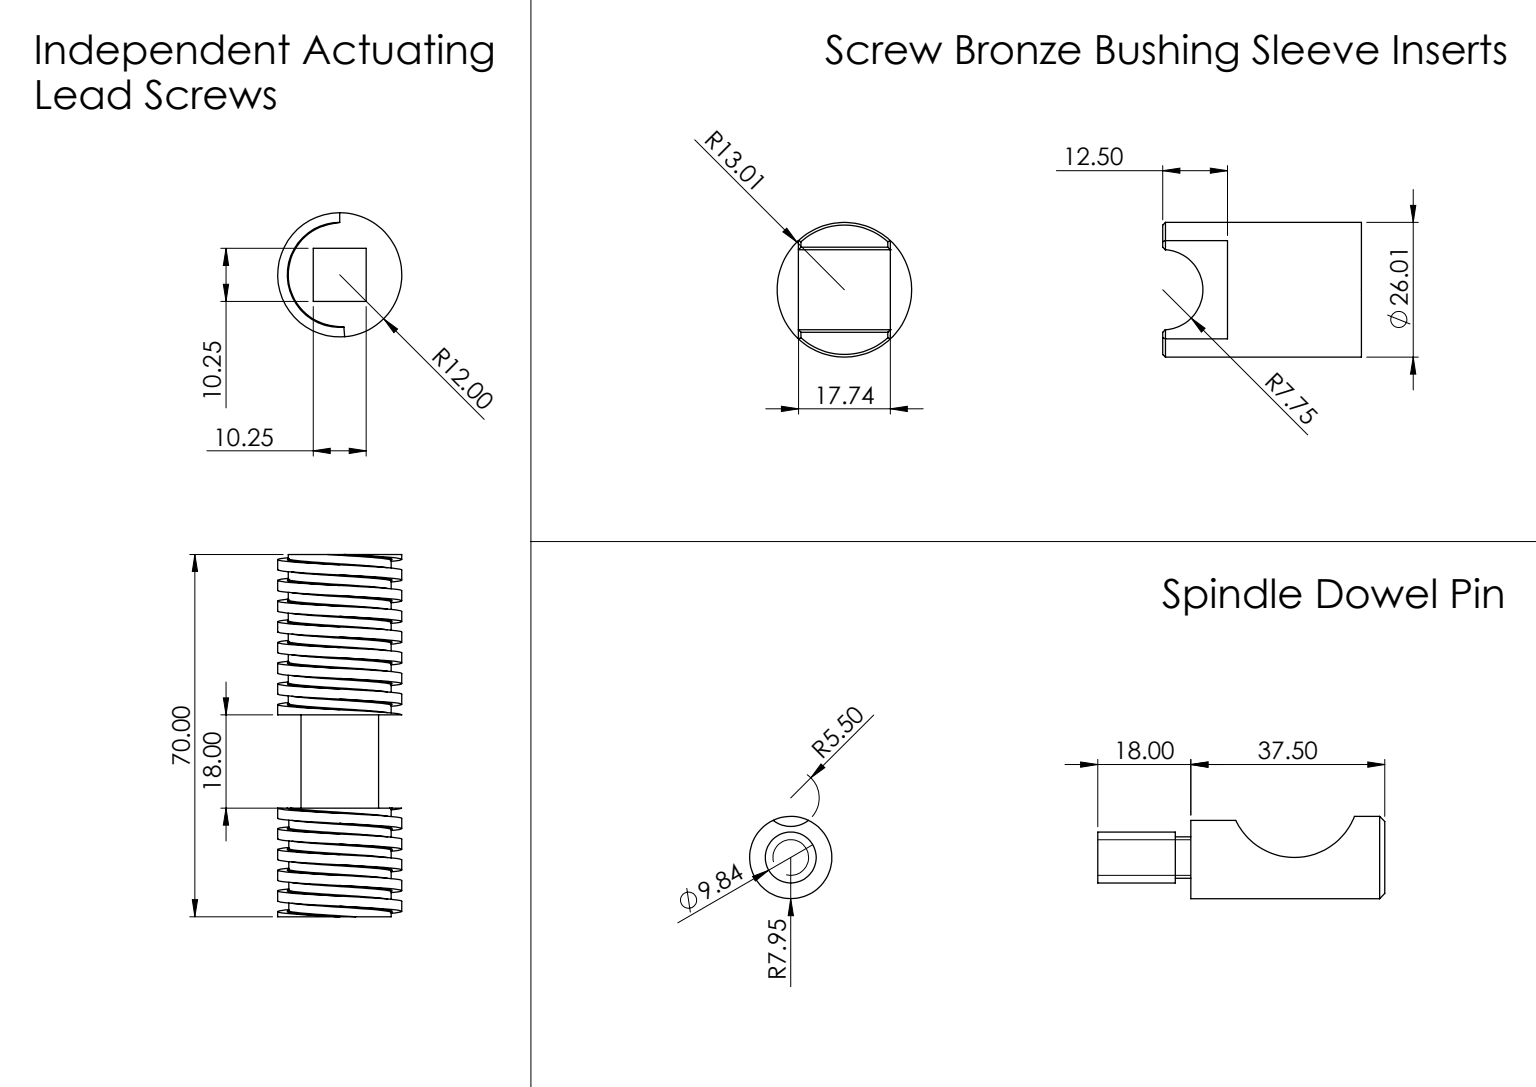
ISO-10303-21;
HEADER;
FILE_DESCRIPTION (('STEP AP214'),
    '1' );
FILE_NAME ('Independent Actuating Lead Screws.step',
    '2026-10-09T08:48:44',
    ( '' ),
    ( '' ),
    'SwSTEP 2.0',
    'SolidWorks 2026',
    '' );
FILE_SCHEMA (( 'AUTOMOTIVE_DESIGN' ));
ENDSEC;

DATA;
#1=( BOUNDED_CURVE ( )  B_SPLINE_CURVE ( 2, ( #10533, #60209, #55118, #80827, #73261, #48394, #10118, #21906, #55527, #48810, #23141, #53876, #74509 ),
 .UNSPECIFIED., .F., .F. ) 
 B_SPLINE_CURVE_WITH_KNOTS ( ( 3, 2, 2, 2, 2, 2, 3 ),
 ( 0.7124999999999999112, 0.7166666666666665630, 0.7208333333333332149, 0.7249999999999998668, 0.7291666666666665186, 0.7333333333333331705, 0.7374999999999999334 ),
 .UNSPECIFIED. ) 
 CURVE ( )  GEOMETRIC_REPRESENTATION_ITEM ( )  RATIONAL_B_SPLINE_CURVE ( ( 1.000000000000000888, 0.9659258262890674240, 1.000000000000000000, 0.9659258262890683122, 1.000000000000000000, 0.9659258262890683122, 1.000000000000000000, 0.9659258262890683122, 1.000000000000000000, 0.9659258262890683122, 1.000000000000000000, 0.9659258262890692004, 0.9999999999999991118 ) ) 
 REPRESENTATION_ITEM ( '' )  );
#2=CARTESIAN_POINT ( 'NONE',  ( 0.3392501089628018329, 0.1958661417322835607, -1.790682414698162805 ) ) ;
#8=CARTESIAN_POINT ( 'NONE',  ( 0.4091458600556403535, 0.2362204724409449896, -1.625328083989501460 ) ) ;
#11=CARTESIAN_POINT ( 'NONE',  ( 0.3949938075777409408, -0.1058382717557499186, -1.133202099737532720 ) ) ;
#20=CARTESIAN_POINT ( 'NONE',  ( 0.1070741851644053388, 0.3996062992125986035, -1.959973753280839892 ) ) ;
#23=CARTESIAN_POINT ( 'NONE',  ( -0.1958661417322834497, -0.3392501089628018884, -1.562972810202412521 ) ) ;
#34=CARTESIAN_POINT ( 'NONE',  ( 0.3996062992125986035, -0.1070741851644052972, -0.03083989501312336262 ) ) ;
#36=CARTESIAN_POINT ( 'NONE',  ( 0.1958661417322836440, -0.3392501089628017219, -0.9639107611548557442 ) ) ;
#40=DIRECTION ( 'NONE',  ( 0.000000000000000000, 0.000000000000000000, 1.000000000000000000 ) ) ;
#45=CARTESIAN_POINT ( 'NONE',  ( 0.4091458600556404646, -0.2362204724409448231, -2.624671916010498762 ) ) ;
#52=CARTESIAN_POINT ( 'NONE',  ( 0.4724409448818898682, 2.892866454678787531E-17, -2.322834645669291209 ) ) ;
#56=CARTESIAN_POINT ( 'NONE',  ( 0.2867679344610366554, -0.2867679344610365444, -2.610236220472440749 ) ) ;
#59=CARTESIAN_POINT ( 'NONE',  ( 5.785732909357575061E-17, -0.4724409448818898682, -0.3937007874015748254 ) ) ;
#60=CARTESIAN_POINT ( 'NONE',  ( -0.1070741851644051862, -0.3996062992125987146, -0.07217847769028871985 ) ) ;
#63=CARTESIAN_POINT ( 'NONE',  ( -0.1049643490035302024, -0.3917322834645671215, -1.796587926509185973 ) ) ;
#64=EDGE_LOOP ( 'NONE', ( #43919, #18024, #48228, #40467 ) ) ;
#66=CARTESIAN_POINT ( 'NONE',  ( -0.4724409448818898682, -8.678599364036362592E-17, -2.716535433070865757 ) ) ;
#74=CARTESIAN_POINT ( 'NONE',  ( 4.797336870675655290E-17, -0.3917322834645669549, -0.9461749099399457963 ) ) ;
#81=CARTESIAN_POINT ( 'NONE',  ( 0.1049643490035304799, -0.3917322834645670104, -2.444245037566615597 ) ) ;
#89=CARTESIAN_POINT ( 'NONE',  ( -0.1049643490035302024, -0.3917322834645671215, -1.416666666666666519 ) ) ;
#104=CARTESIAN_POINT ( 'NONE',  ( -0.3392501089628019995, 0.1958661417322832277, -1.213254593175852936 ) ) ;
#105=CARTESIAN_POINT ( 'NONE',  ( -0.4091458600556405756, 0.2362204724409446288, -0.1030183727034120617 ) ) ;
#108=CARTESIAN_POINT ( 'NONE',  ( 0.2891555358219910499, 0.2891555358219910499, 0.1003937007874015630 ) ) ;
#113=CARTESIAN_POINT ( 'NONE',  ( -0.3949938075777409963, -7.255918531996591613E-17, 0.04133858267716533641 ) ) ;
#120=CARTESIAN_POINT ( 'NONE',  ( -9.787531504996566615E-17, 0.3996062992125985480, -0.7066929133858268486 ) ) ;
#122=CARTESIAN_POINT ( 'NONE',  ( -0.3392501089628017219, -0.1958661417322836718, -0.6745406824146981117 ) ) ;
#124=DIRECTION ( 'NONE',  ( 1.000000000000000000, 0.000000000000000000, -0.000000000000000000 ) ) ;
#139=CARTESIAN_POINT ( 'NONE',  ( -0.2362204724409447953, -0.4091458600556404646, -2.347112860892388575 ) ) ;
#159=CARTESIAN_POINT ( 'NONE',  ( 0.1070741851644053666, 0.3996062992125986035, -0.4658792650918635037 ) ) ;
#160=CARTESIAN_POINT ( 'NONE',  ( -0.1070741851644051862, -0.3996062992125986590, -2.668635170603674833 ) ) ;
#165=CARTESIAN_POINT ( 'NONE',  ( 0.2925321140481932369, 0.2925321140481932369, -2.342519685039369914 ) ) ;
#166=CARTESIAN_POINT ( 'NONE',  ( 0.3420746716998660508, -0.1974969037888703871, -1.994750656167979086 ) ) ;
#167=CARTESIAN_POINT ( 'NONE',  ( -0.3917322834645671215, 0.1049643490035301469, -0.4973753280839895430 ) ) ;
#168=CARTESIAN_POINT ( 'NONE',  ( -1.157146581871515012E-16, 0.4724409448818898682, -2.519685039370078705 ) ) ;
#169=CARTESIAN_POINT ( 'NONE',  ( 0.1049643490035304799, -0.3917322834645669549, -0.8648293963254591876 ) ) ;
#172=CARTESIAN_POINT ( 'NONE',  ( -0.3420746716998662729, 0.1974969037888702206, -2.780183727034121866 ) ) ;
#177=CARTESIAN_POINT ( 'NONE',  ( 0.2362204724409451007, -0.4091458600556402980, -2.769028871391076230 ) ) ;
#178=CARTESIAN_POINT ( 'NONE',  ( 0.2925321140481932369, 0.2925321140481932369, -2.185039370078739829 ) ) ;
#179=CARTESIAN_POINT ( 'NONE',  ( -0.3392501089628017219, -0.1958661417322836995, -0.8366334890101857491 ) ) ;
#185=CARTESIAN_POINT ( 'NONE',  ( -0.2867679344610364334, -0.2867679344610367109, -0.1437007874015748810 ) ) ;
#194=CARTESIAN_POINT ( 'NONE',  ( -0.3917322834645670104, -7.196005306013484475E-17, -0.7539370078740157410 ) ) ;
#195=CARTESIAN_POINT ( 'NONE',  ( 0.3917322834645669549, 0.1049643490035304660, -1.691601049868766360 ) ) ;
#196=CARTESIAN_POINT ( 'NONE',  ( -0.3917322834645671215, 0.1049643490035301469, -2.859580052493438274 ) ) ;
#198=CARTESIAN_POINT ( 'NONE',  ( -0.2925321140481930704, -0.2925321140481933480, -0.2165354330708662012 ) ) ;
#202=CARTESIAN_POINT ( 'NONE',  ( -0.3996062992125986035, -0.1070741851644056997, -1.620734908136482799 ) ) ;
#204=CARTESIAN_POINT ( 'NONE',  ( -0.4724409448818899238, 0.1265901696524986964, -2.471784776902886893 ) ) ;
#207=CARTESIAN_POINT ( 'NONE',  ( 0.3392501089628018884, -0.1958661417322834220, -0.6620734908136483021 ) ) ;
#216=CARTESIAN_POINT ( 'NONE',  ( -0.2362204724409447953, -0.4091458600556404646, -2.112860892388451539 ) ) ;
#223=ADVANCED_FACE ( 'NONE', ( #9541 ), #47687, .T. ) ;
#224=CARTESIAN_POINT ( 'NONE',  ( 0.3458507752293908943, -0.3458507752293908943, -2.537401574803149984 ) ) ;
#228=CARTESIAN_POINT ( 'NONE',  ( -0.3917322834645669549, -7.196005306013483243E-17, -0.7493245162391581893 ) ) ;
#231=CARTESIAN_POINT ( 'NONE',  ( 0.1958661417322836440, -0.3392501089628017219, -0.9639107611548557442 ) ) ;
#236=CARTESIAN_POINT ( 'NONE',  ( -0.3392501089628017219, -0.1958661417322836718, -2.879265091863516979 ) ) ;
#240=CARTESIAN_POINT ( 'NONE',  ( -1.157146581871515012E-16, 0.4724409448818898682, -1.021653543307086576 ) ) ;
#253=CARTESIAN_POINT ( 'NONE',  ( -0.3996062992125984925, -0.1070741851644056858, -2.484908136482939955 ) ) ;
#257=CARTESIAN_POINT ( 'NONE',  ( 0.1070741851644053388, 0.3996062992125986035, -1.330052493438320438 ) ) ;
#263=CARTESIAN_POINT ( 'NONE',  ( -0.2925321140481930149, -0.2925321140481933480, -0.7657480314960628531 ) ) ;
#264=CARTESIAN_POINT ( 'NONE',  ( 0.1998031496062994405, -0.3460692066303958092, -0.8792650918635170898 ) ) ;
#265=CARTESIAN_POINT ( 'NONE',  ( 0.3420746716998659953, 0.1974969037888705536, -0.2887139107611549349 ) ) ;
#271=CARTESIAN_POINT ( 'NONE',  ( -0.1974969037888704149, -0.3420746716998661063, -1.244750656167979086 ) ) ;
#276=CARTESIAN_POINT ( 'NONE',  ( -0.3458507752293906723, -0.3458507752293910609, -1.633858267716534973 ) ) ;
#277=CARTESIAN_POINT ( 'NONE',  ( 4.893765752498283924E-17, -0.3996062992125986035, -2.598425196850393970 ) ) ;
#284=CARTESIAN_POINT ( 'NONE',  ( -9.594673741351310580E-17, 0.3917322834645669549, -1.969796957184039909 ) ) ;
#285=CARTESIAN_POINT ( 'NONE',  ( -9.787531504996566615E-17, 0.3996062992125985480, -2.753937007874015741 ) ) ;
#290=CARTESIAN_POINT ( 'NONE',  ( -0.1958661417322834220, -0.3392501089628018884, -1.317585301837270295 ) ) ;
#293=CARTESIAN_POINT ( 'NONE',  ( 0.1974969037888704704, 0.3420746716998660508, -2.034120734908136718 ) ) ;
#298=CARTESIAN_POINT ( 'NONE',  ( -0.1998031496062994683, 0.3460692066303958092, -0.3280839895013123453 ) ) ;
#306=CARTESIAN_POINT ( 'NONE',  ( 0.1049643490035303689, 0.3917322834645670104, -0.5505249343832020470 ) ) ;
#314=CARTESIAN_POINT ( 'NONE',  ( 0.2925321140481932369, -0.2925321140481931814, -2.064960629921259283 ) ) ;
#320=CARTESIAN_POINT ( 'NONE',  ( -0.3458507752293906723, -0.3458507752293910609, -0.8464566929133857665 ) ) ;
#322=CARTESIAN_POINT ( 'NONE',  ( -0.1049643490035302024, -0.3917322834645671215, -0.2217847769028870319 ) ) ;
#323=CARTESIAN_POINT ( 'NONE',  ( 0.3808816823641231752, -0.09156050430092187165, -1.929133858267716661 ) ) ;
#327=CARTESIAN_POINT ( 'NONE',  ( 0.2362204724409451007, -0.4091458600556402980, -2.845800524934383624 ) ) ;
#331=CARTESIAN_POINT ( 'NONE',  ( -0.1058382717557497660, -0.3949938075777411073, -2.668635170603674833 ) ) ;
#339=CARTESIAN_POINT ( 'NONE',  ( 0.2867679344610365999, -0.2867679344610365444, -1.350393700787401619 ) ) ;
#342=CARTESIAN_POINT ( 'NONE',  ( -0.1265901696524993347, 0.4724409448818895907, 0.2316272965879264956 ) ) ;
#354=CARTESIAN_POINT ( 'NONE',  ( 0.3996062992125985480, 2.446882876249141654E-17, -0.9822834645669291653 ) ) ;
#355=CARTESIAN_POINT ( 'NONE',  ( 0.1049643490035303689, 0.3917322834645670104, -2.597769028871390606 ) ) ;
#365=CARTESIAN_POINT ( 'NONE',  ( -0.3996062992125987146, 0.1070741851644051862, 0.1246719160104986790 ) ) ;
#367=CARTESIAN_POINT ( 'NONE',  ( -0.3917322834645670659, -7.196005306013484475E-17, -1.925872334154542509 ) ) ;
#373=CARTESIAN_POINT ( 'NONE',  ( 0.1049643490035303689, 0.3917322834645670104, -1.810367454068241511 ) ) ;
#380=CARTESIAN_POINT ( 'NONE',  ( 0.1998031496062992740, 0.3460692066303959757, -1.404199475065616820 ) ) ;
#382=CARTESIAN_POINT ( 'NONE',  ( 4.797336870675656522E-17, -0.3917322834645670659, 0.08200168159348891761 ) ) ;
#395=CARTESIAN_POINT ( 'NONE',  ( 0.2867679344610365999, -0.2867679344610365444, -0.2480314960629920740 ) ) ;
#398=CARTESIAN_POINT ( 'NONE',  ( -0.3420746716998661618, 0.1974969037888702206, -0.6561679790026245795 ) ) ;
#400=VERTEX_POINT ( 'NONE', #34658 ) ;
#407=CARTESIAN_POINT ( 'NONE',  ( 0.3392501089628018884, -0.1958661417322833942, -1.519048187172915343 ) ) ;
#414=CARTESIAN_POINT ( 'NONE',  ( -0.1070741851644056997, 0.3996062992125986035, -1.266404199475065440 ) ) ;
#416=CARTESIAN_POINT ( 'NONE',  ( 0.1998031496062994128, -0.3460692066303957537, -0.6410761154855643129 ) ) ;
#417=CARTESIAN_POINT ( 'NONE',  ( -0.3460692066303957537, -0.1998031496062994405, -0.2867454068241469534 ) ) ;
#419=CARTESIAN_POINT ( 'NONE',  ( -0.3460692066303960868, 0.1998031496062990242, -2.860892388451443669 ) ) ;
#420=CARTESIAN_POINT ( 'NONE',  ( 0.2867679344610365999, 0.2867679344610365999, -2.269685039370078705 ) ) ;
#426=CARTESIAN_POINT ( 'NONE',  ( -0.4724409448818898682, -8.678599364036362592E-17, -1.375984251968503713 ) ) ;
#430=CARTESIAN_POINT ( 'NONE',  ( 0.1058382717557500852, -0.3949938075777408852, -1.264435695538058013 ) ) ;
#440=CARTESIAN_POINT ( 'NONE',  ( 0.1070741851644053388, 0.3996062992125986035, -2.274934383202099397 ) ) ;
#442=CARTESIAN_POINT ( 'NONE',  ( 0.2867679344610365999, 0.2867679344610365999, -1.477670972932071614 ) ) ;
#450=CARTESIAN_POINT ( 'NONE',  ( 0.1265901696524989184, 0.4724409448818898127, -2.355643044619422533 ) ) ;
#453=CARTESIAN_POINT ( 'NONE',  ( 0.2925321140481932369, -0.2925321140481931814, -0.01771653543307087630 ) ) ;
#455=CARTESIAN_POINT ( 'NONE',  ( 0.1049643490035304938, -0.3917322834645669549, -1.272309711286089273 ) ) ;
#464=CARTESIAN_POINT ( 'NONE',  ( -0.4724409448818898682, 5.785732909357575061E-17, -2.755905511811024056 ) ) ;
#476=CARTESIAN_POINT ( 'NONE',  ( 0.1049643490035303689, 0.3917322834645670104, -2.505249343832020692 ) ) ;
#479=CARTESIAN_POINT ( 'NONE',  ( -0.3458507752293909498, 0.3458507752293907833, -0.8070866141732284671 ) ) ;
#480=CARTESIAN_POINT ( 'NONE',  ( -0.2925321140481930704, -0.2925321140481933480, 0.09842519685039367860 ) ) ;
#484=CARTESIAN_POINT ( 'NONE',  ( -0.3917322834645671215, 0.1049643490035301469, -1.757217847769028340 ) ) ;
#488=CARTESIAN_POINT ( 'NONE',  ( -0.1265901696524986964, -0.4724409448818899238, -2.906824146981627610 ) ) ;
#495=CARTESIAN_POINT ( 'NONE',  ( -0.1958661417322834497, -0.3392501089628018884, -1.248012180281152794 ) ) ;
#503=ORIENTED_EDGE ( 'NONE', *, *, #38239, .F. ) ;
#504=CARTESIAN_POINT ( 'NONE',  ( 0.1958661417322834775, 0.3392501089628018884, -2.503300155676852157 ) ) ;
#513=CARTESIAN_POINT ( 'NONE',  ( -0.1958661417322834220, -0.3392501089628018884, -1.725065616797900381 ) ) ;
#524=ORIENTED_EDGE ( 'NONE', *, *, #54320, .F. ) ;
#528=CARTESIAN_POINT ( 'NONE',  ( 0.000000000000000000, 0.000000000000000000, -0.3937007874015748254 ) ) ;
#529=CARTESIAN_POINT ( 'NONE',  ( 0.3458507752293908943, -0.3458507752293908943, -0.1751968503937007537 ) ) ;
#532=CARTESIAN_POINT ( 'NONE',  ( 4.837279021331061486E-17, -0.3949938075777409963, -0.3129921259842520231 ) ) ;
#538=CARTESIAN_POINT ( 'NONE',  ( 0.1058382717557500852, -0.3949938075777408852, -0.004593175853018378711 ) ) ;
#545=CARTESIAN_POINT ( 'NONE',  ( 4.893765752498283308E-17, -0.3996062992125985480, -0.7854330708661416693 ) ) ;
#547=CARTESIAN_POINT ( 'NONE',  ( -0.2867679344610365999, 0.2867679344610364889, -0.7992125984251968740 ) ) ;
#563=CARTESIAN_POINT ( 'NONE',  ( 0.1265901696524989462, 0.4724409448818897572, -2.274934383202099397 ) ) ;
#579=CARTESIAN_POINT ( 'NONE',  ( 4.893765752498283924E-17, -0.3996062992125986035, -0.2362204724409449341 ) ) ;
#580=CARTESIAN_POINT ( 'NONE',  ( -0.4724409448818898682, -8.678599364036362592E-17, -1.218503937007874072 ) ) ;
#584=CARTESIAN_POINT ( 'NONE',  ( -0.1070741851644056997, 0.3996062992125986035, -2.526246719160104792 ) ) ;
#585=CARTESIAN_POINT ( 'NONE',  ( -0.3949938075777409963, -7.255918531996591613E-17, -2.086614173228346303 ) ) ;
#586=CARTESIAN_POINT ( 'NONE',  ( -9.594673741351313045E-17, 0.3917322834645670104, -0.6220472440944880832 ) ) ;
#589=CARTESIAN_POINT ( 'NONE',  ( -0.1958661417322834220, -0.3392501089628018884, -1.160104986876640210 ) ) ;
#591=CARTESIAN_POINT ( 'NONE',  ( -0.1049643490035307020, 0.3917322834645669549, -1.258530183727033958 ) ) ;
#593=CARTESIAN_POINT ( 'NONE',  ( -0.3917322834645668994, -0.1049643490035306742, 0.03151537877396508314 ) ) ;
#598=CARTESIAN_POINT ( 'NONE',  ( -0.4091458600556405756, 0.2362204724409446288, -2.860892388451443669 ) ) ;
#599=CARTESIAN_POINT ( 'NONE',  ( 0.3460692066303959757, -0.1998031496062991907, -2.624671916010498762 ) ) ;
#600=CARTESIAN_POINT ( 'NONE',  ( -0.3392501089628017219, -0.1958661417322836995, -1.151594118931445365 ) ) ;
#606=CARTESIAN_POINT ( 'NONE',  ( 0.1049643490035303689, 0.3917322834645670104, -0.07808398950131241467 ) ) ;
#614=CARTESIAN_POINT ( 'NONE',  ( -0.05870088567476314939, -0.3874523867754370854, -1.929133858267717549 ) ) ;
#615=CARTESIAN_POINT ( 'NONE',  ( -0.1958661417322834220, -0.3392501089628018884, -1.790026246719160330 ) ) ;
#616=CARTESIAN_POINT ( 'NONE',  ( 0.3392501089628018329, 0.1958661417322835607, -2.800524934383201714 ) ) ;
#618=CARTESIAN_POINT ( 'NONE',  ( -0.3996062992125986035, -0.1070741851644056997, -0.2034120734908136385 ) ) ;
#622=CARTESIAN_POINT ( 'NONE',  ( 0.1265901696524989184, 0.4724409448818898127, -2.432414698162729483 ) ) ;
#625=CARTESIAN_POINT ( 'NONE',  ( 0.3392501089628018884, -0.1958661417322834220, -0.8195538057742782767 ) ) ;
#645=CARTESIAN_POINT ( 'NONE',  ( 0.1958661417322836162, -0.3392501089628018329, -0.8018179545593683288 ) ) ;
#648=CARTESIAN_POINT ( 'NONE',  ( 0.4091458600556403535, 0.2362204724409449896, -0.7611548556430446366 ) ) ;
#649=( GEOMETRIC_REPRESENTATION_CONTEXT ( 3 ) GLOBAL_UNCERTAINTY_ASSIGNED_CONTEXT ( ( #13385 ) ) GLOBAL_UNIT_ASSIGNED_CONTEXT ( ( #28477, #67211, #3642 ) ) REPRESENTATION_CONTEXT ( 'NONE', 'WORKASPACE' ) );
#654=CARTESIAN_POINT ( 'NONE',  ( 0.1049643490035303689, 0.3917322834645670104, -2.662729658792650778 ) ) ;
#658=CARTESIAN_POINT ( 'NONE',  ( -0.2362204724409447953, -0.4091458600556404646, -1.087270341207349000 ) ) ;
#671=ORIENTED_EDGE ( 'NONE', *, *, #74772, .T. ) ;
#673=CARTESIAN_POINT ( 'NONE',  ( -0.1998031496062991630, -0.3460692066303959202, -2.504593175853018661 ) ) ;
#677=CARTESIAN_POINT ( 'NONE',  ( 0.3996062992125985480, 2.446882876249141654E-17, -1.769685039370078927 ) ) ;
#682=CARTESIAN_POINT ( 'NONE',  ( 0.3996062992125984925, 0.1070741851644054499, -1.146325459317585116 ) ) ;
#683=CARTESIAN_POINT ( 'NONE',  ( -0.3460692066303958092, -0.1998031496062994683, -1.469816272965879245 ) ) ;
#684=CARTESIAN_POINT ( 'NONE',  ( 0.3420746716998659953, 0.1974969037888705536, -0.6036745406824147731 ) ) ;
#690=CARTESIAN_POINT ( 'NONE',  ( -0.3949938075777411073, 0.1058382717557497660, -1.841863517060367661 ) ) ;
#695=CARTESIAN_POINT ( 'NONE',  ( 0.1265901696524989462, 0.4724409448818897572, -1.410761154855643129 ) ) ;
#703=CARTESIAN_POINT ( 'NONE',  ( 0.2867679344610365999, -0.2867679344610365999, -2.068222154034434546 ) ) ;
#710=CARTESIAN_POINT ( 'NONE',  ( 0.1958661417322836440, -0.3392501089628017219, -1.501312335958005173 ) ) ;
#713=CARTESIAN_POINT ( 'NONE',  ( -0.3420746716998661618, 0.1974969037888702206, -1.758530183727034180 ) ) ;
#719=CARTESIAN_POINT ( 'NONE',  ( -0.3996062992125986035, -0.1070741851644056997, -0.3608923884514435576 ) ) ;
#728=CARTESIAN_POINT ( 'NONE',  ( -0.2867679344610364334, -0.2867679344610367109, -0.4586614173228347746 ) ) ;
#735=EDGE_LOOP ( 'NONE', ( #48750, #68189, #51593, #70339 ) ) ;
#736=CARTESIAN_POINT ( 'NONE',  ( -0.1070741851644051862, -0.3996062992125986590, -2.038713910761154491 ) ) ;
#739=FACE_BOUND ( 'NONE', #72764, .T. ) ;
#740=CARTESIAN_POINT ( 'NONE',  ( -0.1265901696524993347, 0.4724409448818895907, -0.7939632545931758489 ) ) ;
#742=CARTESIAN_POINT ( 'NONE',  ( -0.3392501089628019995, 0.1958661417322832277, -0.3333333333333333148 ) ) ;
#747=CARTESIAN_POINT ( 'NONE',  ( -0.1998031496062994405, 0.3460692066303957537, 0.2250656167979002420 ) ) ;
#749=CARTESIAN_POINT ( 'NONE',  ( -0.3458507752293906723, -0.3458507752293910609, -1.080708661417322691 ) ) ;
#752=CARTESIAN_POINT ( 'NONE',  ( -0.2891555358219909388, -0.2891555358219912164, -2.498031496062992574 ) ) ;
#759=CARTESIAN_POINT ( 'NONE',  ( -0.2867679344610365999, 0.2867679344610364889, -1.586614173228346747 ) ) ;
#762=CARTESIAN_POINT ( 'NONE',  ( -0.4091458600556405756, 0.2362204724409446288, 0.2119422572178477626 ) ) ;
#775=CARTESIAN_POINT ( 'NONE',  ( -0.1998031496062994405, 0.3460692066303957537, -1.034776902887139194 ) ) ;
#776=CARTESIAN_POINT ( 'NONE',  ( 0.3917322834645670104, 2.398668435337828261E-17, -2.722440944881889369 ) ) ;
#788=CARTESIAN_POINT ( 'NONE',  ( -0.1958661417322836995, 0.3392501089628017219, -2.372066559876327307 ) ) ;
#795=CARTESIAN_POINT ( 'NONE',  ( -0.3392501089628019995, 0.1958661417322832277, -1.843175853018372834 ) ) ;
#800=CARTESIAN_POINT ( 'NONE',  ( -0.3996062992125985480, -7.340648628747423112E-17, -2.635826771653543066 ) ) ;
#802=CARTESIAN_POINT ( 'NONE',  ( -0.1070741851644056997, 0.3996062992125986035, -1.423884514435695525 ) ) ;
#804=CARTESIAN_POINT ( 'NONE',  ( 0.3917322834645670104, -0.1049643490035303411, -2.938320209973753538 ) ) ;
#818=CARTESIAN_POINT ( 'NONE',  ( 0.1958661417322834775, 0.3392501089628018884, -0.2939632545931757934 ) ) ;
#821=CARTESIAN_POINT ( 'NONE',  ( 0.2891555358219910499, 0.2891555358219910499, -0.7677165354330709457 ) ) ;
#839=CARTESIAN_POINT ( 'NONE',  ( 0.1998031496062994405, -0.3460692066303958092, -1.351706036745406792 ) ) ;
#841=CARTESIAN_POINT ( 'NONE',  ( 0.3996062992125986035, -0.1070741851644052972, -0.8182414698162727706 ) ) ;
#842=CARTESIAN_POINT ( 'NONE',  ( -0.2925321140481930149, -0.2925321140481933480, 0.02165354330708658959 ) ) ;
#844=CARTESIAN_POINT ( 'NONE',  ( 0.2925321140481932369, 0.2925321140481932369, -2.814960629921259727 ) ) ;
#846=CARTESIAN_POINT ( 'NONE',  ( -0.1958661417322836718, 0.3392501089628017219, -1.987532808398950079 ) ) ;
#852=CARTESIAN_POINT ( 'NONE',  ( 0.4724409448818898682, 2.892866454678787531E-17, -1.612204724409448842 ) ) ;
#855=CARTESIAN_POINT ( 'NONE',  ( -0.2891555358219911054, 0.2891555358219909388, -1.513779527559055094 ) ) ;
#865=CARTESIAN_POINT ( 'NONE',  ( 0.2925321140481932369, 0.2925321140481932369, -2.104330708661417582 ) ) ;
#867=CARTESIAN_POINT ( 'NONE',  ( 0.1049643490035303689, 0.3917322834645668994, -1.963235277394014267 ) ) ;
#879=CARTESIAN_POINT ( 'NONE',  ( 0.3460692066303959202, -0.1998031496062991630, -0.02427821522309711946 ) ) ;
#882=CARTESIAN_POINT ( 'NONE',  ( -0.3392501089628017219, -0.1958661417322836718, -1.554461942257217899 ) ) ;
#893=CARTESIAN_POINT ( 'NONE',  ( -0.4724409448818896462, -0.1265901696524993070, -2.565616797900262647 ) ) ;
#905=CARTESIAN_POINT ( 'NONE',  ( 0.1049643490035303689, 0.3917322834645670104, -2.662729658792650778 ) ) ;
#909=CARTESIAN_POINT ( 'NONE',  ( 0.3458507752293908943, -0.3458507752293908943, -0.5708661417322833387 ) ) ;
#910=CARTESIAN_POINT ( 'NONE',  ( -0.1998031496062991907, -0.3460692066303959757, -0.06561679790026248016 ) ) ;
#911=ORIENTED_EDGE ( 'NONE', *, *, #49585, .T. ) ;
#913=CARTESIAN_POINT ( 'NONE',  ( -0.2867679344610364334, -0.2867679344610367109, -1.625984251968503491 ) ) ;
#917=CARTESIAN_POINT ( 'NONE',  ( -0.2362204724409447953, -0.4091458600556404646, -2.900262467191600635 ) ) ;
#924=CARTESIAN_POINT ( 'NONE',  ( 0.1049643490035303689, 0.3917322834645668994, -1.333314017551494368 ) ) ;
#930=CARTESIAN_POINT ( 'NONE',  ( 0.1958661417322834775, 0.3392501089628018884, -2.345819840716222515 ) ) ;
#938=CARTESIAN_POINT ( 'NONE',  ( 0.3917322834645670104, 2.398668435337828261E-17, -1.777559055118110409 ) ) ;
#956=CARTESIAN_POINT ( 'NONE',  ( -0.1265901696524986964, -0.4724409448818899238, -0.1489501312335958227 ) ) ;
#959=CARTESIAN_POINT ( 'NONE',  ( -0.1058382717557497660, -0.3949938075777411073, 0.008530183727034110208 ) ) ;
#965=CARTESIAN_POINT ( 'NONE',  ( 0.3420746716998660508, 0.1974969037888705814, -0.05052493438320211638 ) ) ;
#972=CARTESIAN_POINT ( 'NONE',  ( -0.3996062992125985480, -7.340648628747423112E-17, -1.061023622047243986 ) ) ;
#974=CARTESIAN_POINT ( 'NONE',  ( 0.1049643490035304938, -0.3917322834645669549, -0.7073490813648293241 ) ) ;
#988=CARTESIAN_POINT ( 'NONE',  ( -1.157146581871515012E-16, 0.4724409448818898682, -2.281496062992125928 ) ) ;
#1003=CARTESIAN_POINT ( 'NONE',  ( 0.4724409448818898682, 2.892866454678787531E-17, -0.4330708661417322913 ) ) ;
#1005=CIRCLE ( 'NONE', #37280, 0.2952755905511810774 ) ;
#1006=CARTESIAN_POINT ( 'NONE',  ( 0.3996062992125986035, 2.446882876249141962E-17, -0.4330708661417322913 ) ) ;
#1011=CARTESIAN_POINT ( 'NONE',  ( -0.1070741851644051862, -0.3996062992125987146, -2.749343832020996636 ) ) ;
#1012=CARTESIAN_POINT ( 'NONE',  ( -0.3420746716998659953, -0.1974969037888706647, -2.099737532808398921 ) ) ;
#1013=CARTESIAN_POINT ( 'NONE',  ( -0.3392501089628017219, -0.1958661417322836718, -0.6745406824146981117 ) ) ;
#1015=CARTESIAN_POINT ( 'NONE',  ( -0.1958661417322836718, 0.3392501089628017219, -0.9501312335958004285 ) ) ;
#1017=CARTESIAN_POINT ( 'NONE',  ( -0.1049643490035307020, 0.3917322834645669549, -1.101049868766403872 ) ) ;
#1019=CARTESIAN_POINT ( 'NONE',  ( 4.797336870675655290E-17, -0.3917322834645669549, -0.001293020176166160412 ) ) ;
#1025=CARTESIAN_POINT ( 'NONE',  ( -0.3996062992125986035, -0.1070741851644056997, -2.723097112860892288 ) ) ;
#1026=CARTESIAN_POINT ( 'NONE',  ( 0.1958661417322834775, 0.3392501089628018884, -1.085977321031183163 ) ) ;
#1031=CARTESIAN_POINT ( 'NONE',  ( 0.3917322834645670104, -0.1049643490035303411, -0.5111548556430445256 ) ) ;
#1040=CARTESIAN_POINT ( 'NONE',  ( -0.3917322834645669549, -0.1049643490035306603, -1.927821522309711044 ) ) ;
#1041=ORIENTED_EDGE ( 'NONE', *, *, #25445, .F. ) ;
#1042=CARTESIAN_POINT ( 'NONE',  ( 0.2925321140481932369, -0.2925321140481932369, -0.09842519685039373412 ) ) ;
#1049=CARTESIAN_POINT ( 'NONE',  ( 0.3917322834645670104, -0.1049643490035303411, -0.6686351706036747222 ) ) ;
#1059=CARTESIAN_POINT ( 'NONE',  ( -0.3458507752293909498, 0.3458507752293908388, -2.696850393700787052 ) ) ;
#1060=CYLINDRICAL_SURFACE ( 'NONE', #55948, 0.4724409448818898682 ) ;
#1064=AXIS2_PLACEMENT_3D ( 'NONE', #67446, #9780, #68282 ) ;
#1070=CARTESIAN_POINT ( 'NONE',  ( 0.2867679344610365999, -0.2867679344610365999, -0.8083796343493945269 ) ) ;
#1073=CARTESIAN_POINT ( 'NONE',  ( -0.3676198365746922714, 0.1467283321115996353, -1.216801570222568740 ) ) ;
#1079=CARTESIAN_POINT ( 'NONE',  ( -9.594673741351313045E-17, 0.3917322834645670659, -0.1542187908474559610 ) ) ;
#1083=CARTESIAN_POINT ( 'NONE',  ( 0.1265901696524989462, 0.4724409448818897572, -1.330052493438320216 ) ) ;
#1098=CARTESIAN_POINT ( 'NONE',  ( -0.3460692066303957537, -0.1998031496062994405, -2.333989501312335957 ) ) ;
#1102=CARTESIAN_POINT ( 'NONE',  ( 0.2925321140481932369, 0.2925321140481932369, -1.631889763779527325 ) ) ;
#1108=CARTESIAN_POINT ( 'NONE',  ( 0.3996062992125985480, 2.446882876249141654E-17, -1.139763779527559029 ) ) ;
#1109=CARTESIAN_POINT ( 'NONE',  ( -0.3460692066303960868, 0.1998031496062990242, -1.443569553805774230 ) ) ;
#1110=CARTESIAN_POINT ( 'NONE',  ( 0.1974969037888706369, -0.3420746716998659953, -0.7217847769028871152 ) ) ;
#1116=CARTESIAN_POINT ( 'NONE',  ( 0.3949938075777408852, 0.1058382717557500435, -1.933727034120735100 ) ) ;
#1121=CARTESIAN_POINT ( 'NONE',  ( -0.4724409448818898682, -8.678599364036362592E-17, -1.929133858267716439 ) ) ;
#1122=VECTOR ( 'NONE', #79900, 39.37007874015748143 ) ;
#1129=CARTESIAN_POINT ( 'NONE',  ( 0.3917322834645669549, 2.398668435337827645E-17, -2.245387508365142892 ) ) ;
#1135=CARTESIAN_POINT ( 'NONE',  ( 0.3917322834645670104, -0.1049643490035303411, 0.1187664041994749703 ) ) ;
#1137=CARTESIAN_POINT ( 'NONE',  ( -0.1049643490035307020, 0.3917322834645669549, -2.045931758530183497 ) ) ;
#1140=CARTESIAN_POINT ( 'NONE',  ( -0.1974969037888706647, 0.3420746716998658843, -1.902887139107611869 ) ) ;
#1145=CARTESIAN_POINT ( 'NONE',  ( -9.787531504996567848E-17, 0.3996062992125986035, -0.6299212598425196763 ) ) ;
#1153=CARTESIAN_POINT ( 'NONE',  ( 0.2867679344610365999, -0.2867679344610365444, -0.3405511811023621549 ) ) ;
#1160=CARTESIAN_POINT ( 'NONE',  ( 4.893765752498283308E-17, -0.3996062992125985480, -2.202755905511811108 ) ) ;
#1165=CARTESIAN_POINT ( 'NONE',  ( -0.4724409448818898682, -8.678599364036362592E-17, -1.141732283464566899 ) ) ;
#1167=CARTESIAN_POINT ( 'NONE',  ( 0.3392501089628018329, 0.1958661417322835607, -0.1233595800524933811 ) ) ;
#1168=CARTESIAN_POINT ( 'NONE',  ( -0.2867679344610366554, 0.2867679344610365444, -2.624015748031495843 ) ) ;
#1172=CARTESIAN_POINT ( 'NONE',  ( -0.1070741851644051862, -0.3996062992125986590, -0.1489501312335958227 ) ) ;
#1177=CARTESIAN_POINT ( 'NONE',  ( -0.2891555358219909388, -0.2891555358219912164, -2.812992125984251857 ) ) ;
#1179=CARTESIAN_POINT ( 'NONE',  ( 0.3917322834645670104, 2.398668435337828261E-17, -0.2027559055118111353 ) ) ;
#1184=CARTESIAN_POINT ( 'NONE',  ( 0.3917322834645669549, 0.1049643490035304660, -1.849081364829396223 ) ) ;
#1188=CARTESIAN_POINT ( 'NONE',  ( 0.2362204724409451007, -0.4091458600556402980, 0.1463254593175852825 ) ) ;
#1192=CARTESIAN_POINT ( 'NONE',  ( 0.4091458600556403535, 0.2362204724409449896, -0.6804461942257218343 ) ) ;
#1201=CARTESIAN_POINT ( 'NONE',  ( 0.3996062992125984925, 0.1070741851644054637, -0.9888451443569553634 ) ) ;
#1202=CARTESIAN_POINT ( 'NONE',  ( -0.2867679344610365999, 0.2867679344610364889, -2.781496062992125040 ) ) ;
#1211=CARTESIAN_POINT ( 'NONE',  ( -0.1998031496062994683, 0.3460692066303958092, -0.1706036745406823985 ) ) ;
#1212=CARTESIAN_POINT ( 'NONE',  ( 0.3917322834645670104, 0.1049643490035304660, -2.483615116306773452 ) ) ;
#1219=CARTESIAN_POINT ( 'NONE',  ( 0.2867679344610365999, 0.2867679344610365999, -2.269685039370078705 ) ) ;
#1227=CARTESIAN_POINT ( 'NONE',  ( -0.3460692066303958092, -0.1998031496062994683, -1.469816272965879245 ) ) ;
#1228=ORIENTED_EDGE ( 'NONE', *, *, #71870, .F. ) ;
#1229=CARTESIAN_POINT ( 'NONE',  ( 0.1049643490035303967, 0.3917322834645670659, -0.1476571110574297074 ) ) ;
#1241=CARTESIAN_POINT ( 'NONE',  ( 4.797336870675656522E-17, -0.3917322834645670104, -0.2283464566929133410 ) ) ;
#1244=CARTESIAN_POINT ( 'NONE',  ( 0.3420746716998659953, 0.1974969037888705536, -0.6036745406824147731 ) ) ;
#1260=CARTESIAN_POINT ( 'NONE',  ( 0.1070741851644053527, 0.3996062992125986590, -1.410761154855643129 ) ) ;
#1262=CARTESIAN_POINT ( 'NONE',  ( -0.1070741851644056997, 0.3996062992125984925, -0.7132545931758530466 ) ) ;
#1263=CARTESIAN_POINT ( 'NONE',  ( -0.3460692066303960313, 0.1998031496062989965, -0.1030183727034120894 ) ) ;
#1265=CARTESIAN_POINT ( 'NONE',  ( 0.3460692066303959202, 0.1998031496062993295, -2.650918635170603554 ) ) ;
#1266=CARTESIAN_POINT ( 'NONE',  ( 0.3392501089628018329, 0.1958661417322835607, -1.948162729658792891 ) ) ;
#1272=CARTESIAN_POINT ( 'NONE',  ( 0.1265901696524989462, 0.4724409448818897572, -1.330052493438320216 ) ) ;
#1275=CARTESIAN_POINT ( 'NONE',  ( 0.3420746716998660508, -0.1974969037888704149, -1.284120734908136718 ) ) ;
#1285=CARTESIAN_POINT ( 'NONE',  ( -0.1070741851644051862, -0.3996062992125986590, -2.353674540682414662 ) ) ;
#1286=CARTESIAN_POINT ( 'NONE',  ( 0.2867679344610365999, -0.2867679344610365999, -1.910741839073804016 ) ) ;
#1299=CARTESIAN_POINT ( 'NONE',  ( -0.3996062992125985480, -7.340648628747423112E-17, 0.04133858267716534335 ) ) ;
#1301=CARTESIAN_POINT ( 'NONE',  ( 0.1049643490035304938, -0.3917322834645669549, -1.587270341207349222 ) ) ;
#1322=CARTESIAN_POINT ( 'NONE',  ( 0.2867679344610366554, 0.2867679344610366554, -2.334645669291338432 ) ) ;
#1325=CARTESIAN_POINT ( 'NONE',  ( 0.4724409448818897572, -0.1265901696524988906, -0.7414698162729659314 ) ) ;
#1326=CARTESIAN_POINT ( 'NONE',  ( 0.1070741851644053527, 0.3996062992125986590, 0.006561679790026227546 ) ) ;
#1329=CARTESIAN_POINT ( 'NONE',  ( 4.797336870675656522E-17, -0.3917322834645670104, -1.803149606299212726 ) ) ;
#1339=CARTESIAN_POINT ( 'NONE',  ( 4.797336870675655290E-17, -0.3917322834645669549, -1.103655224900575993 ) ) ;
#1346=CARTESIAN_POINT ( 'NONE',  ( 0.2867679344610366554, 0.2867679344610366554, -2.654218790847456155 ) ) ;
#1348=ORIENTED_EDGE ( 'NONE', *, *, #13593, .T. ) ;
#1354=CARTESIAN_POINT ( 'NONE',  ( 0.1049643490035303689, 0.3917322834645670104, -1.810367454068241511 ) ) ;
#1368=CARTESIAN_POINT ( 'NONE',  ( -0.3458507752293906723, -0.3458507752293910609, -0.4507874015748031815 ) ) ;
#1372=CARTESIAN_POINT ( 'NONE',  ( -0.3420746716998660508, -0.1974969037888706924, -0.1292650918635170898 ) ) ;
#1376=EDGE_CURVE ( 'NONE', #53683, #11079, #1562, .T. ) ;
#1377=CARTESIAN_POINT ( 'NONE',  ( 0.2891555358219910499, -0.2891555358219909944, 0.1397637795275590844 ) ) ;
#1383=CARTESIAN_POINT ( 'NONE',  ( -0.1998031496062994405, 0.3460692066303957537, -0.8772965879265091083 ) ) ;
#1385=CARTESIAN_POINT ( 'NONE',  ( 0.1049643490035304938, -0.3917322834645669549, -0.8648293963254591876 ) ) ;
#1397=CARTESIAN_POINT ( 'NONE',  ( -0.3951562584566667424, -0.01150853369506067876, -1.220472440945443493 ) ) ;
#1399=CARTESIAN_POINT ( 'NONE',  ( 0.4091458600556404646, -0.2362204724409448231, -2.858923884514435798 ) ) ;
#1406=CARTESIAN_POINT ( 'NONE',  ( 0.1265901696524989184, 0.4724409448818898127, -2.040682414698162361 ) ) ;
#1416=CARTESIAN_POINT ( 'NONE',  ( -0.1070741851644057135, 0.3996062992125985480, -0.9514435695538056015 ) ) ;
#1421=CARTESIAN_POINT ( 'NONE',  ( 0.1998031496062994405, -0.3460692066303958092, -2.611548556430446144 ) ) ;
#1422=CARTESIAN_POINT ( 'NONE',  ( 0.1974969037888706369, -0.3420746716998659953, -1.824146981627296382 ) ) ;
#1423=CARTESIAN_POINT ( 'NONE',  ( 0.1049643490035304938, -0.3917322834645669549, -0.7073490813648293241 ) ) ;
#1424=CARTESIAN_POINT ( 'NONE',  ( 0.3917322834645669549, 0.1049643490035304660, -1.061679790026246684 ) ) ;
#1426=CARTESIAN_POINT ( 'NONE',  ( -0.3917322834645671215, 0.1049643490035301469, -1.284776902887139194 ) ) ;
#1428=CARTESIAN_POINT ( 'NONE',  ( 0.2867679344610365999, -0.2867679344610365999, 0.1365022554143850153 ) ) ;
#1434=CARTESIAN_POINT ( 'NONE',  ( 0.1070741851644054915, -0.3996062992125986035, -2.762467191601049255 ) ) ;
#1435=CARTESIAN_POINT ( 'NONE',  ( 0.3917322834645670659, 2.398668435337828261E-17, -1.059730601871078148 ) ) ;
#1441=CARTESIAN_POINT ( 'NONE',  ( -0.1958661417322834220, -0.3392501089628018884, -0.6227034120734910028 ) ) ;
#1449=CARTESIAN_POINT ( 'NONE',  ( 0.4724409448818892576, 0.1265901696524997788, -0.5164041994750656617 ) ) ;
#1450=CARTESIAN_POINT ( 'NONE',  ( -0.1049643490035302024, -0.3917322834645671215, -1.796587926509185973 ) ) ;
#1452=CARTESIAN_POINT ( 'NONE',  ( 0.3460692066303959202, 0.1998031496062993295, -0.2887139107611548794 ) ) ;
#1459=CARTESIAN_POINT ( 'NONE',  ( 0.3392501089628018329, 0.1958661417322835607, -1.003280839895013266 ) ) ;
#1462=CARTESIAN_POINT ( 'NONE',  ( -0.3726288332202236653, -0.1208384647423932784, -1.929133858267952473 ) ) ;
#1481=CARTESIAN_POINT ( 'NONE',  ( 0.3917322834645668994, -0.1049643490035303134, -0.9789833088900768976 ) ) ;
#1484=CARTESIAN_POINT ( 'NONE',  ( -0.1049643490035307020, 0.3917322834645669549, -1.193569553805774230 ) ) ;
#1491=CARTESIAN_POINT ( 'NONE',  ( 0.2867679344610366554, -0.2867679344610365999, -0.09516367273721974829 ) ) ;
#1495=CARTESIAN_POINT ( 'NONE',  ( 0.4724409448818897572, -0.1265901696524988906, -1.448162729658792669 ) ) ;
#1504=CARTESIAN_POINT ( 'NONE',  ( 0.1265901696524989184, 0.4724409448818898127, -2.117454068241469756 ) ) ;
#1510=CARTESIAN_POINT ( 'NONE',  ( 0.1070741851644054776, -0.3996062992125984925, -2.681758530183727895 ) ) ;
#1515=CARTESIAN_POINT ( 'NONE',  ( -0.2925321140481932369, 0.2925321140481931259, -1.986220472440945128 ) ) ;
#1520=CARTESIAN_POINT ( 'NONE',  ( 0.3460692066303959202, -0.1998031496062991630, -0.9691601049868766582 ) ) ;
#1521=CARTESIAN_POINT ( 'NONE',  ( -9.787531504996567848E-17, 0.3996062992125986035, -1.417322834645669216 ) ) ;
#1522=CARTESIAN_POINT ( 'NONE',  ( 0.1058382717557499880, 0.3949938075777411073, -0.4658792650918635592 ) ) ;
#1527=CARTESIAN_POINT ( 'NONE',  ( -9.674558042662122972E-17, 0.3949938075777409963, -1.809055118110236560 ) ) ;
#1532=CARTESIAN_POINT ( 'NONE',  ( 0.1265901696524990294, -0.4724409448818896462, -1.975065616797900381 ) ) ;
#1539=CARTESIAN_POINT ( 'NONE',  ( 0.3392501089628018329, 0.1958661417322835052, -2.573471497866454794 ) ) ;
#1540=CARTESIAN_POINT ( 'NONE',  ( -0.3996062992125984925, -0.1070741851644056858, -2.799868766404198794 ) ) ;
#1546=CARTESIAN_POINT ( 'NONE',  ( -0.2867679344610366554, 0.2867679344610365444, -2.776883571357268821 ) ) ;
#1547=ADVANCED_FACE ( 'NONE', ( #6606 ), #64907, .T. ) ;
#1549=CARTESIAN_POINT ( 'NONE',  ( 0.3917322834645670104, 2.398668435337828261E-17, -2.000000000000000000 ) ) ;
#1552=CARTESIAN_POINT ( 'NONE',  ( 0.3420746716998660508, -0.1974969037888703871, -2.309711286089239035 ) ) ;
#1557=CARTESIAN_POINT ( 'NONE',  ( -0.3996062992125986035, -7.340648628747425578E-17, -0.5118110236220472231 ) ) ;
#1562=LINE ( 'NONE', #70580, #68456 ) ;
#1566=CARTESIAN_POINT ( 'NONE',  ( 0.3917322834645670104, -0.1049643490035303411, -0.5111548556430445256 ) ) ;
#1572=ORIENTED_EDGE ( 'NONE', *, *, #19166, .F. ) ;
#1577=CARTESIAN_POINT ( 'NONE',  ( 0.4091458600556403535, 0.2362204724409449896, -1.076115485564304475 ) ) ;
#1579=CARTESIAN_POINT ( 'NONE',  ( 4.797336870675656522E-17, -0.3917322834645670104, -0.3858267716535432879 ) ) ;
#1580=CARTESIAN_POINT ( 'NONE',  ( -0.1958661417322836718, 0.3392501089628017219, -2.459973753280839670 ) ) ;
#1583=CARTESIAN_POINT ( 'NONE',  ( 0.2925321140481932369, -0.2925321140481931814, 0.1397637795275590289 ) ) ;
#1588=CARTESIAN_POINT ( 'NONE',  ( 0.1058382717557499880, 0.3949938075777409408, -2.589895013123359124 ) ) ;
#1595=CARTESIAN_POINT ( 'NONE',  ( 0.1049643490035303689, 0.3917322834645670104, -1.875328083989501460 ) ) ;
#1598=CARTESIAN_POINT ( 'NONE',  ( -1.157146581871515012E-16, 0.4724409448818898682, -0.3917322834645669549 ) ) ;
#1610=CARTESIAN_POINT ( 'NONE',  ( -0.2925321140481932369, 0.2925321140481931259, -1.198818897637795367 ) ) ;
#1611=CARTESIAN_POINT ( 'NONE',  ( -0.1049643490035302024, -0.3917322834645671215, -2.519028871391075786 ) ) ;
#1620=CARTESIAN_POINT ( 'NONE',  ( 0.2925321140481932369, -0.2925321140481932369, -0.2559055118110235560 ) ) ;
#1621=CARTESIAN_POINT ( 'NONE',  ( -0.2867679344610367109, 0.2867679344610365444, -2.693588869587613566 ) ) ;
#1626=CARTESIAN_POINT ( 'NONE',  ( 4.797336870675656522E-17, -0.3917322834645670104, -2.525590551181102317 ) ) ;
#1631=CARTESIAN_POINT ( 'NONE',  ( 4.893765752498283924E-17, -0.3996062992125986035, -1.968503937007873850 ) ) ;
#1633=CARTESIAN_POINT ( 'NONE',  ( -0.3996062992125986035, -7.340648628747425578E-17, -1.771653543307086576 ) ) ;
#1635=CARTESIAN_POINT ( 'NONE',  ( 0.1049643490035304799, -0.3917322834645670104, -0.5544812580390570123 ) ) ;
#1649=CARTESIAN_POINT ( 'NONE',  ( -0.1958661417322836718, 0.3392501089628017219, -0.6351706036745405903 ) ) ;
#1652=CARTESIAN_POINT ( 'NONE',  ( 0.3420746716998660508, -0.1974969037888703871, -0.4199475065616798952 ) ) ;
#1653=ORIENTED_EDGE ( 'NONE', *, *, #51709, .F. ) ;
#1662=FACE_OUTER_BOUND ( 'NONE', #12098, .T. ) ;
#1667=CARTESIAN_POINT ( 'NONE',  ( -0.1070741851644051862, -0.3996062992125987146, -1.174540682414698001 ) ) ;
#1669=CARTESIAN_POINT ( 'NONE',  ( -0.3460692066303960313, 0.1998031496062989965, -0.5754593175853018883 ) ) ;
#1670=CARTESIAN_POINT ( 'NONE',  ( -0.2925321140481930149, -0.2925321140481933480, -0.6082677165354329896 ) ) ;
#1672=CARTESIAN_POINT ( 'NONE',  ( 0.3458507752293908943, -0.3458507752293908943, 0.05905511811023620578 ) ) ;
#1673=CARTESIAN_POINT ( 'NONE',  ( 0.1049643490035304938, -0.3917322834645669549, -1.902230971128608727 ) ) ;
#1679=CARTESIAN_POINT ( 'NONE',  ( -1.157146581871515012E-16, 0.4724409448818898682, -1.809055118110236560 ) ) ;
#1682=CARTESIAN_POINT ( 'NONE',  ( 4.837279021331061486E-17, -0.3949938075777409963, -1.572834645669291875 ) ) ;
#1693=CARTESIAN_POINT ( 'NONE',  ( 0.3996062992125986035, -0.1070741851644052972, -2.708005249343832688 ) ) ;
#1694=CARTESIAN_POINT ( 'NONE',  ( -0.1049643490035301746, -0.3917322834645670659, -1.884495119913699002 ) ) ;
#1708=CARTESIAN_POINT ( 'NONE',  ( 0.1070741851644054776, -0.3996062992125984925, -0.004593175853018378711 ) ) ;
#1710=CARTESIAN_POINT ( 'NONE',  ( 0.3392501089628018329, 0.1958661417322835607, -1.475721784776902856 ) ) ;
#1727=( BOUNDED_CURVE ( )  B_SPLINE_CURVE ( 2, ( #36399, #4412, #2768, #79802, #48608, #22118, #42290, #3177, #61664, #67987, #10332, #4005, #73479 ),
 .UNSPECIFIED., .F., .F. ) 
 B_SPLINE_CURVE_WITH_KNOTS ( ( 3, 2, 2, 2, 2, 2, 3 ),
 ( 0.2375000000000000167, 0.2416666666666666963, 0.2458333333333333204, 0.2500000000000000000, 0.2541666666666666519, 0.2583333333333333037, 0.2624999999999999556 ),
 .UNSPECIFIED. ) 
 CURVE ( )  GEOMETRIC_REPRESENTATION_ITEM ( )  RATIONAL_B_SPLINE_CURVE ( ( 0.9999999999999997780, 0.9659258262890685343, 1.000000000000000000, 0.9659258262890683122, 1.000000000000000000, 0.9659258262890683122, 1.000000000000000000, 0.9659258262890683122, 1.000000000000000000, 0.9659258262890683122, 1.000000000000000000, 0.9659258262890687563, 0.9999999999999995559 ) ) 
 REPRESENTATION_ITEM ( '' )  );
#1732=CARTESIAN_POINT ( 'NONE',  ( 0.1958661417322834775, 0.3392501089628018884, -2.341207349081364963 ) ) ;
#1735=CARTESIAN_POINT ( 'NONE',  ( 0.1998031496062994405, -0.3460692066303958092, -0.09186351706036746667 ) ) ;
#1738=CARTESIAN_POINT ( 'NONE',  ( 0.2867679344610365999, 0.2867679344610365999, -1.862204724409449064 ) ) ;
#1749=CARTESIAN_POINT ( 'NONE',  ( -9.594673741351310580E-17, 0.3917322834645669549, -1.182395382380890592 ) ) ;
#1755=CARTESIAN_POINT ( 'NONE',  ( 0.2867679344610366554, 0.2867679344610366554, -2.496738475886826070 ) ) ;
#1763=CARTESIAN_POINT ( 'NONE',  ( -0.2867679344610365999, 0.2867679344610364889, -1.994094488188976610 ) ) ;
#1767=CYLINDRICAL_SURFACE ( 'NONE', #31510, 0.4724409448818898682 ) ;
#1772=CARTESIAN_POINT ( 'NONE',  ( 0.3996062992125986590, -0.1070741851644053111, -2.001312335958005395 ) ) ;
#1777=CARTESIAN_POINT ( 'NONE',  ( 0.4724409448818898682, 2.892866454678787531E-17, -0.6673228346456693272 ) ) ;
#1780=CARTESIAN_POINT ( 'NONE',  ( 0.1974969037888706092, -0.3420746716998660508, -0.01115485564304462274 ) ) ;
#1785=CARTESIAN_POINT ( 'NONE',  ( -0.1058382717557497660, -0.3949938075777411073, -0.4639107611548556331 ) ) ;
#1792=CARTESIAN_POINT ( 'NONE',  ( 0.2925321140481932369, -0.2925321140481931814, -0.9625984251968502381 ) ) ;
#1794=CARTESIAN_POINT ( 'NONE',  ( -0.1958661417322834220, -0.3392501089628018884, -0.6876640419947506189 ) ) ;
#1809=CARTESIAN_POINT ( 'NONE',  ( 0.3996062992125985480, 2.446882876249141654E-17, 0.1200787401574802959 ) ) ;
#1816=CARTESIAN_POINT ( 'NONE',  ( -0.4724409448818898682, -8.678599364036362592E-17, -2.086614173228346303 ) ) ;
#1827=CARTESIAN_POINT ( 'NONE',  ( 0.1070741851644053666, 0.3996062992125986035, -0.6233595800524933672 ) ) ;
#1832=EDGE_CURVE ( 'NONE', #2851, #40183, #25750, .T. ) ;
#1833=CARTESIAN_POINT ( 'NONE',  ( -0.3460692066303958092, -0.1998031496062994683, -2.414698162729658648 ) ) ;
#1834=CARTESIAN_POINT ( 'NONE',  ( -0.3420746716998661618, 0.1974969037888702206, -1.758530183727034180 ) ) ;
#1835=CARTESIAN_POINT ( 'NONE',  ( 0.3917322834645669549, 0.1049643490035304660, -0.7467191601049868455 ) ) ;
#1839=CARTESIAN_POINT ( 'NONE',  ( 4.797336870675656522E-17, -0.3917322834645670104, -1.015748031496062964 ) ) ;
#1841=CARTESIAN_POINT ( 'NONE',  ( 0.1049643490035303689, 0.3917322834645668994, -0.07347149786645487679 ) ) ;
#1846=CARTESIAN_POINT ( 'NONE',  ( -0.4724409448818898682, -8.678599364036362592E-17, -0.1161417322834645827 ) ) ;
#1847=CARTESIAN_POINT ( 'NONE',  ( 0.1998031496062994405, -0.3460692066303958092, -2.611548556430446144 ) ) ;
#1848=CARTESIAN_POINT ( 'NONE',  ( -0.1958661417322833942, -0.3392501089628018884, -1.322197793472127625 ) ) ;
#1853=CARTESIAN_POINT ( 'NONE',  ( -0.3917322834645670104, -7.196005306013484475E-17, -0.4389763779527560139 ) ) ;
#1861=LINE ( 'NONE', #14911, #80277 ) ;
#1863=CARTESIAN_POINT ( 'NONE',  ( -0.1958661417322836718, 0.3392501089628017219, -1.895013123359580165 ) ) ;
#1865=CARTESIAN_POINT ( 'NONE',  ( -0.1070741851644051862, -0.3996062992125987146, -0.3871391076115485719 ) ) ;
#1870=CARTESIAN_POINT ( 'NONE',  ( -0.03178304480585582292, 0.3983403474834776858, -2.755905511811024500 ) ) ;
#1872=CARTESIAN_POINT ( 'NONE',  ( -0.3917322834645670104, -7.196005306013484475E-17, -1.383858267716535417 ) ) ;
#1894=CARTESIAN_POINT ( 'NONE',  ( 0.3392501089628018329, -0.1958661417322834497, -1.129901944060680563 ) ) ;
#1897=CARTESIAN_POINT ( 'NONE',  ( 0.1265901696524989184, 0.4724409448818898127, -0.7808398950131233418 ) ) ;
#1903=CARTESIAN_POINT ( 'NONE',  ( -0.3917322834645671770, 0.1049643490035302024, -0.1870271897975872011 ) ) ;
#1906=CARTESIAN_POINT ( 'NONE',  ( -0.1265901696524993347, 0.4724409448818895907, -1.815616797900262425 ) ) ;
#1915=FACE_OUTER_BOUND ( 'NONE', #60545, .T. ) ;
#1922=CARTESIAN_POINT ( 'NONE',  ( -0.3949938075777409963, -7.255918531996591613E-17, 0.1988188976377952832 ) ) ;
#1927=CARTESIAN_POINT ( 'NONE',  ( 0.3460692066303959202, -0.1998031496062991630, -1.914041994750656395 ) ) ;
#1932=CARTESIAN_POINT ( 'NONE',  ( -0.3996062992125986035, 0.1070741851644051584, -1.211942257217847541 ) ) ;
#1934=CARTESIAN_POINT ( 'NONE',  ( 0.3996062992125986035, 2.446882876249141962E-17, -1.535433070866141669 ) ) ;
#1936=CARTESIAN_POINT ( 'NONE',  ( -0.1058382717557503211, 0.3949938075777409408, -0.7939632545931760710 ) ) ;
#1941=CARTESIAN_POINT ( 'NONE',  ( 0.1974969037888706092, -0.3420746716998660508, -1.900918635170603554 ) ) ;
#1945=CARTESIAN_POINT ( 'NONE',  ( -0.1265901696524986964, -0.4724409448818899238, -2.119422572178477626 ) ) ;
#1946=CARTESIAN_POINT ( 'NONE',  ( 0.3874523867751310524, -0.05870088567678984764, -2.755905511811023612 ) ) ;
#1952=CARTESIAN_POINT ( 'NONE',  ( -0.1049643490035306742, 0.3917322834645668994, -2.448799581855955587 ) ) ;
#1958=CARTESIAN_POINT ( 'NONE',  ( -0.1958661417322834497, -0.3392501089628018884, -2.665335014926823121 ) ) ;
#1960=CARTESIAN_POINT ( 'NONE',  ( -0.1958661417322836718, 0.3392501089628017219, -2.052493438320210029 ) ) ;
#1963=CARTESIAN_POINT ( 'NONE',  ( 4.837279021331060870E-17, -0.3949938075777409963, -2.125984251968503713 ) ) ;
#1968=CARTESIAN_POINT ( 'NONE',  ( 0.1998031496062992740, 0.3460692066303959757, -0.7742782152230971437 ) ) ;
#1972=CARTESIAN_POINT ( 'NONE',  ( -0.3917322834645670104, -7.196005306013484475E-17, 0.03346456692913377107 ) ) ;
#1974=CARTESIAN_POINT ( 'NONE',  ( 0.1049643490035304938, -0.3917322834645669549, -0.6423884514435697080 ) ) ;
#1980=CARTESIAN_POINT ( 'NONE',  ( 0.1049643490035303689, 0.3917322834645670104, 0.01443569553805778768 ) ) ;
#1986=CARTESIAN_POINT ( 'NONE',  ( 0.3458507752293908943, -0.3458507752293908943, -1.358267716535433101 ) ) ;
#1988=CARTESIAN_POINT ( 'NONE',  ( -0.3917322834645670104, -7.196005306013484475E-17, -0.5039370078740157410 ) ) ;
#1989=CARTESIAN_POINT ( 'NONE',  ( 0.2867679344610366554, -0.2867679344610365444, -2.545275590551181022 ) ) ;
#1992=CARTESIAN_POINT ( 'NONE',  ( 0.3996062992125985480, 2.446882876249141654E-17, 0.1200787401574802959 ) ) ;
#1997=VECTOR ( 'NONE', #9942, 39.37007874015748143 ) ;
#1998=CARTESIAN_POINT ( 'NONE',  ( -0.1049643490035306742, 0.3917322834645668994, 0.2283657724747524265 ) ) ;
#2000=CARTESIAN_POINT ( 'NONE',  ( -0.3917322834645670104, -7.196005306013484475E-17, -0.1240157480314961758 ) ) ;
#2005=CARTESIAN_POINT ( 'NONE',  ( -0.3917322834645671215, 0.1049643490035301469, -1.757217847769028340 ) ) ;
#2009=CARTESIAN_POINT ( 'NONE',  ( -0.2362204724409451284, 0.4091458600556402425, -0.4048556430446194621 ) ) ;
#2021=CARTESIAN_POINT ( 'NONE',  ( -0.2925321140481932369, 0.2925321140481931259, -1.356299212598425230 ) ) ;
#2023=CARTESIAN_POINT ( 'NONE',  ( 0.2867679344610365999, 0.2867679344610365999, -2.584645669291338876 ) ) ;
#2031=CARTESIAN_POINT ( 'NONE',  ( -0.2925321140481930704, -0.2925321140481933480, 0.09842519685039367860 ) ) ;
#2032=CARTESIAN_POINT ( 'NONE',  ( -0.1958661417322836995, 0.3392501089628017219, -2.529546874836956949 ) ) ;
#2038=CARTESIAN_POINT ( 'NONE',  ( -0.1049643490035307020, 0.3917322834645669549, -2.295931758530183497 ) ) ;
#2047=CARTESIAN_POINT ( 'NONE',  ( -0.1958661417322833942, -0.3392501089628018884, -0.2198355887477184134 ) ) ;
#2060=CARTESIAN_POINT ( 'NONE',  ( -0.2867679344610365999, 0.2867679344610364889, -0.6417322834645668994 ) ) ;
#2062=ORIENTED_EDGE ( 'NONE', *, *, #29607, .F. ) ;
#2063=CARTESIAN_POINT ( 'NONE',  ( 0.3949938075777411073, -0.1058382717557499464, -1.213910761154855633 ) ) ;
#2080=CARTESIAN_POINT ( 'NONE',  ( -0.1998031496062991907, -0.3460692066303959757, -1.325459317585301777 ) ) ;
#2082=CARTESIAN_POINT ( 'NONE',  ( 0.2925321140481932369, 0.2925321140481932369, -1.001968503937007871 ) ) ;
#2083=CARTESIAN_POINT ( 'NONE',  ( 0.1998031496062994128, -0.3460692066303957537, -0.4835958005249343938 ) ) ;
#2085=CARTESIAN_POINT ( 'NONE',  ( -0.2362204724409447953, -0.4091458600556404646, 0.09186351706036745279 ) ) ;
#2086=CARTESIAN_POINT ( 'NONE',  ( 0.3917322834645670104, -0.1049643490035303411, -2.243438320209974357 ) ) ;
#2092=CARTESIAN_POINT ( 'NONE',  ( 0.4724409448818897572, -0.1265901696524988906, -1.763123359580051952 ) ) ;
#2095=CARTESIAN_POINT ( 'NONE',  ( -0.2891555358219911054, 0.2891555358219909388, -1.198818897637795589 ) ) ;
#2105=CARTESIAN_POINT ( 'NONE',  ( 0.1998031496062992463, 0.3460692066303959202, -2.583333333333333481 ) ) ;
#2106=CARTESIAN_POINT ( 'NONE',  ( 0.3917322834645669549, 2.398668435337827645E-17, -2.087907193404512363 ) ) ;
#2116=CARTESIAN_POINT ( 'NONE',  ( -0.2362204724409447953, -0.4091458600556404646, -0.8530183727034120755 ) ) ;
#2119=CARTESIAN_POINT ( 'NONE',  ( -0.2925321140481930149, -0.2925321140481933480, -0.4507874015748031815 ) ) ;
#2122=CARTESIAN_POINT ( 'NONE',  ( -0.1049643490035307020, 0.3917322834645669549, -1.508530183727033736 ) ) ;
#2131=CARTESIAN_POINT ( 'NONE',  ( -0.2925321140481930149, -0.2925321140481933480, -1.080708661417322691 ) ) ;
#2137=CARTESIAN_POINT ( 'NONE',  ( 0.3992723400743284912, 9.133324503354010218E-17, -1.220472440944882164 ) ) ;
#2143=CARTESIAN_POINT ( 'NONE',  ( -0.3917322834645671215, 0.1049643490035301469, -2.702099737532808188 ) ) ;
#2147=CARTESIAN_POINT ( 'NONE',  ( 0.3996062992125986035, 2.446882876249141962E-17, -0.4330708661417322913 ) ) ;
#2150=CARTESIAN_POINT ( 'NONE',  ( -0.1958661417322834220, -0.3392501089628018884, -2.104986876640420057 ) ) ;
#2157=CARTESIAN_POINT ( 'NONE',  ( -0.2362204724409447953, -0.4091458600556404646, -2.032152230971128848 ) ) ;
#2162=CARTESIAN_POINT ( 'NONE',  ( 0.2867679344610365999, -0.2867679344610365999, -1.595781209152543845 ) ) ;
#2168=CARTESIAN_POINT ( 'NONE',  ( 4.837279021331060870E-17, -0.3949938075777409963, 0.07874015748031490403 ) ) ;
#2177=CARTESIAN_POINT ( 'NONE',  ( 0.3392501089628018329, 0.1958661417322835607, -1.633202099737532942 ) ) ;
#2181=FACE_OUTER_BOUND ( 'NONE', #64280, .T. ) ;
#2186=CARTESIAN_POINT ( 'NONE',  ( 0.1998031496062992740, 0.3460692066303959757, -2.034120734908136718 ) ) ;
#2192=CARTESIAN_POINT ( 'NONE',  ( 0.1265901696524990294, -0.4724409448818896462, -0.7919947506561679784 ) ) ;
#2195=CARTESIAN_POINT ( 'NONE',  ( 0.3420746716998660508, -0.1974969037888704149, -0.1817585301837270073 ) ) ;
#2200=CARTESIAN_POINT ( 'NONE',  ( 0.1058382717557499880, 0.3949938075777409408, -0.5426509186351705649 ) ) ;
#2204=CARTESIAN_POINT ( 'NONE',  ( -0.3458507752293906723, -0.3458507752293910609, -0.1358267716535432879 ) ) ;
#2207=CARTESIAN_POINT ( 'NONE',  ( -0.2925321140481930149, -0.2925321140481933480, -1.238188976377952999 ) ) ;
#2209=CARTESIAN_POINT ( 'NONE',  ( -9.594673741351313045E-17, 0.3917322834645670104, -0.9370078740157480324 ) ) ;
#2225=CARTESIAN_POINT ( 'NONE',  ( 0.4091458600556404646, -0.2362204724409448231, -2.701443569553806157 ) ) ;
#2232=CARTESIAN_POINT ( 'NONE',  ( -1.157146581871515012E-16, 0.4724409448818898682, -2.047244094488188892 ) ) ;
#2241=CARTESIAN_POINT ( 'NONE',  ( -0.2925321140481932369, 0.2925321140481931814, -0.6496062992125984925 ) ) ;
#2242=CARTESIAN_POINT ( 'NONE',  ( 0.4724409448818898682, 2.892866454678787531E-17, -0.5098425196850393526 ) ) ;
#2245=CARTESIAN_POINT ( 'NONE',  ( 0.2925321140481932369, -0.2925321140481932369, -2.460629921259842146 ) ) ;
#2246=CARTESIAN_POINT ( 'NONE',  ( 0.3949938075777409408, 0.1058382717557500574, -2.171916010498687655 ) ) ;
#2248=CARTESIAN_POINT ( 'NONE',  ( -0.1958661417322834220, -0.3392501089628018884, -0.8451443569553805935 ) ) ;
#2251=CARTESIAN_POINT ( 'NONE',  ( -0.1958661417322834220, -0.3392501089628018884, -1.160104986876640210 ) ) ;
#2254=CARTESIAN_POINT ( 'NONE',  ( 0.1049643490035304522, -0.3917322834645668994, 0.1496256149944375224 ) ) ;
#2261=CARTESIAN_POINT ( 'NONE',  ( 0.3996062992125986590, -0.1070741851644053111, -2.631233595800525293 ) ) ;
#2262=CARTESIAN_POINT ( 'NONE',  ( 0.3392501089628018884, -0.1958661417322833942, -1.361567872212285257 ) ) ;
#2270=CARTESIAN_POINT ( 'NONE',  ( -0.3392501089628019995, 0.1958661417322832277, -0.5833333333333334814 ) ) ;
#2278=CARTESIAN_POINT ( 'NONE',  ( 0.1584414948832921777, -0.3588842212252807418, -1.929133858267716883 ) ) ;
#2279=CARTESIAN_POINT ( 'NONE',  ( -0.1958661417322836718, 0.3392501089628017219, -2.052493438320210029 ) ) ;
#2280=ORIENTED_EDGE ( 'NONE', *, *, #7637, .T. ) ;
#2282=CARTESIAN_POINT ( 'NONE',  ( -0.2925321140481932924, 0.2925321140481931814, -0.3346456692913385988 ) ) ;
#2290=CARTESIAN_POINT ( 'NONE',  ( 0.1958661417322834775, 0.3392501089628018884, -1.331364829396325611 ) ) ;
#2300=CARTESIAN_POINT ( 'NONE',  ( 4.893765752498283308E-17, -0.3996062992125985480, -2.045275590551181466 ) ) ;
#2310=CARTESIAN_POINT ( 'NONE',  ( 0.1049643490035303689, 0.3917322834645668994, -1.333314017551494368 ) ) ;
#2313=CARTESIAN_POINT ( 'NONE',  ( 0.3392501089628018329, 0.1958661417322835607, -1.160761154855643129 ) ) ;
#2320=CARTESIAN_POINT ( 'NONE',  ( -0.3917322834645671770, 0.1049643490035302024, 0.1279334401236726371 ) ) ;
#2326=CARTESIAN_POINT ( 'NONE',  ( -1.157146581871515012E-16, 0.4724409448818898682, -1.494094488188976388 ) ) ;
#2327=AXIS2_PLACEMENT_3D ( 'NONE', #62752, #43773, #24838 ) ;
#2343=CARTESIAN_POINT ( 'NONE',  ( -0.2925321140481932369, 0.2925321140481931259, -2.616141732283464805 ) ) ;
#2348=CARTESIAN_POINT ( 'NONE',  ( -0.1070741851644056997, 0.3996062992125984925, -1.815616797900262425 ) ) ;
#2353=CARTESIAN_POINT ( 'NONE',  ( -0.3460692066303957537, -0.1998031496062994405, -0.9166666666666666297 ) ) ;
#2354=CARTESIAN_POINT ( 'NONE',  ( 0.2925321140481932369, -0.2925321140481932369, -1.358267716535433101 ) ) ;
#2355=CARTESIAN_POINT ( 'NONE',  ( 0.1974969037888704704, 0.3420746716998660508, -0.7742782152230970327 ) ) ;
#2356=CARTESIAN_POINT ( 'NONE',  ( 4.797336870675656522E-17, -0.3917322834645670104, -0.07086614173228342195 ) ) ;
#2360=CARTESIAN_POINT ( 'NONE',  ( -0.2891555358219909388, -0.2891555358219912164, -1.868110236220472009 ) ) ;
#2365=CARTESIAN_POINT ( 'NONE',  ( -0.3458507752293909498, 0.3458507752293907833, -2.224409448818897239 ) ) ;
#2366=CARTESIAN_POINT ( 'NONE',  ( 0.1988659768032885744, -0.3401783215957593365, -2.755905511811026276 ) ) ;
#2367=ORIENTED_EDGE ( 'NONE', *, *, #75384, .F. ) ;
#2373=CARTESIAN_POINT ( 'NONE',  ( 0.1049643490035303689, 0.3917322834645668994, -2.593156537236534387 ) ) ;
#2376=CARTESIAN_POINT ( 'NONE',  ( -0.4091458600556402980, -0.2362204724409451284, -2.414698162729658648 ) ) ;
#2380=CARTESIAN_POINT ( 'NONE',  ( 0.2867679344610365999, -0.2867679344610365999, -2.698143413876953556 ) ) ;
#2382=CARTESIAN_POINT ( 'NONE',  ( 0.3917322834645670104, -0.1049643490035303411, -1.993438320209974135 ) ) ;
#2385=CARTESIAN_POINT ( 'NONE',  ( 4.837279021331060870E-17, -0.3949938075777409963, -2.440944881889763884 ) ) ;
#2391=CARTESIAN_POINT ( 'NONE',  ( -9.787531504996567848E-17, 0.3996062992125986035, -0.4724409448818898127 ) ) ;
#2394=LINE ( 'NONE', #80257, #1997 ) ;
#2395=CARTESIAN_POINT ( 'NONE',  ( 0.02500110683995874009, -0.3941128856533797631, -2.755905511810075481 ) ) ;
#2396=CARTESIAN_POINT ( 'NONE',  ( 0.1049643490035304938, -0.3917322834645669549, -0.01246719160104995359 ) ) ;
#2402=CARTESIAN_POINT ( 'NONE',  ( -0.1958661417322836718, 0.3392501089628017219, -0.005249343832020952200 ) ) ;
#2406=DIRECTION ( 'NONE',  ( 0.000000000000000000, 0.000000000000000000, 1.000000000000000000 ) ) ;
#2407=CARTESIAN_POINT ( 'NONE',  ( -0.3458507752293906723, -0.3458507752293910609, -1.161417322834645383 ) ) ;
#2409=CARTESIAN_POINT ( 'NONE',  ( 0.3392501089628018884, -0.1958661417322834220, -0.7270341207349080292 ) ) ;
#2410=CARTESIAN_POINT ( 'NONE',  ( 0.1958661417322836440, -0.3392501089628017219, -2.381233595800524849 ) ) ;
#2413=CARTESIAN_POINT ( 'NONE',  ( 0.3460692066303959202, -0.1998031496062991630, 0.1332020997375328031 ) ) ;
#2419=CARTESIAN_POINT ( 'NONE',  ( 0.3917322834645668994, 0.1049643490035304522, 0.1102555362542800566 ) ) ;
#2421=CARTESIAN_POINT ( 'NONE',  ( 0.3917322834645669549, 0.1049643490035304660, -0.05183727034120743510 ) ) ;
#2427=CARTESIAN_POINT ( 'NONE',  ( -0.3392501089628017219, -0.1958661417322836718, -2.091863517060367439 ) ) ;
#2431=CARTESIAN_POINT ( 'NONE',  ( 0.3458507752293908943, -0.3458507752293908943, -0.4901574803149606474 ) ) ;
#2444=CARTESIAN_POINT ( 'NONE',  ( -0.2925321140481932369, 0.2925321140481931259, -1.671259842519685179 ) ) ;
#2454=CARTESIAN_POINT ( 'NONE',  ( -0.1070741851644051862, -0.3996062992125987146, -0.2296587926509186250 ) ) ;
#2455=CARTESIAN_POINT ( 'NONE',  ( -0.1049643490035302301, -0.3917322834645671770, -2.588601992947193509 ) ) ;
#2458=LINE ( 'NONE', #54186, #1122 ) ;
#2460=CARTESIAN_POINT ( 'NONE',  ( -0.3917322834645670104, -7.196005306013484475E-17, -2.486220472440944906 ) ) ;
#2465=CARTESIAN_POINT ( 'NONE',  ( 0.3460692066303959202, 0.1998031496062993295, -2.020997375328084100 ) ) ;
#2468=CARTESIAN_POINT ( 'NONE',  ( -0.2867679344610365444, -0.2867679344610367664, -0.5282345388789521090 ) ) ;
#2481=CARTESIAN_POINT ( 'NONE',  ( 0.2867679344610365999, -0.2867679344610365444, -0.4055118110236220486 ) ) ;
#2484=CARTESIAN_POINT ( 'NONE',  ( 0.1058382717557500713, -0.3949938075777409408, -0.8727034120734908917 ) ) ;
#2500=VERTEX_POINT ( 'NONE', #7271 ) ;
#2501=CARTESIAN_POINT ( 'NONE',  ( 0.3996062992125986035, 0.1070741851644054776, -1.856955380577427928 ) ) ;
#2503=CARTESIAN_POINT ( 'NONE',  ( -0.3460692066303960313, 0.1998031496062989965, -1.205380577427821454 ) ) ;
#2504=CARTESIAN_POINT ( 'NONE',  ( 0.1998031496062994128, -0.3460692066303957537, -0.6410761154855643129 ) ) ;
#2506=CARTESIAN_POINT ( 'NONE',  ( 0.1265901696524989462, 0.4724409448818897572, 0.006561679790026246628 ) ) ;
#2507=CARTESIAN_POINT ( 'NONE',  ( 0.2867679344610365999, 0.2867679344610365999, -2.427165354330708347 ) ) ;
#2513=CARTESIAN_POINT ( 'NONE',  ( -0.1265901696524993347, 0.4724409448818895907, -2.130577427821522374 ) ) ;
#2517=CARTESIAN_POINT ( 'NONE',  ( -0.1974969037888704149, -0.3420746716998661063, -2.032152230971128848 ) ) ;
#2527=CARTESIAN_POINT ( 'NONE',  ( -0.3460692066303957537, -0.1998031496062994405, -2.491469816272966042 ) ) ;
#2528=CARTESIAN_POINT ( 'NONE',  ( -0.2867679344610364334, -0.2867679344610368219, -1.871371760333646606 ) ) ;
#2540=CARTESIAN_POINT ( 'NONE',  ( -0.2925321140481932369, 0.2925321140481931259, -0.09645669291338582196 ) ) ;
#2542=CARTESIAN_POINT ( 'NONE',  ( -0.3917322834645671215, 0.1049643490035301469, -1.692257217847769057 ) ) ;
#2547=LINE ( 'NONE', #74080, #7790 ) ;
#2551=CARTESIAN_POINT ( 'NONE',  ( -0.3460692066303960313, 0.1998031496062989965, -0.8904199475065617264 ) ) ;
#2566=CARTESIAN_POINT ( 'NONE',  ( 0.1998031496062994405, -0.3460692066303958092, -0.4068241469816273326 ) ) ;
#2569=CARTESIAN_POINT ( 'NONE',  ( -0.2867679344610365999, 0.2867679344610364889, -2.216535433070866201 ) ) ;
#2570=VERTEX_POINT ( 'NONE', #45553 ) ;
#2576=CYLINDRICAL_SURFACE ( 'NONE', #22505, 0.4724409448818898682 ) ;
#2580=CARTESIAN_POINT ( 'NONE',  ( -0.2867679344610366554, 0.2867679344610365444, -1.674521366632859110 ) ) ;
#2586=CARTESIAN_POINT ( 'NONE',  ( 0.3917322834645670659, 2.398668435337828261E-17, -2.949494381398636733 ) ) ;
#2596=CARTESIAN_POINT ( 'NONE',  ( -0.3392501089628017219, -0.1958661417322836718, -2.026902887139107712 ) ) ;
#2603=CARTESIAN_POINT ( 'NONE',  ( 4.893765752498283308E-17, -0.3996062992125985480, 0.1594488188976377896 ) ) ;
#2605=CARTESIAN_POINT ( 'NONE',  ( -0.1070741851644056997, 0.3996062992125986035, -2.053805774278214979 ) ) ;
#2612=CARTESIAN_POINT ( 'NONE',  ( 0.4724409448818898682, 2.892866454678787531E-17, -0.5098425196850393526 ) ) ;
#2616=CARTESIAN_POINT ( 'NONE',  ( -0.2891555358219911054, 0.2891555358219909388, -0.5688976377952756902 ) ) ;
#2621=CARTESIAN_POINT ( 'NONE',  ( -0.1974969037888704149, -0.3420746716998661063, -0.4573490813648294906 ) ) ;
#2628=CARTESIAN_POINT ( 'NONE',  ( -0.3996062992125985480, -7.340648628747423112E-17, -1.533464566929134021 ) ) ;
#2630=CARTESIAN_POINT ( 'NONE',  ( -0.1049643490035307020, 0.3917322834645669549, -0.9435695538057740084 ) ) ;
#2631=CARTESIAN_POINT ( 'NONE',  ( 0.1265901696524990572, -0.4724409448818897017, -0.4770341207349080848 ) ) ;
#2640=CARTESIAN_POINT ( 'NONE',  ( -0.3458507752293909498, 0.3458507752293908388, -0.2539370078740156855 ) ) ;
#2642=CARTESIAN_POINT ( 'NONE',  ( -0.1070741851644051862, -0.3996062992125986590, 0.1660104986876640154 ) ) ;
#2659=CARTESIAN_POINT ( 'NONE',  ( 0.3996062992125986035, -0.1070741851644053111, -0.8989501312335956840 ) ) ;
#2663=CARTESIAN_POINT ( 'NONE',  ( -0.2362204724409451284, 0.4091458600556402425, 0.1443569553805774397 ) ) ;
#2664=CARTESIAN_POINT ( 'NONE',  ( 0.1058382717557499880, 0.3949938075777411073, -2.355643044619422533 ) ) ;
#2667=CARTESIAN_POINT ( 'NONE',  ( 0.1958661417322834775, 0.3392501089628018884, -0.9238845144356954142 ) ) ;
#2673=CARTESIAN_POINT ( 'NONE',  ( 0.3392501089628018329, -0.1958661417322834497, -0.4999806842181608868 ) ) ;
#2679=CARTESIAN_POINT ( 'NONE',  ( 0.2925321140481932369, 0.2925321140481932369, -2.814960629921259727 ) ) ;
#2680=CARTESIAN_POINT ( 'NONE',  ( 0.3392501089628018884, -0.1958661417322833942, -1.519048187172915343 ) ) ;
#2686=CARTESIAN_POINT ( 'NONE',  ( 0.1958661417322834775, 0.3392501089628018884, -0.8589238845144357981 ) ) ;
#2695=CARTESIAN_POINT ( 'NONE',  ( 0.3392501089628018884, -0.1958661417322834220, -2.459317585301837195 ) ) ;
#2703=CARTESIAN_POINT ( 'NONE',  ( 0.3917322834645670104, 2.398668435337828261E-17, -1.305118110236220375 ) ) ;
#2704=CARTESIAN_POINT ( 'NONE',  ( 0.3996062992125984925, 0.1070741851644054637, -2.091207349081364519 ) ) ;
#2712=CARTESIAN_POINT ( 'NONE',  ( 0.3460692066303958092, 0.1998031496062993018, -2.097769028871391050 ) ) ;
#2715=CARTESIAN_POINT ( 'NONE',  ( 0.3392501089628018329, 0.1958661417322835607, 0.03412073490813653104 ) ) ;
#2722=CARTESIAN_POINT ( 'NONE',  ( -0.3917322834645670659, 0.1049643490035301607, -1.215203781331021915 ) ) ;
#2732=CARTESIAN_POINT ( 'NONE',  ( 0.3392501089628018329, 0.1958661417322835607, -0.2854523866479808936 ) ) ;
#2737=CARTESIAN_POINT ( 'NONE',  ( 0.2362204724409451007, -0.4091458600556402980, -1.743438320209973469 ) ) ;
#2753=CARTESIAN_POINT ( 'NONE',  ( -0.1998031496062991630, -0.3460692066303959202, -2.662073490813648746 ) ) ;
#2759=CARTESIAN_POINT ( 'NONE',  ( -0.1070741851644051862, -0.3996062992125986590, -2.196194225721784576 ) ) ;
#2765=CARTESIAN_POINT ( 'NONE',  ( 0.1070741851644054915, -0.3996062992125986035, -1.975065616797900381 ) ) ;
#2766=CARTESIAN_POINT ( 'NONE',  ( -0.1974969037888703871, -0.3420746716998661063, -1.167979002624671914 ) ) ;
#2767=CARTESIAN_POINT ( 'NONE',  ( 0.2925321140481932369, -0.2925321140481932369, -2.618110236220472675 ) ) ;
#2768=CARTESIAN_POINT ( 'NONE',  ( 0.4091458600556403535, 0.2362204724409449896, -0.6036745406824146620 ) ) ;
#2769=CARTESIAN_POINT ( 'NONE',  ( -0.3917322834645670104, -7.196005306013484475E-17, -0.3464566929133857665 ) ) ;
#2773=CARTESIAN_POINT ( 'NONE',  ( 0.1974969037888704704, 0.3420746716998660508, -2.110892388451443225 ) ) ;
#2777=CARTESIAN_POINT ( 'NONE',  ( 0.4091458600556404646, -0.2362204724409448231, -1.994750656167979086 ) ) ;
#2778=CARTESIAN_POINT ( 'NONE',  ( 0.1324727617108047706, 0.3692639355350287866, -2.755905511811024944 ) ) ;
#2785=CARTESIAN_POINT ( 'NONE',  ( 0.2867679344610365999, -0.2867679344610365999, -2.225702468995064187 ) ) ;
#2788=CARTESIAN_POINT ( 'NONE',  ( -0.3458507752293906723, -0.3458507752293910609, -2.421259842519684735 ) ) ;
#2793=CARTESIAN_POINT ( 'NONE',  ( -9.594673741351313045E-17, 0.3917322834645670104, 0.07283464566929125084 ) ) ;
#2795=CARTESIAN_POINT ( 'NONE',  ( -0.3917322834645671215, 0.1049643490035301469, -1.757217847769028340 ) ) ;
#2797=VERTEX_POINT ( 'NONE', #53539 ) ;
#2798=CARTESIAN_POINT ( 'NONE',  ( 0.3949938075777409408, 0.1058382717557500574, -2.486876640419947382 ) ) ;
#2802=CARTESIAN_POINT ( 'NONE',  ( 0.1070741851644053527, 0.3996062992125986590, -0.4658792650918635592 ) ) ;
#2807=CARTESIAN_POINT ( 'NONE',  ( 0.3392501089628018884, -0.1958661417322834220, -0.1896325459317586282 ) ) ;
#2813=CARTESIAN_POINT ( 'NONE',  ( -0.2867679344610364334, -0.2867679344610367109, -0.05118110236220468900 ) ) ;
#2817=CARTESIAN_POINT ( 'NONE',  ( 0.2362204724409449064, 0.4091458600556404646, -1.246719160104986734 ) ) ;
#2820=CARTESIAN_POINT ( 'NONE',  ( 0.1049643490035304938, -0.3917322834645669549, -0.7073490813648293241 ) ) ;
#2821=CARTESIAN_POINT ( 'NONE',  ( 0.1958661417322836440, -0.3392501089628017219, -2.538713910761154491 ) ) ;
#2824=CARTESIAN_POINT ( 'NONE',  ( 0.2925321140481932369, 0.2925321140481932369, -0.2145669291338583029 ) ) ;
#2829=CARTESIAN_POINT ( 'NONE',  ( 0.1049643490035304522, -0.3917322834645668994, -0.007854699966192403571 ) ) ;
#2831=CARTESIAN_POINT ( 'NONE',  ( -0.2867679344610364334, -0.2867679344610367109, -0.3011811023622048000 ) ) ;
#2836=CARTESIAN_POINT ( 'NONE',  ( -9.594673741351313045E-17, 0.3917322834645670104, -1.724409448818897683 ) ) ;
#2840=CARTESIAN_POINT ( 'NONE',  ( 0.1265901696524989462, 0.4724409448818897572, -0.5426509186351704539 ) ) ;
#2851=VERTEX_POINT ( 'NONE', #40925 ) ;
#2852=CARTESIAN_POINT ( 'NONE',  ( -0.3460692066303957537, -0.1998031496062994405, -1.704068241469816058 ) ) ;
#2861=CARTESIAN_POINT ( 'NONE',  ( 0.1998031496062992740, 0.3460692066303959757, -0.3018372703412073310 ) ) ;
#2862=CARTESIAN_POINT ( 'NONE',  ( -0.3420746716998661618, 0.1974969037888702206, -0.02624671916010504202 ) ) ;
#2864=CARTESIAN_POINT ( 'NONE',  ( -0.01966910102760595011, -0.3928700489057011525, -1.862014699505723656E-17 ) ) ;
#2868=CARTESIAN_POINT ( 'NONE',  ( 0.3392501089628018329, 0.1958661417322835607, -2.420603674540682260 ) ) ;
#2873=CARTESIAN_POINT ( 'NONE',  ( -0.1265901696524986964, -0.4724409448818899238, -0.7020997375328084100 ) ) ;
#2878=CARTESIAN_POINT ( 'NONE',  ( 0.1049643490035304799, -0.3917322834645670104, -0.2395206281177972019 ) ) ;
#2885=EDGE_CURVE ( 'NONE', #60134, #49144, #47453, .T. ) ;
#2892=CARTESIAN_POINT ( 'NONE',  ( -0.1049643490035307020, 0.3917322834645669549, -0.6286089238845143923 ) ) ;
#2895=CARTESIAN_POINT ( 'NONE',  ( 0.3420746716998660508, -0.1974969037888703871, -0.8923884514435694859 ) ) ;
#2912=CARTESIAN_POINT ( 'NONE',  ( 4.893765752498283924E-17, -0.3996062992125986035, -1.653543307086614123 ) ) ;
#2915=CARTESIAN_POINT ( 'NONE',  ( -0.2925321140481930149, -0.2925321140481933480, -1.238188976377952999 ) ) ;
#2916=CARTESIAN_POINT ( 'NONE',  ( -0.3996062992125984925, -0.1070741851644056858, -0.5951443569553805935 ) ) ;
#2919=CARTESIAN_POINT ( 'NONE',  ( -0.3458507752293906723, -0.3458507752293910609, 0.09842519685039372024 ) ) ;
#2920=CARTESIAN_POINT ( 'NONE',  ( -0.1049643490035302024, -0.3917322834645671215, -2.519028871391075786 ) ) ;
#2926=CARTESIAN_POINT ( 'NONE',  ( -0.4091458600556405756, 0.2362204724409446288, -1.992782152230971437 ) ) ;
#2929=CARTESIAN_POINT ( 'NONE',  ( -0.3949938075777409963, -7.255918531996591613E-17, -1.848425196850393970 ) ) ;
#2932=CYLINDRICAL_SURFACE ( 'NONE', #72948, 0.2952755905511810774 ) ;
#2938=CARTESIAN_POINT ( 'NONE',  ( -0.3460692066303957537, -0.1998031496062994405, -2.648950131233595684 ) ) ;
#2939=CARTESIAN_POINT ( 'NONE',  ( 0.3917322834645668994, 0.1049643490035304522, -2.409429503115799065 ) ) ;
#2948=CARTESIAN_POINT ( 'NONE',  ( 0.3458507752293908943, -0.3458507752293908943, -0.8858267716535431768 ) ) ;
#2951=CARTESIAN_POINT ( 'NONE',  ( 0.3460692066303958092, 0.1998031496062993018, -0.3654855643044619407 ) ) ;
#2953=CARTESIAN_POINT ( 'NONE',  ( -0.2867679344610364334, -0.2867679344610367109, -1.875984251968503935 ) ) ;
#2962=CARTESIAN_POINT ( 'NONE',  ( 0.3996062992125985480, 2.446882876249141654E-17, -0.9822834645669291653 ) ) ;
#2969=CARTESIAN_POINT ( 'NONE',  ( 0.3960428127060660608, 0.01218835185196203222, -1.220472440944882386 ) ) ;
#2978=CARTESIAN_POINT ( 'NONE',  ( 0.1998031496062994405, -0.3460692066303958092, -0.5643044619422572516 ) ) ;
#2981=CARTESIAN_POINT ( 'NONE',  ( -0.1049643490035302024, -0.3917322834645671215, -2.426509186351705427 ) ) ;
#2988=CARTESIAN_POINT ( 'NONE',  ( -0.4724409448818914226, -0.1265901696524962816, -2.012467191601050143 ) ) ;
#2991=CARTESIAN_POINT ( 'NONE',  ( 4.797336870675655290E-17, -0.3917322834645669549, -1.576096169782465140 ) ) ;
#2997=CARTESIAN_POINT ( 'NONE',  ( 0.3420746716998659953, 0.1974969037888705536, 0.02624671916010492753 ) ) ;
#3006=CARTESIAN_POINT ( 'NONE',  ( -0.3392501089628017219, -0.1958661417322836718, -2.341863517060367439 ) ) ;
#3015=CARTESIAN_POINT ( 'NONE',  ( -0.2925321140481930704, -0.2925321140481933480, -1.791338582677165059 ) ) ;
#3020=CARTESIAN_POINT ( 'NONE',  ( 0.1265901696524990294, -0.4724409448818896462, -0.6345144356955381149 ) ) ;
#3023=CARTESIAN_POINT ( 'NONE',  ( 0.1058382717557499880, 0.3949938075777409408, -0.3851706036745406458 ) ) ;
#3029=CARTESIAN_POINT ( 'NONE',  ( -0.1058382717557503072, 0.3949938075777408852, -0.5557742782152231831 ) ) ;
#3037=CARTESIAN_POINT ( 'NONE',  ( 0.3996062992125985480, 2.446882876249141654E-17, -1.297244094488189115 ) ) ;
#3039=CARTESIAN_POINT ( 'NONE',  ( -0.3392501089628017219, -0.1958661417322836718, -1.146981627296587813 ) ) ;
#3041=CARTESIAN_POINT ( 'NONE',  ( -0.2661962643026954400, 0.2881610400590603471, -1.506228638669167268E-17 ) ) ;
#3053=CARTESIAN_POINT ( 'NONE',  ( -0.4091458600556402980, -0.2362204724409451284, -0.2867454068241469534 ) ) ;
#3067=CARTESIAN_POINT ( 'NONE',  ( -0.2925321140481930704, -0.2925321140481933480, -0.8464566929133857665 ) ) ;
#3072=CARTESIAN_POINT ( 'NONE',  ( -0.4724409448818898682, -8.678599364036362592E-17, 0.1181102362204724532 ) ) ;
#3073=CARTESIAN_POINT ( 'NONE',  ( 0.2891555358219910499, -0.2891555358219909944, -2.460629921259842590 ) ) ;
#3077=CARTESIAN_POINT ( 'NONE',  ( -0.1049643490035302024, -0.3917322834645671215, -1.166666666666666519 ) ) ;
#3085=CARTESIAN_POINT ( 'NONE',  ( -0.1049643490035301746, -0.3917322834645670659, -0.1522116553467698086 ) ) ;
#3091=CARTESIAN_POINT ( 'NONE',  ( 0.1998031496062992740, 0.3460692066303959757, -2.821522309711286258 ) ) ;
#3092=CARTESIAN_POINT ( 'NONE',  ( -0.2867679344610365444, -0.2867679344610367664, -1.630596743603361265 ) ) ;
#3098=CARTESIAN_POINT ( 'NONE',  ( 0.3392501089628018884, -0.1958661417322834220, -0.8195538057742782767 ) ) ;
#3107=CARTESIAN_POINT ( 'NONE',  ( -9.594673741351313045E-17, 0.3917322834645670104, -2.511811023622047223 ) ) ;
#3112=CARTESIAN_POINT ( 'NONE',  ( 0.000000000000000000, 0.000000000000000000, -2.755905511811024056 ) ) ;
#3115=CARTESIAN_POINT ( 'NONE',  ( -0.1958661417322834220, -0.3392501089628018884, -1.095144356955380704 ) ) ;
#3116=CARTESIAN_POINT ( 'NONE',  ( 0.3460692066303958092, 0.1998031496062993018, -2.412729658792650778 ) ) ;
#3118=CIRCLE ( 'NONE', #50133, 0.2952755905511810774 ) ;
#3128=CARTESIAN_POINT ( 'NONE',  ( 4.797336870675656522E-17, -0.3917322834645670104, 0.08661417322834649712 ) ) ;
#3136=CARTESIAN_POINT ( 'NONE',  ( -0.3392501089628019439, 0.1958661417322832554, -1.051161786580365742 ) ) ;
#3146=CARTESIAN_POINT ( 'NONE',  ( 0.3917322834645670104, 0.1049643490035304660, -0.4363710218185846146 ) ) ;
#3148=CARTESIAN_POINT ( 'NONE',  ( 0.2362204724409451007, -0.4091458600556402980, -0.2493438320209973857 ) ) ;
#3149=CARTESIAN_POINT ( 'NONE',  ( 0.4091458600556404646, -0.2362204724409448231, -1.756561679790026309 ) ) ;
#3162=CARTESIAN_POINT ( 'NONE',  ( 0.000000000000000000, 0.000000000000000000, -2.755905511811024056 ) ) ;
#3169=CARTESIAN_POINT ( 'NONE',  ( -0.1998031496062991630, -0.3460692066303959202, -2.347112860892388575 ) ) ;
#3174=CARTESIAN_POINT ( 'NONE',  ( -0.1070741851644051862, -0.3996062992125987146, -1.804461942257217677 ) ) ;
#3175=CARTESIAN_POINT ( 'NONE',  ( -0.1058382717557503211, 0.3949938075777409408, -1.108923884514435798 ) ) ;
#3176=CARTESIAN_POINT ( 'NONE',  ( 0.2925321140481932369, -0.2925321140481932369, -2.303149606299212060 ) ) ;
#3177=CARTESIAN_POINT ( 'NONE',  ( -0.1265901696524993347, 0.4724409448818896462, -0.6364829396325458744 ) ) ;
#3179=CARTESIAN_POINT ( 'NONE',  ( 4.797336870675656522E-17, -0.3917322834645670104, -0.3858267716535432879 ) ) ;
#3183=CARTESIAN_POINT ( 'NONE',  ( -0.1058382717557497660, -0.3949938075777411073, -2.038713910761155379 ) ) ;
#3187=CARTESIAN_POINT ( 'NONE',  ( 0.4091458600556404646, -0.2362204724409448231, -2.624671916010498762 ) ) ;
#3188=CARTESIAN_POINT ( 'NONE',  ( -0.1070741851644056997, 0.3996062992125986035, -1.896325459317584894 ) ) ;
#3196=CARTESIAN_POINT ( 'NONE',  ( 0.1958661417322836440, -0.3392501089628017219, 0.1384514435695537171 ) ) ;
#3199=CARTESIAN_POINT ( 'NONE',  ( 0.4724409448818898127, -0.1265901696524988629, -2.473753280839894764 ) ) ;
#3204=CARTESIAN_POINT ( 'NONE',  ( 0.1958661417322836440, -0.3392501089628017219, -0.01902887139107619849 ) ) ;
#3207=CARTESIAN_POINT ( 'NONE',  ( -0.3917322834645670104, -7.196005306013484475E-17, -2.236220472440944906 ) ) ;
#3210=CARTESIAN_POINT ( 'NONE',  ( -0.1058382717557497937, -0.3949938075777411628, -2.119422572178478070 ) ) ;
#3214=CARTESIAN_POINT ( 'NONE',  ( -0.2925321140481932924, 0.2925321140481931814, -1.122047244094488194 ) ) ;
#3219=CARTESIAN_POINT ( 'NONE',  ( 0.1049643490035304938, -0.3917322834645669549, 0.1450131233595799429 ) ) ;
#3228=DIRECTION ( 'NONE',  ( 0.000000000000000000, 0.000000000000000000, 1.000000000000000000 ) ) ;
#3229=CARTESIAN_POINT ( 'NONE',  ( 0.2362204724409449064, 0.4091458600556404646, -1.876640419947506411 ) ) ;
#3231=ADVANCED_FACE ( 'NONE', ( #37078 ), #31584, .T. ) ;
#3232=CARTESIAN_POINT ( 'NONE',  ( 0.3917322834645670104, -0.1049643490035303411, -0.7335958005249343383 ) ) ;
#3233=CARTESIAN_POINT ( 'NONE',  ( 0.4724409448818898682, 2.892866454678787531E-17, -0.9822834645669291653 ) ) ;
#3237=CARTESIAN_POINT ( 'NONE',  ( -0.4724409448818898682, 5.785732909357575061E-17, -2.755905511811024056 ) ) ;
#3240=CARTESIAN_POINT ( 'NONE',  ( 0.1049643490035303689, 0.3917322834645668994, 0.08400881709417505616 ) ) ;
#3242=CARTESIAN_POINT ( 'NONE',  ( 0.1958661417322836440, -0.3392501089628017219, -0.4914698162729659869 ) ) ;
#3249=CARTESIAN_POINT ( 'NONE',  ( 0.2867679344610365999, 0.2867679344610365999, -2.334645669291338432 ) ) ;
#3253=CARTESIAN_POINT ( 'NONE',  ( 0.4724409448818896462, 0.1265901696524990294, -0.3589238845144357426 ) ) ;
#3263=CARTESIAN_POINT ( 'NONE',  ( -0.1998031496062991630, -0.3460692066303959202, -1.402230971128609172 ) ) ;
#3272=CARTESIAN_POINT ( 'NONE',  ( -0.3996062992125985480, -7.340648628747423112E-17, -0.2736220472440945017 ) ) ;
#3273=CARTESIAN_POINT ( 'NONE',  ( -0.1070741851644051862, -0.3996062992125987146, -0.7020997375328084100 ) ) ;
#3274=CARTESIAN_POINT ( 'NONE',  ( -0.1958661417322836995, 0.3392501089628017219, -2.844507504758217120 ) ) ;
#3279=CARTESIAN_POINT ( 'NONE',  ( 4.837279021331061486E-17, -0.3949938075777409963, -0.9429133858267715329 ) ) ;
#3284=CARTESIAN_POINT ( 'NONE',  ( -0.2362204724409447953, -0.4091458600556404646, -1.325459317585301777 ) ) ;
#3285=CARTESIAN_POINT ( 'NONE',  ( 4.893765752498283924E-17, -0.3996062992125986035, -2.283464566929133799 ) ) ;
#3288=CARTESIAN_POINT ( 'NONE',  ( -0.3392501089628019995, 0.1958661417322831999, -0.4954261399288207857 ) ) ;
#3300=CARTESIAN_POINT ( 'NONE',  ( 0.1958661417322836440, -0.3392501089628017219, -0.8713910761154854967 ) ) ;
#3303=CARTESIAN_POINT ( 'NONE',  ( -0.3949938075777411628, 0.1058382717557497937, -1.135170603674540812 ) ) ;
#3307=CARTESIAN_POINT ( 'NONE',  ( -0.3460692066303958092, -0.1998031496062994683, 0.1049868766404199322 ) ) ;
#3315=CARTESIAN_POINT ( 'NONE',  ( -0.4724409448818904789, -0.1265901696524977804, -0.5951443569553804824 ) ) ;
#3320=CARTESIAN_POINT ( 'NONE',  ( 0.3996062992125986035, 2.446882876249141962E-17, -1.535433070866141669 ) ) ;
#3323=CARTESIAN_POINT ( 'NONE',  ( -0.1998031496062994405, 0.3460692066303957537, -1.034776902887139194 ) ) ;
#3324=CARTESIAN_POINT ( 'NONE',  ( -0.3460692066303957537, -0.1998031496062994405, -0.4442257217847768724 ) ) ;
#3327=CARTESIAN_POINT ( 'NONE',  ( -0.4091458600556402980, -0.2362204724409451284, -0.05249343832020997302 ) ) ;
#3328=CARTESIAN_POINT ( 'NONE',  ( -0.1049643490035302024, -0.3917322834645671215, -2.676509186351705871 ) ) ;
#3334=CARTESIAN_POINT ( 'NONE',  ( -0.4091458600556405756, 0.2362204724409446288, -2.307742782152230721 ) ) ;
#3337=CARTESIAN_POINT ( 'NONE',  ( -9.674558042662122972E-17, 0.3949938075777409963, -1.651574803149606474 ) ) ;
#3347=CARTESIAN_POINT ( 'NONE',  ( -0.1958661417322834497, -0.3392501089628018884, -2.350374385005562505 ) ) ;
#3362=CARTESIAN_POINT ( 'NONE',  ( -0.1070741851644051862, -0.3996062992125986590, -0.4639107611548556331 ) ) ;
#3364=CARTESIAN_POINT ( 'NONE',  ( -0.1049643490035307020, 0.3917322834645669549, -1.666010498687664043 ) ) ;
#3374=CARTESIAN_POINT ( 'NONE',  ( -0.3460692066303960313, 0.1998031496062989965, -1.047900262467191590 ) ) ;
#3383=CARTESIAN_POINT ( 'NONE',  ( -0.2867679344610365999, 0.2867679344610364889, -1.679133858267716661 ) ) ;
#3388=CARTESIAN_POINT ( 'NONE',  ( 0.2925321140481931814, -0.2925321140481931259, -2.222440944881889813 ) ) ;
#3390=CARTESIAN_POINT ( 'NONE',  ( 4.893765752498283924E-17, -0.3996062992125986035, -0.5511811023622047445 ) ) ;
#3394=CARTESIAN_POINT ( 'NONE',  ( -0.1049643490035302024, -0.3917322834645671215, -2.111548556430446144 ) ) ;
#3404=CARTESIAN_POINT ( 'NONE',  ( -0.2867679344610364334, -0.2867679344610368219, -1.398930815451756793 ) ) ;
#3411=CARTESIAN_POINT ( 'NONE',  ( -0.1049643490035307158, 0.3917322834645670104, -2.837945824968191477 ) ) ;
#3419=CARTESIAN_POINT ( 'NONE',  ( 0.3917322834645670659, -0.1049643490035303273, -1.053168922081052283 ) ) ;
#3421=CARTESIAN_POINT ( 'NONE',  ( 0.3917322834645670104, 2.398668435337828261E-17, -2.407480314960630086 ) ) ;
#3427=CARTESIAN_POINT ( 'NONE',  ( -0.3460692066303957537, -0.1998031496062994405, 0.1856955380577427484 ) ) ;
#3429=CARTESIAN_POINT ( 'NONE',  ( 0.1070741851644053527, 0.3996062992125986590, -1.725721784776903078 ) ) ;
#3435=CARTESIAN_POINT ( 'NONE',  ( -0.4724409448818895907, -0.1265901696524993070, -0.5951443569553805935 ) ) ;
#3438=CARTESIAN_POINT ( 'NONE',  ( -0.3949938075777408852, -0.1058382717557502933, -0.5951443569553805935 ) ) ;
#3443=CARTESIAN_POINT ( 'NONE',  ( 0.1974969037888704704, 0.3420746716998660508, -0.5360892388451443669 ) ) ;
#3450=CARTESIAN_POINT ( 'NONE',  ( 4.893765752498283308E-17, -0.3996062992125985480, -1.415354330708661568 ) ) ;
#3452=CARTESIAN_POINT ( 'NONE',  ( 0.1049643490035303689, 0.3917322834645670104, -1.087926509186351476 ) ) ;
#3454=CARTESIAN_POINT ( 'NONE',  ( -0.3738583250858234508, -0.1188761721681601269, 7.390873527593494894E-17 ) ) ;
#3464=CARTESIAN_POINT ( 'NONE',  ( 0.4091458600556403535, 0.2362204724409449896, -0.2080052493438320216 ) ) ;
#3480=CARTESIAN_POINT ( 'NONE',  ( 0.1070741851644054915, -0.3996062992125985480, -1.030183727034120533 ) ) ;
#3485=CARTESIAN_POINT ( 'NONE',  ( -0.3458507752293909498, 0.3458507752293907833, -0.01968503937007874335 ) ) ;
#3486=CARTESIAN_POINT ( 'NONE',  ( -0.2891555358219911054, 0.2891555358219909388, -2.539370078740157854 ) ) ;
#3489=CARTESIAN_POINT ( 'NONE',  ( -0.3917322834645671215, 0.1049643490035301469, -0.9698162729658791337 ) ) ;
#3491=CARTESIAN_POINT ( 'NONE',  ( 0.2362204724409449064, 0.4091458600556404646, -2.349081364829396446 ) ) ;
#3497=CARTESIAN_POINT ( 'NONE',  ( 0.3392501089628018329, -0.1958661417322834497, -0.1850200542969010764 ) ) ;
#3503=CARTESIAN_POINT ( 'NONE',  ( -0.2925321140481932924, 0.2925321140481931814, -2.854330708661417138 ) ) ;
#3504=CARTESIAN_POINT ( 'NONE',  ( -0.3392501089628019995, 0.1958661417322831999, -1.755268659613860249 ) ) ;
#3510=CARTESIAN_POINT ( 'NONE',  ( -0.1958661417322834220, -0.3392501089628018884, -0.9376640419947508409 ) ) ;
#3518=CARTESIAN_POINT ( 'NONE',  ( -0.3458507752293906723, -0.3458507752293910609, -0.9232283464566929387 ) ) ;
#3519=CARTESIAN_POINT ( 'NONE',  ( 0.1958661417322834775, 0.3392501089628018884, -2.498687664041994605 ) ) ;
#3529=CARTESIAN_POINT ( 'NONE',  ( -0.3917322834645669549, -0.1049643490035306603, -0.9179790026246721357 ) ) ;
#3531=CARTESIAN_POINT ( 'NONE',  ( 0.3980111619244091625, 0.03175677952935741788, -1.929133858267720436 ) ) ;
#3532=CARTESIAN_POINT ( 'NONE',  ( 0.3917322834645669549, 0.1049643490035304660, -1.469160104986876769 ) ) ;
#3533=CARTESIAN_POINT ( 'NONE',  ( 0.1998031496062992463, 0.3460692066303959202, -2.583333333333333481 ) ) ;
#3542=CARTESIAN_POINT ( 'NONE',  ( -9.787531504996566615E-17, 0.3996062992125985480, -1.966535433070866201 ) ) ;
#3544=CARTESIAN_POINT ( 'NONE',  ( -0.1049643490035307020, 0.3917322834645669549, 0.1587926509186352031 ) ) ;
#3553=CARTESIAN_POINT ( 'NONE',  ( -0.2867679344610364334, -0.2867679344610368219, -1.398930815451756793 ) ) ;
#3561=CARTESIAN_POINT ( 'NONE',  ( -0.3917322834645670104, -0.1049643490035307020, -0.6725914942595296875 ) ) ;
#3564=CARTESIAN_POINT ( 'NONE',  ( -0.4724409448818899238, 0.1265901696524986686, -1.999343832020997525 ) ) ;
#3585=CARTESIAN_POINT ( 'NONE',  ( 0.3996062992125985480, 2.446882876249141654E-17, -2.242125984251968518 ) ) ;
#3591=CARTESIAN_POINT ( 'NONE',  ( 0.2925321140481932369, -0.2925321140481932369, -1.830708661417322913 ) ) ;
#3592=CARTESIAN_POINT ( 'NONE',  ( 0.2891555358219910499, -0.2891555358219909944, -1.200787401574803237 ) ) ;
#3593=CARTESIAN_POINT ( 'NONE',  ( -0.3996062992125987146, 0.1070741851644051862, -2.395013123359580387 ) ) ;
#3595=CARTESIAN_POINT ( 'NONE',  ( 0.3392501089628018329, 0.1958661417322835607, -0.1233595800524933811 ) ) ;
#3599=CARTESIAN_POINT ( 'NONE',  ( -0.1058382717557503072, 0.3949938075777408852, -2.288057742782152459 ) ) ;
#3603=CARTESIAN_POINT ( 'NONE',  ( 0.4724409448818898682, 2.892866454678787531E-17, -2.637795275590551380 ) ) ;
#3604=CARTESIAN_POINT ( 'NONE',  ( 0.2925321140481932369, 0.2925321140481932369, -1.870078740157480546 ) ) ;
#3611=CARTESIAN_POINT ( 'NONE',  ( -0.2867679344610365999, 0.2867679344610364889, 0.2106299212598424508 ) ) ;
#3618=CARTESIAN_POINT ( 'NONE',  ( -0.3917322834645670104, -7.196005306013484475E-17, 0.03346456692913377107 ) ) ;
#3620=CARTESIAN_POINT ( 'NONE',  ( 0.1958661417322836440, -0.3392501089628017219, -2.288713910761154935 ) ) ;
#3623=CARTESIAN_POINT ( 'NONE',  ( -0.1974969037888703871, -0.3420746716998661063, -2.585301837270341352 ) ) ;
#3627=CARTESIAN_POINT ( 'NONE',  ( 0.2925321140481932369, 0.2925321140481932369, -0.9251968503937008093 ) ) ;
#3631=CARTESIAN_POINT ( 'NONE',  ( 0.08106202739151405212, -0.3841287887292352266, -2.755905511811023612 ) ) ;
#3632=CARTESIAN_POINT ( 'NONE',  ( -9.594673741351313045E-17, 0.3917322834645670104, 0.07283464566929125084 ) ) ;
#3638=CARTESIAN_POINT ( 'NONE',  ( -0.2867679344610365999, 0.2867679344610364889, -0.01181102362204719709 ) ) ;
#3642=( NAMED_UNIT ( * ) SI_UNIT ( $, .STERADIAN. ) SOLID_ANGLE_UNIT ( ) );
#3644=CARTESIAN_POINT ( 'NONE',  ( -0.3458507752293909498, 0.3458507752293907833, -1.594488188976378229 ) ) ;
#3647=CARTESIAN_POINT ( 'NONE',  ( -0.3917322834645670104, -7.196005306013484475E-17, -0.6614173228346454936 ) ) ;
#3655=CARTESIAN_POINT ( 'NONE',  ( -0.1265901696524986964, -0.4724409448818899238, -1.961942257217847763 ) ) ;
#3658=CARTESIAN_POINT ( 'NONE',  ( -0.3917322834645669549, -7.196005306013483243E-17, 0.03807705856399132283 ) ) ;
#3660=CARTESIAN_POINT ( 'NONE',  ( 0.2867679344610366554, 0.2867679344610366554, -0.3799212598425197318 ) ) ;
#3665=CARTESIAN_POINT ( 'NONE',  ( 0.3392501089628018884, -0.1958661417322834220, -2.459317585301837195 ) ) ;
#3668=CARTESIAN_POINT ( 'NONE',  ( -0.4091458600556402980, -0.2362204724409451284, -0.9166666666666666297 ) ) ;
#3678=CARTESIAN_POINT ( 'NONE',  ( -0.3460692066303960313, 0.1998031496062989965, -1.677821522309711266 ) ) ;
#3686=CARTESIAN_POINT ( 'NONE',  ( 0.3996062992125984925, 0.1070741851644054499, -0.2014435695538057958 ) ) ;
#3687=CARTESIAN_POINT ( 'NONE',  ( 0.2925321140481932369, -0.2925321140481932369, -0.7283464566929134243 ) ) ;
#3688=CARTESIAN_POINT ( 'NONE',  ( -0.3917322834645671770, 0.1049643490035302024, -2.864192544128295825 ) ) ;
#3694=CARTESIAN_POINT ( 'NONE',  ( 0.1058382717557500852, -0.3949938075777408852, -0.7919947506561679784 ) ) ;
#3700=CARTESIAN_POINT ( 'NONE',  ( -0.2362204724409451284, 0.4091458600556402425, -1.272965879265091749 ) ) ;
#3702=CARTESIAN_POINT ( 'NONE',  ( -0.3460692066303960868, 0.1998031496062990242, -2.388451443569553856 ) ) ;
#3705=CARTESIAN_POINT ( 'NONE',  ( -9.594673741351313045E-17, 0.3917322834645670659, -0.7841400506899758316 ) ) ;
#3716=CARTESIAN_POINT ( 'NONE',  ( -0.1958661417322836718, 0.3392501089628017219, -0.9501312335958004285 ) ) ;
#3719=CARTESIAN_POINT ( 'NONE',  ( -0.1974969037888706647, 0.3420746716998658843, -0.9580052493438320216 ) ) ;
#3735=CARTESIAN_POINT ( 'NONE',  ( -0.2925321140481932924, 0.2925321140481931814, -1.751968503937007648 ) ) ;
#3738=CARTESIAN_POINT ( 'NONE',  ( 0.1070741851644054776, -0.3996062992125984925, -1.106955380577427706 ) ) ;
#3742=CARTESIAN_POINT ( 'NONE',  ( 0.4724409448818898682, 2.892866454678787531E-17, -0.4330708661417322913 ) ) ;
#3743=CARTESIAN_POINT ( 'NONE',  ( 4.797336870675656522E-17, -0.3917322834645670104, -2.683070866141731958 ) ) ;
#3749=CARTESIAN_POINT ( 'NONE',  ( -1.157146581871515012E-16, 0.4724409448818898682, -2.438976377952756014 ) ) ;
#3751=CARTESIAN_POINT ( 'NONE',  ( 0.3420746716998660508, 0.1974969037888705814, -1.782808398950131101 ) ) ;
#3762=CARTESIAN_POINT ( 'NONE',  ( 0.1049643490035304522, -0.3917322834645668994, -2.527539739336271296 ) ) ;
#3766=CARTESIAN_POINT ( 'NONE',  ( 0.4724409448818897017, 0.1265901696524990294, -0.9888451443569553634 ) ) ;
#3776=CARTESIAN_POINT ( 'NONE',  ( -0.1998031496062991630, -0.3460692066303959202, -0.2998687664041995160 ) ) ;
#3779=CARTESIAN_POINT ( 'NONE',  ( 0.3392501089628018329, 0.1958661417322835607, -1.633202099737532942 ) ) ;
#3788=CARTESIAN_POINT ( 'NONE',  ( 0.3460692066303959202, -0.1998031496062991630, -1.441601049868766582 ) ) ;
#3795=CARTESIAN_POINT ( 'NONE',  ( 0.2867679344610365999, 0.2867679344610365999, -1.639763779527558807 ) ) ;
#3801=CARTESIAN_POINT ( 'NONE',  ( 0.3460692066303958092, 0.1998031496062993018, -2.412729658792650778 ) ) ;
#3804=CARTESIAN_POINT ( 'NONE',  ( 0.2925321140481932369, 0.2925321140481932369, -0.6102362204724409711 ) ) ;
#3807=CARTESIAN_POINT ( 'NONE',  ( 0.3392501089628018884, -0.1958661417322834220, -2.301837270341207553 ) ) ;
#3814=CARTESIAN_POINT ( 'NONE',  ( 0.4724409448818898682, 2.892866454678787531E-17, -0.5905511811023621549 ) ) ;
#3817=CARTESIAN_POINT ( 'NONE',  ( -0.1958661417322836440, 0.3392501089628016664, -1.667959686842832356 ) ) ;
#3821=CARTESIAN_POINT ( 'NONE',  ( -0.2867679344610365999, 0.2867679344610364889, -2.624015748031495399 ) ) ;
#3824=CARTESIAN_POINT ( 'NONE',  ( 0.1049643490035303967, 0.3917322834645670659, -2.824822465388138415 ) ) ;
#3833=CARTESIAN_POINT ( 'NONE',  ( -0.3392501089628019995, 0.1958661417322831999, -1.282827714731970215 ) ) ;
#3835=CARTESIAN_POINT ( 'NONE',  ( 0.3392501089628018329, 0.1958661417322835607, -2.263123359580052618 ) ) ;
#3840=CARTESIAN_POINT ( 'NONE',  ( -0.3996062992125986035, -0.1070741851644056997, -0.3608923884514435576 ) ) ;
#3842=CARTESIAN_POINT ( 'NONE',  ( -0.3996062992125984925, -0.1070741851644056858, 0.03477690288713909672 ) ) ;
#3844=CARTESIAN_POINT ( 'NONE',  ( 0.3460692066303959202, 0.1998031496062993295, -2.178477690288713742 ) ) ;
#3849=CARTESIAN_POINT ( 'NONE',  ( 0.1265901696524990294, -0.4724409448818896462, -0.9494750656167976199 ) ) ;
#3852=CARTESIAN_POINT ( 'NONE',  ( -0.1058382717557503072, 0.3949938075777408852, -0.3982939632545932640 ) ) ;
#3866=CARTESIAN_POINT ( 'NONE',  ( -0.3996062992125986590, 0.1070741851644051723, -1.211942257217847541 ) ) ;
#3868=CARTESIAN_POINT ( 'NONE',  ( 0.3917322834645670104, -0.1049643490035303411, -1.206036745406823707 ) ) ;
#3870=CARTESIAN_POINT ( 'NONE',  ( -0.1988659768032651487, 0.3401783215957732143, 1.649893717844496181E-17 ) ) ;
#3878=CARTESIAN_POINT ( 'NONE',  ( 0.1265901696524989184, 0.4724409448818898127, -0.2276902887139107545 ) ) ;
#3889=CARTESIAN_POINT ( 'NONE',  ( 0.1049643490035303967, 0.3917322834645670659, -2.194901205545618961 ) ) ;
#3896=CARTESIAN_POINT ( 'NONE',  ( -0.1070741851644057135, 0.3996062992125985480, -1.108923884514435798 ) ) ;
#3900=CARTESIAN_POINT ( 'NONE',  ( 0.1070741851644054915, -0.3996062992125986035, -2.919947506561679784 ) ) ;
#3901=CARTESIAN_POINT ( 'NONE',  ( -9.674558042662121740E-17, 0.3949938075777409963, -2.204724409448819422 ) ) ;
#3904=CARTESIAN_POINT ( 'NONE',  ( -0.3392501089628019995, 0.1958661417322832277, -0.8057742782152230721 ) ) ;
#3906=CARTESIAN_POINT ( 'NONE',  ( 0.4724409448818896462, 0.1265901696524990294, -2.329396325459317296 ) ) ;
#3912=CARTESIAN_POINT ( 'NONE',  ( 0.1958661417322834497, 0.3392501089628018329, -0.3818704479976884336 ) ) ;
#3918=CARTESIAN_POINT ( 'NONE',  ( 0.3996062992125986035, 0.1070741851644054776, -2.801837270341207553 ) ) ;
#3919=CARTESIAN_POINT ( 'NONE',  ( 0.3917322834645670104, 0.1049643490035304660, -1.696213541503623912 ) ) ;
#3924=EDGE_CURVE ( 'NONE', #65725, #23851, #35905, .T. ) ;
#3927=CARTESIAN_POINT ( 'NONE',  ( -0.1049643490035302024, -0.3917322834645671215, -0.9442257217847768169 ) ) ;
#3938=CARTESIAN_POINT ( 'NONE',  ( 0.1049643490035303689, 0.3917322834645670104, -2.347769028871391050 ) ) ;
#3945=CARTESIAN_POINT ( 'NONE',  ( -0.3917322834645671215, 0.1049643490035301469, -0.9048556430446195176 ) ) ;
#3946=CARTESIAN_POINT ( 'NONE',  ( 0.1265901696524990294, -0.4724409448818896462, -0.004593175853018378711 ) ) ;
#3947=CARTESIAN_POINT ( 'NONE',  ( 0.1998031496062992463, 0.3460692066303959202, -2.268372703412073310 ) ) ;
#3957=CARTESIAN_POINT ( 'NONE',  ( -0.3917322834645671215, 0.1049643490035301469, -0.02493438320209968861 ) ) ;
#3964=CARTESIAN_POINT ( 'NONE',  ( -0.3917322834645669549, -7.196005306013483243E-17, -1.694206406002937593 ) ) ;
#3973=CARTESIAN_POINT ( 'NONE',  ( -0.1049643490035302301, -0.3917322834645671770, -0.5413578984590045051 ) ) ;
#3976=CARTESIAN_POINT ( 'NONE',  ( -0.4724409448818899238, 0.1265901696524986686, -2.156824146981627166 ) ) ;
#3996=CARTESIAN_POINT ( 'NONE',  ( 4.893765752498283924E-17, -0.3996062992125986035, -0.07874015748031498729 ) ) ;
#3997=CARTESIAN_POINT ( 'NONE',  ( -0.1070741851644051862, -0.3996062992125986590, -2.353674540682414662 ) ) ;
#4002=CARTESIAN_POINT ( 'NONE',  ( -0.2925321140481932924, 0.2925321140481931814, -1.751968503937007648 ) ) ;
#4003=CARTESIAN_POINT ( 'NONE',  ( 0.2891555358219910499, -0.2891555358219909944, -0.8858267716535433989 ) ) ;
#4004=CARTESIAN_POINT ( 'NONE',  ( 0.3460692066303959757, -0.1998031496062991907, -2.309711286089239035 ) ) ;
#4005=CARTESIAN_POINT ( 'NONE',  ( -0.4724409448818890911, 0.1265901696525001952, -0.6627296587926508886 ) ) ;
#4006=CARTESIAN_POINT ( 'NONE',  ( -0.2867679344610364334, -0.2867679344610367109, -0.05118110236220467513 ) ) ;
#4010=CARTESIAN_POINT ( 'NONE',  ( -0.1974969037888704149, -0.3420746716998661063, -2.347112860892388575 ) ) ;
#4014=CARTESIAN_POINT ( 'NONE',  ( -0.1265901696524986964, -0.4724409448818899238, -2.276902887139107268 ) ) ;
#4015=CARTESIAN_POINT ( 'NONE',  ( 0.1998031496062994405, -0.3460692066303958092, -1.666666666666666741 ) ) ;
#4022=CARTESIAN_POINT ( 'NONE',  ( -0.3917322834645669549, -7.196005306013483243E-17, -2.796568610727347082 ) ) ;
#4029=CARTESIAN_POINT ( 'NONE',  ( -0.3917322834645670104, -7.196005306013484475E-17, -0.1240157480314961758 ) ) ;
#4031=CARTESIAN_POINT ( 'NONE',  ( 0.2867679344610365999, -0.2867679344610365444, -2.137795275590551380 ) ) ;
#4034=CARTESIAN_POINT ( 'NONE',  ( -0.3949938075777411628, 0.1058382717557497937, -2.867454068241469756 ) ) ;
#4038=CARTESIAN_POINT ( 'NONE',  ( 0.1070741851644054915, -0.3996062992125986035, -1.030183727034120533 ) ) ;
#4043=CARTESIAN_POINT ( 'NONE',  ( -0.3392501089628017219, -0.1958661417322836718, -0.6095800524934383846 ) ) ;
#4049=CARTESIAN_POINT ( 'NONE',  ( 0.1049643490035303689, 0.3917322834645670104, -0.3005249343832020470 ) ) ;
#4052=CARTESIAN_POINT ( 'NONE',  ( -0.4724409448818899238, 0.1265901696524986686, -1.765091863517059823 ) ) ;
#4058=CARTESIAN_POINT ( 'NONE',  ( 0.4091458600556404646, -0.2362204724409448231, -1.994750656167979086 ) ) ;
#4061=CARTESIAN_POINT ( 'NONE',  ( -0.1049643490035306742, 0.3917322834645668994, -0.4015554873677671943 ) ) ;
#4063=CARTESIAN_POINT ( 'NONE',  ( -0.2867679344610364334, -0.2867679344610367109, -0.6161417322834645827 ) ) ;
#4068=CARTESIAN_POINT ( 'NONE',  ( 0.1958661417322834775, 0.3392501089628018884, -2.341207349081364963 ) ) ;
#4071=CARTESIAN_POINT ( 'NONE',  ( -0.4724409448818899238, 0.1265901696524986686, -0.5820209973753280863 ) ) ;
#4082=CARTESIAN_POINT ( 'NONE',  ( 0.1070741851644053388, 0.3996062992125986035, -2.117454068241469756 ) ) ;
#4090=CARTESIAN_POINT ( 'NONE',  ( 0.1998031496062992463, 0.3460692066303959202, -0.06364829396325462352 ) ) ;
#4091=CARTESIAN_POINT ( 'NONE',  ( 0.2925321140481932369, -0.2925321140481932369, -0.4133858267716534196 ) ) ;
#4092=CARTESIAN_POINT ( 'NONE',  ( 0.3917322834645670659, -0.1049643490035303273, -2.785452386647981449 ) ) ;
#4099=CARTESIAN_POINT ( 'NONE',  ( -0.3949938075777411073, 0.1058382717557497660, -0.8969816272965878134 ) ) ;
#4106=CARTESIAN_POINT ( 'NONE',  ( -0.3458507752293906723, -0.3458507752293910609, -1.161417322834645383 ) ) ;
#4107=CARTESIAN_POINT ( 'NONE',  ( 0.1998031496062994405, -0.3460692066303958092, -2.454068241469816058 ) ) ;
#4110=CARTESIAN_POINT ( 'NONE',  ( -0.3917322834645670104, -0.1049643490035307020, -0.8300718092201594400 ) ) ;
#4122=CARTESIAN_POINT ( 'NONE',  ( -0.2867679344610365999, 0.2867679344610364889, -0.9566929133858265155 ) ) ;
#4125=CARTESIAN_POINT ( 'NONE',  ( -9.674558042662121740E-17, 0.3949938075777409963, -1.259842519685039353 ) ) ;
#4136=CARTESIAN_POINT ( 'NONE',  ( -0.1958661417322834220, -0.3392501089628018884, 0.007217847769028785422 ) ) ;
#4141=CARTESIAN_POINT ( 'NONE',  ( -9.787531504996567848E-17, 0.3996062992125986035, -2.204724409448818978 ) ) ;
#4144=CARTESIAN_POINT ( 'NONE',  ( -0.1070741851644051862, -0.3996062992125986590, -1.408792650918635259 ) ) ;
#4148=CARTESIAN_POINT ( 'NONE',  ( 0.1265901696524990294, -0.4724409448818896462, -0.5577427821522309426 ) ) ;
#4150=CARTESIAN_POINT ( 'NONE',  ( 0.2867679344610365999, -0.2867679344610365444, -2.702755905511810663 ) ) ;
#4156=CARTESIAN_POINT ( 'NONE',  ( 0.4724409448818897572, -0.1265901696524988906, -2.235564304461942431 ) ) ;
#4158=CARTESIAN_POINT ( 'NONE',  ( -0.2891555358219911054, 0.2891555358219909388, -1.986220472440945128 ) ) ;
#4169=CARTESIAN_POINT ( 'NONE',  ( 0.3917322834645669549, 2.398668435337827645E-17, -2.402867823325772090 ) ) ;
#4183=CARTESIAN_POINT ( 'NONE',  ( 0.2925321140481932369, 0.2925321140481932369, -0.5295275590551181688 ) ) ;
#4184=CARTESIAN_POINT ( 'NONE',  ( -0.3917322834645669549, -0.1049643490035306603, -1.862860892388451761 ) ) ;
#4193=CARTESIAN_POINT ( 'NONE',  ( -0.3460692066303957537, -0.1998031496062994405, -1.231627296587926690 ) ) ;
#4200=CARTESIAN_POINT ( 'NONE',  ( 0.2867679344610365999, -0.2867679344610365444, -1.757874015748031260 ) ) ;
#4205=CARTESIAN_POINT ( 'NONE',  ( -0.1070741851644057135, 0.3996062992125984925, -2.288057742782152015 ) ) ;
#4207=CARTESIAN_POINT ( 'NONE',  ( 0.1070741851644053527, 0.3996062992125986590, -0.9383202099737533164 ) ) ;
#4210=CARTESIAN_POINT ( 'NONE',  ( -9.594673741351313045E-17, 0.3917322834645670104, -2.669291338582676865 ) ) ;
#4220=CARTESIAN_POINT ( 'NONE',  ( -0.3392501089628018329, -0.1958661417322836440, -2.179770710464879802 ) ) ;
#4223=CARTESIAN_POINT ( 'NONE',  ( -0.1958661417322836718, 0.3392501089628017219, 0.1522309711286089495 ) ) ;
#4226=CARTESIAN_POINT ( 'NONE',  ( 0.1974969037888706369, -0.3420746716998659953, -0.09186351706036749443 ) ) ;
#4234=CARTESIAN_POINT ( 'NONE',  ( -0.2867679344610367109, 0.2867679344610365444, -1.118785719981314264 ) ) ;
#4236=CARTESIAN_POINT ( 'NONE',  ( 0.1958661417322836440, -0.3392501089628017219, -2.066272965879265122 ) ) ;
#4242=CARTESIAN_POINT ( 'NONE',  ( 0.1998031496062992740, 0.3460692066303959757, -0.4593175853018372501 ) ) ;
#4244=CARTESIAN_POINT ( 'NONE',  ( 0.1998031496062992463, 0.3460692066303959202, -0.06364829396325459576 ) ) ;
#4247=CARTESIAN_POINT ( 'NONE',  ( -0.2925321140481930704, -0.2925321140481933480, -2.106299212598425452 ) ) ;
#4252=CARTESIAN_POINT ( 'NONE',  ( 0.4724409448818896462, 0.1265901696524990294, -1.146325459317585116 ) ) ;
#4255=CARTESIAN_POINT ( 'NONE',  ( 0.2891555358219910499, 0.2891555358219910499, -0.6870078740157480324 ) ) ;
#4269=CARTESIAN_POINT ( 'NONE',  ( -0.1070741851644051862, -0.3996062992125986590, -1.566272965879265344 ) ) ;
#4272=CARTESIAN_POINT ( 'NONE',  ( 0.1958661417322836440, -0.3392501089628017219, -1.658792650918635259 ) ) ;
#4293=CARTESIAN_POINT ( 'NONE',  ( -0.3392501089628017219, -0.1958661417322836995, -2.096476008695224991 ) ) ;
#4304=CARTESIAN_POINT ( 'NONE',  ( -1.157146581871515012E-16, 0.4724409448818898682, 0.000000000000000000 ) ) ;
#4305=CARTESIAN_POINT ( 'NONE',  ( -0.3420746716998661618, 0.1974969037888702206, -2.703412073490814027 ) ) ;
#4308=CARTESIAN_POINT ( 'NONE',  ( 0.3917322834645669549, 0.1049643490035304660, -1.219160104986876325 ) ) ;
#4310=CARTESIAN_POINT ( 'NONE',  ( 0.2362204724409451007, -0.4091458600556402980, -2.611548556430446144 ) ) ;
#4311=CARTESIAN_POINT ( 'NONE',  ( -0.4091458600556405756, 0.2362204724409446288, -0.8904199475065617264 ) ) ;
#4316=CARTESIAN_POINT ( 'NONE',  ( -0.1049643490035306742, 0.3917322834645668994, -0.2440751724071372475 ) ) ;
#4321=CARTESIAN_POINT ( 'NONE',  ( -0.1265901696524993347, 0.4724409448818896462, -0.006561679790026246628 ) ) ;
#4322=CARTESIAN_POINT ( 'NONE',  ( 0.1070741851644053527, 0.3996062992125986590, -2.828083989501312345 ) ) ;
#4323=CARTESIAN_POINT ( 'NONE',  ( -0.3917322834645670659, -7.196005306013484475E-17, -1.768392019193912423 ) ) ;
#4329=CARTESIAN_POINT ( 'NONE',  ( -0.2867679344610365999, 0.2867679344610364889, -0.8917322834645667884 ) ) ;
#4339=CARTESIAN_POINT ( 'NONE',  ( 0.3917322834645669549, 0.1049643490035304660, -2.321522309711285814 ) ) ;
#4346=CARTESIAN_POINT ( 'NONE',  ( 0.2867679344610365999, -0.2867679344610365444, -0.6555118110236222151 ) ) ;
#4349=CARTESIAN_POINT ( 'NONE',  ( -0.3460692066303957537, -0.1998031496062994405, -2.491469816272966042 ) ) ;
#4359=CARTESIAN_POINT ( 'NONE',  ( 0.2925321140481932369, -0.2925321140481931814, -0.3326771653543306728 ) ) ;
#4368=CARTESIAN_POINT ( 'NONE',  ( -9.594673741351310580E-17, 0.3917322834645669549, -1.812316642223410046 ) ) ;
#4378=CARTESIAN_POINT ( 'NONE',  ( -0.3917322834645670659, -7.196005306013484475E-17, -0.5085494995088732928 ) ) ;
#4382=CARTESIAN_POINT ( 'NONE',  ( -0.2362204724409447953, -0.4091458600556404646, -1.874671916010498762 ) ) ;
#4403=CARTESIAN_POINT ( 'NONE',  ( 0.3460692066303959757, -0.1998031496062991907, -0.1049868766404199599 ) ) ;
#4404=CARTESIAN_POINT ( 'NONE',  ( 0.3996062992125985480, 2.446882876249141654E-17, -2.399606299212598604 ) ) ;
#4409=CARTESIAN_POINT ( 'NONE',  ( -0.2925321140481930704, -0.2925321140481933480, -1.791338582677165059 ) ) ;
#4410=CARTESIAN_POINT ( 'NONE',  ( -0.3949938075777409963, -7.255918531996591613E-17, -1.299212598425196985 ) ) ;
#4411=CARTESIAN_POINT ( 'NONE',  ( 0.2925321140481932369, 0.2925321140481932369, -2.657480314960630530 ) ) ;
#4412=CARTESIAN_POINT ( 'NONE',  ( 0.4724409448818892576, 0.1265901696524997788, -0.5971128608923885750 ) ) ;
#4413=CARTESIAN_POINT ( 'NONE',  ( 4.797336870675656522E-17, -0.3917322834645670104, -0.7007874015748030150 ) ) ;
#4417=CARTESIAN_POINT ( 'NONE',  ( -0.1974969037888706924, 0.3420746716998658843, -1.979658792650919041 ) ) ;
#4422=CARTESIAN_POINT ( 'NONE',  ( -0.4091458600556405756, 0.2362204724409446288, -2.545931758530183497 ) ) ;
#4424=CARTESIAN_POINT ( 'NONE',  ( -0.3996062992125987146, 0.1070741851644051862, -1.765091863517059823 ) ) ;
#4428=EDGE_CURVE ( 'NONE', #59522, #59098, #41765, .T. ) ;
#4432=CARTESIAN_POINT ( 'NONE',  ( -0.3392501089628019995, 0.1958661417322832277, 0.2040682414698161695 ) ) ;
#4439=CARTESIAN_POINT ( 'NONE',  ( -0.3917322834645671215, 0.1049643490035301469, -0.1174540682414699083 ) ) ;
#4441=CARTESIAN_POINT ( 'NONE',  ( -0.3917322834645669549, -0.1049643490035306603, -2.400262467191600635 ) ) ;
#4445=CARTESIAN_POINT ( 'NONE',  ( -0.2891555358219908833, -0.2891555358219912164, -2.893700787401575436 ) ) ;
#4449=CARTESIAN_POINT ( 'NONE',  ( 0.3460692066303959757, -0.1998031496062991907, -1.049868766404199460 ) ) ;
#4451=CARTESIAN_POINT ( 'NONE',  ( -0.4724409448818896462, -0.1265901696524993070, -0.7526246719160104570 ) ) ;
#4454=CARTESIAN_POINT ( 'NONE',  ( 0.3917322834645670104, 2.398668435337828261E-17, -0.3602362204724410266 ) ) ;
#4460=CARTESIAN_POINT ( 'NONE',  ( -0.3392501089628019995, 0.1958661417322832277, -0.1758530183727033402 ) ) ;
#4464=CARTESIAN_POINT ( 'NONE',  ( -1.157146581871515012E-16, 0.4724409448818898682, -1.732283464566929165 ) ) ;
#4471=CARTESIAN_POINT ( 'NONE',  ( 0.3392501089628018329, 0.1958661417322835052, -0.3687470884176359265 ) ) ;
#4473=CARTESIAN_POINT ( 'NONE',  ( -0.1049643490035307020, 0.3917322834645669549, -0.2486876640419948270 ) ) ;
#4478=CARTESIAN_POINT ( 'NONE',  ( 0.2867679344610365999, -0.2867679344610365444, -2.295275590551181022 ) ) ;
#4481=CARTESIAN_POINT ( 'NONE',  ( -0.2362204724409447953, -0.4091458600556404646, -0.7723097112860892732 ) ) ;
#4495=CARTESIAN_POINT ( 'NONE',  ( 0.1998031496062992463, 0.3460692066303959202, -1.795931758530183719 ) ) ;
#4503=CARTESIAN_POINT ( 'NONE',  ( -9.787531504996566615E-17, 0.3996062992125985480, -0.2342519685039370358 ) ) ;
#4504=CARTESIAN_POINT ( 'NONE',  ( -0.3460692066303960868, 0.1998031496062990242, -0.4986876640419947715 ) ) ;
#4505=CARTESIAN_POINT ( 'NONE',  ( 0.3949938075777409963, 2.418639510665530435E-17, 0.03937007874015741732 ) ) ;
#4509=CARTESIAN_POINT ( 'NONE',  ( 0.1974969037888704704, 0.3420746716998660508, -1.008530183727033958 ) ) ;
#4514=CARTESIAN_POINT ( 'NONE',  ( -0.1265901696524986964, -0.4724409448818899238, -1.332020997375328086 ) ) ;
#4515=CARTESIAN_POINT ( 'NONE',  ( -0.3996062992125985480, -0.1070741851644057135, -2.250656167979002475 ) ) ;
#4518=CARTESIAN_POINT ( 'NONE',  ( -0.3392501089628017219, -0.1958661417322836995, -0.9941138039708155016 ) ) ;
#4529=CARTESIAN_POINT ( 'NONE',  ( 0.1958661417322834775, 0.3392501089628018884, -1.081364829396325389 ) ) ;
#4532=CARTESIAN_POINT ( 'NONE',  ( 0.1974969037888706369, -0.3420746716998659953, -1.351706036745407014 ) ) ;
#4542=CARTESIAN_POINT ( 'NONE',  ( -0.1265901696524986964, -0.4724409448818899238, -1.017060367454068137 ) ) ;
#4543=CARTESIAN_POINT ( 'NONE',  ( 0.3392501089628018884, -0.1958661417322834220, -0.03215223097112869521 ) ) ;
#4550=CARTESIAN_POINT ( 'NONE',  ( -0.2925321140481930704, -0.2925321140481933480, -2.106299212598425452 ) ) ;
#4553=CARTESIAN_POINT ( 'NONE',  ( -0.3996062992125984925, -0.1070741851644056858, -1.697506561679789971 ) ) ;
#4557=CARTESIAN_POINT ( 'NONE',  ( -0.3458507752293906723, -0.3458507752293910609, -0.3740157480314960092 ) ) ;
#4559=CARTESIAN_POINT ( 'NONE',  ( 0.3917322834645670104, -0.1049643490035303411, -2.873359580052493811 ) ) ;
#4565=CARTESIAN_POINT ( 'NONE',  ( 0.2362204724409451007, -0.4091458600556402980, -2.530839895013123453 ) ) ;
#4568=CARTESIAN_POINT ( 'NONE',  ( -0.3949938075777411073, 0.1058382717557497660, -2.314304461942256808 ) ) ;
#4585=CARTESIAN_POINT ( 'NONE',  ( 4.893765752498283924E-17, -0.3996062992125986035, -2.755905511811023612 ) ) ;
#4588=CARTESIAN_POINT ( 'NONE',  ( -0.3996062992125986590, 0.1070741851644051723, -0.5820209973753280863 ) ) ;
#4589=CARTESIAN_POINT ( 'NONE',  ( 0.3917322834645670104, 2.398668435337828261E-17, -2.092519685039370358 ) ) ;
#4605=CARTESIAN_POINT ( 'NONE',  ( -0.2867679344610365999, 0.2867679344610364889, -1.521653543307086354 ) ) ;
#4610=CARTESIAN_POINT ( 'NONE',  ( -0.1998031496062991630, -0.3460692066303959202, -2.504593175853018661 ) ) ;
#4612=CARTESIAN_POINT ( 'NONE',  ( 0.1998031496062992740, 0.3460692066303959757, -0.7742782152230971437 ) ) ;
#4616=CARTESIAN_POINT ( 'NONE',  ( 4.797336870675656522E-17, -0.3917322834645670104, -2.433070866141732402 ) ) ;
#4623=DIRECTION ( 'NONE',  ( 1.000000000000000000, 0.000000000000000000, 0.000000000000000000 ) ) ;
#4626=CARTESIAN_POINT ( 'NONE',  ( -0.3917322834645668994, -0.1049643490035306742, -1.858248400753593987 ) ) ;
#4629=CARTESIAN_POINT ( 'NONE',  ( 0.3392501089628018329, 0.1958661417322835607, 0.03412073490813653104 ) ) ;
#4632=CARTESIAN_POINT ( 'NONE',  ( -0.3420746716998661618, 0.1974969037888702206, -0.1837270341207349611 ) ) ;
#4640=CARTESIAN_POINT ( 'NONE',  ( 4.797336870675656522E-17, -0.3917322834645670659, -1.177840838091550602 ) ) ;
#4642=CARTESIAN_POINT ( 'NONE',  ( 0.1049643490035304938, -0.3917322834645669549, -2.847112860892388131 ) ) ;
#4647=CARTESIAN_POINT ( 'NONE',  ( 0.1998031496062992740, 0.3460692066303959757, -0.7742782152230971437 ) ) ;
#4649=CARTESIAN_POINT ( 'NONE',  ( 0.3460692066303959202, -0.1998031496062991630, -0.1817585301837270351 ) ) ;
#4651=CARTESIAN_POINT ( 'NONE',  ( -0.1070741851644051862, -0.3996062992125987146, -2.119422572178477626 ) ) ;
#4655=CARTESIAN_POINT ( 'NONE',  ( 0.4724409448818897572, -0.1265901696524988906, -1.133202099737532720 ) ) ;
#4658=CARTESIAN_POINT ( 'NONE',  ( 0.1058382717557500852, -0.3949938075777408852, -0.7919947506561679784 ) ) ;
#4671=CARTESIAN_POINT ( 'NONE',  ( 4.893765752498283308E-17, -0.3996062992125985480, -1.572834645669291431 ) ) ;
#4674=CARTESIAN_POINT ( 'NONE',  ( 0.1049643490035303689, 0.3917322834645670104, -1.402887139107611647 ) ) ;
#4690=CARTESIAN_POINT ( 'NONE',  ( 0.4709442531824356015, 0.03757601356358734185, -1.929133858267717549 ) ) ;
#4704=CARTESIAN_POINT ( 'NONE',  ( 0.1998031496062992740, 0.3460692066303959757, -1.089238845144356871 ) ) ;
#4706=CARTESIAN_POINT ( 'NONE',  ( 0.3917322834645669549, 0.1049643490035304660, -2.164041994750655729 ) ) ;
#4709=CARTESIAN_POINT ( 'NONE',  ( -0.2362204724409447953, -0.4091458600556404646, -0.5380577427821522374 ) ) ;
#4710=CARTESIAN_POINT ( 'NONE',  ( -0.1058382717557497937, -0.3949938075777411628, -2.906824146981628054 ) ) ;
#4713=CARTESIAN_POINT ( 'NONE',  ( 0.1049643490035303689, 0.3917322834645670104, -1.402887139107611647 ) ) ;
#4715=CARTESIAN_POINT ( 'NONE',  ( 0.4091458600556403535, 0.2362204724409449896, -2.650918635170603554 ) ) ;
#4721=CARTESIAN_POINT ( 'NONE',  ( 0.3917322834645668994, -0.1049643490035303134, -0.6640226789688171705 ) ) ;
#4730=CARTESIAN_POINT ( 'NONE',  ( 0.2867679344610366554, -0.2867679344610365999, -1.984927452264778847 ) ) ;
#4735=VECTOR ( 'NONE', #36418, 39.37007874015748143 ) ;
#4738=CARTESIAN_POINT ( 'NONE',  ( 0.1958661417322836440, -0.3392501089628017219, -1.436351706036745446 ) ) ;
#4748=CARTESIAN_POINT ( 'NONE',  ( -0.1049643490035307020, 0.3917322834645669549, -2.675853018372703396 ) ) ;
#4755=CARTESIAN_POINT ( 'NONE',  ( -0.2867679344610364334, -0.2867679344610367109, -0.6161417322834646937 ) ) ;
#4756=CARTESIAN_POINT ( 'NONE',  ( -0.3458507752293906723, -0.3458507752293910609, 0.1791338582677165503 ) ) ;
#4758=CARTESIAN_POINT ( 'NONE',  ( 0.3996062992125985480, 2.446882876249141654E-17, -2.557086614173228689 ) ) ;
#4768=CARTESIAN_POINT ( 'NONE',  ( 0.3996062992125984925, 0.1070741851644054637, -0.3589238845144357426 ) ) ;
#4770=CARTESIAN_POINT ( 'NONE',  ( -0.2867679344610365999, 0.2867679344610364889, -0.3267716535433070613 ) ) ;
#4777=CARTESIAN_POINT ( 'NONE',  ( 0.3917322834645668994, 0.1049643490035304522, -1.464547613352018773 ) ) ;
#4786=CARTESIAN_POINT ( 'NONE',  ( 0.3917322834645670659, 2.398668435337828261E-17, -0.7447699719498183102 ) ) ;
#4790=CARTESIAN_POINT ( 'NONE',  ( 0.2362204724409451007, -0.4091458600556402980, -2.058398950131233640 ) ) ;
#4811=CARTESIAN_POINT ( 'NONE',  ( 0.1070741851644054915, -0.3996062992125985480, -0.08530183727034119923 ) ) ;
#4812=CARTESIAN_POINT ( 'NONE',  ( 0.3996062992125985480, 2.446882876249141654E-17, -2.557086614173228689 ) ) ;
#4817=CARTESIAN_POINT ( 'NONE',  ( -0.3460692066303960868, 0.1998031496062990242, -2.388451443569553856 ) ) ;
#4818=CARTESIAN_POINT ( 'NONE',  ( -0.3949938075777411628, 0.1058382717557497937, -1.450131233595800762 ) ) ;
#4819=CARTESIAN_POINT ( 'NONE',  ( 0.1070741851644054915, -0.3996062992125986035, -2.919947506561679784 ) ) ;
#4821=CARTESIAN_POINT ( 'NONE',  ( -0.3392501089628017219, -0.1958661417322836718, -0.5170603674540682482 ) ) ;
#4825=CARTESIAN_POINT ( 'NONE',  ( 0.1058382717557500852, -0.3949938075777408852, -2.524278215223097366 ) ) ;
#4830=CARTESIAN_POINT ( 'NONE',  ( -0.3458507752293909498, 0.3458507752293907833, -2.539370078740157410 ) ) ;
#4831=CARTESIAN_POINT ( 'NONE',  ( 0.3996062992125986035, 0.1070741851644054776, -2.171916010498687211 ) ) ;
#4841=CARTESIAN_POINT ( 'NONE',  ( -0.2867679344610366554, 0.2867679344610365444, -2.619403256396638735 ) ) ;
#4848=CARTESIAN_POINT ( 'NONE',  ( 4.797336870675656522E-17, -0.3917322834645670104, -0.3208661417322835607 ) ) ;
#4849=CARTESIAN_POINT ( 'NONE',  ( -0.1049643490035307020, 0.3917322834645669549, -1.573490813648293907 ) ) ;
#4850=CARTESIAN_POINT ( 'NONE',  ( -0.3392501089628019995, 0.1958661417322832277, -2.223097112860892288 ) ) ;
#4853=CARTESIAN_POINT ( 'NONE',  ( 0.1974969037888704704, 0.3420746716998660508, -2.821522309711286258 ) ) ;
#4858=CARTESIAN_POINT ( 'NONE',  ( 0.1998031496062994405, -0.3460692066303958092, -1.351706036745406792 ) ) ;
#4861=CARTESIAN_POINT ( 'NONE',  ( -0.4724409448818898682, -8.678599364036362592E-17, -0.9035433070866141225 ) ) ;
#4863=CARTESIAN_POINT ( 'NONE',  ( -0.2867679344610365999, 0.2867679344610364889, -0.4192913385826772532 ) ) ;
#4869=CARTESIAN_POINT ( 'NONE',  ( 0.1049643490035303689, 0.3917322834645670104, -0.1430446194225721002 ) ) ;
#4874=CARTESIAN_POINT ( 'NONE',  ( -0.1265901696524986964, -0.4724409448818899238, -1.489501312335957950 ) ) ;
#4877=CARTESIAN_POINT ( 'NONE',  ( -0.4724409448818899238, 0.1265901696524986964, -0.9776902887139107268 ) ) ;
#4885=CARTESIAN_POINT ( 'NONE',  ( -0.1958661417322836440, 0.3392501089628016664, -0.5655974821184234225 ) ) ;
#4887=CARTESIAN_POINT ( 'NONE',  ( -0.1958661417322836718, 0.3392501089628017219, -1.042650918635170676 ) ) ;
#4892=CARTESIAN_POINT ( 'NONE',  ( 0.1958661417322836440, -0.3392501089628017219, -2.288713910761154935 ) ) ;
#4894=EDGE_CURVE ( 'NONE', #21217, #49832, #69102, .T. ) ;
#4898=CARTESIAN_POINT ( 'NONE',  ( -0.4724409448818895907, -0.1265901696524993070, -0.5951443569553805935 ) ) ;
#4907=CARTESIAN_POINT ( 'NONE',  ( -1.157146581871515012E-16, 0.4724409448818898682, -0.3149606299212598381 ) ) ;
#4910=CARTESIAN_POINT ( 'NONE',  ( 0.1070741851644054776, -0.3996062992125984925, -1.894356955380577023 ) ) ;
#4921=CARTESIAN_POINT ( 'NONE',  ( -0.3460692066303957537, -0.1998031496062994405, -0.1292650918635170898 ) ) ;
#4922=CARTESIAN_POINT ( 'NONE',  ( -0.2925321140481932924, 0.2925321140481931814, -0.3346456692913385988 ) ) ;
#4923=CARTESIAN_POINT ( 'NONE',  ( -0.3949938075777409408, -0.1058382717557502933, -0.3608923884514436686 ) ) ;
#4929=CARTESIAN_POINT ( 'NONE',  ( -0.1974969037888706924, 0.3420746716998658843, -0.8772965879265093303 ) ) ;
#4935=CARTESIAN_POINT ( 'NONE',  ( 0.4091458600556403535, 0.2362204724409449896, -1.233595800524934338 ) ) ;
#4936=CARTESIAN_POINT ( 'NONE',  ( 0.2925321140481932369, 0.2925321140481932369, -2.185039370078739829 ) ) ;
#4939=CARTESIAN_POINT ( 'NONE',  ( -0.3917322834645670104, -0.1049643490035307020, -0.6725914942595296875 ) ) ;
#4949=CARTESIAN_POINT ( 'NONE',  ( 0.3392501089628018329, 0.1958661417322835607, -0.9107611548556429071 ) ) ;
#4952=CARTESIAN_POINT ( 'NONE',  ( 4.837279021331060870E-17, -0.3949938075777409963, -1.338582677165354173 ) ) ;
#4967=CARTESIAN_POINT ( 'NONE',  ( 0.3917322834645670104, -0.1049643490035303411, -0.03871391076115493490 ) ) ;
#4974=CARTESIAN_POINT ( 'NONE',  ( -9.787531504996567848E-17, 0.3996062992125986035, -2.047244094488188892 ) ) ;
#4977=CARTESIAN_POINT ( 'NONE',  ( 0.2925321140481932369, -0.2925321140481931814, -1.750000000000000222 ) ) ;
#4981=CARTESIAN_POINT ( 'NONE',  ( -1.157146581871515012E-16, 0.4724409448818898682, -0.4724409448818898127 ) ) ;
#4983=CARTESIAN_POINT ( 'NONE',  ( 0.1049643490035304938, -0.3917322834645669549, -0.07742782152230966164 ) ) ;
#4989=CARTESIAN_POINT ( 'NONE',  ( -0.3458507752293906723, -0.3458507752293910609, -2.498031496062992574 ) ) ;
#4991=CARTESIAN_POINT ( 'NONE',  ( -0.1058382717557503072, 0.3949938075777408852, -2.445538057742782101 ) ) ;
#5012=CARTESIAN_POINT ( 'NONE',  ( -0.1998031496062991630, -0.3460692066303959202, -0.6148293963254594097 ) ) ;
#5014=CARTESIAN_POINT ( 'NONE',  ( 0.3917322834645669549, 0.1049643490035304660, -2.256561679790026531 ) ) ;
#5024=CARTESIAN_POINT ( 'NONE',  ( -0.4724409448818917001, 0.1265901696524956710, -2.629265091863517867 ) ) ;
#5030=CARTESIAN_POINT ( 'NONE',  ( -0.1049643490035302024, -0.3917322834645671215, -1.574146981627296604 ) ) ;
#5035=CARTESIAN_POINT ( 'NONE',  ( -0.3460692066303957537, -0.1998031496062994405, -2.491469816272966042 ) ) ;
#5037=CARTESIAN_POINT ( 'NONE',  ( 0.3996062992125986590, -0.1070741851644053111, -1.056430446194225992 ) ) ;
#5040=CARTESIAN_POINT ( 'NONE',  ( 0.2867679344610365999, 0.2867679344610365999, -2.492125984251968518 ) ) ;
#5041=EDGE_LOOP ( 'NONE', ( #59399, #1348, #43449, #26373 ) ) ;
#5052=CARTESIAN_POINT ( 'NONE',  ( 0.3917322834645669549, 0.1049643490035304660, -2.729002624671915900 ) ) ;
#5054=VERTEX_POINT ( 'NONE', #31612 ) ;
#5055=CARTESIAN_POINT ( 'NONE',  ( -0.3420746716998661618, 0.1974969037888702206, -0.3412073490813648524 ) ) ;
#5063=CARTESIAN_POINT ( 'NONE',  ( 0.2867679344610366554, 0.2867679344610366554, -1.236895956201786717 ) ) ;
#5065=CARTESIAN_POINT ( 'NONE',  ( -0.2867679344610364334, -0.2867679344610367109, -2.505905511811023612 ) ) ;
#5070=CARTESIAN_POINT ( 'NONE',  ( 4.893765752498283924E-17, -0.3996062992125986035, -0.7086614173228346081 ) ) ;
#5072=CARTESIAN_POINT ( 'NONE',  ( -0.2925321140481932369, 0.2925321140481931259, -0.2539370078740156855 ) ) ;
#5074=CARTESIAN_POINT ( 'NONE',  ( -9.787531504996567848E-17, 0.3996062992125986035, -2.204724409448818978 ) ) ;
#5075=CARTESIAN_POINT ( 'NONE',  ( 0.3917322834645670104, -0.1049643490035303411, -1.770997375328083656 ) ) ;
#5079=CARTESIAN_POINT ( 'NONE',  ( 0.4091458600556404646, -0.2362204724409448231, -1.284120734908136496 ) ) ;
#5082=CARTESIAN_POINT ( 'NONE',  ( 0.3949938075777409963, 2.418639510665530743E-17, -0.9822834645669292764 ) ) ;
#5095=CARTESIAN_POINT ( 'NONE',  ( -0.3996062992125984925, -0.1070741851644056858, -1.854986876640420057 ) ) ;
#5110=CARTESIAN_POINT ( 'NONE',  ( 0.2867679344610365999, 0.2867679344610365999, -0.8523622047244096001 ) ) ;
#5126=CARTESIAN_POINT ( 'NONE',  ( 0.1998031496062994405, -0.3460692066303958092, -1.036745406824147064 ) ) ;
#5132=CARTESIAN_POINT ( 'NONE',  ( -0.4724409448818898682, -8.678599364036362592E-17, -0.5118110236220472231 ) ) ;
#5133=CARTESIAN_POINT ( 'NONE',  ( -0.3949938075777409963, -7.255918531996591613E-17, -2.559055118110236560 ) ) ;
#5134=ORIENTED_EDGE ( 'NONE', *, *, #64537, .T. ) ;
#5136=CARTESIAN_POINT ( 'NONE',  ( 0.3917322834645670104, -0.1049643490035303411, -1.363517060367453793 ) ) ;
#5138=CARTESIAN_POINT ( 'NONE',  ( -0.4091458600556402980, -0.2362204724409451284, -2.414698162729658648 ) ) ;
#5144=CARTESIAN_POINT ( 'NONE',  ( -0.2867679344610364334, -0.2867679344610368219, -0.7690095556092370055 ) ) ;
#5152=CARTESIAN_POINT ( 'NONE',  ( -0.3392501089628017219, -0.1958661417322836995, -2.096476008695224991 ) ) ;
#5160=CARTESIAN_POINT ( 'NONE',  ( -0.1049643490035307020, 0.3917322834645669549, -1.351049868766404538 ) ) ;
#5169=CARTESIAN_POINT ( 'NONE',  ( 0.3917322834645670104, 2.398668435337828261E-17, -2.944881889763779181 ) ) ;
#5176=CARTESIAN_POINT ( 'NONE',  ( -0.1049643490035302024, -0.3917322834645671215, -1.259186351706037099 ) ) ;
#5177=CARTESIAN_POINT ( 'NONE',  ( 0.2362204724409451007, -0.4091458600556402980, 0.1463254593175852825 ) ) ;
#5179=CARTESIAN_POINT ( 'NONE',  ( -0.3420746716998662729, 0.1974969037888702206, 0.2119422572178478181 ) ) ;
#5188=CARTESIAN_POINT ( 'NONE',  ( 0.1070741851644053388, 0.3996062992125986035, -0.5426509186351704539 ) ) ;
#5190=CARTESIAN_POINT ( 'NONE',  ( 0.1958661417322836440, -0.3392501089628017219, -0.3989501312335957950 ) ) ;
#5197=B_SPLINE_CURVE_WITH_KNOTS ( 'NONE', 3,
 ( #46124, #52851, #2366, #20888, #46539, #33926, #78562, #26773, #52013, #14588, #34345, #71819, #58760, #46953, #73062, #60010, #1946, #59589, #65924, #7847, #8261, #27608, #53269, #78979, #21300, #72645, #53681, #9095, #20048, #21708, #14995, #40652, #66336, #34768, #60427, #2778, #45700, #71396 ),
 .UNSPECIFIED., .F., .F.,
 ( 4, 2, 2, 2, 2, 2, 2, 2, 2, 2, 2, 2, 2, 2, 2, 2, 2, 2, 4 ),
 ( 2.754675881573757960E-16, 0.003207193274590246918, 0.004810789911885232466, 0.006414386549180218881, 0.007216184867827709487, 0.008017983186475202695, 0.009621579823770182172, 0.01042337814241767538, 0.01122517646106516512, 0.01282877309836014459, 0.01363057141700763954, 0.01443236973565512754, 0.01603596637295011049, 0.01763956301024508996, 0.01924315964754007291, 0.02084675628483505239, 0.02245035292213002839, 0.02405394955942500787, 0.02565754619671998388 ),
 .UNSPECIFIED. ) ;
#5206=CARTESIAN_POINT ( 'NONE',  ( -0.3392501089628019995, 0.1958661417322831999, -0.9678670848107107094 ) ) ;
#5210=CARTESIAN_POINT ( 'NONE',  ( -0.4091458600556402980, -0.2362204724409451284, -2.019028871391076230 ) ) ;
#5225=EDGE_LOOP ( 'NONE', ( #25021, #51193, #5134, #58563 ) ) ;
#5230=CARTESIAN_POINT ( 'NONE',  ( 0.1998031496062992463, 0.3460692066303959202, -2.740813648293963567 ) ) ;
#5235=CARTESIAN_POINT ( 'NONE',  ( 0.1070741851644053527, 0.3996062992125986590, -2.040682414698162361 ) ) ;
#5236=CARTESIAN_POINT ( 'NONE',  ( 0.1058382717557500713, -0.3949938075777409408, -1.660104986876640654 ) ) ;
#5239=CARTESIAN_POINT ( 'NONE',  ( -0.1958661417322836718, 0.3392501089628017219, -0.4776902887139107268 ) ) ;
#5243=CARTESIAN_POINT ( 'NONE',  ( 0.3949938075777409408, -0.1058382717557499186, -2.708005249343832244 ) ) ;
#5247=CARTESIAN_POINT ( 'NONE',  ( 0.2362204724409451007, -0.4091458600556402980, -2.926509186351706315 ) ) ;
#5248=CARTESIAN_POINT ( 'NONE',  ( -9.787531504996567848E-17, 0.3996062992125986035, -2.204724409448818978 ) ) ;
#5255=CARTESIAN_POINT ( 'NONE',  ( 0.1049643490035304938, -0.3917322834645669549, -0.1699475065616798397 ) ) ;
#5262=CARTESIAN_POINT ( 'NONE',  ( -0.1049643490035302024, -0.3917322834645671215, -0.6292650918635172008 ) ) ;
#5263=CARTESIAN_POINT ( 'NONE',  ( 0.3392501089628018329, 0.1958661417322835607, -1.540682414698162805 ) ) ;
#5264=CARTESIAN_POINT ( 'NONE',  ( 0.3917322834645670104, -0.1049643490035303411, -2.780839895013122565 ) ) ;
#5267=CARTESIAN_POINT ( 'NONE',  ( 0.3420746716998659953, 0.1974969037888705536, -2.808398950131233640 ) ) ;
#5271=CARTESIAN_POINT ( 'NONE',  ( -0.3460692066303960868, 0.1998031496062990242, -1.443569553805774230 ) ) ;
#5277=CARTESIAN_POINT ( 'NONE',  ( 0.1958661417322834775, 0.3392501089628018884, -0.5439632545931759600 ) ) ;
#5278=( BOUNDED_CURVE ( )  B_SPLINE_CURVE ( 2, ( #67497, #9832, #61167, #3518, #22870, #48531, #16576, #6401, #17813, #69144, #76694, #69558, #50587 ),
 .UNSPECIFIED., .F., .F. ) 
 B_SPLINE_CURVE_WITH_KNOTS ( ( 3, 2, 2, 2, 2, 2, 3 ),
 ( 0.3624999999999999889, 0.3666666666666666408, 0.3708333333333333481, 0.3750000000000000000, 0.3791666666666666519, 0.3833333333333333592, 0.3875000000000000111 ),
 .UNSPECIFIED. ) 
 CURVE ( )  GEOMETRIC_REPRESENTATION_ITEM ( )  RATIONAL_B_SPLINE_CURVE ( ( 1.000000000000000000, 0.9659258262890683122, 1.000000000000000000, 0.9659258262890683122, 1.000000000000000000, 0.9659258262890683122, 1.000000000000000000, 0.9659258262890683122, 1.000000000000000000, 0.9659258262890683122, 1.000000000000000000, 0.9659258262890683122, 1.000000000000000000 ) ) 
 REPRESENTATION_ITEM ( '' )  );
#5289=CARTESIAN_POINT ( 'NONE',  ( -0.4724409448818895907, -0.1265901696524993070, -1.935695538057742526 ) ) ;
#5297=CARTESIAN_POINT ( 'NONE',  ( 0.2362204724409451007, -0.4091458600556402980, -2.688320209973753538 ) ) ;
#5301=CARTESIAN_POINT ( 'NONE',  ( -0.1958661417322834497, -0.3392501089628018884, -0.4606106054780034764 ) ) ;
#5303=CARTESIAN_POINT ( 'NONE',  ( -9.594673741351313045E-17, 0.3917322834645670104, -0.7145669291338584417 ) ) ;
#5308=CARTESIAN_POINT ( 'NONE',  ( -0.1958661417322834220, -0.3392501089628018884, -2.734908136482939511 ) ) ;
#5312=CARTESIAN_POINT ( 'NONE',  ( 5.785732909357575061E-17, -0.4724409448818898682, -0.9429133858267716439 ) ) ;
#5324=CARTESIAN_POINT ( 'NONE',  ( -0.3460692066303957537, -0.1998031496062994405, -2.019028871391076230 ) ) ;
#5332=CARTESIAN_POINT ( 'NONE',  ( -0.1998031496062991630, -0.3460692066303959202, -0.6148293963254594097 ) ) ;
#5333=CARTESIAN_POINT ( 'NONE',  ( 4.893765752498283924E-17, -0.3996062992125986035, -1.023622047244094446 ) ) ;
#5334=CARTESIAN_POINT ( 'NONE',  ( 0.3420746716998659953, 0.1974969037888705536, -0.1312335958005249881 ) ) ;
#5340=CARTESIAN_POINT ( 'NONE',  ( -0.3949938075777409963, -7.255918531996591613E-17, -1.375984251968503713 ) ) ;
#5345=CARTESIAN_POINT ( 'NONE',  ( -0.2362204724409447953, -0.4091458600556404646, -1.482939632545931863 ) ) ;
#5346=CARTESIAN_POINT ( 'NONE',  ( 0.1070741851644053666, 0.3996062992125986035, -2.670603674540682260 ) ) ;
#5359=CARTESIAN_POINT ( 'NONE',  ( 0.1049643490035303689, 0.3917322834645670104, -1.245406824146981561 ) ) ;
#5362=CARTESIAN_POINT ( 'NONE',  ( -0.3420746716998659953, -0.1974969037888706647, -1.312335958005249159 ) ) ;
#5367=CARTESIAN_POINT ( 'NONE',  ( -0.3996062992125986035, -0.1070741851644056997, -0.04593175853018373334 ) ) ;
#5374=CARTESIAN_POINT ( 'NONE',  ( -0.1049643490035302024, -0.3917322834645671215, 0.0006561679790025351077 ) ) ;
#5380=CARTESIAN_POINT ( 'NONE',  ( -0.3996062992125986035, -0.1070741851644056997, -2.093175853018372834 ) ) ;
#5383=CARTESIAN_POINT ( 'NONE',  ( 0.3996062992125985480, 2.446882876249141654E-17, -1.612204724409448842 ) ) ;
#5387=CARTESIAN_POINT ( 'NONE',  ( 0.3458507752293908943, 0.3458507752293908943, -0.6102362204724409711 ) ) ;
#5389=CARTESIAN_POINT ( 'NONE',  ( -0.3392501089628017219, -0.1958661417322836718, -2.814304461942257252 ) ) ;
#5395=CARTESIAN_POINT ( 'NONE',  ( -0.2925321140481930149, -0.2925321140481933480, 0.1791338582677164948 ) ) ;
#5397=CARTESIAN_POINT ( 'NONE',  ( -0.1974969037888706924, 0.3420746716998658843, -2.137139107611548905 ) ) ;
#5411=CARTESIAN_POINT ( 'NONE',  ( 0.000000000000000000, 0.000000000000000000, -2.755905511811024056 ) ) ;
#5420=CARTESIAN_POINT ( 'NONE',  ( 0.3460692066303958092, 0.1998031496062993018, -0.8379265091863516979 ) ) ;
#5421=CARTESIAN_POINT ( 'NONE',  ( -0.3392501089628017219, -0.1958661417322836718, -2.184383202099737797 ) ) ;
#5438=CARTESIAN_POINT ( 'NONE',  ( -0.2867679344610365999, 0.2867679344610364889, -1.994094488188976610 ) ) ;
#5442=LINE ( 'NONE', #24378, #55679 ) ;
#5445=CARTESIAN_POINT ( 'NONE',  ( 4.893765752498283924E-17, -0.3996062992125986035, -0.7086614173228346081 ) ) ;
#5447=CARTESIAN_POINT ( 'NONE',  ( -0.3917322834645671215, 0.1049643490035301469, -2.702099737532808632 ) ) ;
#5454=DIRECTION ( 'NONE',  ( 0.000000000000000000, 0.000000000000000000, 1.000000000000000000 ) ) ;
#5459=CARTESIAN_POINT ( 'NONE',  ( 0.3392501089628018884, -0.1958661417322834220, -2.866797900262466836 ) ) ;
#5462=CARTESIAN_POINT ( 'NONE',  ( -0.3949938075777411628, 0.1058382717557497937, -0.3477690288713912170 ) ) ;
#5470=CARTESIAN_POINT ( 'NONE',  ( 0.3917322834645670104, 0.1049643490035304660, -1.696213541503623912 ) ) ;
#5472=CARTESIAN_POINT ( 'NONE',  ( 0.2867679344610365999, -0.2867679344610365444, -2.545275590551181022 ) ) ;
#5478=CARTESIAN_POINT ( 'NONE',  ( -0.3460692066303958092, -0.1998031496062994683, -0.6824146981627295938 ) ) ;
#5480=CARTESIAN_POINT ( 'NONE',  ( 0.2925321140481932369, -0.2925321140481931814, -0.4901574803149606474 ) ) ;
#5483=CARTESIAN_POINT ( 'NONE',  ( 0.3996062992125986590, -0.1070741851644053111, -2.473753280839894764 ) ) ;
#5484=CARTESIAN_POINT ( 'NONE',  ( 0.2867679344610365999, 0.2867679344610365999, -1.797244094488188892 ) ) ;
#5488=CARTESIAN_POINT ( 'NONE',  ( -0.1265901696524993347, 0.4724409448818895907, -1.185695538057742526 ) ) ;
#5491=CARTESIAN_POINT ( 'NONE',  ( -9.674558042662122972E-17, 0.3949938075777409963, -1.179133858267716661 ) ) ;
#5501=CARTESIAN_POINT ( 'NONE',  ( 0.1998031496062994128, -0.3460692066303957537, -1.743438320209973913 ) ) ;
#5515=CARTESIAN_POINT ( 'NONE',  ( -0.1958661417322834220, -0.3392501089628018884, -1.095144356955380704 ) ) ;
#5521=EDGE_CURVE ( 'NONE', #50887, #11079, #40322, .T. ) ;
#5532=CARTESIAN_POINT ( 'NONE',  ( 0.4724409448818902568, -0.1265901696524981135, -0.5839895013123360679 ) ) ;
#5536=CARTESIAN_POINT ( 'NONE',  ( 0.1958661417322836440, -0.3392501089628017219, -2.131233595800524849 ) ) ;
#5539=CARTESIAN_POINT ( 'NONE',  ( 0.3458507752293908943, -0.3458507752293908943, -0.2559055118110235560 ) ) ;
#5540=CARTESIAN_POINT ( 'NONE',  ( 0.1058382717557499880, 0.3949938075777411073, -2.670603674540682260 ) ) ;
#5543=CARTESIAN_POINT ( 'NONE',  ( 4.797336870675656522E-17, -0.3917322834645670104, -1.330708661417322691 ) ) ;
#5545=CARTESIAN_POINT ( 'NONE',  ( -0.2362204724409451284, 0.4091458600556402425, -2.690288713910760965 ) ) ;
#5546=DIRECTION ( 'NONE',  ( 1.000000000000000000, 0.000000000000000000, 0.000000000000000000 ) ) ;
#5553=CARTESIAN_POINT ( 'NONE',  ( -0.3917322834645670659, 0.1049643490035301607, -0.5852825214885022387 ) ) ;
#5560=CARTESIAN_POINT ( 'NONE',  ( 0.1958661417322834775, 0.3392501089628018884, -1.873378895834332258 ) ) ;
#5567=CARTESIAN_POINT ( 'NONE',  ( 0.3917322834645669549, 0.1049643490035304660, -1.469160104986876769 ) ) ;
#5576=CARTESIAN_POINT ( 'NONE',  ( 0.3392501089628018329, 0.1958661417322835607, -2.643044619422571628 ) ) ;
#5583=CARTESIAN_POINT ( 'NONE',  ( -0.2867679344610364334, -0.2867679344610367109, -1.088582677165354173 ) ) ;
#5584=CARTESIAN_POINT ( 'NONE',  ( -0.4724409448818899238, 0.1265901696524986686, 0.04790026246719158304 ) ) ;
#5585=CARTESIAN_POINT ( 'NONE',  ( -0.3996062992125986590, 0.1070741851644051723, -2.786745406824146620 ) ) ;
#5596=CARTESIAN_POINT ( 'NONE',  ( 0.3460692066303959202, -0.1998031496062991630, -0.4967191601049869010 ) ) ;
#5598=CARTESIAN_POINT ( 'NONE',  ( -9.594673741351313045E-17, 0.3917322834645670104, -0.3070866141732283006 ) ) ;
#5612=CARTESIAN_POINT ( 'NONE',  ( -0.3392501089628017219, -0.1958661417322836995, -0.9941138039708155016 ) ) ;
#5617=B_SPLINE_CURVE_WITH_KNOTS ( 'NONE', 3,
 ( #41673, #42085, #67780, #67365, #61034, #29046, #54717, #56767, #82062, #82873, #69419, #37011, #50450, #49634, #81656, #43717, #57595, #76152, #23967, #25197, #6256, #63512, #75327, #56363, #11353, #31933, #25608, #17673, #83285, #30699, #62269, #50863, #24375, #51271, #18492, #38244, #63921, #50046 ),
 .UNSPECIFIED., .F., .F.,
 ( 4, 2, 2, 2, 2, 2, 2, 2, 2, 2, 2, 2, 2, 2, 2, 2, 2, 2, 4 ),
 ( 0.000000000000000000, 0.003207193274590005357, 0.004810789911885009554, 0.006414386549180013317, 0.007216184867827516065, 0.008017983186475018814, 0.009621579823770027781, 0.01042337814241752966, 0.01122517646106503328, 0.01282877309836003878, 0.01363057141700754413, 0.01443236973565504601, 0.01603596637295005151, 0.01763956301024505874, 0.01924315964754006250, 0.02084675628483506973, 0.02245035292213007003, 0.02405394955942507726, 0.02565754619672007755 ),
 .UNSPECIFIED. ) ;
#5618=CARTESIAN_POINT ( 'NONE',  ( 0.2362204724409449064, 0.4091458600556404646, -2.425853018372703396 ) ) ;
#5636=CARTESIAN_POINT ( 'NONE',  ( -0.3460692066303960868, 0.1998031496062990242, -0.3412073490813647969 ) ) ;
#5637=CARTESIAN_POINT ( 'NONE',  ( -0.3996062992125984925, -0.1070741851644056858, -2.642388451443570041 ) ) ;
#5642=CARTESIAN_POINT ( 'NONE',  ( -0.1070741851644051862, -0.3996062992125987146, -2.276902887139107268 ) ) ;
#5643=CARTESIAN_POINT ( 'NONE',  ( 0.3420746716998659953, 0.1974969037888705536, -1.548556430446194065 ) ) ;
#5645=CARTESIAN_POINT ( 'NONE',  ( 0.4724409448818898682, 2.892866454678787531E-17, -2.480314960629921295 ) ) ;
#5646=CARTESIAN_POINT ( 'NONE',  ( 0.1049643490035304799, -0.3917322834645669549, -0.5498687664041993495 ) ) ;
#5650=CARTESIAN_POINT ( 'NONE',  ( 0.3949938075777408852, 0.1058382717557500435, -2.406167979002624691 ) ) ;
#5654=CARTESIAN_POINT ( 'NONE',  ( -0.4091458600556405756, 0.2362204724409446288, -2.703412073490813583 ) ) ;
#5655=CARTESIAN_POINT ( 'NONE',  ( 0.3996062992125986590, -0.1070741851644053111, -2.001312335958005395 ) ) ;
#5661=CARTESIAN_POINT ( 'NONE',  ( -0.3917322834645670104, -7.196005306013484475E-17, -0.1240157480314961758 ) ) ;
#5668=CARTESIAN_POINT ( 'NONE',  ( -9.594673741351313045E-17, 0.3917322834645670104, -0.7145669291338584417 ) ) ;
#5669=CARTESIAN_POINT ( 'NONE',  ( 0.3392501089628018884, -0.1958661417322834220, -1.671916010498687655 ) ) ;
#5670=CARTESIAN_POINT ( 'NONE',  ( 0.3392501089628018329, 0.1958661417322835607, -2.643044619422571628 ) ) ;
#5672=CARTESIAN_POINT ( 'NONE',  ( 4.893765752498283924E-17, -0.3996062992125986035, -0.07874015748031498729 ) ) ;
#5675=CARTESIAN_POINT ( 'NONE',  ( -0.1070741851644051862, -0.3996062992125987146, -1.332020997375328086 ) ) ;
#5680=CARTESIAN_POINT ( 'NONE',  ( 0.3392501089628018884, -0.1958661417322834220, -0.3471128608923885195 ) ) ;
#5689=CARTESIAN_POINT ( 'NONE',  ( 0.1265901696524990294, -0.4724409448818896462, -1.975065616797900381 ) ) ;
#5699=CARTESIAN_POINT ( 'NONE',  ( 0.1049643490035304522, -0.3917322834645668994, -0.3228153298874523180 ) ) ;
#5701=CARTESIAN_POINT ( 'NONE',  ( -0.3392501089628019995, 0.1958661417322832277, -0.8982939632545933195 ) ) ;
#5707=CARTESIAN_POINT ( 'NONE',  ( 0.2867679344610365999, -0.2867679344610365444, -2.925196850393700920 ) ) ;
#5711=CARTESIAN_POINT ( 'NONE',  ( -0.4724409448818899238, 0.1265901696524986686, -1.369422572178477404 ) ) ;
#5723=CARTESIAN_POINT ( 'NONE',  ( -0.3996062992125984925, -0.1070741851644056858, -2.012467191601049699 ) ) ;
#5726=CARTESIAN_POINT ( 'NONE',  ( -0.3460692066303957537, -0.1998031496062994405, -1.546587926509186639 ) ) ;
#5732=CARTESIAN_POINT ( 'NONE',  ( 0.2925321140481931814, -0.2925321140481931259, -0.4901574803149605919 ) ) ;
#5733=CARTESIAN_POINT ( 'NONE',  ( 0.3996062992125986035, 0.1070741851644054776, -1.069553805774278166 ) ) ;
#5734=CARTESIAN_POINT ( 'NONE',  ( 0.3949938075777409963, 2.418639510665530435E-17, -0.4330708661417323468 ) ) ;
#5741=CARTESIAN_POINT ( 'NONE',  ( -0.1058382717557503072, 0.3949938075777408852, -1.500656167979002253 ) ) ;
#5746=CARTESIAN_POINT ( 'NONE',  ( 0.3458507752293908943, 0.3458507752293908943, -1.555118110236220597 ) ) ;
#5747=CARTESIAN_POINT ( 'NONE',  ( -0.1070741851644057135, 0.3996062992125985480, -2.683727034120734878 ) ) ;
#5751=VERTEX_POINT ( 'NONE', #24608 ) ;
#5763=CARTESIAN_POINT ( 'NONE',  ( -0.3917322834645671215, 0.1049643490035301469, -1.442257217847769057 ) ) ;
#5766=CARTESIAN_POINT ( 'NONE',  ( 0.3949938075777409963, 2.418639510665530435E-17, -1.535433070866141447 ) ) ;
#5771=CARTESIAN_POINT ( 'NONE',  ( 0.2925321140481932369, 0.2925321140481932369, -0.2952755905511811330 ) ) ;
#5778=CARTESIAN_POINT ( 'NONE',  ( 0.1049643490035303689, 0.3917322834645670104, 0.07939632545931750440 ) ) ;
#5784=CARTESIAN_POINT ( 'NONE',  ( 0.3996062992125986590, -0.1070741851644053111, -2.158792650918635037 ) ) ;
#5787=CARTESIAN_POINT ( 'NONE',  ( 0.1070741851644053388, 0.3996062992125986035, -1.645013123359579943 ) ) ;
#5792=CARTESIAN_POINT ( 'NONE',  ( 0.1265901696524989462, 0.4724409448818897572, -0.9383202099737533164 ) ) ;
#5794=CARTESIAN_POINT ( 'NONE',  ( 0.1049643490035304938, -0.3917322834645669549, 0.08005249343832024356 ) ) ;
#5796=CARTESIAN_POINT ( 'NONE',  ( -0.1958661417322836718, 0.3392501089628017219, -2.145013123359580387 ) ) ;
#5800=CARTESIAN_POINT ( 'NONE',  ( 0.2362204724409449064, 0.4091458600556404646, -2.583333333333333481 ) ) ;
#5803=CARTESIAN_POINT ( 'NONE',  ( -0.1974969037888706924, 0.3420746716998658843, -2.294619422572178102 ) ) ;
#5824=CARTESIAN_POINT ( 'NONE',  ( 0.3996062992125984925, 0.1070741851644054637, -0.6738845144356955252 ) ) ;
#5825=CARTESIAN_POINT ( 'NONE',  ( -0.3917322834645671215, 0.1049643490035301469, -2.322178477690288734 ) ) ;
#5834=CARTESIAN_POINT ( 'NONE',  ( 0.4724409448818905899, -0.1265901696524973641, -0.7414698162729659314 ) ) ;
#5835=CARTESIAN_POINT ( 'NONE',  ( -0.1049643490035302301, -0.3917322834645671770, -2.116161048065303696 ) ) ;
#5841=CARTESIAN_POINT ( 'NONE',  ( 0.1958661417322836440, -0.3392501089628017219, -2.066272965879265122 ) ) ;
#5848=CARTESIAN_POINT ( 'NONE',  ( 4.893765752498283924E-17, -0.3996062992125986035, -1.181102362204724310 ) ) ;
#5850=CARTESIAN_POINT ( 'NONE',  ( 0.1958661417322836440, -0.3392501089628017219, -2.761154855643044304 ) ) ;
#5863=CARTESIAN_POINT ( 'NONE',  ( -0.3917322834645670104, -7.196005306013484475E-17, -0.03149606299212594218 ) ) ;
#5866=CARTESIAN_POINT ( 'NONE',  ( -0.3420746716998659953, -0.1974969037888706647, -0.3674540682414698667 ) ) ;
#5875=CARTESIAN_POINT ( 'NONE',  ( 0.2867679344610366554, -0.2867679344610365999, -1.669966822343518897 ) ) ;
#5878=CARTESIAN_POINT ( 'NONE',  ( -0.3917322834645669549, -0.1049643490035306603, -2.650262467191601079 ) ) ;
#5882=CARTESIAN_POINT ( 'NONE',  ( 0.3460692066303959202, 0.1998031496062993295, -0.9186351706036745002 ) ) ;
#5884=CARTESIAN_POINT ( 'NONE',  ( 0.3996062992125986035, -0.1070741851644052972, -0.1883202099737532054 ) ) ;
#5885=CARTESIAN_POINT ( 'NONE',  ( 0.3460692066303958092, 0.1998031496062993018, -0.05052493438320212332 ) ) ;
#5887=CARTESIAN_POINT ( 'NONE',  ( -0.1998031496062991907, -0.3460692066303959757, -2.900262467191600635 ) ) ;
#5888=( BOUNDED_CURVE ( )  B_SPLINE_CURVE ( 2, ( #58608, #60281, #32942, #65782, #59859, #77570, #8941, #2631, #46391, #51865, #39674, #72086, #7702 ),
 .UNSPECIFIED., .F., .F. ) 
 B_SPLINE_CURVE_WITH_KNOTS ( ( 3, 2, 2, 2, 2, 2, 3 ),
 ( 0.2125000000000000222, 0.2166666666666667018, 0.2208333333333333537, 0.2250000000000000333, 0.2291666666666666852, 0.2333333333333333648, 0.2375000000000000167 ),
 .UNSPECIFIED. ) 
 CURVE ( )  GEOMETRIC_REPRESENTATION_ITEM ( )  RATIONAL_B_SPLINE_CURVE ( ( 0.9999999999999997780, 0.9659258262890685343, 1.000000000000000000, 0.9659258262890683122, 1.000000000000000000, 0.9659258262890683122, 1.000000000000000000, 0.9659258262890683122, 1.000000000000000000, 0.9659258262890683122, 1.000000000000000000, 0.9659258262890680902, 1.000000000000000222 ) ) 
 REPRESENTATION_ITEM ( '' )  );
#5889=CARTESIAN_POINT ( 'NONE',  ( 0.1049643490035303689, 0.3917322834645670104, -1.652887139107611425 ) ) ;
#5894=CARTESIAN_POINT ( 'NONE',  ( 0.1265901696524989462, 0.4724409448818897572, -1.487532808398950301 ) ) ;
#5898=CARTESIAN_POINT ( 'NONE',  ( -0.3949938075777411073, 0.1058382717557497660, -0.8969816272965878134 ) ) ;
#5908=CARTESIAN_POINT ( 'NONE',  ( -0.3996062992125986590, 0.1070741851644051723, -2.156824146981627166 ) ) ;
#5924=CARTESIAN_POINT ( 'NONE',  ( 0.1049643490035304938, -0.3917322834645669549, -0.7998687664041995715 ) ) ;
#5932=VECTOR ( 'NONE', #55530, 39.37007874015748143 ) ;
#5934=DIRECTION ( 'NONE',  ( 0.000000000000000000, 0.000000000000000000, 1.000000000000000000 ) ) ;
#5946=CARTESIAN_POINT ( 'NONE',  ( -0.3726288332202236653, -0.1208384647423932784, -1.929133858267952473 ) ) ;
#5949=CARTESIAN_POINT ( 'NONE',  ( 0.1265901696524989462, 0.4724409448818897572, -0.3083989501312335846 ) ) ;
#5950=CARTESIAN_POINT ( 'NONE',  ( 0.3420746716998659953, 0.1974969037888705536, -2.650918635170603554 ) ) ;
#5953=CARTESIAN_POINT ( 'NONE',  ( 0.1958661417322836440, -0.3392501089628017219, -1.186351706036745446 ) ) ;
#5962=CARTESIAN_POINT ( 'NONE',  ( -0.1049643490035301746, -0.3917322834645670659, -0.6246526002286596491 ) ) ;
#5969=VERTEX_POINT ( 'NONE', #1003 ) ;
#5970=CARTESIAN_POINT ( 'NONE',  ( 0.3392501089628018884, -0.1958661417322833942, -1.991489132054804934 ) ) ;
#5977=CARTESIAN_POINT ( 'NONE',  ( -0.3392501089628017219, -0.1958661417322836718, -1.239501312335958172 ) ) ;
#5983=CARTESIAN_POINT ( 'NONE',  ( -0.004548682155566147710, 0.3974711515625344305, 1.060393565926956833E-17 ) ) ;
#5987=CARTESIAN_POINT ( 'NONE',  ( 0.1049643490035303689, 0.3917322834645670104, -2.820209973753280419 ) ) ;
#5994=CARTESIAN_POINT ( 'NONE',  ( 0.2867679344610365999, 0.2867679344610365999, -1.167322834645669438 ) ) ;
#5995=CARTESIAN_POINT ( 'NONE',  ( 0.4091458600556403535, 0.2362204724409449896, -0.3654855643044619407 ) ) ;
#6000=CARTESIAN_POINT ( 'NONE',  ( 0.2891555358219910499, -0.2891555358219909944, 0.1397637795275590844 ) ) ;
#6010=CARTESIAN_POINT ( 'NONE',  ( -0.3996062992125986590, 0.1070741851644051723, -0.4245406824146981672 ) ) ;
#6012=CARTESIAN_POINT ( 'NONE',  ( 0.2867679344610365999, 0.2867679344610365999, -0.4448818897637794589 ) ) ;
#6025=CARTESIAN_POINT ( 'NONE',  ( 0.1049643490035304799, -0.3917322834645670104, -1.026922202920946825 ) ) ;
#6030=CARTESIAN_POINT ( 'NONE',  ( 0.4091458600556403535, 0.2362204724409449896, -2.255249343832020692 ) ) ;
#6048=CARTESIAN_POINT ( 'NONE',  ( 0.1998031496062992740, 0.3460692066303959757, -0.4593175853018372501 ) ) ;
#6049=CARTESIAN_POINT ( 'NONE',  ( -0.3996062992125985480, -7.340648628747423112E-17, -2.478346456692913868 ) ) ;
#6054=CARTESIAN_POINT ( 'NONE',  ( -0.1070741851644056997, 0.3996062992125986035, -2.211286089238845065 ) ) ;
#6056=CARTESIAN_POINT ( 'NONE',  ( -0.1058382717557497937, -0.3949938075777411628, -1.489501312335957950 ) ) ;
#6057=CARTESIAN_POINT ( 'NONE',  ( 0.1070741851644053527, 0.3996062992125986590, -2.828083989501312345 ) ) ;
#6059=CARTESIAN_POINT ( 'NONE',  ( -9.594673741351313045E-17, 0.3917322834645670104, -0.6220472440944880832 ) ) ;
#6062=CARTESIAN_POINT ( 'NONE',  ( -0.3949938075777411073, 0.1058382717557497660, -2.471784776902887337 ) ) ;
#6066=CARTESIAN_POINT ( 'NONE',  ( 0.3458507752293908943, 0.3458507752293908943, -2.657480314960630530 ) ) ;
#6067=CARTESIAN_POINT ( 'NONE',  ( -0.1998031496062994683, 0.3460692066303958092, -2.375328083989501238 ) ) ;
#6068=CARTESIAN_POINT ( 'NONE',  ( 0.000000000000000000, 0.000000000000000000, -2.755905511811024056 ) ) ;
#6073=CARTESIAN_POINT ( 'NONE',  ( -0.1049643490035307020, 0.3917322834645669549, 0.06627296587926499727 ) ) ;
#6081=CARTESIAN_POINT ( 'NONE',  ( 0.3917322834645670104, -0.1049643490035303411, -0.6686351706036747222 ) ) ;
#6082=CARTESIAN_POINT ( 'NONE',  ( 0.3917322834645669549, 0.1049643490035304660, -1.376640419947506189 ) ) ;
#6083=CARTESIAN_POINT ( 'NONE',  ( -0.1958661417322836718, 0.3392501089628017219, -2.682414698162729483 ) ) ;
#6085=CARTESIAN_POINT ( 'NONE',  ( -0.3996062992125986035, -7.340648628747425578E-17, -0.1968503937007874405 ) ) ;
#6089=CARTESIAN_POINT ( 'NONE',  ( 0.3460692066303959757, -0.1998031496062991907, -1.522309711286089273 ) ) ;
#6091=CARTESIAN_POINT ( 'NONE',  ( 0.4724409448818898682, 2.892866454678787531E-17, -2.399606299212598604 ) ) ;
#6094=CARTESIAN_POINT ( 'NONE',  ( -0.3392501089628019995, 0.1958661417322832277, -0.7408136482939633449 ) ) ;
#6104=CARTESIAN_POINT ( 'NONE',  ( -0.4091458600556405756, 0.2362204724409446288, -1.916010498687664043 ) ) ;
#6110=EDGE_LOOP ( 'NONE', ( #77754, #42485, #48014, #57282 ) ) ;
#6115=CARTESIAN_POINT ( 'NONE',  ( 4.797336870675655290E-17, -0.3917322834645669549, -0.6312142800186859581 ) ) ;
#6117=CARTESIAN_POINT ( 'NONE',  ( -0.3917322834645671215, 0.1049643490035301469, -0.9048556430446195176 ) ) ;
#6122=CARTESIAN_POINT ( 'NONE',  ( -0.1958661417322834220, -0.3392501089628018884, -2.892388451443569153 ) ) ;
#6125=CARTESIAN_POINT ( 'NONE',  ( 0.2362204724409449064, 0.4091458600556404646, -1.008530183727034180 ) ) ;
#6137=CARTESIAN_POINT ( 'NONE',  ( -9.787531504996566615E-17, 0.3996062992125985480, -2.281496062992125928 ) ) ;
#6141=CARTESIAN_POINT ( 'NONE',  ( -9.787531504996566615E-17, 0.3996062992125985480, -1.336614173228346525 ) ) ;
#6146=CARTESIAN_POINT ( 'NONE',  ( -0.4724409448818896462, -0.1265901696524993070, -0.04593175853018372640 ) ) ;
#6148=CARTESIAN_POINT ( 'NONE',  ( -9.787531504996566615E-17, 0.3996062992125985480, -0.5492125984251968740 ) ) ;
#6149=CARTESIAN_POINT ( 'NONE',  ( 0.3460692066303959202, 0.1998031496062993295, -0.7611548556430446366 ) ) ;
#6150=CARTESIAN_POINT ( 'NONE',  ( -0.3949938075777409408, -0.1058382717557502933, -0.2034120734908137218 ) ) ;
#6155=CARTESIAN_POINT ( 'NONE',  ( 5.785732909357575061E-17, -0.4724409448818898682, -2.360236220472441193 ) ) ;
#6156=CARTESIAN_POINT ( 'NONE',  ( 0.2891555358219910499, -0.2891555358219909944, -1.277559055118109965 ) ) ;
#6161=CARTESIAN_POINT ( 'NONE',  ( 0.4091458600556404646, -0.2362204724409448231, -1.679790026246719137 ) ) ;
#6162=CARTESIAN_POINT ( 'NONE',  ( -0.1998031496062994683, 0.3460692066303958092, -2.690288713910760965 ) ) ;
#6169=CARTESIAN_POINT ( 'NONE',  ( 0.1049643490035303689, 0.3917322834645668994, -2.120715592354644130 ) ) ;
#6176=CARTESIAN_POINT ( 'NONE',  ( 0.3392501089628018329, 0.1958661417322835607, -1.540682414698162805 ) ) ;
#6179=CARTESIAN_POINT ( 'NONE',  ( 0.1058382717557499880, 0.3949938075777411073, -1.883202099737532720 ) ) ;
#6180=ORIENTED_EDGE ( 'NONE', *, *, #54557, .T. ) ;
#6184=CARTESIAN_POINT ( 'NONE',  ( -0.2925321140481930704, -0.2925321140481933480, -0.3740157480314960092 ) ) ;
#6191=CARTESIAN_POINT ( 'NONE',  ( -9.594673741351313045E-17, 0.3917322834645670104, -0.2421259842519686289 ) ) ;
#6198=CARTESIAN_POINT ( 'NONE',  ( -0.2925321140481932369, 0.2925321140481931259, -1.828740157480315265 ) ) ;
#6203=CARTESIAN_POINT ( 'NONE',  ( -0.4091458600556405756, 0.2362204724409446288, -0.6561679790026246906 ) ) ;
#6205=CARTESIAN_POINT ( 'NONE',  ( -0.1958661417322834220, -0.3392501089628018884, -2.827427821522309426 ) ) ;
#6207=CARTESIAN_POINT ( 'NONE',  ( -0.2867679344610364334, -0.2867679344610367109, -2.190944881889763440 ) ) ;
#6212=CARTESIAN_POINT ( 'NONE',  ( -0.3458507752293906723, -0.3458507752293910609, -2.812992125984251857 ) ) ;
#6215=CARTESIAN_POINT ( 'NONE',  ( 0.3420746716998660508, 0.1974969037888705814, -2.097769028871391495 ) ) ;
#6222=CARTESIAN_POINT ( 'NONE',  ( -0.1958661417322836718, 0.3392501089628017219, -1.422572178477690574 ) ) ;
#6226=CARTESIAN_POINT ( 'NONE',  ( 0.3458507752293908943, -0.3458507752293908943, 0.1397637795275590289 ) ) ;
#6237=CARTESIAN_POINT ( 'NONE',  ( 4.893765752498283308E-17, -0.3996062992125985480, -1.100393700787401619 ) ) ;
#6238=CARTESIAN_POINT ( 'NONE',  ( 0.2867679344610365999, 0.2867679344610365999, -2.427165354330708347 ) ) ;
#6249=CARTESIAN_POINT ( 'NONE',  ( -0.1958661417322833942, -0.3392501089628018884, -2.109599368275277609 ) ) ;
#6255=CARTESIAN_POINT ( 'NONE',  ( -0.1049643490035307020, 0.3917322834645669549, -2.138451443569553412 ) ) ;
#6256=CARTESIAN_POINT ( 'NONE',  ( -0.03611438844013053345, 0.3902087894128228873, -1.220472440944881498 ) ) ;
#6262=CARTESIAN_POINT ( 'NONE',  ( -0.1070741851644051862, -0.3996062992125986035, -2.668635170603674833 ) ) ;
#6264=CARTESIAN_POINT ( 'NONE',  ( 0.3460692066303959202, 0.1998031496062993295, -1.233595800524934338 ) ) ;
#6266=CARTESIAN_POINT ( 'NONE',  ( -0.3917322834645671770, 0.1049643490035302024, -0.02954687483695727160 ) ) ;
#6280=CARTESIAN_POINT ( 'NONE',  ( 0.3917322834645670104, -0.1049643490035303411, -0.2611548556430445256 ) ) ;
#6282=EDGE_LOOP ( 'NONE', ( #33449, #15016, #81145, #15753 ) ) ;
#6283=CARTESIAN_POINT ( 'NONE',  ( -0.3949938075777409963, -7.255918531996591613E-17, -0.5118110236220473341 ) ) ;
#6291=CARTESIAN_POINT ( 'NONE',  ( -0.2867679344610367109, 0.2867679344610365444, -1.591226664863204077 ) ) ;
#6293=CARTESIAN_POINT ( 'NONE',  ( 0.3917322834645669549, 0.1049643490035304660, -2.571522309711286258 ) ) ;
#6297=CARTESIAN_POINT ( 'NONE',  ( 0.1070741851644054915, -0.3996062992125986035, -1.030183727034120533 ) ) ;
#6299=CARTESIAN_POINT ( 'NONE',  ( -0.2925321140481930149, -0.2925321140481933480, -0.1358267716535432879 ) ) ;
#6300=CARTESIAN_POINT ( 'NONE',  ( -0.1998031496062994405, 0.3460692066303957537, -0.08989501312335959615 ) ) ;
#6302=CARTESIAN_POINT ( 'NONE',  ( -0.1070741851644051862, -0.3996062992125987146, -2.906824146981627610 ) ) ;
#6303=CARTESIAN_POINT ( 'NONE',  ( -0.1049643490035302024, -0.3917322834645671215, -1.731627296587926468 ) ) ;
#6308=CARTESIAN_POINT ( 'NONE',  ( -0.3458507752293906723, -0.3458507752293910609, -1.553149606299212726 ) ) ;
#6311=CARTESIAN_POINT ( 'NONE',  ( -0.2891555358219911054, 0.2891555358219909388, -1.041338582677165503 ) ) ;
#6322=CARTESIAN_POINT ( 'NONE',  ( 0.2925321140481932369, 0.2925321140481932369, -2.261811023622047223 ) ) ;
#6326=CARTESIAN_POINT ( 'NONE',  ( 0.2867679344610365999, 0.2867679344610365999, -1.792631602853332007 ) ) ;
#6340=CARTESIAN_POINT ( 'NONE',  ( -0.2925321140481930149, -0.2925321140481933480, 0.02165354330708659653 ) ) ;
#6342=CARTESIAN_POINT ( 'NONE',  ( 0.2867679344610365999, -0.2867679344610365444, -0.8129921259842518566 ) ) ;
#6363=CARTESIAN_POINT ( 'NONE',  ( -0.1958661417322834220, -0.3392501089628018884, -2.577427821522309426 ) ) ;
#6366=CARTESIAN_POINT ( 'NONE',  ( 0.3458507752293908943, -0.3458507752293908943, -0.4133858267716534196 ) ) ;
#6367=CARTESIAN_POINT ( 'NONE',  ( 0.3996062992125986035, 2.446882876249141962E-17, -0.2755905511811024278 ) ) ;
#6370=CARTESIAN_POINT ( 'NONE',  ( 0.3917322834645670104, 2.398668435337828261E-17, -1.685039370078740051 ) ) ;
#6379=CARTESIAN_POINT ( 'NONE',  ( -0.1049643490035306742, 0.3917322834645668994, -0.5590358023283972244 ) ) ;
#6387=CARTESIAN_POINT ( 'NONE',  ( 4.797336870675656522E-17, -0.3917322834645670659, -2.122722727855329783 ) ) ;
#6389=ORIENTED_EDGE ( 'NONE', *, *, #38792, .F. ) ;
#6395=CARTESIAN_POINT ( 'NONE',  ( -0.3392501089628017219, -0.1958661417322836718, -1.396981627296587813 ) ) ;
#6399=CARTESIAN_POINT ( 'NONE',  ( -0.04037479286078369395, 0.3917864676224473985, 9.485496803828532453E-13 ) ) ;
#6401=CARTESIAN_POINT ( 'NONE',  ( 0.1265901696524990572, -0.4724409448818897017, -0.9494750656167977310 ) ) ;
#6410=CARTESIAN_POINT ( 'NONE',  ( 5.785732909357575061E-17, -0.4724409448818898682, -0.3937007874015748254 ) ) ;
#6411=CARTESIAN_POINT ( 'NONE',  ( -0.2867679344610365999, 0.2867679344610364889, -1.206692913385826627 ) ) ;
#6412=CARTESIAN_POINT ( 'NONE',  ( 0.4724409448818898682, 2.892866454678787531E-17, -0.3523622047244094335 ) ) ;
#6416=CARTESIAN_POINT ( 'NONE',  ( 0.3949938075777408852, 0.1058382717557500435, 0.1135170603674540979 ) ) ;
#6421=CARTESIAN_POINT ( 'NONE',  ( 0.1058382717557499880, 0.3949938075777409408, 0.08727034120734906975 ) ) ;
#6428=CARTESIAN_POINT ( 'NONE',  ( -0.1998031496062991630, -0.3460692066303959202, -1.087270341207349000 ) ) ;
#6430=CARTESIAN_POINT ( 'NONE',  ( -9.594673741351313045E-17, 0.3917322834645670104, -0.1496062992125983815 ) ) ;
#6443=CARTESIAN_POINT ( 'NONE',  ( 0.3917322834645670104, 0.1049643490035304660, -0.9088119667004745938 ) ) ;
#6448=CARTESIAN_POINT ( 'NONE',  ( 0.3458507752293908943, 0.3458507752293908943, -2.261811023622047223 ) ) ;
#6465=CARTESIAN_POINT ( 'NONE',  ( 0.3460692066303959202, 0.1998031496062993295, -0.2887139107611548794 ) ) ;
#6466=CARTESIAN_POINT ( 'NONE',  ( -0.3460692066303957537, -0.1998031496062994405, -2.491469816272966042 ) ) ;
#6472=CARTESIAN_POINT ( 'NONE',  ( 0.2925321140481932369, -0.2925321140481932369, -2.303149606299212060 ) ) ;
#6473=CARTESIAN_POINT ( 'NONE',  ( 0.2891555358219910499, 0.2891555358219910499, -2.027559055118110631 ) ) ;
#6474=CARTESIAN_POINT ( 'NONE',  ( 0.3460692066303959757, -0.1998031496062991907, -2.939632545931758489 ) ) ;
#6476=CARTESIAN_POINT ( 'NONE',  ( 0.1049643490035303689, 0.3917322834645670104, -0.9304461942257216123 ) ) ;
#6480=CARTESIAN_POINT ( 'NONE',  ( 0.1974969037888704704, 0.3420746716998660508, -2.740813648293963567 ) ) ;
#6485=CARTESIAN_POINT ( 'NONE',  ( 0.3460692066303959757, -0.1998031496062991907, -2.152230971128608950 ) ) ;
#6486=CARTESIAN_POINT ( 'NONE',  ( 0.3917322834645670659, 2.398668435337828261E-17, -0.7447699719498183102 ) ) ;
#6492=CARTESIAN_POINT ( 'NONE',  ( -0.3917322834645671215, 0.1049643490035301469, -0.2749343832020998413 ) ) ;
#6500=CARTESIAN_POINT ( 'NONE',  ( -0.1958661417322836718, 0.3392501089628017219, -0.4127296587926510552 ) ) ;
#6501=CARTESIAN_POINT ( 'NONE',  ( 0.2867679344610365999, -0.2867679344610365444, -1.665354330708661124 ) ) ;
#6502=CARTESIAN_POINT ( 'NONE',  ( -0.3917322834645670104, -7.196005306013484475E-17, -2.551181102362204633 ) ) ;
#6504=CARTESIAN_POINT ( 'NONE',  ( -0.1998031496062994683, 0.3460692066303958092, 0.1443569553805774119 ) ) ;
#6509=CARTESIAN_POINT ( 'NONE',  ( -9.787531504996567848E-17, 0.3996062992125986035, -1.259842519685039353 ) ) ;
#6513=CARTESIAN_POINT ( 'NONE',  ( 0.2362204724409451007, -0.4091458600556402980, -1.194225721784776928 ) ) ;
#6514=CARTESIAN_POINT ( 'NONE',  ( 0.1049643490035303689, 0.3917322834645670104, -1.022965879265091749 ) ) ;
#6523=CARTESIAN_POINT ( 'NONE',  ( -0.4091458600556405756, 0.2362204724409446288, -2.073490813648294129 ) ) ;
#6525=FACE_OUTER_BOUND ( 'NONE', #47789, .T. ) ;
#6531=CARTESIAN_POINT ( 'NONE',  ( 0.4724409448818898682, 2.892866454678787531E-17, -2.714566929133858331 ) ) ;
#6534=CARTESIAN_POINT ( 'NONE',  ( 0.2867679344610365999, -0.2867679344610365999, -0.6508993193887645523 ) ) ;
#6536=CARTESIAN_POINT ( 'NONE',  ( -0.3392501089628017219, -0.1958661417322836718, -0.9245406824146982228 ) ) ;
#6541=CARTESIAN_POINT ( 'NONE',  ( 0.1958661417322834775, 0.3392501089628018884, -2.813648293963254776 ) ) ;
#6544=CARTESIAN_POINT ( 'NONE',  ( 0.3458507752293908943, 0.3458507752293908943, -1.159448818897637734 ) ) ;
#6556=CARTESIAN_POINT ( 'NONE',  ( 4.893765752498283308E-17, -0.3996062992125985480, -2.360236220472441193 ) ) ;
#6560=CARTESIAN_POINT ( 'NONE',  ( 4.893765752498283308E-17, -0.3996062992125985480, -1.415354330708661568 ) ) ;
#6566=CARTESIAN_POINT ( 'NONE',  ( -0.3460692066303960313, 0.1998031496062989965, -0.5754593175853018883 ) ) ;
#6567=ADVANCED_FACE ( 'NONE', ( #54813 ), #80515, .F. ) ;
#6568=CARTESIAN_POINT ( 'NONE',  ( -0.3460692066303960868, 0.1998031496062990242, -0.8136482939632546652 ) ) ;
#6569=CARTESIAN_POINT ( 'NONE',  ( 4.837279021331060870E-17, -0.3949938075777409963, -0.2362204724409449619 ) ) ;
#6575=CARTESIAN_POINT ( 'NONE',  ( 0.3420746716998660508, 0.1974969037888705814, -1.152887139107611425 ) ) ;
#6580=CARTESIAN_POINT ( 'NONE',  ( -0.4724409448818895907, -0.1265901696524993070, -1.463254593175853158 ) ) ;
#6581=CARTESIAN_POINT ( 'NONE',  ( -0.3996062992125985480, -0.1070741851644057135, -2.723097112860891844 ) ) ;
#6583=VERTEX_POINT ( 'NONE', #52 ) ;
#6588=CARTESIAN_POINT ( 'NONE',  ( -0.2867679344610364334, -0.2867679344610368219, -2.186332390254906777 ) ) ;
#6589=CARTESIAN_POINT ( 'NONE',  ( -0.2925321140481930149, -0.2925321140481933480, -2.812992125984251857 ) ) ;
#6594=CARTESIAN_POINT ( 'NONE',  ( 4.797336870675656522E-17, -0.3917322834645670104, -1.645669291338582640 ) ) ;
#6597=CARTESIAN_POINT ( 'NONE',  ( -0.2891555358219911054, 0.2891555358219909388, -1.909448818897637956 ) ) ;
#6602=CARTESIAN_POINT ( 'NONE',  ( 0.1070741851644053527, 0.3996062992125986590, 0.006561679790026237087 ) ) ;
#6606=FACE_OUTER_BOUND ( 'NONE', #58034, .T. ) ;
#6609=CARTESIAN_POINT ( 'NONE',  ( 0.3392501089628018884, -0.1958661417322834220, -0.3471128608923885195 ) ) ;
#6614=ORIENTED_EDGE ( 'NONE', *, *, #13640, .F. ) ;
#6616=CARTESIAN_POINT ( 'NONE',  ( -0.1998031496062991630, -0.3460692066303959202, -1.874671916010498762 ) ) ;
#6621=CARTESIAN_POINT ( 'NONE',  ( -0.2362204724409451284, 0.4091458600556402425, -0.8005249343832020470 ) ) ;
#6623=CARTESIAN_POINT ( 'NONE',  ( -0.1049643490035302024, -0.3917322834645671215, -0.3792650918635169233 ) ) ;
#6627=CARTESIAN_POINT ( 'NONE',  ( 0.4091458600556403535, 0.2362204724409449896, -2.727690288713910949 ) ) ;
#6631=CARTESIAN_POINT ( 'NONE',  ( 0.2891555358219910499, 0.2891555358219910499, -2.576771653543307838 ) ) ;
#6639=CARTESIAN_POINT ( 'NONE',  ( -0.3392501089628019995, 0.1958661417322832277, -1.435695538057742970 ) ) ;
#6642=CARTESIAN_POINT ( 'NONE',  ( 0.2362204724409449064, 0.4091458600556404646, 0.09383202099737532331 ) ) ;
#6654=CARTESIAN_POINT ( 'NONE',  ( 4.893765752498283308E-17, -0.3996062992125985480, -1.257874015748031260 ) ) ;
#6656=CARTESIAN_POINT ( 'NONE',  ( 0.1958661417322836440, -0.3392501089628017219, -2.696194225721784576 ) ) ;
#6667=CARTESIAN_POINT ( 'NONE',  ( -0.1070741851644056997, 0.3996062992125986035, 0.1509186351706036100 ) ) ;
#6669=CARTESIAN_POINT ( 'NONE',  ( 0.2867679344610366554, -0.2867679344610365999, -2.142407767225408932 ) ) ;
#6675=CARTESIAN_POINT ( 'NONE',  ( 0.3917322834645669549, 0.1049643490035304660, -1.941601049868766582 ) ) ;
#6683=CARTESIAN_POINT ( 'NONE',  ( 0.3996062992125986035, 2.446882876249141962E-17, -1.377952755905511806 ) ) ;
#6685=CARTESIAN_POINT ( 'NONE',  ( -0.3392501089628017219, -0.1958661417322836995, -0.04923191420703601495 ) ) ;
#6699=CARTESIAN_POINT ( 'NONE',  ( -0.3917322834645669549, -0.1049643490035306603, -0.03805774278215218187 ) ) ;
#6702=CARTESIAN_POINT ( 'NONE',  ( -0.3949938075777411628, 0.1058382717557497937, -0.5052493438320211361 ) ) ;
#6709=CARTESIAN_POINT ( 'NONE',  ( -9.594673741351313045E-17, 0.3917322834645670659, -1.571541625493125149 ) ) ;
#6715=CARTESIAN_POINT ( 'NONE',  ( -0.3460692066303958092, -0.1998031496062994683, -1.312335958005249381 ) ) ;
#6717=CARTESIAN_POINT ( 'NONE',  ( -0.1070741851644051862, -0.3996062992125986590, -0.9363517060367454459 ) ) ;
#6718=CARTESIAN_POINT ( 'NONE',  ( -0.1998031496062991630, -0.3460692066303959202, -0.1423884514435695692 ) ) ;
#6720=CARTESIAN_POINT ( 'NONE',  ( 0.1998031496062994405, -0.3460692066303958092, -2.769028871391076230 ) ) ;
#6721=CARTESIAN_POINT ( 'NONE',  ( 0.3392501089628018329, 0.1958661417322835607, -1.633202099737532942 ) ) ;
#6727=CARTESIAN_POINT ( 'NONE',  ( -0.3458507752293909498, 0.3458507752293907833, -1.356299212598425230 ) ) ;
#6730=CARTESIAN_POINT ( 'NONE',  ( -0.1974969037888706924, 0.3420746716998658843, -1.349737532808398921 ) ) ;
#6740=CARTESIAN_POINT ( 'NONE',  ( -0.1070741851644051862, -0.3996062992125986590, -2.038713910761154491 ) ) ;
#6742=CARTESIAN_POINT ( 'NONE',  ( -0.3392501089628019439, 0.1958661417322832554, -1.681083046422885197 ) ) ;
#6753=CARTESIAN_POINT ( 'NONE',  ( 0.1070741851644054776, -0.3996062992125984925, 0.1528871391076115360 ) ) ;
#6755=CARTESIAN_POINT ( 'NONE',  ( -0.3392501089628019995, 0.1958661417322832277, -1.528215223097112885 ) ) ;
#6764=CARTESIAN_POINT ( 'NONE',  ( -0.3458507752293906723, -0.3458507752293910609, -2.578740157480315265 ) ) ;
#6776=CARTESIAN_POINT ( 'NONE',  ( 0.3917322834645670104, 2.398668435337828261E-17, -2.314960629921259727 ) ) ;
#6779=CARTESIAN_POINT ( 'NONE',  ( -0.3458507752293909498, 0.3458507752293907833, -0.6496062992125984925 ) ) ;
#6780=CARTESIAN_POINT ( 'NONE',  ( -0.1998031496062994683, 0.3460692066303958092, -0.1706036745406824540 ) ) ;
#6783=CARTESIAN_POINT ( 'NONE',  ( 0.3917322834645669549, 0.1049643490035304660, -1.849081364829396223 ) ) ;
#6795=CARTESIAN_POINT ( 'NONE',  ( -0.3917322834645670659, 0.1049643490035301607, -1.057723466370391829 ) ) ;
#6802=CARTESIAN_POINT ( 'NONE',  ( 0.1958661417322836718, -0.3392501089628017219, -2.293326402396012487 ) ) ;
#6810=CARTESIAN_POINT ( 'NONE',  ( 0.3917322834645669549, 0.1049643490035304660, -1.941601049868766582 ) ) ;
#6822=EDGE_CURVE ( 'NONE', #55042, #62471, #74745, .T. ) ;
#6823=ORIENTED_EDGE ( 'NONE', *, *, #5521, .F. ) ;
#6828=CARTESIAN_POINT ( 'NONE',  ( -0.2362204724409451284, 0.4091458600556402425, -0.2473753280839895152 ) ) ;
#6831=CARTESIAN_POINT ( 'NONE',  ( -0.3460692066303957537, -0.1998031496062994405, -2.806430446194225770 ) ) ;
#6836=CARTESIAN_POINT ( 'NONE',  ( 0.3420746716998660508, -0.1974969037888704149, -0.02427821522309712640 ) ) ;
#6844=CARTESIAN_POINT ( 'NONE',  ( -0.1070741851644056997, 0.3996062992125984925, -1.028215223097112663 ) ) ;
#6846=CARTESIAN_POINT ( 'NONE',  ( 0.1958661417322836440, -0.3392501089628017219, -0.5564304461942257696 ) ) ;
#6862=CARTESIAN_POINT ( 'NONE',  ( 0.4091458600556403535, 0.2362204724409449896, -2.570209973753280863 ) ) ;
#6879=CARTESIAN_POINT ( 'NONE',  ( 0.3460692066303959757, -0.1998031496062991907, -0.4199475065616797842 ) ) ;
#6885=CARTESIAN_POINT ( 'NONE',  ( 0.2925321140481932369, -0.2925321140481932369, -2.775590551181101429 ) ) ;
#6886=CARTESIAN_POINT ( 'NONE',  ( -0.3949938075777409963, -7.255918531996591613E-17, -1.929133858267716439 ) ) ;
#6887=CARTESIAN_POINT ( 'NONE',  ( -0.3392501089628017219, -0.1958661417322836718, -0.5170603674540682482 ) ) ;
#6889=CARTESIAN_POINT ( 'NONE',  ( 0.3917322834645669549, 0.1049643490035304660, -0.9041994750656167090 ) ) ;
#6890=EDGE_CURVE ( 'NONE', #49627, #80266, #43488, .T. ) ;
#6892=CARTESIAN_POINT ( 'NONE',  ( -9.594673741351313045E-17, 0.3917322834645670104, -1.251968503937008093 ) ) ;
#6894=CARTESIAN_POINT ( 'NONE',  ( 0.3392501089628018329, 0.1958661417322835052, 0.1036938564642537891 ) ) ;
#6898=CARTESIAN_POINT ( 'NONE',  ( -0.3458507752293909498, 0.3458507752293907833, -2.854330708661417138 ) ) ;
#6899=CARTESIAN_POINT ( 'NONE',  ( 0.3996062992125986035, 2.446882876249141962E-17, -2.480314960629921295 ) ) ;
#6900=CARTESIAN_POINT ( 'NONE',  ( -0.3917322834645671770, 0.1049643490035302024, -1.131909079561366882 ) ) ;
#6906=CARTESIAN_POINT ( 'NONE',  ( -0.1049643490035302024, -0.3917322834645671215, 0.0006561679790025351077 ) ) ;
#6915=CARTESIAN_POINT ( 'NONE',  ( -0.1049643490035302024, -0.3917322834645671215, -0.4717847769028871152 ) ) ;
#6916=CARTESIAN_POINT ( 'NONE',  ( 0.2867679344610365999, 0.2867679344610365999, -1.862204724409449064 ) ) ;
#6917=CARTESIAN_POINT ( 'NONE',  ( -0.3917322834645670104, -7.196005306013484475E-17, -2.708661417322834275 ) ) ;
#6919=CARTESIAN_POINT ( 'NONE',  ( 0.1070741851644054915, -0.3996062992125986035, -0.08530183727034119923 ) ) ;
#6923=CARTESIAN_POINT ( 'NONE',  ( 0.1070741851644054915, -0.3996062992125986035, -1.975065616797900381 ) ) ;
#6926=CARTESIAN_POINT ( 'NONE',  ( 0.3957358693849762354, 0.01930322177395801808, -1.929133858268277546 ) ) ;
#6927=CARTESIAN_POINT ( 'NONE',  ( 0.1049643490035303689, 0.3917322834645670104, -0.8654855643044619962 ) ) ;
#6947=CARTESIAN_POINT ( 'NONE',  ( -0.1049643490035306742, 0.3917322834645668994, -0.8739964322496570626 ) ) ;
#6950=CARTESIAN_POINT ( 'NONE',  ( 0.1958661417322834775, 0.3392501089628018884, -1.173884514435695525 ) ) ;
#6956=CARTESIAN_POINT ( 'NONE',  ( -0.3917322834645671215, 0.1049643490035301469, -2.859580052493438274 ) ) ;
#6959=CARTESIAN_POINT ( 'NONE',  ( 0.1265901696524989462, 0.4724409448818897572, -1.172572178477690352 ) ) ;
#6974=CARTESIAN_POINT ( 'NONE',  ( -0.2925321140481932369, 0.2925321140481931259, -2.301181102362204633 ) ) ;
#6978=CARTESIAN_POINT ( 'NONE',  ( 0.1998031496062994128, -0.3460692066303957537, -1.900918635170603999 ) ) ;
#6984=CARTESIAN_POINT ( 'NONE',  ( -0.3996062992125984925, -0.1070741851644056719, -1.067585301837270517 ) ) ;
#6985=CARTESIAN_POINT ( 'NONE',  ( -0.3460692066303960868, 0.1998031496062990242, -0.9711286089238845287 ) ) ;
#6987=CARTESIAN_POINT ( 'NONE',  ( -0.1058382717557503211, 0.3949938075777409408, -0.4790026246719162328 ) ) ;
#6993=CARTESIAN_POINT ( 'NONE',  ( -0.3420746716998660508, -0.1974969037888706924, -1.389107611548556553 ) ) ;
#6999=CARTESIAN_POINT ( 'NONE',  ( 0.2362204724409449064, 0.4091458600556404646, -1.719160104986876769 ) ) ;
#7001=ORIENTED_EDGE ( 'NONE', *, *, #4428, .F. ) ;
#7007=CARTESIAN_POINT ( 'NONE',  ( -0.1958661417322836440, 0.3392501089628016664, -1.825440001803462886 ) ) ;
#7008=CARTESIAN_POINT ( 'NONE',  ( -0.3996062992125986590, 0.1070741851644051723, -2.786745406824146620 ) ) ;
#7014=CARTESIAN_POINT ( 'NONE',  ( 0.1049643490035303689, 0.3917322834645670104, -1.402887139107611647 ) ) ;
#7017=CARTESIAN_POINT ( 'NONE',  ( -0.2891555358219908833, -0.2891555358219912164, -1.948818897637795144 ) ) ;
#7022=CARTESIAN_POINT ( 'NONE',  ( 4.893765752498283924E-17, -0.3996062992125986035, -0.07874015748031498729 ) ) ;
#7027=CARTESIAN_POINT ( 'NONE',  ( -0.2867679344610365999, 0.2867679344610364889, 0.2106299212598424508 ) ) ;
#7030=CARTESIAN_POINT ( 'NONE',  ( -0.2867679344610364334, -0.2867679344610367109, -0.3011811023622048000 ) ) ;
#7037=CARTESIAN_POINT ( 'NONE',  ( 0.1070741851644053388, 0.3996062992125986035, -1.802493438320209584 ) ) ;
#7043=CARTESIAN_POINT ( 'NONE',  ( 0.1265901696524989462, 0.4724409448818897572, -0.7808398950131233418 ) ) ;
#7045=CARTESIAN_POINT ( 'NONE',  ( 0.1049643490035303689, 0.3917322834645670104, -0.1430446194225721002 ) ) ;
#7046=CARTESIAN_POINT ( 'NONE',  ( 0.1049643490035303689, 0.3917322834645670104, -1.967847769028871374 ) ) ;
#7050=CARTESIAN_POINT ( 'NONE',  ( -0.1070741851644056997, 0.3996062992125984925, 0.2316272965879264956 ) ) ;
#7056=CARTESIAN_POINT ( 'NONE',  ( -0.3420746716998660508, -0.1974969037888706924, -2.648950131233596128 ) ) ;
#7058=CARTESIAN_POINT ( 'NONE',  ( 0.000000000000000000, 0.000000000000000000, -2.755905511811024056 ) ) ;
#7063=CARTESIAN_POINT ( 'NONE',  ( 0.1958661417322834775, 0.3392501089628018884, -1.553805774278215202 ) ) ;
#7066=CARTESIAN_POINT ( 'NONE',  ( -0.1265901696524986964, -0.4724409448818899238, 0.008530183727034111943 ) ) ;
#7078=CARTESIAN_POINT ( 'NONE',  ( -0.1998031496062994405, 0.3460692066303957537, -1.192257217847769057 ) ) ;
#7079=CARTESIAN_POINT ( 'NONE',  ( -9.594673741351313045E-17, 0.3917322834645670104, -2.604330708661416693 ) ) ;
#7090=CARTESIAN_POINT ( 'NONE',  ( 0.2867679344610366554, -0.2867679344610365999, -2.457368397146668659 ) ) ;
#7096=CARTESIAN_POINT ( 'NONE',  ( -0.3392501089628017219, -0.1958661417322836718, -2.026902887139107712 ) ) ;
#7101=CARTESIAN_POINT ( 'NONE',  ( -0.03178304480585582292, 0.3983403474834776858, -2.755905511811024500 ) ) ;
#7103=CARTESIAN_POINT ( 'NONE',  ( -0.3460692066303960868, 0.1998031496062990242, -1.286089238845144367 ) ) ;
#7105=CARTESIAN_POINT ( 'NONE',  ( 0.3917322834645670659, -0.1049643490035303273, -0.1082870323172722415 ) ) ;
#7118=CARTESIAN_POINT ( 'NONE',  ( -0.1958661417322834220, -0.3392501089628018884, -0.3727034120734908362 ) ) ;
#7121=CARTESIAN_POINT ( 'NONE',  ( 0.3949938075777409963, 2.418639510665530435E-17, -0.7480314960629920185 ) ) ;
#7130=CARTESIAN_POINT ( 'NONE',  ( -0.4724409448818880364, -0.1265901696525023323, -2.723097112860892732 ) ) ;
#7135=CARTESIAN_POINT ( 'NONE',  ( -0.3996062992125987146, 0.1070741851644051862, -1.135170603674540590 ) ) ;
#7137=CARTESIAN_POINT ( 'NONE',  ( 0.1070741851644053388, 0.3996062992125986035, -0.7001312335958002064 ) ) ;
#7138=CARTESIAN_POINT ( 'NONE',  ( -0.3996062992125986590, 0.1070741851644051723, -0.2670603674540683037 ) ) ;
#7140=CARTESIAN_POINT ( 'NONE',  ( -0.1070741851644056997, 0.3996062992125986035, -2.683727034120735322 ) ) ;
#7141=CARTESIAN_POINT ( 'NONE',  ( 0.3917322834645669549, 0.1049643490035304660, -2.099081364829396446 ) ) ;
#7147=CARTESIAN_POINT ( 'NONE',  ( 0.4724409448818897572, -0.1265901696524988906, -1.448162729658792669 ) ) ;
#7152=CARTESIAN_POINT ( 'NONE',  ( -9.674558042662122972E-17, 0.3949938075777409963, -1.494094488188976388 ) ) ;
#7162=CARTESIAN_POINT ( 'NONE',  ( -0.3996062992125985480, -7.340648628747423112E-17, -2.320866141732283783 ) ) ;
#7164=CARTESIAN_POINT ( 'NONE',  ( 0.3392501089628018329, 0.1958661417322835052, -1.943550238023935561 ) ) ;
#7176=CARTESIAN_POINT ( 'NONE',  ( 0.1998031496062994128, -0.3460692066303957537, 0.1463254593175852825 ) ) ;
#7178=CARTESIAN_POINT ( 'NONE',  ( -0.3917322834645669549, -0.1049643490035306603, -1.547900262467191590 ) ) ;
#7199=CARTESIAN_POINT ( 'NONE',  ( -0.1049643490035307020, 0.3917322834645669549, -2.518372703412073754 ) ) ;
#7203=CARTESIAN_POINT ( 'NONE',  ( 0.4724409448818896462, 0.1265901696524990294, -0.7545931758530182165 ) ) ;
#7204=CARTESIAN_POINT ( 'NONE',  ( 0.3996062992125986590, -0.1070741851644053111, -0.1115485564304461857 ) ) ;
#7208=CARTESIAN_POINT ( 'NONE',  ( -0.2867679344610364334, -0.2867679344610367109, -1.783464566929133577 ) ) ;
#7212=CARTESIAN_POINT ( 'NONE',  ( -0.4091458600556402980, -0.2362204724409451284, -2.729658792650918375 ) ) ;
#7218=CARTESIAN_POINT ( 'NONE',  ( -0.3917322834645669549, -7.196005306013483243E-17, -1.221765461121048224 ) ) ;
#7225=CARTESIAN_POINT ( 'NONE',  ( 0.3917322834645670659, -0.1049643490035303273, -2.470491756726720833 ) ) ;
#7233=CARTESIAN_POINT ( 'NONE',  ( -0.1049643490035307020, 0.3917322834645669549, -1.980971128608924214 ) ) ;
#7237=DIRECTION ( 'NONE',  ( 1.000000000000000000, 0.000000000000000000, 0.000000000000000000 ) ) ;
#7250=CARTESIAN_POINT ( 'NONE',  ( -1.157146581871515012E-16, 0.4724409448818898682, -0.2342519685039370358 ) ) ;
#7253=CARTESIAN_POINT ( 'NONE',  ( -0.1974969037888704149, -0.3420746716998661063, 0.01509186351706036378 ) ) ;
#7259=CARTESIAN_POINT ( 'NONE',  ( -0.1974969037888704149, -0.3420746716998661063, 0.01509186351706036378 ) ) ;
#7266=CARTESIAN_POINT ( 'NONE',  ( -0.3460692066303960313, 0.1998031496062989965, -1.047900262467191590 ) ) ;
#7268=CARTESIAN_POINT ( 'NONE',  ( 0.1049643490035303689, 0.3917322834645670104, -0.4580052493438320216 ) ) ;
#7271=CARTESIAN_POINT ( 'NONE',  ( 0.3983403474834781299, 0.03178304480585100733, -1.929133858267716661 ) ) ;
#7282=CARTESIAN_POINT ( 'NONE',  ( -0.3937527723457945883, 0.009287274676460462175, -1.220472440944884163 ) ) ;
#7284=CARTESIAN_POINT ( 'NONE',  ( -0.4724409448818899238, 0.1265901696524986686, -2.629265091863517423 ) ) ;
#7301=CARTESIAN_POINT ( 'NONE',  ( 0.1998031496062992740, 0.3460692066303959757, -0.3018372703412073865 ) ) ;
#7306=CARTESIAN_POINT ( 'NONE',  ( 0.3460692066303959202, 0.1998031496062993295, -2.808398950131233640 ) ) ;
#7307=CARTESIAN_POINT ( 'NONE',  ( -0.2891555358219908833, -0.2891555358219912164, -1.948818897637795144 ) ) ;
#7308=CARTESIAN_POINT ( 'NONE',  ( -0.3917322834645669549, -0.1049643490035306603, -0.6679790026246719137 ) ) ;
#7311=CARTESIAN_POINT ( 'NONE',  ( -0.3917322834645670104, -7.196005306013484475E-17, -0.9763779527559053317 ) ) ;
#7313=CARTESIAN_POINT ( 'NONE',  ( -0.3917322834645670104, -7.196005306013484475E-17, -1.133858267716535195 ) ) ;
#7315=CARTESIAN_POINT ( 'NONE',  ( 4.837279021331061486E-17, -0.3949938075777409963, -2.832677165354331006 ) ) ;
#7321=CARTESIAN_POINT ( 'NONE',  ( 0.2925321140481932369, 0.2925321140481932369, -2.657480314960630530 ) ) ;
#7322=CARTESIAN_POINT ( 'NONE',  ( -0.2867679344610365444, -0.2867679344610367664, -1.158155798721471896 ) ) ;
#7328=CARTESIAN_POINT ( 'NONE',  ( -9.594673741351313045E-17, 0.3917322834645670104, -0.3996062992125985480 ) ) ;
#7336=CARTESIAN_POINT ( 'NONE',  ( -0.4724409448818890911, 0.1265901696525001952, -0.5820209973753279753 ) ) ;
#7337=CARTESIAN_POINT ( 'NONE',  ( 0.3392501089628018329, 0.1958661417322835607, -1.855643044619422533 ) ) ;
#7339=CARTESIAN_POINT ( 'NONE',  ( 0.3996062992125986035, 2.446882876249141962E-17, -0.1181102362204724671 ) ) ;
#7346=CARTESIAN_POINT ( 'NONE',  ( -0.2867679344610365999, 0.2867679344610364889, -1.049212598425196763 ) ) ;
#7366=CARTESIAN_POINT ( 'NONE',  ( -0.3392501089628019439, 0.1958661417322832554, -0.8936814716197357678 ) ) ;
#7369=CARTESIAN_POINT ( 'NONE',  ( -0.1049643490035301885, -0.3917322834645671215, -1.101706036745407014 ) ) ;
#7370=CARTESIAN_POINT ( 'NONE',  ( -0.1070741851644056997, 0.3996062992125984925, -0.2408136482939632061 ) ) ;
#7377=CARTESIAN_POINT ( 'NONE',  ( 0.1049643490035303967, 0.3917322834645670659, -0.1476571110574297074 ) ) ;
#7381=CARTESIAN_POINT ( 'NONE',  ( 0.3458507752293908943, 0.3458507752293908943, -1.316929133858267598 ) ) ;
#7397=CARTESIAN_POINT ( 'NONE',  ( 0.2925321140481932369, 0.2925321140481932369, -2.576771653543307394 ) ) ;
#7402=CARTESIAN_POINT ( 'NONE',  ( 4.893765752498283308E-17, -0.3996062992125985480, -1.887795275590551158 ) ) ;
#7409=CARTESIAN_POINT ( 'NONE',  ( 0.2925321140481931814, -0.2925321140481931259, -1.120078740157480324 ) ) ;
#7410=CARTESIAN_POINT ( 'NONE',  ( -0.3996062992125986035, -7.340648628747425578E-17, -1.299212598425196985 ) ) ;
#7411=CARTESIAN_POINT ( 'NONE',  ( -0.3420746716998659953, -0.1974969037888706647, -0.5249343832020998413 ) ) ;
#7417=CARTESIAN_POINT ( 'NONE',  ( -0.3420746716998662729, 0.1974969037888702206, -1.835301837270341130 ) ) ;
#7422=CARTESIAN_POINT ( 'NONE',  ( 0.3458507752293908943, -0.3458507752293908943, -1.988188976377952777 ) ) ;
#7430=CARTESIAN_POINT ( 'NONE',  ( 0.3917322834645668994, 0.1049643490035304522, -2.409429503115799065 ) ) ;
#7436=CARTESIAN_POINT ( 'NONE',  ( -0.1958661417322834220, -0.3392501089628018884, 0.1646981627296586759 ) ) ;
#7438=CARTESIAN_POINT ( 'NONE',  ( -9.594673741351313045E-17, 0.3917322834645670104, -2.039370078740157410 ) ) ;
#7441=CARTESIAN_POINT ( 'NONE',  ( 0.2891555358219910499, 0.2891555358219910499, -1.712598425196850682 ) ) ;
#7443=CARTESIAN_POINT ( 'NONE',  ( 0.000000000000000000, 0.000000000000000000, -1.220472440944881942 ) ) ;
#7447=CARTESIAN_POINT ( 'NONE',  ( -0.2925321140481930704, -0.2925321140481933480, -0.6889763779527556808 ) ) ;
#7455=CARTESIAN_POINT ( 'NONE',  ( 0.2867679344610365999, 0.2867679344610365999, -0.5374015748031496509 ) ) ;
#7462=CARTESIAN_POINT ( 'NONE',  ( 0.3460692066303958092, 0.1998031496062993018, -2.097769028871391050 ) ) ;
#7467=CARTESIAN_POINT ( 'NONE',  ( -0.4724409448818899238, 0.1265901696524986686, -1.135170603674540590 ) ) ;
#7470=CARTESIAN_POINT ( 'NONE',  ( -0.1958661417322836718, 0.3392501089628017219, -0.4776902887139107268 ) ) ;
#7475=CARTESIAN_POINT ( 'NONE',  ( -0.3996062992125985480, -7.340648628747423112E-17, -0.2736220472440945017 ) ) ;
#7477=CARTESIAN_POINT ( 'NONE',  ( 0.1265901696524990572, -0.4724409448818897017, -1.106955380577427706 ) ) ;
#7478=B_SPLINE_CURVE_WITH_KNOTS ( 'NONE', 3,
 ( #51804, #20261, #56878, #50559, #12285, #32882, #82983, #58551, #25303, #26574, #50968, #68539, #30644, #68948, #62216, #75688, #29403, #29810 ),
 .UNSPECIFIED., .F., .F.,
 ( 4, 2, 2, 2, 2, 2, 2, 2, 4 ),
 ( 2.786138856325813435E-16, 0.001588476978679812012, 0.002382715468019578481, 0.002779834712689461824, 0.002978394335024402845, 0.003077674146191874006, 0.003127314051775609369, 0.003152134004567477051, 0.003176953957359344299 ),
 .UNSPECIFIED. ) ;
#7481=CARTESIAN_POINT ( 'NONE',  ( 0.1974969037888704704, 0.3420746716998660508, -2.583333333333333481 ) ) ;
#7483=CYLINDRICAL_SURFACE ( 'NONE', #73407, 0.4724409448818898682 ) ;
#7489=CARTESIAN_POINT ( 'NONE',  ( -0.3392501089628019995, 0.1958661417322832277, -1.908136482939632561 ) ) ;
#7493=CARTESIAN_POINT ( 'NONE',  ( -0.3458507752293906723, -0.3458507752293910609, 0.1791338582677165503 ) ) ;
#7506=CARTESIAN_POINT ( 'NONE',  ( 0.3996062992125985480, 2.446882876249141654E-17, -1.297244094488188670 ) ) ;
#7507=CARTESIAN_POINT ( 'NONE',  ( 0.3917322834645670104, -0.1049643490035303411, -2.873359580052493811 ) ) ;
#7517=CARTESIAN_POINT ( 'NONE',  ( -0.3460692066303958092, -0.1998031496062994683, 0.1049868766404199322 ) ) ;
#7518=CARTESIAN_POINT ( 'NONE',  ( -9.594673741351313045E-17, 0.3917322834645670659, -2.516423515256904331 ) ) ;
#7520=CARTESIAN_POINT ( 'NONE',  ( 0.02899565511876438934, -0.3969271875946648320, -3.856971560569901962E-17 ) ) ;
#7524=CARTESIAN_POINT ( 'NONE',  ( -0.3392501089628017219, -0.1958661417322836718, -2.341863517060367439 ) ) ;
#7532=CARTESIAN_POINT ( 'NONE',  ( -0.3996062992125987146, 0.1070741851644051862, -1.450131233595800317 ) ) ;
#7533=ORIENTED_EDGE ( 'NONE', *, *, #41165, .F. ) ;
#7534=CARTESIAN_POINT ( 'NONE',  ( 0.3917322834645670659, 2.398668435337828261E-17, -0.1148487121072984812 ) ) ;
#7546=CARTESIAN_POINT ( 'NONE',  ( 0.3392501089628018884, -0.1958661417322834220, -0.09711286089238840846 ) ) ;
#7549=CARTESIAN_POINT ( 'NONE',  ( 0.1974969037888704704, 0.3420746716998660508, -0.7742782152230970327 ) ) ;
#7566=CARTESIAN_POINT ( 'NONE',  ( -0.2925321140481930704, -0.2925321140481933480, -1.476377952755905554 ) ) ;
#7568=CARTESIAN_POINT ( 'NONE',  ( 0.1998031496062992463, 0.3460692066303959202, -0.5360892388451443669 ) ) ;
#7569=CARTESIAN_POINT ( 'NONE',  ( 0.2925321140481932369, 0.2925321140481932369, -0.05708661417322837689 ) ) ;
#7571=CARTESIAN_POINT ( 'NONE',  ( -0.2925321140481932924, 0.2925321140481931814, -2.696850393700787052 ) ) ;
#7572=CARTESIAN_POINT ( 'NONE',  ( 0.1049643490035303689, 0.3917322834645670104, -2.282808398950130879 ) ) ;
#7579=CARTESIAN_POINT ( 'NONE',  ( -0.3458507752293909498, 0.3458507752293907833, -1.671259842519685179 ) ) ;
#7582=CARTESIAN_POINT ( 'NONE',  ( -0.3949938075777411073, 0.1058382717557497660, -1.526902887139107934 ) ) ;
#7592=CARTESIAN_POINT ( 'NONE',  ( -0.3460692066303957537, -0.1998031496062994405, -2.333989501312335957 ) ) ;
#7594=CARTESIAN_POINT ( 'NONE',  ( 0.3392501089628018329, 0.1958661417322835052, -2.258510867945195066 ) ) ;
#7609=CARTESIAN_POINT ( 'NONE',  ( 0.1049643490035303689, 0.3917322834645670104, -1.495406824146981117 ) ) ;
#7626=CARTESIAN_POINT ( 'NONE',  ( 0.3985446848723406266, 0.001150535885505707878, -1.220472440944882386 ) ) ;
#7628=( BOUNDED_CURVE ( )  B_SPLINE_CURVE ( 2, ( #67773, #30271, #30692, #23958, #82054, #50037, #75734, #48804, #43297, #42484, #18074, #10928, #68587 ),
 .UNSPECIFIED., .F., .F. ) 
 B_SPLINE_CURVE_WITH_KNOTS ( ( 3, 2, 2, 2, 2, 2, 3 ),
 ( 0.7374999999999999334, 0.7416666666666665853, 0.7458333333333333481, 0.7500000000000000000, 0.7541666666666666519, 0.7583333333333334147, 0.7625000000000000666 ),
 .UNSPECIFIED. ) 
 CURVE ( )  GEOMETRIC_REPRESENTATION_ITEM ( )  RATIONAL_B_SPLINE_CURVE ( ( 1.000000000000000888, 0.9659258262890674240, 1.000000000000000000, 0.9659258262890683122, 1.000000000000000000, 0.9659258262890683122, 1.000000000000000000, 0.9659258262890683122, 1.000000000000000000, 0.9659258262890683122, 1.000000000000000000, 0.9659258262890674240, 1.000000000000000888 ) ) 
 REPRESENTATION_ITEM ( '' )  );
#7633=CARTESIAN_POINT ( 'NONE',  ( 0.1049643490035304799, -0.3917322834645669549, -2.597112860892388131 ) ) ;
#7636=CARTESIAN_POINT ( 'NONE',  ( -0.4724409448818895907, -0.1265901696524993070, -0.6758530183727035068 ) ) ;
#7637=EDGE_CURVE ( 'NONE', #65743, #23063, #1, .T. ) ;
#7638=CARTESIAN_POINT ( 'NONE',  ( 0.3460692066303959757, -0.1998031496062991907, 0.05249343832020995915 ) ) ;
#7641=CARTESIAN_POINT ( 'NONE',  ( -0.1049643490035302024, -0.3917322834645671215, -1.639107611548556109 ) ) ;
#7652=CARTESIAN_POINT ( 'NONE',  ( 0.1958661417322836162, -0.3392501089628018329, -1.274258899441258031 ) ) ;
#7658=CARTESIAN_POINT ( 'NONE',  ( -0.2867679344610365444, -0.2867679344610367664, -2.417998318406511249 ) ) ;
#7666=CARTESIAN_POINT ( 'NONE',  ( 0.1958661417322834775, 0.3392501089628018884, -1.961286089238845287 ) ) ;
#7682=CARTESIAN_POINT ( 'NONE',  ( -0.4091458600556402980, -0.2362204724409451284, -0.4442257217847768724 ) ) ;
#7685=CARTESIAN_POINT ( 'NONE',  ( -0.1974969037888704149, -0.3420746716998661063, -0.1423884514435695414 ) ) ;
#7691=CARTESIAN_POINT ( 'NONE',  ( 0.2891555358219910499, 0.2891555358219910499, -0.2145669291338582474 ) ) ;
#7698=CARTESIAN_POINT ( 'NONE',  ( -0.1070741851644051862, -0.3996062992125986590, -0.9363517060367454459 ) ) ;
#7700=CARTESIAN_POINT ( 'NONE',  ( 4.797336870675656522E-17, -0.3917322834645670104, -0.8582677165354329896 ) ) ;
#7702=CARTESIAN_POINT ( 'NONE',  ( 0.4724409448818898682, 2.892866454678787531E-17, -0.5098425196850393526 ) ) ;
#7714=CARTESIAN_POINT ( 'NONE',  ( 0.4724409448818897572, -0.1265901696524988906, -2.708005249343832688 ) ) ;
#7732=CARTESIAN_POINT ( 'NONE',  ( 0.1998031496062994405, -0.3460692066303958092, -0.7217847769028871152 ) ) ;
#7738=CARTESIAN_POINT ( 'NONE',  ( 0.1998031496062992740, 0.3460692066303959757, -2.821522309711286258 ) ) ;
#7739=CARTESIAN_POINT ( 'NONE',  ( -0.3420746716998659953, -0.1974969037888706647, -1.942257217847769279 ) ) ;
#7740=CARTESIAN_POINT ( 'NONE',  ( -0.2867679344610365999, 0.2867679344610364889, -0.6417322834645668994 ) ) ;
#7742=CARTESIAN_POINT ( 'NONE',  ( 0.3917322834645669549, 0.06192927228921583233, -1.216469835425646240 ) ) ;
#7744=CARTESIAN_POINT ( 'NONE',  ( -0.3392501089628019995, 0.1958661417322832277, -1.278215223097112885 ) ) ;
#7746=CARTESIAN_POINT ( 'NONE',  ( 4.797336870675655290E-17, -0.3917322834645669549, 0.1561872947844637760 ) ) ;
#7752=CARTESIAN_POINT ( 'NONE',  ( -0.1070741851644051862, -0.3996062992125987146, -2.749343832020996636 ) ) ;
#7753=CARTESIAN_POINT ( 'NONE',  ( 0.2867679344610366554, -0.2867679344610365999, -1.355006192422259170 ) ) ;
#7759=CARTESIAN_POINT ( 'NONE',  ( -0.3917322834645670104, -7.196005306013484475E-17, -0.7539370078740157410 ) ) ;
#7768=CARTESIAN_POINT ( 'NONE',  ( 0.1049643490035304938, -0.3917322834645669549, -2.124671916010498762 ) ) ;
#7770=CARTESIAN_POINT ( 'NONE',  ( 0.1998031496062994405, -0.3460692066303958092, -0.4068241469816273326 ) ) ;
#7776=CARTESIAN_POINT ( 'NONE',  ( -0.3917322834645670104, -7.196005306013484475E-17, -0.9114173228346457156 ) ) ;
#7790=VECTOR ( 'NONE', #9685, 39.37007874015748143 ) ;
#7796=CARTESIAN_POINT ( 'NONE',  ( -0.2867679344610364334, -0.2867679344610368219, -0.9264898705698668691 ) ) ;
#7800=CARTESIAN_POINT ( 'NONE',  ( 0.2867679344610366554, -0.2867679344610365444, -1.127952755905511806 ) ) ;
#7806=CARTESIAN_POINT ( 'NONE',  ( -0.1049643490035302301, -0.3917322834645671770, -0.2263972685377446670 ) ) ;
#7809=CARTESIAN_POINT ( 'NONE',  ( -0.2362204724409451284, 0.4091458600556402425, -1.507217847769029007 ) ) ;
#7818=CARTESIAN_POINT ( 'NONE',  ( 0.4724409448818914781, 0.1265901696524960318, -2.091207349081364519 ) ) ;
#7824=CARTESIAN_POINT ( 'NONE',  ( -0.1974969037888706924, 0.3420746716998658843, 0.2250656167979003253 ) ) ;
#7828=CARTESIAN_POINT ( 'NONE',  ( -0.3460692066303960313, 0.1998031496062989965, -1.992782152230971437 ) ) ;
#7833=CARTESIAN_POINT ( 'NONE',  ( 0.4724409448818898682, 2.892866454678787531E-17, -0.8248031496062991907 ) ) ;
#7834=CARTESIAN_POINT ( 'NONE',  ( -0.3996062992125986035, -0.1070741851644056997, -1.305774278215223072 ) ) ;
#7835=CARTESIAN_POINT ( 'NONE',  ( -0.3949938075777409408, -0.1058382717557502933, -0.5183727034120736432 ) ) ;
#7840=CARTESIAN_POINT ( 'NONE',  ( 0.3420746716998660508, -0.1974969037888704149, -1.756561679790026309 ) ) ;
#7845=CARTESIAN_POINT ( 'NONE',  ( -0.1265901696524993347, 0.4724409448818895907, -2.053805774278214979 ) ) ;
#7847=CARTESIAN_POINT ( 'NONE',  ( 0.3910482532979353554, 0.02544847934400223943, -2.755905511811024500 ) ) ;
#7848=ORIENTED_EDGE ( 'NONE', *, *, #9813, .T. ) ;
#7853=CARTESIAN_POINT ( 'NONE',  ( -0.1049643490035306742, 0.3917322834645668994, -2.291319266895325946 ) ) ;
#7860=CARTESIAN_POINT ( 'NONE',  ( -0.1958661417322834497, -0.3392501089628018884, -2.822815329887452318 ) ) ;
#7863=CARTESIAN_POINT ( 'NONE',  ( -0.1049643490035307020, 0.3917322834645669549, -1.888451443569553412 ) ) ;
#7865=VERTEX_POINT ( 'NONE', #22323 ) ;
#7866=CARTESIAN_POINT ( 'NONE',  ( -0.3420746716998661618, 0.1974969037888702206, -2.073490813648294129 ) ) ;
#7871=CARTESIAN_POINT ( 'NONE',  ( 0.3996062992125986035, 0.1070741851644054776, -0.7545931758530182165 ) ) ;
#7879=CARTESIAN_POINT ( 'NONE',  ( -0.3917322834645669549, -0.1049643490035306603, -0.4455380577427821565 ) ) ;
#7891=CARTESIAN_POINT ( 'NONE',  ( -0.3458507752293906723, -0.3458507752293910609, -1.318897637795275690 ) ) ;
#7894=CARTESIAN_POINT ( 'NONE',  ( 0.1958661417322834775, 0.3392501089628018884, -0.2939632545931757934 ) ) ;
#7895=CARTESIAN_POINT ( 'NONE',  ( 0.3917322834645670104, 2.398668435337828261E-17, -2.250000000000000000 ) ) ;
#7899=CARTESIAN_POINT ( 'NONE',  ( -0.3460692066303960313, 0.1998031496062989965, 0.05446194225721782967 ) ) ;
#7904=CARTESIAN_POINT ( 'NONE',  ( 0.1058382717557500852, -0.3949938075777408852, -2.839238845144357093 ) ) ;
#7911=CARTESIAN_POINT ( 'NONE',  ( -0.3917322834645670104, -7.196005306013484475E-17, -1.921259842519684957 ) ) ;
#7914=CARTESIAN_POINT ( 'NONE',  ( -0.4724409448818899238, 0.1265901696524986686, 0.2053805774278214813 ) ) ;
#7927=CARTESIAN_POINT ( 'NONE',  ( -9.787531504996566615E-17, 0.3996062992125985480, -1.336614173228346303 ) ) ;
#7928=CARTESIAN_POINT ( 'NONE',  ( -0.3917322834645671215, 0.1049643490035301469, -2.794619422572177658 ) ) ;
#7937=CARTESIAN_POINT ( 'NONE',  ( -0.3460692066303958092, -0.1998031496062994683, -0.2099737532808398921 ) ) ;
#7938=CARTESIAN_POINT ( 'NONE',  ( 0.3392501089628018329, 0.1958661417322835607, -2.647657111057429624 ) ) ;
#7945=CARTESIAN_POINT ( 'NONE',  ( 0.3917322834645670104, -0.1049643490035303411, -2.558398950131233196 ) ) ;
#7949=DIRECTION ( 'NONE',  ( 1.000000000000000000, 0.000000000000000000, 0.000000000000000000 ) ) ;
#7952=CARTESIAN_POINT ( 'NONE',  ( 0.3996062992125986590, -0.1070741851644053111, -1.843832020997375309 ) ) ;
#7954=CARTESIAN_POINT ( 'NONE',  ( -0.1049643490035307158, 0.3917322834645670104, -0.003300155676852285953 ) ) ;
#7966=CARTESIAN_POINT ( 'NONE',  ( 0.1049643490035304938, -0.3917322834645669549, -0.5498687664041993495 ) ) ;
#7969=CARTESIAN_POINT ( 'NONE',  ( -0.3420746716998661618, 0.1974969037888702206, -0.8136482939632546652 ) ) ;
#7984=CARTESIAN_POINT ( 'NONE',  ( 0.2925321140481932369, 0.2925321140481932369, -1.082677165354330562 ) ) ;
#7986=CARTESIAN_POINT ( 'NONE',  ( 0.3996062992125986035, -0.1070741851644052972, -0.6607611548556431291 ) ) ;
#7987=CARTESIAN_POINT ( 'NONE',  ( -0.1998031496062991630, -0.3460692066303959202, -0.4573490813648293796 ) ) ;
#7989=CARTESIAN_POINT ( 'NONE',  ( 0.4724409448818896462, 0.1265901696524990294, -0.1246719160104986929 ) ) ;
#7990=CARTESIAN_POINT ( 'NONE',  ( 0.3917322834645669549, 0.1049643490035304660, -1.941601049868766582 ) ) ;
#7996=CARTESIAN_POINT ( 'NONE',  ( -0.4091458600556405756, 0.2362204724409446288, -1.835301837270341352 ) ) ;
#7998=( BOUNDED_CURVE ( )  B_SPLINE_CURVE ( 2, ( #80631, #16651, #60001, #73893, #74304, #67574, #10333, #41880, #35995, #4006, #22942, #48609, #2356, #73480, #35166, #14984, #40643, #66327, #22119, #54924, #3595, #9086, #61665, #72636, #46944, #8665, #67163, #47362, #29260, #60827, #41478, #60418, #34336, #54088, #22535, #67988, #42291, #29670, #16233, #28012, #53672, #78970, #21291, #79380, #54505, #21699, #80219, #73053, #35578, #15403, #41063, #48198, #66752, #34758, #2769, #28428, #79803, #15830, #9906, #28843, #3179, #61241, #82271, #11568, #49025, #23354, #62075, #70032, #30903, #38043, #74721, #68403, #17479, #43110, #5239, #63308, #56570, #75954, #31313, #36400, #4821, #81452, #17885, #24991, #82675, #5646, #55744, #37632, #24589, #37227, #62904, #30082, #81865, #75545, #17070, #68806, #6059, #56978, #69220, #62487, #75134, #23769, #50666, #56162, #50257, #18293, #76366, #18699, #4413, #43938, #44341, #69632, #12385, #11977, #63719, #55332, #81041, #42707, #49440, #49846, #10743, #36811, #11152, #30499, #24177, #43521, #58222, #45170, #46430, #25407, #83085, #51070, #19944, #169, #39713, #45594, #77611, #13225, #70445, #6889, #58648, #14480, #32146, #6476, #72122, #31730, #1015, #33407, #78450, #38457, #7311, #64143, #32980, #57802, #71705, #25822, #51482, #26668, #65819, #77185, #19517, #70876, #32559, #1424, #59069, #52323, #51904, #57394, #78029, #71287, #76769, #19100, #38873, #40134, #20358, #44749, #12802, #64552, #589, #26245, #64974, #13635, #39287, #46009, #20776, #14059, #65404, #7742, #27080 ),
 .UNSPECIFIED., .F., .F. ) 
 B_SPLINE_CURVE_WITH_KNOTS ( ( 3, 2, 2, 2, 2, 2, 2, 2, 2, 2, 2, 2, 2, 2, 2, 2, 2, 2, 2, 2, 2, 2, 2, 2, 2, 2, 2, 2, 2, 2, 2, 2, 2, 2, 2, 2, 2, 2, 2, 2, 2, 2, 2, 2, 2, 2, 2, 2, 2, 2, 2, 2, 2, 2, 2, 2, 2, 2, 2, 2, 2, 2, 2, 2, 2, 2, 2, 2, 2, 2, 2, 2, 2, 2, 2, 2, 2, 2, 2, 2, 2, 2, 2, 2, 2, 2, 2, 2, 2, 2, 2, 2, 2, 2, 3 ),
 ( 0.05249317594045464080, 0.05416666666666666852, 0.05833333333333333426, 0.06250000000000000000, 0.06666666666666666574, 0.07083333333333333148, 0.07499999999999999722, 0.07916666666666666297, 0.08333333333333332871, 0.08749999999999999445, 0.09166666666666666019, 0.09583333333333333981, 0.1000000000000000056, 0.1041666666666666713, 0.1083333333333333370, 0.1125000000000000028, 0.1166666666666666685, 0.1208333333333333204, 0.1250000000000000000, 0.1291666666666666796, 0.1333333333333333315, 0.1375000000000000111, 0.1416666666666666630, 0.1458333333333333426, 0.1500000000000000222, 0.1541666666666666741, 0.1583333333333333259, 0.1625000000000000056, 0.1666666666666666574, 0.1708333333333333370, 0.1749999999999999889, 0.1791666666666666685, 0.1833333333333333204, 0.1875000000000000000, 0.1916666666666666796, 0.1958333333333333315, 0.2000000000000000111, 0.2041666666666666630, 0.2083333333333333426, 0.2124999999999999944, 0.2166666666666666741, 0.2208333333333333259, 0.2250000000000000333, 0.2291666666666666574, 0.2333333333333333370, 0.2374999999999999889, 0.2416666666666666685, 0.2458333333333333204, 0.2499999999999999722, 0.2541666666666666519, 0.2583333333333333592, 0.2625000000000000111, 0.2666666666666666630, 0.2708333333333333148, 0.2750000000000000222, 0.2791666666666666741, 0.2833333333333333259, 0.2874999999999999778, 0.2916666666666666852, 0.2958333333333333370, 0.2999999999999999889, 0.3041666666666666408, 0.3083333333333333481, 0.3125000000000000000, 0.3166666666666666519, 0.3208333333333333592, 0.3250000000000000111, 0.3291666666666666630, 0.3333333333333333148, 0.3375000000000000222, 0.3416666666666666741, 0.3458333333333333259, 0.3499999999999999778, 0.3541666666666666852, 0.3583333333333333370, 0.3624999999999999889, 0.3666666666666666408, 0.3708333333333333481, 0.3750000000000000000, 0.3791666666666666519, 0.3833333333333334147, 0.3875000000000000111, 0.3916666666666666630, 0.3958333333333333148, 0.4000000000000000222, 0.4041666666666666741, 0.4083333333333333814, 0.4124999999999999778, 0.4166666666666666852, 0.4208333333333332815, 0.4249999999999999889, 0.4291666666666666408, 0.4333333333333333481, 0.4375000000000000000, 0.4399931759404547282 ),
 .UNSPECIFIED. ) 
 CURVE ( )  GEOMETRIC_REPRESENTATION_ITEM ( )  RATIONAL_B_SPLINE_CURVE ( ( 0.9836222570911056229, 0.9863145247099402990, 1.000000000000000000, 0.9659258262890683122, 1.000000000000000000, 0.9659258262890683122, 1.000000000000000000, 0.9659258262890683122, 1.000000000000000000, 0.9659258262890683122, 1.000000000000000000, 0.9659258262890683122, 1.000000000000000000, 0.9659258262890683122, 1.000000000000000000, 0.9659258262890683122, 1.000000000000000000, 0.9659258262890683122, 1.000000000000000000, 0.9659258262890683122, 1.000000000000000000, 0.9659258262890683122, 1.000000000000000000, 0.9659258262890683122, 1.000000000000000000, 0.9659258262890683122, 1.000000000000000000, 0.9659258262890683122, 1.000000000000000000, 0.9659258262890683122, 1.000000000000000000, 0.9659258262890683122, 1.000000000000000000, 0.9659258262890683122, 1.000000000000000000, 0.9659258262890683122, 1.000000000000000000, 0.9659258262890683122, 1.000000000000000000, 0.9659258262890683122, 1.000000000000000000, 0.9659258262890683122, 1.000000000000000000, 0.9659258262890683122, 1.000000000000000000, 0.9659258262890683122, 1.000000000000000000, 0.9659258262890683122, 1.000000000000000000, 0.9659258262890683122, 1.000000000000000000, 0.9659258262890683122, 1.000000000000000000, 0.9659258262890683122, 1.000000000000000000, 0.9659258262890683122, 1.000000000000000000, 0.9659258262890683122, 1.000000000000000000, 0.9659258262890683122, 1.000000000000000000, 0.9659258262890683122, 1.000000000000000000, 0.9659258262890683122, 1.000000000000000000, 0.9659258262890683122, 1.000000000000000000, 0.9659258262890683122, 1.000000000000000000, 0.9659258262890683122, 1.000000000000000000, 0.9659258262890683122, 1.000000000000000000, 0.9659258262890683122, 1.000000000000000000, 0.9659258262890683122, 1.000000000000000000, 0.9659258262890683122, 1.000000000000000000, 0.9659258262890683122, 1.000000000000000000, 0.9659258262890683122, 1.000000000000000000, 0.9659258262890683122, 1.000000000000000000, 0.9659258262890683122, 1.000000000000000000, 0.9659258262890683122, 1.000000000000000000, 0.9659258262890683122, 1.000000000000000000, 0.9659258262890683122, 1.000000000000000000, 0.9659258262890683122, 1.000000000000000000, 0.9659258262890683122, 1.000000000000000000, 0.9659258262890683122, 1.000000000000000000, 0.9659258262890683122, 1.000000000000000000, 0.9659258262890683122, 1.000000000000000000, 0.9659258262890683122, 1.000000000000000000, 0.9659258262890683122, 1.000000000000000000, 0.9659258262890683122, 1.000000000000000000, 0.9659258262890683122, 1.000000000000000000, 0.9659258262890683122, 1.000000000000000000, 0.9659258262890683122, 1.000000000000000000, 0.9659258262890683122, 1.000000000000000000, 0.9659258262890683122, 1.000000000000000000, 0.9659258262890683122, 1.000000000000000000, 0.9659258262890683122, 1.000000000000000000, 0.9659258262890683122, 1.000000000000000000, 0.9659258262890683122, 1.000000000000000000, 0.9659258262890683122, 1.000000000000000000, 0.9659258262890683122, 1.000000000000000000, 0.9659258262890683122, 1.000000000000000000, 0.9659258262890683122, 1.000000000000000000, 0.9659258262890683122, 1.000000000000000000, 0.9659258262890683122, 1.000000000000000000, 0.9659258262890683122, 1.000000000000000000, 0.9659258262890683122, 1.000000000000000000, 0.9659258262890683122, 1.000000000000000000, 0.9659258262890683122, 1.000000000000000000, 0.9659258262890683122, 1.000000000000000000, 0.9659258262890683122, 1.000000000000000000, 0.9659258262890683122, 1.000000000000000000, 0.9659258262890683122, 1.000000000000000000, 0.9659258262890683122, 1.000000000000000000, 0.9659258262890683122, 1.000000000000000000, 0.9659258262890683122, 1.000000000000000000, 0.9659258262890683122, 1.000000000000000000, 0.9659258262890683122, 1.000000000000000000, 0.9659258262890683122, 1.000000000000000000, 0.9659258262890683122, 1.000000000000000000, 0.9659258262890683122, 1.000000000000000000, 0.9659258262890683122, 1.000000000000000000, 0.9659258262890683122, 1.000000000000000000, 0.9659258262890683122, 1.000000000000000000, 0.9659258262890683122, 1.000000000000000000, 0.9659258262890683122, 1.000000000000000000, 0.9659258262890683122, 1.000000000000000000, 0.9659258262890683122, 1.000000000000000000, 0.9659258262890683122, 1.000000000000000000, 0.9796113015791271250, 0.9836222570911059560 ) ) 
 REPRESENTATION_ITEM ( '' )  );
#8000=CARTESIAN_POINT ( 'NONE',  ( -0.3420746716998660508, -0.1974969037888706924, -1.546587926509186417 ) ) ;
#8010=CARTESIAN_POINT ( 'NONE',  ( 0.2925321140481932369, -0.2925321140481931814, -2.694881889763780070 ) ) ;
#8011=CARTESIAN_POINT ( 'NONE',  ( 0.3392501089628018329, 0.1958661417322835052, -2.101030552984564981 ) ) ;
#8023=EDGE_CURVE ( 'NONE', #72980, #79206, #5617, .T. ) ;
#8025=CARTESIAN_POINT ( 'NONE',  ( -0.1070741851644051862, -0.3996062992125986590, 0.1660104986876640432 ) ) ;
#8027=CARTESIAN_POINT ( 'NONE',  ( -0.2867679344610364334, -0.2867679344610367109, -1.403543307086614123 ) ) ;
#8050=CARTESIAN_POINT ( 'NONE',  ( 0.3392501089628018329, 0.1958661417322835607, -2.485564304461941987 ) ) ;
#8053=CARTESIAN_POINT ( 'NONE',  ( 4.893765752498283924E-17, -0.3996062992125986035, -0.2362204724409449341 ) ) ;
#8057=CARTESIAN_POINT ( 'NONE',  ( -0.1958661417322834220, -0.3392501089628018884, -1.790026246719160330 ) ) ;
#8058=ORIENTED_EDGE ( 'NONE', *, *, #54557, .F. ) ;
#8068=CARTESIAN_POINT ( 'NONE',  ( 0.2867679344610365999, 0.2867679344610365999, -1.320190657971441528 ) ) ;
#8074=CARTESIAN_POINT ( 'NONE',  ( -0.1958661417322836995, 0.3392501089628017219, -2.372066559876327307 ) ) ;
#8082=CARTESIAN_POINT ( 'NONE',  ( -0.2867679344610365999, 0.2867679344610364889, -1.836614173228346747 ) ) ;
#8095=CARTESIAN_POINT ( 'NONE',  ( 0.4724409448818897572, -0.1265901696524988906, -0.5032808398950130435 ) ) ;
#8098=CARTESIAN_POINT ( 'NONE',  ( -0.1058382717557503072, 0.3949938075777408852, -0.2408136482939632617 ) ) ;
#8103=CARTESIAN_POINT ( 'NONE',  ( -0.1974969037888706924, 0.3420746716998658843, -0.2473753280839895707 ) ) ;
#8110=CARTESIAN_POINT ( 'NONE',  ( 4.893765752498283308E-17, -0.3996062992125985480, -0.9429133858267716439 ) ) ;
#8112=CARTESIAN_POINT ( 'NONE',  ( 0.3392501089628018884, -0.1958661417322834220, -0.7270341207349080292 ) ) ;
#8125=( BOUNDED_CURVE ( )  B_SPLINE_CURVE ( 2, ( #27115, #46466, #71323, #52778, #78487, #25859, #20811, #13672, #6513, #40168, #38910, #72160, #14515 ),
 .UNSPECIFIED., .F., .F. ) 
 B_SPLINE_CURVE_WITH_KNOTS ( ( 3, 2, 2, 2, 2, 2, 3 ),
 ( 0.4125000000000000333, 0.4166666666666667407, 0.4208333333333333925, 0.4250000000000000444, 0.4291666666666666408, 0.4333333333333333481, 0.4375000000000000000 ),
 .UNSPECIFIED. ) 
 CURVE ( )  GEOMETRIC_REPRESENTATION_ITEM ( )  RATIONAL_B_SPLINE_CURVE ( ( 0.9999999999999995559, 0.9659258262890687563, 1.000000000000000000, 0.9659258262890683122, 1.000000000000000000, 0.9659258262890683122, 1.000000000000000000, 0.9659258262890683122, 1.000000000000000000, 0.9659258262890683122, 1.000000000000000000, 0.9659258262890683122, 1.000000000000000000 ) ) 
 REPRESENTATION_ITEM ( '' )  );
#8128=CARTESIAN_POINT ( 'NONE',  ( 0.1070741851644054776, -0.3996062992125984925, 0.1528871391076114805 ) ) ;
#8144=CARTESIAN_POINT ( 'NONE',  ( -0.3996062992125985480, -0.1070741851644057135, -0.6758530183727033958 ) ) ;
#8149=CARTESIAN_POINT ( 'NONE',  ( -0.1070741851644051862, -0.3996062992125987146, -2.434383202099737353 ) ) ;
#8150=CARTESIAN_POINT ( 'NONE',  ( 0.1058382717557500713, -0.3949938075777409408, -1.975065616797900159 ) ) ;
#8151=CARTESIAN_POINT ( 'NONE',  ( 0.3917322834645670104, -0.1049643490035303411, -0.7335958005249343383 ) ) ;
#8154=CARTESIAN_POINT ( 'NONE',  ( -0.1049643490035302024, -0.3917322834645671215, -1.009186351706036433 ) ) ;
#8156=CARTESIAN_POINT ( 'NONE',  ( -0.1958661417322836440, 0.3392501089628016664, 0.2218040926847262562 ) ) ;
#8162=CARTESIAN_POINT ( 'NONE',  ( 0.1070741851644054915, -0.3996062992125986035, -2.447506561679789527 ) ) ;
#8163=CARTESIAN_POINT ( 'NONE',  ( 0.3392501089628018884, -0.1958661417322833942, -1.046607242291025752 ) ) ;
#8168=CARTESIAN_POINT ( 'NONE',  ( 0.1958661417322836440, -0.3392501089628017219, -0.6489501312335959060 ) ) ;
#8176=CARTESIAN_POINT ( 'NONE',  ( 0.3527845929030716809, -0.1716039559343439380, -1.929133858267717549 ) ) ;
#8177=CARTESIAN_POINT ( 'NONE',  ( -0.1049643490035307020, 0.3917322834645669549, -2.045931758530183497 ) ) ;
#8179=CARTESIAN_POINT ( 'NONE',  ( 0.2925321140481932369, 0.2925321140481932369, -0.4527559055118109965 ) ) ;
#8186=CARTESIAN_POINT ( 'NONE',  ( 0.3917322834645669549, 0.1049643490035304660, -1.311679790026246906 ) ) ;
#8208=CARTESIAN_POINT ( 'NONE',  ( 0.3917322834645668994, 0.1049643490035304522, -1.307067298391389354 ) ) ;
#8211=CARTESIAN_POINT ( 'NONE',  ( 4.797336870675656522E-17, -0.3917322834645670104, -1.108267716535433101 ) ) ;
#8218=CARTESIAN_POINT ( 'NONE',  ( 0.2867679344610366554, 0.2867679344610366554, -0.1345337514773772281 ) ) ;
#8220=CARTESIAN_POINT ( 'NONE',  ( 0.4091458600556404646, -0.2362204724409448231, -0.2624671916010498651 ) ) ;
#8221=CARTESIAN_POINT ( 'NONE',  ( -1.157146581871515012E-16, 0.4724409448818898682, -1.809055118110236560 ) ) ;
#8236=CARTESIAN_POINT ( 'NONE',  ( -0.3460692066303957537, -0.1998031496062994405, -2.648950131233595684 ) ) ;
#8241=CARTESIAN_POINT ( 'NONE',  ( -0.1998031496062994405, 0.3460692066303957537, -1.822178477690288956 ) ) ;
#8247=CARTESIAN_POINT ( 'NONE',  ( -0.3983403474834782965, -0.03178304480584832892, -1.220472440944881942 ) ) ;
#8248=CARTESIAN_POINT ( 'NONE',  ( -0.1070741851644056997, 0.3996062992125986035, -1.423884514435695525 ) ) ;
#8249=CARTESIAN_POINT ( 'NONE',  ( -0.1974969037888703871, -0.3420746716998661063, -0.5380577427821522374 ) ) ;
#8255=CARTESIAN_POINT ( 'NONE',  ( -0.2891555358219909388, -0.2891555358219912164, -1.710629921259842590 ) ) ;
#8260=CARTESIAN_POINT ( 'NONE',  ( -0.1265901696524993347, 0.4724409448818895907, -2.211286089238845065 ) ) ;
#8261=CARTESIAN_POINT ( 'NONE',  ( 0.3902087894128212775, 0.03611438844014681904, -2.755905511811024944 ) ) ;
#8267=CARTESIAN_POINT ( 'NONE',  ( 0.3917322834645669549, 2.398668435337827645E-17, -2.402867823325772090 ) ) ;
#8273=CARTESIAN_POINT ( 'NONE',  ( -9.594673741351310580E-17, 0.3917322834645669549, -2.757198531987190115 ) ) ;
#8275=CARTESIAN_POINT ( 'NONE',  ( -0.1049643490035302024, -0.3917322834645671215, -1.954068241469816503 ) ) ;
#8278=CARTESIAN_POINT ( 'NONE',  ( -0.2891555358219911054, 0.2891555358219909388, -2.381889763779527769 ) ) ;
#8283=CARTESIAN_POINT ( 'NONE',  ( 0.3460692066303959757, -0.1998031496062991907, -0.4199475065616797842 ) ) ;
#8288=CARTESIAN_POINT ( 'NONE',  ( 0.3392501089628018329, 0.1958661417322835607, -0.2158792650918636147 ) ) ;
#8290=CARTESIAN_POINT ( 'NONE',  ( 0.1049643490035303689, 0.3917322834645670104, -0.7080052493438320216 ) ) ;
#8301=CARTESIAN_POINT ( 'NONE',  ( 0.3458507752293908943, 0.3458507752293908943, -1.240157480314960647 ) ) ;
#8304=CARTESIAN_POINT ( 'NONE',  ( -0.2867679344610365999, 0.2867679344610364889, -0.4842519685039369248 ) ) ;
#8305=CARTESIAN_POINT ( 'NONE',  ( -0.3917322834645669549, -0.1049643490035306603, -2.492782152230970993 ) ) ;
#8308=CARTESIAN_POINT ( 'NONE',  ( 0.1998031496062992463, 0.3460692066303959202, 0.09383202099737530943 ) ) ;
#8313=CARTESIAN_POINT ( 'NONE',  ( 4.837279021331061486E-17, -0.3949938075777409963, -2.675196850393700920 ) ) ;
#8321=CARTESIAN_POINT ( 'NONE',  ( -0.3392501089628019995, 0.1958661417322832277, -2.065616797900262647 ) ) ;
#8325=CARTESIAN_POINT ( 'NONE',  ( 0.4091458600556403535, 0.2362204724409449896, -0.2080052493438320216 ) ) ;
#8329=CARTESIAN_POINT ( 'NONE',  ( 0.1265901696524989184, 0.4724409448818898127, -0.7001312335958003175 ) ) ;
#8339=CARTESIAN_POINT ( 'NONE',  ( -0.3996062992125985480, -7.340648628747423112E-17, -1.375984251968503713 ) ) ;
#8340=CARTESIAN_POINT ( 'NONE',  ( -0.3392501089628019995, 0.1958661417322832277, -2.788057742782152459 ) ) ;
#8348=CARTESIAN_POINT ( 'NONE',  ( 0.1070741851644054915, -0.3996062992125986035, -0.08530183727034119923 ) ) ;
#8349=CARTESIAN_POINT ( 'NONE',  ( 0.3917322834645670659, 2.398668435337828261E-17, -2.319573121556117279 ) ) ;
#8354=CARTESIAN_POINT ( 'NONE',  ( 0.1049643490035304938, -0.3917322834645669549, -2.374671916010498762 ) ) ;
#8363=CARTESIAN_POINT ( 'NONE',  ( -0.3917322834645670659, -7.196005306013484475E-17, -0.3510691845482433182 ) ) ;
#8377=CARTESIAN_POINT ( 'NONE',  ( -9.594673741351313045E-17, 0.3917322834645670104, -0.7795275590551180578 ) ) ;
#8380=CARTESIAN_POINT ( 'NONE',  ( 0.3420746716998659953, 0.1974969037888705536, -0.9186351706036742781 ) ) ;
#8395=CARTESIAN_POINT ( 'NONE',  ( -0.1998031496062994683, 0.3460692066303958092, -1.272965879265091749 ) ) ;
#8397=CARTESIAN_POINT ( 'NONE',  ( 0.3460692066303959202, -0.1998031496062991630, -0.6541994750656167090 ) ) ;
#8398=CARTESIAN_POINT ( 'NONE',  ( -0.3460692066303960313, 0.1998031496062989965, -0.7329396325459317518 ) ) ;
#8400=CARTESIAN_POINT ( 'NONE',  ( -0.4091458600556402980, -0.2362204724409451284, 0.1049868766404199460 ) ) ;
#8401=CARTESIAN_POINT ( 'NONE',  ( -0.3392501089628019995, 0.1958661417322832277, -2.158136482939632561 ) ) ;
#8407=CARTESIAN_POINT ( 'NONE',  ( 0.1265901696524990294, -0.4724409448818896462, -2.051837270341206665 ) ) ;
#8410=CARTESIAN_POINT ( 'NONE',  ( -0.3949938075777408852, -0.1058382717557502933, -1.225065616797900159 ) ) ;
#8420=CARTESIAN_POINT ( 'NONE',  ( 0.3996062992125985480, 2.446882876249141654E-17, -2.557086614173228689 ) ) ;
#8421=CARTESIAN_POINT ( 'NONE',  ( -0.3392501089628018329, -0.1958661417322836440, -2.022290395504250160 ) ) ;
#8430=CARTESIAN_POINT ( 'NONE',  ( -0.1265901696524986964, -0.4724409448818899238, -0.8595800524934383846 ) ) ;
#8434=CARTESIAN_POINT ( 'NONE',  ( -0.1070741851644056997, 0.3996062992125984925, -0.2408136482939632061 ) ) ;
#8436=CARTESIAN_POINT ( 'NONE',  ( 0.3917322834645670104, -0.1049643490035303411, -1.456036745406824151 ) ) ;
#8445=CARTESIAN_POINT ( 'NONE',  ( 0.2925321140481932369, 0.2925321140481932369, -1.001968503937007871 ) ) ;
#8462=CARTESIAN_POINT ( 'NONE',  ( -0.3460692066303958092, -0.1998031496062994683, -0.3674540682414698112 ) ) ;
#8465=CARTESIAN_POINT ( 'NONE',  ( -0.2867679344610365999, 0.2867679344610364889, -2.059055118110236116 ) ) ;
#8466=ORIENTED_EDGE ( 'NONE', *, *, #18760, .F. ) ;
#8477=CARTESIAN_POINT ( 'NONE',  ( 0.1049643490035303689, 0.3917322834645668994, -1.175833702590864283 ) ) ;
#8483=CARTESIAN_POINT ( 'NONE',  ( -0.3917322834645670659, -7.196005306013484475E-17, -2.555793593997062629 ) ) ;
#8491=( BOUNDED_CURVE ( )  B_SPLINE_CURVE ( 2, ( #58214, #52314, #78021, #72533, #45161, #20769, #13627, #64543, #39279, #27073, #39705, #20349, #580 ),
 .UNSPECIFIED., .F., .F. ) 
 B_SPLINE_CURVE_WITH_KNOTS ( ( 3, 2, 2, 2, 2, 2, 3 ),
 ( 0.4375000000000000000, 0.4416666666666666519, 0.4458333333333334147, 0.4500000000000000666, 0.4541666666666667185, 0.4583333333333334259, 0.4625000000000001332 ),
 .UNSPECIFIED. ) 
 CURVE ( )  GEOMETRIC_REPRESENTATION_ITEM ( )  RATIONAL_B_SPLINE_CURVE ( ( 1.000000000000000000, 0.9659258262890683122, 1.000000000000000000, 0.9659258262890683122, 1.000000000000000000, 0.9659258262890683122, 1.000000000000000000, 0.9659258262890683122, 1.000000000000000000, 0.9659258262890683122, 1.000000000000000000, 0.9659258262890674240, 1.000000000000000888 ) ) 
 REPRESENTATION_ITEM ( '' )  );
#8494=CARTESIAN_POINT ( 'NONE',  ( 0.2867679344610365999, 0.2867679344610365999, -1.639763779527558807 ) ) ;
#8499=CARTESIAN_POINT ( 'NONE',  ( -0.05060072268091472814, 0.3900885325447118746, -8.192289201638894699E-18 ) ) ;
#8504=CARTESIAN_POINT ( 'NONE',  ( 0.2925321140481932369, -0.2925321140481932369, -1.673228346456692828 ) ) ;
#8509=CARTESIAN_POINT ( 'NONE',  ( -0.4091458600556402980, -0.2362204724409451284, -0.7591863517060367661 ) ) ;
#8512=CARTESIAN_POINT ( 'NONE',  ( -9.674558042662122972E-17, 0.3949938075777409963, -0.2342519685039370914 ) ) ;
#8517=CARTESIAN_POINT ( 'NONE',  ( -0.3949938075777411073, 0.1058382717557497660, -0.5820209973753280863 ) ) ;
#8524=CARTESIAN_POINT ( 'NONE',  ( -0.1070741851644051862, -0.3996062992125986590, -1.408792650918635259 ) ) ;
#8526=CARTESIAN_POINT ( 'NONE',  ( -0.3917322834645669549, -0.1049643490035306603, -0.6679790026246719137 ) ) ;
#8540=CARTESIAN_POINT ( 'NONE',  ( -0.3974833285012852047, -0.03087045868620486369, -1.220472440944937453 ) ) ;
#8542=CARTESIAN_POINT ( 'NONE',  ( 0.2362204724409449064, 0.4091458600556404646, -2.740813648293963567 ) ) ;
#8558=CARTESIAN_POINT ( 'NONE',  ( -0.3996062992125986590, 0.1070741851644051862, -0.6627296587926508886 ) ) ;
#8562=CARTESIAN_POINT ( 'NONE',  ( 4.893765752498283924E-17, -0.3996062992125986035, -2.440944881889763884 ) ) ;
#8563=CARTESIAN_POINT ( 'NONE',  ( 0.3949938075777411073, -0.1058382717557499464, -2.473753280839894764 ) ) ;
#8565=CARTESIAN_POINT ( 'NONE',  ( -0.3917322834645669549, -0.1049643490035306603, -0.9829396325459317518 ) ) ;
#8568=CARTESIAN_POINT ( 'NONE',  ( -0.2867679344610365999, 0.2867679344610364889, -0.9566929133858265155 ) ) ;
#8570=CARTESIAN_POINT ( 'NONE',  ( -0.1049643490035301746, -0.3917322834645670659, 0.1627489745744900018 ) ) ;
#8575=CARTESIAN_POINT ( 'NONE',  ( -0.1998031496062991907, -0.3460692066303959757, -2.427821522309711266 ) ) ;
#8576=CARTESIAN_POINT ( 'NONE',  ( -0.3392501089628019995, 0.1958661417322831999, -1.282827714731970215 ) ) ;
#8582=CARTESIAN_POINT ( 'NONE',  ( -0.2867679344610364334, -0.2867679344610367109, -0.4586614173228347746 ) ) ;
#8591=CARTESIAN_POINT ( 'NONE',  ( 0.1188761721695186374, -0.3738583250853876883, -1.929133858267716883 ) ) ;
#8592=CARTESIAN_POINT ( 'NONE',  ( -0.3392501089628019995, 0.1958661417322832277, -1.750656167979002698 ) ) ;
#8594=CARTESIAN_POINT ( 'NONE',  ( -0.1998031496062994683, 0.3460692066303958092, -0.6430446194225721834 ) ) ;
#8601=CARTESIAN_POINT ( 'NONE',  ( 4.797336870675656522E-17, -0.3917322834645670104, -1.265748031496062964 ) ) ;
#8604=CARTESIAN_POINT ( 'NONE',  ( -0.3985446848722469237, -0.001150535885714259370, -1.929133858267716217 ) ) ;
#8612=CARTESIAN_POINT ( 'NONE',  ( 0.1070741851644053527, 0.3996062992125985480, -2.117454068241469756 ) ) ;
#8623=CARTESIAN_POINT ( 'NONE',  ( -0.2867679344610364334, -0.2867679344610368219, -1.083970185530496844 ) ) ;
#8626=CARTESIAN_POINT ( 'NONE',  ( 0.3917322834645670104, 2.398668435337828261E-17, -1.147637795275590733 ) ) ;
#8632=CARTESIAN_POINT ( 'NONE',  ( 0.3917322834645670659, 2.398668435337828261E-17, -0.2723290270679284419 ) ) ;
#8635=CARTESIAN_POINT ( 'NONE',  ( 0.4091458600556403535, 0.2362204724409449896, -1.625328083989501460 ) ) ;
#8651=CARTESIAN_POINT ( 'NONE',  ( 0.2925321140481932369, 0.2925321140481932369, -2.734251968503936148 ) ) ;
#8656=CARTESIAN_POINT ( 'NONE',  ( -0.3460692066303957537, -0.1998031496062994405, -1.704068241469816281 ) ) ;
#8661=CARTESIAN_POINT ( 'NONE',  ( 0.1070741851644054637, -0.3996062992125984925, -0.9494750656167977310 ) ) ;
#8662=CARTESIAN_POINT ( 'NONE',  ( -0.3460692066303958092, -0.1998031496062994683, -1.154855643044619518 ) ) ;
#8664=CARTESIAN_POINT ( 'NONE',  ( 0.3420746716998659953, 0.1974969037888705536, -0.7611548556430446366 ) ) ;
#8665=CARTESIAN_POINT ( 'NONE',  ( -0.1049643490035307020, 0.3917322834645669549, -0.1561679790026246073 ) ) ;
#8669=CARTESIAN_POINT ( 'NONE',  ( -0.1974969037888706924, 0.3420746716998658843, -1.822178477690288512 ) ) ;
#8673=CARTESIAN_POINT ( 'NONE',  ( 0.2362204724409449064, 0.4091458600556404646, -1.876640419947506411 ) ) ;
#8682=CARTESIAN_POINT ( 'NONE',  ( 0.1049643490035304522, -0.3917322834645668994, -2.527539739336271296 ) ) ;
#8685=CARTESIAN_POINT ( 'NONE',  ( -0.4724409448818896462, -0.1265901696524993070, -2.408136482939632561 ) ) ;
#8689=CARTESIAN_POINT ( 'NONE',  ( 4.797336870675655290E-17, -0.3917322834645669549, -2.678458374506874851 ) ) ;
#8691=CARTESIAN_POINT ( 'NONE',  ( 0.3392501089628018884, -0.1958661417322834220, -1.986876640419947604 ) ) ;
#8694=CARTESIAN_POINT ( 'NONE',  ( -0.3949938075777409408, -0.1058382717557502933, -2.093175853018372834 ) ) ;
#8699=CARTESIAN_POINT ( 'NONE',  ( -0.3460692066303960868, 0.1998031496062990242, -0.8136482939632546652 ) ) ;
#8704=CARTESIAN_POINT ( 'NONE',  ( -0.1958661417322834220, -0.3392501089628018884, -0.1502624671916011345 ) ) ;
#8715=CARTESIAN_POINT ( 'NONE',  ( 5.785732909357575061E-17, -0.4724409448818898682, -1.338582677165354173 ) ) ;
#8717=CARTESIAN_POINT ( 'NONE',  ( 0.3392501089628018884, -0.1958661417322834220, -0.5695538057742781657 ) ) ;
#8718=CARTESIAN_POINT ( 'NONE',  ( -0.1049643490035301885, -0.3917322834645671215, -2.519028871391075786 ) ) ;
#8721=CARTESIAN_POINT ( 'NONE',  ( 0.2925321140481932369, -0.2925321140481931814, -0.1751968503937008370 ) ) ;
#8727=CARTESIAN_POINT ( 'NONE',  ( 4.797336870675655290E-17, -0.3917322834645669549, 0.1561872947844637760 ) ) ;
#8729=CARTESIAN_POINT ( 'NONE',  ( 0.1049643490035304799, -0.3917322834645669549, -0.01246719160104995359 ) ) ;
#8734=CARTESIAN_POINT ( 'NONE',  ( -0.2867679344610365999, 0.2867679344610364889, -1.901574803149606252 ) ) ;
#8738=CARTESIAN_POINT ( 'NONE',  ( 0.2362204724409449064, 0.4091458600556404646, -0.3786089238845143923 ) ) ;
#8750=CARTESIAN_POINT ( 'NONE',  ( 0.1998031496062992463, 0.3460692066303959202, -1.638451443569553634 ) ) ;
#8759=CARTESIAN_POINT ( 'NONE',  ( -0.3996062992125987146, 0.1070741851644051862, -0.03280839895013124008 ) ) ;
#8760=CARTESIAN_POINT ( 'NONE',  ( 0.1049643490035304799, -0.3917322834645670104, -2.601725352527246127 ) ) ;
#8765=CARTESIAN_POINT ( 'NONE',  ( 0.3392501089628018329, 0.1958661417322835607, -2.263123359580052618 ) ) ;
#8775=CARTESIAN_POINT ( 'NONE',  ( -0.3917322834645670104, -0.1049643490035307020, -0.5151111792988996019 ) ) ;
#8788=CARTESIAN_POINT ( 'NONE',  ( -0.1958661417322836718, 0.3392501089628017219, -0.4776902887139107268 ) ) ;
#8791=CARTESIAN_POINT ( 'NONE',  ( 0.1974969037888706369, -0.3420746716998659953, -0.8792650918635170898 ) ) ;
#8807=CARTESIAN_POINT ( 'NONE',  ( -0.1998031496062994683, 0.3460692066303958092, -1.902887139107611647 ) ) ;
#8809=CARTESIAN_POINT ( 'NONE',  ( -0.2925321140481932369, 0.2925321140481931259, -1.198818897637795367 ) ) ;
#8810=CARTESIAN_POINT ( 'NONE',  ( 0.2925321140481932369, -0.2925321140481931814, -0.3326771653543306728 ) ) ;
#8812=CARTESIAN_POINT ( 'NONE',  ( -0.3458507752293909498, 0.3458507752293907833, -0.1771653543307086520 ) ) ;
#8813=CARTESIAN_POINT ( 'NONE',  ( -0.2867679344610365999, 0.2867679344610364889, -2.151574803149605586 ) ) ;
#8819=CARTESIAN_POINT ( 'NONE',  ( -0.2362204724409451284, 0.4091458600556402425, -1.979658792650918597 ) ) ;
#8822=CARTESIAN_POINT ( 'NONE',  ( -0.3949938075777408852, -0.1058382717557502933, -2.012467191601050143 ) ) ;
#8832=CARTESIAN_POINT ( 'NONE',  ( -0.3996062992125985480, -7.340648628747423112E-17, -2.635826771653543066 ) ) ;
#8833=CARTESIAN_POINT ( 'NONE',  ( 0.1958661417322836162, -0.3392501089628018329, -2.219140789205037656 ) ) ;
#8846=CARTESIAN_POINT ( 'NONE',  ( 4.893765752498283308E-17, -0.3996062992125985480, -0.1555118110236220763 ) ) ;
#8848=CARTESIAN_POINT ( 'NONE',  ( -0.2867679344610365999, 0.2867679344610364889, -1.994094488188976610 ) ) ;
#8857=CARTESIAN_POINT ( 'NONE',  ( 4.893765752498283308E-17, -0.3996062992125985480, -1.100393700787401619 ) ) ;
#8874=CARTESIAN_POINT ( 'NONE',  ( 0.1070741851644053527, 0.3996062992125986590, -0.6233595800524933672 ) ) ;
#8877=CARTESIAN_POINT ( 'NONE',  ( -9.594673741351313045E-17, 0.3917322834645670104, -2.039370078740157410 ) ) ;
#8888=CARTESIAN_POINT ( 'NONE',  ( -0.2867679344610364334, -0.2867679344610368219, -1.713891445373016520 ) ) ;
#8894=CARTESIAN_POINT ( 'NONE',  ( 0.3420746716998660508, -0.1974969037888703871, 0.05249343832020991057 ) ) ;
#8904=CARTESIAN_POINT ( 'NONE',  ( -0.2867679344610365999, 0.2867679344610364889, -2.309055118110235671 ) ) ;
#8912=CARTESIAN_POINT ( 'NONE',  ( -0.2925321140481932369, 0.2925321140481931259, 0.06102362204724409017 ) ) ;
#8914=CARTESIAN_POINT ( 'NONE',  ( -0.3996062992125986035, -0.1070741851644056997, -1.778215223097112663 ) ) ;
#8921=CARTESIAN_POINT ( 'NONE',  ( 0.4091458600556403535, 0.2362204724409449896, -0.8379265091863516979 ) ) ;
#8924=CARTESIAN_POINT ( 'NONE',  ( -0.1974969037888704149, -0.3420746716998661063, -0.2998687664041995715 ) ) ;
#8929=CARTESIAN_POINT ( 'NONE',  ( -0.2891555358219909388, -0.2891555358219912164, -0.2933070866141732624 ) ) ;
#8935=CARTESIAN_POINT ( 'NONE',  ( -0.3996062992125986590, 0.1070741851644051723, -1.526902887139107490 ) ) ;
#8938=CARTESIAN_POINT ( 'NONE',  ( -0.1049643490035302024, -0.3917322834645671215, -1.009186351706036433 ) ) ;
#8941=CARTESIAN_POINT ( 'NONE',  ( 5.785732909357575061E-17, -0.4724409448818898682, -0.4704724409448819422 ) ) ;
#8953=CARTESIAN_POINT ( 'NONE',  ( -0.3996062992125986590, 0.1070741851644051723, 0.2053805774278214813 ) ) ;
#8961=CARTESIAN_POINT ( 'NONE',  ( -0.2362204724409451284, 0.4091458600556402425, -2.060367454068241511 ) ) ;
#8971=CARTESIAN_POINT ( 'NONE',  ( -0.1070741851644051862, -0.3996062992125986590, -0.8595800524934383846 ) ) ;
#8977=CARTESIAN_POINT ( 'NONE',  ( -0.1070741851644051862, -0.3996062992125987146, -2.906824146981627610 ) ) ;
#8978=CARTESIAN_POINT ( 'NONE',  ( 0.2891555358219910499, 0.2891555358219910499, -2.342519685039370358 ) ) ;
#8981=CARTESIAN_POINT ( 'NONE',  ( 0.1958661417322836440, -0.3392501089628017219, -1.028871391076115360 ) ) ;
#8987=CARTESIAN_POINT ( 'NONE',  ( 0.2867679344610365999, -0.2867679344610365999, -0.4934190044281346332 ) ) ;
#8996=CARTESIAN_POINT ( 'NONE',  ( 0.2867679344610366554, -0.2867679344610365999, -1.669966822343518897 ) ) ;
#9003=CARTESIAN_POINT ( 'NONE',  ( 0.1049643490035303689, 0.3917322834645670104, -0.7080052493438320216 ) ) ;
#9012=CARTESIAN_POINT ( 'NONE',  ( -0.3392501089628017219, -0.1958661417322836718, -2.406824146981627166 ) ) ;
#9019=CARTESIAN_POINT ( 'NONE',  ( 0.3977953519386753789, 0.03143970413924940949, -1.929133858267772839 ) ) ;
#9020=CARTESIAN_POINT ( 'NONE',  ( 0.3392501089628018884, -0.1958661417322834220, -1.449475065616798064 ) ) ;
#9021=CARTESIAN_POINT ( 'NONE',  ( 0.1998031496062994128, -0.3460692066303957537, -2.058398950131233640 ) ) ;
#9030=CARTESIAN_POINT ( 'NONE',  ( 0.1070741851644053527, 0.3996062992125985480, -1.959973753280839892 ) ) ;
#9032=CARTESIAN_POINT ( 'NONE',  ( 0.2017716535433070613, -0.2017716535433070890, 0.000000000000000000 ) ) ;
#9039=CARTESIAN_POINT ( 'NONE',  ( -0.3917322834645668994, -0.1049643490035306742, -1.385807455871704175 ) ) ;
#9048=CARTESIAN_POINT ( 'NONE',  ( 0.1049643490035304799, -0.3917322834645670104, 0.07544000180346267792 ) ) ;
#9054=CARTESIAN_POINT ( 'NONE',  ( -0.1265901696524986964, -0.4724409448818899238, -1.723753280839894986 ) ) ;
#9072=CARTESIAN_POINT ( 'NONE',  ( -0.3996062992125985480, -7.340648628747423112E-17, -2.793307086614173151 ) ) ;
#9077=CARTESIAN_POINT ( 'NONE',  ( -0.1998031496062991630, -0.3460692066303959202, -2.189632545931758489 ) ) ;
#9083=CARTESIAN_POINT ( 'NONE',  ( -0.3996062992125987146, 0.1070741851644051862, -1.292650918635170454 ) ) ;
#9084=CARTESIAN_POINT ( 'NONE',  ( -0.2891555358219908833, -0.2891555358219912164, -1.161417322834645827 ) ) ;
#9085=CARTESIAN_POINT ( 'NONE',  ( 0.3996062992125986035, 0.1070741851644054776, -2.329396325459317296 ) ) ;
#9086=CARTESIAN_POINT ( 'NONE',  ( 0.2867679344610366554, 0.2867679344610366554, -0.1299212598425196485 ) ) ;
#9090=CARTESIAN_POINT ( 'NONE',  ( -0.3420746716998660508, -0.1974969037888706924, -1.704068241469815836 ) ) ;
#9094=CARTESIAN_POINT ( 'NONE',  ( 0.2362204724409451007, -0.4091458600556402980, -1.824146981627296604 ) ) ;
#9095=CARTESIAN_POINT ( 'NONE',  ( 0.3285422586334079686, 0.2143816077119419516, -2.755905511811022723 ) ) ;
#9097=ORIENTED_EDGE ( 'NONE', *, *, #13640, .T. ) ;
#9102=CARTESIAN_POINT ( 'NONE',  ( -0.2867679344610364334, -0.2867679344610368219, -2.501293020176166504 ) ) ;
#9109=CARTESIAN_POINT ( 'NONE',  ( 0.3917322834645669549, 0.1049643490035304660, 0.1056430446194224632 ) ) ;
#9111=( BOUNDED_CURVE ( )  B_SPLINE_CURVE ( 2, ( #66054, #7130, #21016, #34056, #59720, #52980, #65651 ),
 .UNSPECIFIED., .F., .F. ) 
 B_SPLINE_CURVE_WITH_KNOTS ( ( 3, 2, 2, 3 ),
 ( 0.9125000000000000888, 0.9166666666666667407, 0.9208333333333332815, 0.9250000000000000444 ),
 .UNSPECIFIED. ) 
 CURVE ( )  GEOMETRIC_REPRESENTATION_ITEM ( )  RATIONAL_B_SPLINE_CURVE ( ( 0.9999999999999991118, 0.9659258262890692004, 1.000000000000000000, 0.9659258262890683122, 1.000000000000000000, 0.9659258262890683122, 1.000000000000000000 ) ) 
 REPRESENTATION_ITEM ( '' )  );
#9112=CARTESIAN_POINT ( 'NONE',  ( 0.2867679344610365999, -0.2867679344610365444, -1.665354330708661124 ) ) ;
#9115=CARTESIAN_POINT ( 'NONE',  ( 0.1974969037888706369, -0.3420746716998659953, -2.296587926509186417 ) ) ;
#9121=CARTESIAN_POINT ( 'NONE',  ( 0.3996062992125986035, 0.1070741851644054776, -0.4396325459317584339 ) ) ;
#9126=CARTESIAN_POINT ( 'NONE',  ( -0.1049643490035302024, -0.3917322834645671215, 0.0006561679790025351077 ) ) ;
#9132=CARTESIAN_POINT ( 'NONE',  ( -0.3392501089628017219, -0.1958661417322836718, -0.04461942257217842850 ) ) ;
#9136=CARTESIAN_POINT ( 'NONE',  ( 0.000000000000000000, 0.000000000000000000, 0.000000000000000000 ) ) ;
#9137=CARTESIAN_POINT ( 'NONE',  ( -0.4091458600556402980, -0.2362204724409451284, -1.312335958005249381 ) ) ;
#9139=CARTESIAN_POINT ( 'NONE',  ( 0.1958661417322836440, -0.3392501089628017219, -0.7139107611548556331 ) ) ;
#9140=CARTESIAN_POINT ( 'NONE',  ( 0.1958661417322836440, -0.3392501089628017219, -2.223753280839895208 ) ) ;
#9143=CARTESIAN_POINT ( 'NONE',  ( -0.3996062992125986590, 0.1070741851644051723, 0.04790026246719156916 ) ) ;
#9148=CARTESIAN_POINT ( 'NONE',  ( -0.2867679344610366554, 0.2867679344610365444, -0.09971821702655986330 ) ) ;
#9150=CARTESIAN_POINT ( 'NONE',  ( -0.1049643490035301885, -0.3917322834645671215, -0.6292650918635172008 ) ) ;
#9155=CARTESIAN_POINT ( 'NONE',  ( 0.2867679344610365999, -0.2867679344610365444, -1.822834645669291653 ) ) ;
#9158=CARTESIAN_POINT ( 'NONE',  ( 0.3458507752293908943, 0.3458507752293908943, -0.5295275590551181688 ) ) ;
#9167=CARTESIAN_POINT ( 'NONE',  ( 0.2362204724409449064, 0.4091458600556404646, -1.953412073490813805 ) ) ;
#9170=CARTESIAN_POINT ( 'NONE',  ( 0.1998031496062994128, -0.3460692066303957537, -1.428477690288713964 ) ) ;
#9179=CARTESIAN_POINT ( 'NONE',  ( -0.3996062992125987146, 0.1070741851644051862, -0.1902887139107611314 ) ) ;
#9180=CARTESIAN_POINT ( 'NONE',  ( 0.3392501089628018884, -0.1958661417322833942, -2.936371021818584115 ) ) ;
#9185=CARTESIAN_POINT ( 'NONE',  ( 0.2867679344610365999, -0.2867679344610365444, -2.230314960629921295 ) ) ;
#9190=CARTESIAN_POINT ( 'NONE',  ( -0.4724409448818898682, -8.678599364036362592E-17, -0.6692913385826770867 ) ) ;
#9194=CARTESIAN_POINT ( 'NONE',  ( 0.2867679344610366554, -0.2867679344610365999, -0.4101243026584795448 ) ) ;
#9207=CARTESIAN_POINT ( 'NONE',  ( -0.3392501089628017219, -0.1958661417322836718, -0.6745406824146981117 ) ) ;
#9210=CARTESIAN_POINT ( 'NONE',  ( 0.1058382717557499880, 0.3949938075777411073, -0.9383202099737534274 ) ) ;
#9220=CARTESIAN_POINT ( 'NONE',  ( -1.157146581871515012E-16, 0.4724409448818898682, -0.3917322834645669549 ) ) ;
#9226=CARTESIAN_POINT ( 'NONE',  ( 0.3996062992125986035, 0.1070741851644054776, -1.699475065616798064 ) ) ;
#9229=CARTESIAN_POINT ( 'NONE',  ( -0.3460692066303957537, -0.1998031496062994405, -1.231627296587926468 ) ) ;
#9230=CARTESIAN_POINT ( 'NONE',  ( 0.3996062992125986035, -0.1070741851644052972, -0.6607611548556431291 ) ) ;
#9232=CARTESIAN_POINT ( 'NONE',  ( 0.4724409448818897572, -0.1265901696524988906, -0.1115485564304461719 ) ) ;
#9234=CARTESIAN_POINT ( 'NONE',  ( -0.3917322834645671215, 0.1049643490035301469, -2.637139107611548461 ) ) ;
#9240=CARTESIAN_POINT ( 'NONE',  ( 0.4724409448818896462, 0.1265901696524990294, -2.091207349081364519 ) ) ;
#9243=CARTESIAN_POINT ( 'NONE',  ( 0.3949938075777408852, 0.1058382717557500435, -1.776246719160105236 ) ) ;
#9250=CARTESIAN_POINT ( 'NONE',  ( -0.2362204724409451284, 0.4091458600556402425, -2.294619422572178102 ) ) ;
#9253=CARTESIAN_POINT ( 'NONE',  ( -0.3996062992125985480, -7.340648628747423112E-17, -2.478346456692913868 ) ) ;
#9255=CARTESIAN_POINT ( 'NONE',  ( 0.3392501089628018329, 0.1958661417322835052, -2.415991182905824708 ) ) ;
#9268=CARTESIAN_POINT ( 'NONE',  ( -0.3996062992125985480, -7.340648628747423112E-17, -0.2736220472440945017 ) ) ;
#9270=CARTESIAN_POINT ( 'NONE',  ( -0.2867679344610364334, -0.2867679344610367109, -1.718503937007874072 ) ) ;
#9279=CARTESIAN_POINT ( 'NONE',  ( 0.3996062992125986035, -0.1070741851644052972, -0.9757217847769029673 ) ) ;
#9285=CARTESIAN_POINT ( 'NONE',  ( 0.3964540044758441684, 0.009627693921947956882, -1.220472440942466541 ) ) ;
#9294=CARTESIAN_POINT ( 'NONE',  ( 0.1998031496062992740, 0.3460692066303959757, -0.3018372703412073865 ) ) ;
#9297=CARTESIAN_POINT ( 'NONE',  ( -0.3392501089628017219, -0.1958661417322836718, -2.406824146981627166 ) ) ;
#9307=CARTESIAN_POINT ( 'NONE',  ( 0.1049643490035304522, -0.3917322834645668994, -1.425177534611861585 ) ) ;
#9313=CARTESIAN_POINT ( 'NONE',  ( 0.3949938075777409963, 2.418639510665530435E-17, 0.03937007874015741732 ) ) ;
#9315=ORIENTED_EDGE ( 'NONE', *, *, #25445, .T. ) ;
#9322=CARTESIAN_POINT ( 'NONE',  ( -0.3917322834645671215, 0.1049643490035301469, -2.322178477690288734 ) ) ;
#9329=CARTESIAN_POINT ( 'NONE',  ( -0.1998031496062994405, 0.3460692066303957537, -0.08989501312335958227 ) ) ;
#9331=CARTESIAN_POINT ( 'NONE',  ( 0.3996062992125986035, 0.1070741851644054776, -1.699475065616798064 ) ) ;
#9336=CARTESIAN_POINT ( 'NONE',  ( -1.157146581871515012E-16, 0.4724409448818898682, -0.7066929133858268486 ) ) ;
#9338=VECTOR ( 'NONE', #52257, 39.37007874015748143 ) ;
#9340=CARTESIAN_POINT ( 'NONE',  ( -0.1974969037888704149, -0.3420746716998661063, -0.6148293963254595207 ) ) ;
#9345=CARTESIAN_POINT ( 'NONE',  ( 0.3949938075777408852, 0.1058382717557500435, -0.3589238845144356871 ) ) ;
#9352=CARTESIAN_POINT ( 'NONE',  ( 0.3460692066303959202, -0.1998031496062991630, -1.126640419947506633 ) ) ;
#9354=CARTESIAN_POINT ( 'NONE',  ( -0.1958661417322836718, 0.3392501089628017219, -1.107611548556430403 ) ) ;
#9382=CARTESIAN_POINT ( 'NONE',  ( -9.787531504996567848E-17, 0.3996062992125986035, -0.7874015748031496509 ) ) ;
#9386=CARTESIAN_POINT ( 'NONE',  ( -0.1998031496062991907, -0.3460692066303959757, -2.900262467191600635 ) ) ;
#9387=CARTESIAN_POINT ( 'NONE',  ( 0.3949938075777409963, 2.418639510665530435E-17, -2.480314960629921295 ) ) ;
#9390=CARTESIAN_POINT ( 'NONE',  ( -0.3392501089628017219, -0.1958661417322836718, -1.146981627296587813 ) ) ;
#9396=CARTESIAN_POINT ( 'NONE',  ( -0.3917322834645670659, 0.1049643490035301607, -0.1128415766066123566 ) ) ;
#9403=CARTESIAN_POINT ( 'NONE',  ( -1.157146581871515012E-16, 0.4724409448818898682, -1.102362204724409489 ) ) ;
#9404=CARTESIAN_POINT ( 'NONE',  ( 0.1958661417322836718, -0.3392501089628017219, -1.505924827592862503 ) ) ;
#9410=CARTESIAN_POINT ( 'NONE',  ( 4.797336870675656522E-17, -0.3917322834645670104, -1.108267716535433101 ) ) ;
#9420=CARTESIAN_POINT ( 'NONE',  ( -0.3392501089628019995, 0.1958661417322832277, -2.380577427821522374 ) ) ;
#9429=CARTESIAN_POINT ( 'NONE',  ( -0.1958661417322836718, 0.3392501089628017219, -1.357611548556430625 ) ) ;
#9430=CARTESIAN_POINT ( 'NONE',  ( 0.2925321140481932369, 0.2925321140481932369, -2.419291338582676865 ) ) ;
#9438=CARTESIAN_POINT ( 'NONE',  ( -0.3460692066303960313, 0.1998031496062989965, -2.150262467191601079 ) ) ;
#9447=CARTESIAN_POINT ( 'NONE',  ( -0.1958661417322836440, 0.3392501089628016664, -1.038038427000312902 ) ) ;
#9456=CARTESIAN_POINT ( 'NONE',  ( -0.3917322834645670104, -0.1049643490035307020, -0.3576308643382697383 ) ) ;
#9459=CARTESIAN_POINT ( 'NONE',  ( 5.785732909357575061E-17, -0.4724409448818898682, -1.730314960629921517 ) ) ;
#9477=CARTESIAN_POINT ( 'NONE',  ( -0.3460692066303960313, 0.1998031496062989965, -2.622703412073490892 ) ) ;
#9482=CARTESIAN_POINT ( 'NONE',  ( -0.1998031496062991630, -0.3460692066303959202, -2.032152230971128848 ) ) ;
#9488=CARTESIAN_POINT ( 'NONE',  ( 0.3996062992125986590, -0.1070741851644053111, -1.686351706036745446 ) ) ;
#9489=CARTESIAN_POINT ( 'NONE',  ( 0.2891555358219910499, 0.2891555358219910499, -1.240157480314960869 ) ) ;
#9490=CARTESIAN_POINT ( 'NONE',  ( 0.2925321140481932369, -0.2925321140481932369, -2.460629921259842146 ) ) ;
#9497=CARTESIAN_POINT ( 'NONE',  ( -9.674558042662122972E-17, 0.3949938075777409963, -1.966535433070866423 ) ) ;
#9501=CARTESIAN_POINT ( 'NONE',  ( 0.2362204724409451007, -0.4091458600556402980, -2.296587926509186417 ) ) ;
#9502=CARTESIAN_POINT ( 'NONE',  ( 0.1070741851644054915, -0.3996062992125986035, -1.660104986876640210 ) ) ;
#9510=CARTESIAN_POINT ( 'NONE',  ( 0.1049643490035304938, -0.3917322834645669549, 0.1450131233595799429 ) ) ;
#9518=CARTESIAN_POINT ( 'NONE',  ( 0.3917322834645670104, -0.1049643490035303411, -0.3536745406824148286 ) ) ;
#9520=CARTESIAN_POINT ( 'NONE',  ( 0.1958661417322836440, -0.3392501089628017219, -2.131233595800524849 ) ) ;
#9523=CARTESIAN_POINT ( 'NONE',  ( -0.1058382717557497937, -0.3949938075777411628, -2.434383202099737353 ) ) ;
#9527=CARTESIAN_POINT ( 'NONE',  ( -0.2925321140481930704, -0.2925321140481933480, -1.003937007874015741 ) ) ;
#9533=CARTESIAN_POINT ( 'NONE',  ( 0.2867679344610365999, 0.2867679344610365999, -0.06496062992125994917 ) ) ;
#9541=FACE_OUTER_BOUND ( 'NONE', #735, .T. ) ;
#9545=CARTESIAN_POINT ( 'NONE',  ( 0.2362204724409449064, 0.4091458600556404646, -1.561679790026246684 ) ) ;
#9547=CARTESIAN_POINT ( 'NONE',  ( -0.1049643490035307020, 0.3917322834645669549, -0.6286089238845143923 ) ) ;
#9548=CARTESIAN_POINT ( 'NONE',  ( 0.3917322834645669549, 0.1049643490035304660, -2.414041994750655729 ) ) ;
#9551=CARTESIAN_POINT ( 'NONE',  ( -0.2925321140481932369, 0.2925321140481931259, -0.4114173228346455491 ) ) ;
#9556=CARTESIAN_POINT ( 'NONE',  ( 0.2867679344610365999, -0.2867679344610365999, -0.1784583745068747673 ) ) ;
#9558=CARTESIAN_POINT ( 'NONE',  ( 0.3392501089628018329, 0.1958661417322835607, -0.3733595800524935338 ) ) ;
#9563=CARTESIAN_POINT ( 'NONE',  ( 0.3392501089628018329, 0.1958661417322835607, -2.170603674540682260 ) ) ;
#9567=CARTESIAN_POINT ( 'NONE',  ( 0.2362204724409449064, 0.4091458600556404646, -0.2211286089238845010 ) ) ;
#9578=CARTESIAN_POINT ( 'NONE',  ( 0.1998031496062994128, -0.3460692066303957537, -1.743438320209973469 ) ) ;
#9588=CARTESIAN_POINT ( 'NONE',  ( -0.3460692066303960313, 0.1998031496062989965, -0.2604986876640419946 ) ) ;
#9589=CARTESIAN_POINT ( 'NONE',  ( -0.3460692066303958092, -0.1998031496062994683, -0.5249343832020997302 ) ) ;
#9590=CARTESIAN_POINT ( 'NONE',  ( 0.3917322834645670104, 0.1049643490035304660, -2.798575746228034067 ) ) ;
#9596=CARTESIAN_POINT ( 'NONE',  ( -0.3949938075777408852, -0.1058382717557502933, -0.9101049868766403206 ) ) ;
#9601=CARTESIAN_POINT ( 'NONE',  ( 0.4724409448818898682, 2.892866454678787531E-17, -0.5905511811023621549 ) ) ;
#9602=CARTESIAN_POINT ( 'NONE',  ( -9.787531504996567848E-17, 0.3996062992125986035, -2.204724409448818978 ) ) ;
#9605=CARTESIAN_POINT ( 'NONE',  ( -0.1958661417322836995, 0.3392501089628017219, -0.4823027803487682785 ) ) ;
#9617=CARTESIAN_POINT ( 'NONE',  ( 0.3392501089628018329, 0.1958661417322835607, -0.5958005249343831800 ) ) ;
#9620=CARTESIAN_POINT ( 'NONE',  ( 0.1974969037888704704, 0.3420746716998660508, -0.9317585301837268963 ) ) ;
#9621=ORIENTED_EDGE ( 'NONE', *, *, #27502, .F. ) ;
#9624=CARTESIAN_POINT ( 'NONE',  ( -0.3996062992125987146, 0.1070741851644051862, 0.1246719160104986790 ) ) ;
#9632=CARTESIAN_POINT ( 'NONE',  ( 0.4724409448818898682, 2.892866454678787531E-17, -0.6673228346456693272 ) ) ;
#9638=CARTESIAN_POINT ( 'NONE',  ( -0.3996062992125986035, -0.1070741851644056997, -1.778215223097112663 ) ) ;
#9641=CARTESIAN_POINT ( 'NONE',  ( -9.787531504996566615E-17, 0.3996062992125985480, -1.179133858267716661 ) ) ;
#9642=CARTESIAN_POINT ( 'NONE',  ( 0.1998031496062992463, 0.3460692066303959202, -0.6935695538057742304 ) ) ;
#9645=CARTESIAN_POINT ( 'NONE',  ( -1.157146581871515012E-16, 0.4724409448818898682, 0.000000000000000000 ) ) ;
#9646=CARTESIAN_POINT ( 'NONE',  ( -0.2867679344610365999, 0.2867679344610364889, -2.466535433070865757 ) ) ;
#9652=CARTESIAN_POINT ( 'NONE',  ( 0.4724409448818897572, -0.1265901696524988906, -2.078083989501312345 ) ) ;
#9655=CARTESIAN_POINT ( 'NONE',  ( 0.3420746716998660508, -0.1974969037888704149, -1.914041994750656395 ) ) ;
#9664=CARTESIAN_POINT ( 'NONE',  ( 0.1998031496062994128, -0.3460692066303957537, -2.688320209973753538 ) ) ;
#9666=CARTESIAN_POINT ( 'NONE',  ( -0.3392501089628019439, 0.1958661417322832554, -2.311004306265404651 ) ) ;
#9678=CARTESIAN_POINT ( 'NONE',  ( -0.1998031496062991630, -0.3460692066303959202, -0.1423884514435695414 ) ) ;
#9680=CARTESIAN_POINT ( 'NONE',  ( -0.3917322834645671215, 0.1049643490035301469, -1.849737532808399143 ) ) ;
#9685=DIRECTION ( 'NONE',  ( 0.000000000000000000, 0.000000000000000000, 1.000000000000000000 ) ) ;
#9689=CARTESIAN_POINT ( 'NONE',  ( 0.1070741851644053388, 0.3996062992125986035, -1.015091863517060267 ) ) ;
#9698=CARTESIAN_POINT ( 'NONE',  ( 0.3392501089628018329, 0.1958661417322835607, -1.633202099737532942 ) ) ;
#9705=CARTESIAN_POINT ( 'NONE',  ( -0.3996062992125987146, 0.1070741851644051862, -0.5052493438320209140 ) ) ;
#9708=CARTESIAN_POINT ( 'NONE',  ( -0.3392501089628019995, 0.1958661417322832277, -2.065616797900262647 ) ) ;
#9718=CARTESIAN_POINT ( 'NONE',  ( 0.1049643490035303689, 0.3917322834645668994, -1.490794332512124010 ) ) ;
#9724=CARTESIAN_POINT ( 'NONE',  ( -0.1049643490035302301, -0.3917322834645671770, -2.903562622868453680 ) ) ;
#9733=CARTESIAN_POINT ( 'NONE',  ( 0.2867679344610366554, 0.2867679344610366554, -1.394376271162416359 ) ) ;
#9735=CARTESIAN_POINT ( 'NONE',  ( 0.3917322834645669549, 0.1049643490035304660, -2.256561679790026531 ) ) ;
#9741=CARTESIAN_POINT ( 'NONE',  ( 0.2925321140481932369, 0.2925321140481932369, 0.1003937007874015769 ) ) ;
#9743=CARTESIAN_POINT ( 'NONE',  ( 0.3460692066303959757, -0.1998031496062991907, -1.837270341207349000 ) ) ;
#9747=CARTESIAN_POINT ( 'NONE',  ( 0.2362204724409451007, -0.4091458600556402980, -0.6410761154855643129 ) ) ;
#9750=CARTESIAN_POINT ( 'NONE',  ( -0.1974969037888706924, 0.3420746716998658843, -0.5623359580052492701 ) ) ;
#9755=CARTESIAN_POINT ( 'NONE',  ( 0.1974969037888706092, -0.3420746716998660508, -0.4835958005249345049 ) ) ;
#9760=CARTESIAN_POINT ( 'NONE',  ( 0.4724409448818898682, 2.892866454678787531E-17, -0.1948818897637795422 ) ) ;
#9763=CARTESIAN_POINT ( 'NONE',  ( 0.3996062992125985480, 2.446882876249141654E-17, -1.139763779527559029 ) ) ;
#9765=CARTESIAN_POINT ( 'NONE',  ( -0.3392501089628019995, 0.1958661417322832277, -1.120734908136482799 ) ) ;
#9767=CARTESIAN_POINT ( 'NONE',  ( -0.3285422586334152406, -0.2143816077119310159, -5.947530023412593222E-17 ) ) ;
#9780=DIRECTION ( 'NONE',  ( 0.000000000000000000, 0.000000000000000000, 1.000000000000000000 ) ) ;
#9794=DIRECTION ( 'NONE',  ( 0.000000000000000000, 0.000000000000000000, 1.000000000000000000 ) ) ;
#9797=CARTESIAN_POINT ( 'NONE',  ( 0.1998031496062994405, -0.3460692066303958092, -2.926509186351706315 ) ) ;
#9798=CARTESIAN_POINT ( 'NONE',  ( 0.2891555358219910499, -0.2891555358219909944, -2.145669291338582862 ) ) ;
#9802=CARTESIAN_POINT ( 'NONE',  ( 0.1958661417322836440, -0.3392501089628017219, -0.8713910761154854967 ) ) ;
#9809=CARTESIAN_POINT ( 'NONE',  ( 0.1049643490035304522, -0.3917322834645668994, -0.3228153298874523180 ) ) ;
#9813=EDGE_CURVE ( 'NONE', #59522, #83292, #80656, .T. ) ;
#9817=CARTESIAN_POINT ( 'NONE',  ( -0.3392501089628017219, -0.1958661417322836995, -1.624035063813334956 ) ) ;
#9824=CARTESIAN_POINT ( 'NONE',  ( -0.1958661417322836718, 0.3392501089628017219, -0.8851706036745407014 ) ) ;
#9832=CARTESIAN_POINT ( 'NONE',  ( -0.4724409448818896462, -0.1265901696524993070, -0.9101049868766404316 ) ) ;
#9833=CARTESIAN_POINT ( 'NONE',  ( -0.1049643490035307020, 0.3917322834645669549, -2.203412073490814027 ) ) ;
#9840=CARTESIAN_POINT ( 'NONE',  ( 0.1049643490035304938, -0.3917322834645669549, -0.7998687664041995715 ) ) ;
#9843=CARTESIAN_POINT ( 'NONE',  ( 0.3917322834645670104, -0.1049643490035303411, -1.456036745406824151 ) ) ;
#9844=CARTESIAN_POINT ( 'NONE',  ( -0.1998031496062994405, 0.3460692066303957537, -2.452099737532808188 ) ) ;
#9855=CARTESIAN_POINT ( 'NONE',  ( -0.3996062992125986035, 0.1070741851644051584, -1.999343832020997525 ) ) ;
#9864=CARTESIAN_POINT ( 'NONE',  ( -0.2867679344610366554, 0.2867679344610365444, -1.044600106790339433 ) ) ;
#9874=CARTESIAN_POINT ( 'NONE',  ( -0.3392501089628017219, -0.1958661417322836995, -0.5216728590889256889 ) ) ;
#9877=CARTESIAN_POINT ( 'NONE',  ( -0.4724409448818898682, -8.678599364036362592E-17, -1.848425196850393526 ) ) ;
#9897=CARTESIAN_POINT ( 'NONE',  ( 0.3460692066303959202, -0.1998031496062991630, -2.229002624671916344 ) ) ;
#9902=CARTESIAN_POINT ( 'NONE',  ( 4.893765752498283924E-17, -0.3996062992125986035, -1.653543307086614123 ) ) ;
#9903=CARTESIAN_POINT ( 'NONE',  ( -0.3949938075777409408, -0.1058382717557502933, -1.148293963254593431 ) ) ;
#9904=CARTESIAN_POINT ( 'NONE',  ( 0.1070741851644054915, -0.3996062992125986035, -2.604986876640420057 ) ) ;
#9906=CARTESIAN_POINT ( 'NONE',  ( -0.1958661417322834220, -0.3392501089628018884, -0.3727034120734908362 ) ) ;
#9910=CARTESIAN_POINT ( 'NONE',  ( -0.3949938075777409963, -7.255918531996591613E-17, -2.005905511811023612 ) ) ;
#9914=CARTESIAN_POINT ( 'NONE',  ( 0.2362204724409451007, -0.4091458600556402980, -2.611548556430446144 ) ) ;
#9915=CARTESIAN_POINT ( 'NONE',  ( -0.2925321140481932924, 0.2925321140481931814, -1.751968503937007648 ) ) ;
#9916=CARTESIAN_POINT ( 'NONE',  ( -1.157146581871515012E-16, 0.4724409448818898682, -2.753937007874015741 ) ) ;
#9923=CARTESIAN_POINT ( 'NONE',  ( -0.1958661417322836440, 0.3392501089628016664, -2.770321891567242734 ) ) ;
#9930=CARTESIAN_POINT ( 'NONE',  ( -0.1958661417322836718, 0.3392501089628017219, -0.2552493438320210806 ) ) ;
#9932=CARTESIAN_POINT ( 'NONE',  ( 4.797336870675656522E-17, -0.3917322834645670104, -2.275590551181102317 ) ) ;
#9934=ORIENTED_EDGE ( 'NONE', *, *, #1832, .F. ) ;
#9935=CARTESIAN_POINT ( 'NONE',  ( 0.3420746716998659953, 0.1974969037888705536, -2.178477690288714186 ) ) ;
#9939=CARTESIAN_POINT ( 'NONE',  ( 0.3996062992125986590, -0.1070741851644053111, -1.213910761154855189 ) ) ;
#9941=CARTESIAN_POINT ( 'NONE',  ( 0.4724409448818898682, 2.892866454678787531E-17, -0.8248031496062991907 ) ) ;
#9942=DIRECTION ( 'NONE',  ( 0.000000000000000000, 0.000000000000000000, 1.000000000000000000 ) ) ;
#9943=CARTESIAN_POINT ( 'NONE',  ( 0.009627693921961720178, -0.3964540044758448900, -2.755905511808609987 ) ) ;
#9944=CARTESIAN_POINT ( 'NONE',  ( 0.3917322834645670104, -0.1049643490035303411, -0.03871391076115493490 ) ) ;
#9950=CARTESIAN_POINT ( 'NONE',  ( -0.1049643490035307020, 0.3917322834645669549, 0.1587926509186352031 ) ) ;
#9956=( LENGTH_UNIT ( ) NAMED_UNIT ( * ) SI_UNIT ( $, .METRE. ) );
#9957=CARTESIAN_POINT ( 'NONE',  ( 0.4724409448818897572, -0.1265901696524988906, -1.528871391076114916 ) ) ;
#9960=CARTESIAN_POINT ( 'NONE',  ( 4.797336870675656522E-17, -0.3917322834645670104, -0.5433070866141732624 ) ) ;
#9968=CARTESIAN_POINT ( 'NONE',  ( -0.3917322834645670659, 0.1049643490035301607, 0.04463873835401757639 ) ) ;
#9971=CARTESIAN_POINT ( 'NONE',  ( -0.3392501089628019995, 0.1958661417322832277, -0.5833333333333334814 ) ) ;
#9972=AXIS2_PLACEMENT_3D ( 'NONE', #7443, #51609, #33114 ) ;
#9978=CARTESIAN_POINT ( 'NONE',  ( 4.797336870675656522E-17, -0.3917322834645670104, -2.275590551181102317 ) ) ;
#9982=CARTESIAN_POINT ( 'NONE',  ( 0.4091458600556403535, 0.2362204724409449896, -0.3654855643044619407 ) ) ;
#9995=CARTESIAN_POINT ( 'NONE',  ( 0.3996062992125986035, -0.1070741851644052972, -1.605643044619422977 ) ) ;
#10003=CARTESIAN_POINT ( 'NONE',  ( 0.3996062992125984925, 0.1070741851644054499, -0.3589238845144357426 ) ) ;
#10004=CARTESIAN_POINT ( 'NONE',  ( 4.893765752498283924E-17, -0.3996062992125986035, -0.7086614173228346081 ) ) ;
#10005=CARTESIAN_POINT ( 'NONE',  ( -0.1058382717557497937, -0.3949938075777411628, 0.08530183727034117147 ) ) ;
#10011=CARTESIAN_POINT ( 'NONE',  ( 0.1058382717557500852, -0.3949938075777408852, -1.106955380577427706 ) ) ;
#10016=CARTESIAN_POINT ( 'NONE',  ( 0.4724409448818897572, -0.1265901696524988906, -1.056430446194225992 ) ) ;
#10017=CARTESIAN_POINT ( 'NONE',  ( -0.1070741851644051862, -0.3996062992125986590, -2.276902887139107268 ) ) ;
#10020=CARTESIAN_POINT ( 'NONE',  ( -0.2867679344610365444, -0.2867679344610367664, -0.8431951688002119472 ) ) ;
#10033=CARTESIAN_POINT ( 'NONE',  ( 4.797336870675656522E-17, -0.3917322834645670104, -1.173228346456692828 ) ) ;
#10036=CARTESIAN_POINT ( 'NONE',  ( 4.837279021331060870E-17, -0.3949938075777409963, -0.8661417322834645827 ) ) ;
#10053=CARTESIAN_POINT ( 'NONE',  ( 0.1998031496062992740, 0.3460692066303959757, -1.561679790026246684 ) ) ;
#10056=CARTESIAN_POINT ( 'NONE',  ( -0.3996062992125986590, 0.1070741851644051723, -1.054461942257217899 ) ) ;
#10060=CARTESIAN_POINT ( 'NONE',  ( 0.1265901696524990294, -0.4724409448818896462, -0.2427821522309711322 ) ) ;
#10061=CARTESIAN_POINT ( 'NONE',  ( 0.3917322834645670104, 2.398668435337828261E-17, -2.722440944881889369 ) ) ;
#10067=CARTESIAN_POINT ( 'NONE',  ( 0.4091458600556403535, 0.2362204724409449896, -2.412729658792650778 ) ) ;
#10070=CARTESIAN_POINT ( 'NONE',  ( -0.1058382717557503072, 0.3949938075777408852, -1.658136482939632339 ) ) ;
#10076=CARTESIAN_POINT ( 'NONE',  ( 0.2362204724409449064, 0.4091458600556404646, -2.268372703412073310 ) ) ;
#10081=CARTESIAN_POINT ( 'NONE',  ( 0.2867679344610365999, 0.2867679344610365999, -2.422552862695851683 ) ) ;
#10095=CARTESIAN_POINT ( 'NONE',  ( 0.1070741851644054776, -0.3996062992125984925, -0.3195538057742782212 ) ) ;
#10098=CARTESIAN_POINT ( 'NONE',  ( -0.3917322834645669549, -0.1049643490035306603, -1.705380577427821898 ) ) ;
#10109=CARTESIAN_POINT ( 'NONE',  ( -0.1070741851644051862, -0.3996062992125986590, -0.9363517060367454459 ) ) ;
#10117=CARTESIAN_POINT ( 'NONE',  ( -0.3392501089628017219, -0.1958661417322836718, -1.554461942257217899 ) ) ;
#10118=CARTESIAN_POINT ( 'NONE',  ( 5.785732909357575061E-17, -0.4724409448818898682, -2.125984251968504157 ) ) ;
#10121=CARTESIAN_POINT ( 'NONE',  ( 0.4724409448818897017, 0.1265901696524990294, -0.4396325459317584894 ) ) ;
#10122=CARTESIAN_POINT ( 'NONE',  ( 0.2925321140481931814, -0.2925321140481931259, -2.379921259842519898 ) ) ;
#10124=CARTESIAN_POINT ( 'NONE',  ( -0.3460692066303958092, -0.1998031496062994683, -0.5249343832020997302 ) ) ;
#10127=CARTESIAN_POINT ( 'NONE',  ( 0.2867679344610365999, -0.2867679344610365444, -2.137795275590551380 ) ) ;
#10138=CARTESIAN_POINT ( 'NONE',  ( 0.3917322834645668994, -0.1049643490035303134, -1.451424253771966599 ) ) ;
#10142=CARTESIAN_POINT ( 'NONE',  ( 0.1049643490035304938, -0.3917322834645669549, 0.08005249343832024356 ) ) ;
#10145=CARTESIAN_POINT ( 'NONE',  ( -0.1049643490035307158, 0.3917322834645670104, -2.680465510007561836 ) ) ;
#10153=CARTESIAN_POINT ( 'NONE',  ( -9.594673741351313045E-17, 0.3917322834645670659, -1.414061310532495286 ) ) ;
#10155=CARTESIAN_POINT ( 'NONE',  ( -0.3392501089628017219, -0.1958661417322836718, -2.184383202099737797 ) ) ;
#10160=CARTESIAN_POINT ( 'NONE',  ( 0.2925321140481932369, 0.2925321140481932369, -0.2952755905511811885 ) ) ;
#10162=CARTESIAN_POINT ( 'NONE',  ( 0.2925321140481932369, -0.2925321140481931814, 0.1397637795275590289 ) ) ;
#10164=CARTESIAN_POINT ( 'NONE',  ( -0.3996062992125987146, 0.1070741851644051862, -2.080052493438320216 ) ) ;
#10170=CARTESIAN_POINT ( 'NONE',  ( -0.3458507752293906723, -0.3458507752293910609, -0.9232283464566929387 ) ) ;
#10173=CARTESIAN_POINT ( 'NONE',  ( -0.2891555358219909388, -0.2891555358219912164, -0.7657480314960630752 ) ) ;
#10178=CARTESIAN_POINT ( 'NONE',  ( 0.1058382717557500852, -0.3949938075777408852, -0.4770341207349081403 ) ) ;
#10186=CARTESIAN_POINT ( 'NONE',  ( 0.2925321140481932369, 0.2925321140481932369, -1.159448818897637734 ) ) ;
#10188=CARTESIAN_POINT ( 'NONE',  ( 0.2867679344610365999, -0.2867679344610365444, -1.192913385826771755 ) ) ;
#10190=CARTESIAN_POINT ( 'NONE',  ( -0.3436793299028276794, 0.1882840440723393405, 1.128668216881735357E-17 ) ) ;
#10198=CARTESIAN_POINT ( 'NONE',  ( -0.4724409448818898682, -8.678599364036362592E-17, -0.2736220472440945017 ) ) ;
#10220=CARTESIAN_POINT ( 'NONE',  ( 0.4724409448818896462, 0.1265901696524990294, -0.1246719160104986929 ) ) ;
#10221=CARTESIAN_POINT ( 'NONE',  ( -0.1974969037888706647, 0.3420746716998658843, -2.217847769028871596 ) ) ;
#10224=CARTESIAN_POINT ( 'NONE',  ( 0.2867679344610365999, 0.2867679344610365999, -0.9173228346456693272 ) ) ;
#10226=CARTESIAN_POINT ( 'NONE',  ( 0.4091458600556404646, -0.2362204724409448231, -2.467191601049868677 ) ) ;
#10227=CARTESIAN_POINT ( 'NONE',  ( 0.2362204724409449064, 0.4091458600556404646, -0.8510498687664042050 ) ) ;
#10233=CARTESIAN_POINT ( 'NONE',  ( 0.3392501089628018329, 0.1958661417322835052, -0.3687470884176359265 ) ) ;
#10239=CARTESIAN_POINT ( 'NONE',  ( -0.1049643490035307158, 0.3917322834645670104, -1.420622990322521373 ) ) ;
#10245=CARTESIAN_POINT ( 'NONE',  ( -0.1049643490035307020, 0.3917322834645669549, -1.036089238845144589 ) ) ;
#10254=CARTESIAN_POINT ( 'NONE',  ( 0.3392501089628018884, -0.1958661417322834220, -2.301837270341207553 ) ) ;
#10264=CARTESIAN_POINT ( 'NONE',  ( 0.1958661417322836440, -0.3392501089628017219, -0.9639107611548557442 ) ) ;
#10267=CARTESIAN_POINT ( 'NONE',  ( 0.3996062992125986035, -0.1070741851644052972, -2.393044619422572072 ) ) ;
#10276=CARTESIAN_POINT ( 'NONE',  ( 0.3996062992125985480, -0.1070741851644052972, -2.078083989501312345 ) ) ;
#10286=CARTESIAN_POINT ( 'NONE',  ( -0.3917322834645668994, -0.1049643490035306742, -1.543287770832334038 ) ) ;
#10295=CARTESIAN_POINT ( 'NONE',  ( 0.1049643490035303967, 0.3917322834645670659, -0.4626177409786895178 ) ) ;
#10299=CARTESIAN_POINT ( 'NONE',  ( 5.785732909357575061E-17, -0.4724409448818898682, -1.887795275590550936 ) ) ;
#10322=CARTESIAN_POINT ( 'NONE',  ( -0.3460692066303960313, 0.1998031496062989965, -2.307742782152231165 ) ) ;
#10329=CARTESIAN_POINT ( 'NONE',  ( -0.3996062992125987146, 0.1070741851644051862, -1.607611548556430403 ) ) ;
#10330=CARTESIAN_POINT ( 'NONE',  ( -0.3949938075777411628, 0.1058382717557497937, -1.292650918635170676 ) ) ;
#10331=CARTESIAN_POINT ( 'NONE',  ( -0.1070741851644051862, -0.3996062992125987146, -2.434383202099737353 ) ) ;
#10332=CARTESIAN_POINT ( 'NONE',  ( -0.4091458600556405756, 0.2362204724409446288, -0.6561679790026246906 ) ) ;
#10333=CARTESIAN_POINT ( 'NONE',  ( -0.3917322834645670104, -7.196005306013484475E-17, -0.03149606299212594218 ) ) ;
#10337=CARTESIAN_POINT ( 'NONE',  ( -0.3949938075777408852, -0.1058382717557502933, -2.327427821522309870 ) ) ;
#10342=CARTESIAN_POINT ( 'NONE',  ( -0.2362204724409447953, -0.4091458600556404646, -2.427821522309711266 ) ) ;
#10343=CARTESIAN_POINT ( 'NONE',  ( 0.2925321140481932369, -0.2925321140481932369, -1.673228346456692828 ) ) ;
#10350=CARTESIAN_POINT ( 'NONE',  ( 0.3917322834645668994, -0.1049643490035303134, -2.868747088417636704 ) ) ;
#10357=CARTESIAN_POINT ( 'NONE',  ( -0.3917322834645669549, -0.1049643490035306603, -0.1305774278215224293 ) ) ;
#10359=CARTESIAN_POINT ( 'NONE',  ( -0.3917322834645670104, -7.196005306013484475E-17, -2.393700787401574992 ) ) ;
#10362=CARTESIAN_POINT ( 'NONE',  ( 0.1058382717557499880, 0.3949938075777411073, -2.828083989501312345 ) ) ;
#10366=CARTESIAN_POINT ( 'NONE',  ( -0.3996062992125986035, -7.340648628747425578E-17, -0.9842519685039369248 ) ) ;
#10370=CARTESIAN_POINT ( 'NONE',  ( 0.002049465651556450167, -0.3981765293560898256, -2.755905511811024056 ) ) ;
#10371=CARTESIAN_POINT ( 'NONE',  ( -9.594673741351313045E-17, 0.3917322834645670104, -0.2421259842519686289 ) ) ;
#10378=CARTESIAN_POINT ( 'NONE',  ( 0.1958661417322836440, -0.3392501089628017219, -0.2414698162729658204 ) ) ;
#10382=LENGTH_MEASURE_WITH_UNIT ( LENGTH_MEASURE( 0.02539999999999999897 ), #9956 );
#10384=CARTESIAN_POINT ( 'NONE',  ( -0.1265901696524993347, 0.4724409448818895907, -1.738845144356955696 ) ) ;
#10395=CARTESIAN_POINT ( 'NONE',  ( -0.1958661417322836440, 0.3392501089628016664, -0.09315653723653360974 ) ) ;
#10397=CARTESIAN_POINT ( 'NONE',  ( -0.2867679344610366554, 0.2867679344610365444, -0.5767716535433071723 ) ) ;
#10402=CARTESIAN_POINT ( 'NONE',  ( 0.3392501089628018884, -0.1958661417322834220, -2.301837270341207553 ) ) ;
#10405=CARTESIAN_POINT ( 'NONE',  ( -0.4724409448818899238, 0.1265901696524986686, -0.8969816272965877024 ) ) ;
#10413=CARTESIAN_POINT ( 'NONE',  ( 0.4724409448818898682, 2.892866454678787531E-17, -0.2755905511811023723 ) ) ;
#10416=CARTESIAN_POINT ( 'NONE',  ( -0.1998031496062991630, -0.3460692066303959202, -2.189632545931758489 ) ) ;
#10424=CARTESIAN_POINT ( 'NONE',  ( 0.1070741851644053527, 0.3996062992125985480, -0.2276902887139107545 ) ) ;
#10425=CARTESIAN_POINT ( 'NONE',  ( 0.3460692066303959202, 0.1998031496062993295, -0.6036745406824146620 ) ) ;
#10426=CARTESIAN_POINT ( 'NONE',  ( 0.1049643490035304799, -0.3917322834645670104, -2.916685982448506298 ) ) ;
#10433=CARTESIAN_POINT ( 'NONE',  ( 0.3949938075777409408, -0.1058382717557499186, -0.8182414698162731037 ) ) ;
#10438=CARTESIAN_POINT ( 'NONE',  ( 0.1265901696524990294, -0.4724409448818896462, -1.187664041994750619 ) ) ;
#10440=CARTESIAN_POINT ( 'NONE',  ( -0.3460692066303958092, -0.1998031496062994683, -2.257217847769029007 ) ) ;
#10443=CARTESIAN_POINT ( 'NONE',  ( 0.1049643490035303967, 0.3917322834645670659, -0.9350586858605794971 ) ) ;
#10456=CARTESIAN_POINT ( 'NONE',  ( -0.1049643490035302024, -0.3917322834645671215, -1.166666666666666519 ) ) ;
#10459=CARTESIAN_POINT ( 'NONE',  ( -0.3949938075777409408, -0.1058382717557502933, -1.463254593175853158 ) ) ;
#10463=CARTESIAN_POINT ( 'NONE',  ( -0.2925321140481930704, -0.2925321140481933480, 0.09842519685039367860 ) ) ;
#10475=CARTESIAN_POINT ( 'NONE',  ( -0.2925321140481930704, -0.2925321140481933480, -1.791338582677165059 ) ) ;
#10478=CARTESIAN_POINT ( 'NONE',  ( -0.1998031496062994405, 0.3460692066303957537, -1.664698162729658426 ) ) ;
#10482=CARTESIAN_POINT ( 'NONE',  ( -0.4724409448818895907, -0.1265901696524993070, -0.5183727034120735322 ) ) ;
#10484=CARTESIAN_POINT ( 'NONE',  ( -0.3392501089628019995, 0.1958661417322832277, -2.630577427821522374 ) ) ;
#10490=CARTESIAN_POINT ( 'NONE',  ( -0.4091458600556402980, -0.2362204724409451284, -2.333989501312335957 ) ) ;
#10492=CARTESIAN_POINT ( 'NONE',  ( -9.674558042662122972E-17, 0.3949938075777409963, -1.966535433070866423 ) ) ;
#10498=CARTESIAN_POINT ( 'NONE',  ( 0.4724409448818915891, -0.1265901696524958653, -2.235564304461942875 ) ) ;
#10502=CARTESIAN_POINT ( 'NONE',  ( -0.3392501089628018329, -0.1958661417322836440, -2.337251025425510331 ) ) ;
#10515=CARTESIAN_POINT ( 'NONE',  ( 0.2925321140481932369, 0.2925321140481932369, -0.8444881889763780070 ) ) ;
#10516=CARTESIAN_POINT ( 'NONE',  ( -0.1958661417322836718, 0.3392501089628017219, -1.830052493438320216 ) ) ;
#10525=CARTESIAN_POINT ( 'NONE',  ( -0.1998031496062991630, -0.3460692066303959202, -1.402230971128609172 ) ) ;
#10532=CARTESIAN_POINT ( 'NONE',  ( -0.1049643490035307020, 0.3917322834645669549, -1.666010498687664043 ) ) ;
#10533=CARTESIAN_POINT ( 'NONE',  ( -0.4724409448818898682, -8.678599364036362592E-17, -2.086614173228346303 ) ) ;
#10537=CARTESIAN_POINT ( 'NONE',  ( 0.3460692066303959202, -0.1998031496062991630, -2.386482939632545985 ) ) ;
#10539=CARTESIAN_POINT ( 'NONE',  ( 0.1998031496062994405, -0.3460692066303958092, -0.8792650918635170898 ) ) ;
#10542=CARTESIAN_POINT ( 'NONE',  ( 0.1958661417322834775, 0.3392501089628018884, -2.498687664041994605 ) ) ;
#10552=CARTESIAN_POINT ( 'NONE',  ( 0.3917322834645668994, -0.1049643490035303134, -1.608904568732596685 ) ) ;
#10555=CARTESIAN_POINT ( 'NONE',  ( 0.3917322834645670104, -0.1049643490035303411, -2.715879265091863726 ) ) ;
#10558=CARTESIAN_POINT ( 'NONE',  ( -0.3917322834645670104, -0.1049643490035307020, -2.877315903708348444 ) ) ;
#10566=CARTESIAN_POINT ( 'NONE',  ( 0.1958661417322836718, -0.3392501089628017219, -1.190964197671602998 ) ) ;
#10569=CARTESIAN_POINT ( 'NONE',  ( 0.3917322834645670104, 2.398668435337828261E-17, -2.250000000000000000 ) ) ;
#10574=CARTESIAN_POINT ( 'NONE',  ( -0.3460692066303958092, -0.1998031496062994683, -0.3674540682414698112 ) ) ;
#10576=CARTESIAN_POINT ( 'NONE',  ( -0.1070741851644051862, -0.3996062992125986590, 0.1660104986876640432 ) ) ;
#10578=CARTESIAN_POINT ( 'NONE',  ( -0.1070741851644051862, -0.3996062992125987146, -2.276902887139107268 ) ) ;
#10583=CARTESIAN_POINT ( 'NONE',  ( 0.4091458600556404646, -0.2362204724409448231, -0.9691601049868766582 ) ) ;
#10587=CARTESIAN_POINT ( 'NONE',  ( 0.1974969037888704704, 0.3420746716998660508, -0.3786089238845145033 ) ) ;
#10601=CARTESIAN_POINT ( 'NONE',  ( 0.1998031496062994128, -0.3460692066303957537, -1.585958005249344049 ) ) ;
#10603=CARTESIAN_POINT ( 'NONE',  ( -9.594673741351313045E-17, 0.3917322834645670104, -1.251968503937008093 ) ) ;
#10612=EDGE_CURVE ( 'NONE', #35624, #2570, #16294, .T. ) ;
#10625=CARTESIAN_POINT ( 'NONE',  ( -0.3917322834645670104, -0.1049643490035307020, -1.932434013944568818 ) ) ;
#10636=CARTESIAN_POINT ( 'NONE',  ( -0.1265901696524993347, 0.4724409448818895907, 0.1509186351706036378 ) ) ;
#10637=CARTESIAN_POINT ( 'NONE',  ( 0.3420746716998659953, 0.1974969037888705536, -2.808398950131233640 ) ) ;
#10640=CARTESIAN_POINT ( 'NONE',  ( 0.1958661417322834775, 0.3392501089628018884, -1.238845144356955252 ) ) ;
#10642=CARTESIAN_POINT ( 'NONE',  ( -0.3458507752293906723, -0.3458507752293910609, -2.263779527559055094 ) ) ;
#10648=CARTESIAN_POINT ( 'NONE',  ( -0.3917322834645669549, -7.196005306013483243E-17, -0.2768835713572685431 ) ) ;
#10653=CARTESIAN_POINT ( 'NONE',  ( -0.4091458600556405756, 0.2362204724409446288, -0.02624671916010498651 ) ) ;
#10654=CARTESIAN_POINT ( 'NONE',  ( 0.1070741851644054915, -0.3996062992125986035, -2.919947506561679784 ) ) ;
#10655=CARTESIAN_POINT ( 'NONE',  ( 4.797336870675656522E-17, -0.3917322834645670659, -1.807762097934070278 ) ) ;
#10662=CARTESIAN_POINT ( 'NONE',  ( 0.1958661417322834775, 0.3392501089628018884, -1.173884514435695525 ) ) ;
#10672=CARTESIAN_POINT ( 'NONE',  ( 0.1049643490035303689, 0.3917322834645670104, -2.190288713910760521 ) ) ;
#10673=VERTEX_POINT ( 'NONE', #41938 ) ;
#10679=CARTESIAN_POINT ( 'NONE',  ( -0.3392501089628019995, 0.1958661417322832277, -0.8982939632545933195 ) ) ;
#10683=CARTESIAN_POINT ( 'NONE',  ( 0.3460692066303959202, -0.1998031496062991630, -2.386482939632545985 ) ) ;
#10701=CARTESIAN_POINT ( 'NONE',  ( 0.2867679344610365999, -0.2867679344610365999, -1.595781209152543845 ) ) ;
#10710=CARTESIAN_POINT ( 'NONE',  ( 0.3917322834645670659, 2.398668435337828261E-17, -0.4298093420285583055 ) ) ;
#10714=CARTESIAN_POINT ( 'NONE',  ( 0.3458507752293908943, -0.3458507752293908943, -2.064960629921259283 ) ) ;
#10734=CARTESIAN_POINT ( 'NONE',  ( 0.3996062992125985480, 2.446882876249141654E-17, -2.084645669291338876 ) ) ;
#10739=CARTESIAN_POINT ( 'NONE',  ( -0.1998031496062991907, -0.3460692066303959757, -1.797900262467191590 ) ) ;
#10740=CARTESIAN_POINT ( 'NONE',  ( 0.1058382717557499880, 0.3949938075777411073, -0.9383202099737534274 ) ) ;
#10741=CARTESIAN_POINT ( 'NONE',  ( -0.3460692066303958092, -0.1998031496062994683, -2.414698162729658648 ) ) ;
#10743=CARTESIAN_POINT ( 'NONE',  ( -9.594673741351313045E-17, 0.3917322834645670104, -0.7795275590551180578 ) ) ;
#10747=CARTESIAN_POINT ( 'NONE',  ( 0.3949938075777408852, 0.1058382717557500435, -2.248687664041995049 ) ) ;
#10750=CARTESIAN_POINT ( 'NONE',  ( 0.2362204724409449064, 0.4091458600556404646, -2.506561679790026087 ) ) ;
#10751=CARTESIAN_POINT ( 'NONE',  ( 0.2925321140481932369, 0.2925321140481932369, -1.712598425196850460 ) ) ;
#10757=CARTESIAN_POINT ( 'NONE',  ( 0.1958661417322836162, -0.3392501089628018329, -2.849062049047557998 ) ) ;
#10758=CARTESIAN_POINT ( 'NONE',  ( -0.2017716535433071445, 0.2017716535433070613, -0.3937007874015748254 ) ) ;
#10764=CARTESIAN_POINT ( 'NONE',  ( 0.3392501089628018884, -0.1958661417322834220, -0.03215223097112869521 ) ) ;
#10766=CARTESIAN_POINT ( 'NONE',  ( 0.3917322834645669549, 0.1049643490035304660, -2.321522309711285814 ) ) ;
#10769=CARTESIAN_POINT ( 'NONE',  ( -9.674558042662121740E-17, 0.3949938075777409963, -2.834645669291338432 ) ) ;
#10773=CARTESIAN_POINT ( 'NONE',  ( 4.893765752498283924E-17, -0.3996062992125986035, -1.023622047244094446 ) ) ;
#10778=CARTESIAN_POINT ( 'NONE',  ( -0.1049643490035307020, 0.3917322834645669549, -0.4061679790026246351 ) ) ;
#10784=CARTESIAN_POINT ( 'NONE',  ( 0.1958661417322834775, 0.3392501089628018884, -0.2939632545931757934 ) ) ;
#10788=CARTESIAN_POINT ( 'NONE',  ( -0.4724409448818895907, -0.1265901696524993070, -1.620734908136482799 ) ) ;
#10790=CARTESIAN_POINT ( 'NONE',  ( -0.3917322834645670104, -7.196005306013484475E-17, -2.643700787401574548 ) ) ;
#10797=CARTESIAN_POINT ( 'NONE',  ( 0.2867679344610365999, 0.2867679344610365999, -0.2178284532470323442 ) ) ;
#10799=CARTESIAN_POINT ( 'NONE',  ( 0.3917322834645669549, 0.1049643490035304660, -0.5242782152230972548 ) ) ;
#10804=CARTESIAN_POINT ( 'NONE',  ( 0.1049643490035304938, -0.3917322834645669549, -2.439632545931758045 ) ) ;
#10807=CARTESIAN_POINT ( 'NONE',  ( -1.157146581871515012E-16, 0.4724409448818898682, -0.7066929133858268486 ) ) ;
#10818=CARTESIAN_POINT ( 'NONE',  ( 0.3996062992125985480, 2.446882876249141654E-17, -1.927165354330708569 ) ) ;
#10827=CARTESIAN_POINT ( 'NONE',  ( -0.3996062992125984925, -0.1070741851644056719, -0.4376640419947506744 ) ) ;
#10828=CARTESIAN_POINT ( 'NONE',  ( 0.3996062992125986590, -0.1070741851644053111, -0.5839895013123358458 ) ) ;
#10829=CARTESIAN_POINT ( 'NONE',  ( -0.1974969037888706647, 0.3420746716998658843, 0.1443569553805773842 ) ) ;
#10835=CARTESIAN_POINT ( 'NONE',  ( -0.2891555358219911054, 0.2891555358219909388, -1.041338582677165503 ) ) ;
#10840=CARTESIAN_POINT ( 'NONE',  ( -0.4091458600556402980, -0.2362204724409451284, -1.312335958005249381 ) ) ;
#10841=CARTESIAN_POINT ( 'NONE',  ( -9.787531504996567848E-17, 0.3996062992125986035, -2.362204724409448620 ) ) ;
#10844=CARTESIAN_POINT ( 'NONE',  ( -0.2867679344610367109, 0.2867679344610365444, -0.9613054050206844003 ) ) ;
#10855=EDGE_CURVE ( 'NONE', #32199, #5751, #15011, .T. ) ;
#10856=CARTESIAN_POINT ( 'NONE',  ( -0.1049643490035307020, 0.3917322834645669549, -0.9435695538057740084 ) ) ;
#10859=CARTESIAN_POINT ( 'NONE',  ( 0.3420746716998660508, -0.1974969037888703871, -1.364829396325459410 ) ) ;
#10870=CARTESIAN_POINT ( 'NONE',  ( -0.3392501089628019995, 0.1958661417322832277, 0.04658792650918625738 ) ) ;
#10875=CARTESIAN_POINT ( 'NONE',  ( -0.3460692066303958092, -0.1998031496062994683, -2.257217847769029007 ) ) ;
#10878=CARTESIAN_POINT ( 'NONE',  ( -0.3996062992125985480, -7.340648628747423112E-17, -1.690944881889763884 ) ) ;
#10883=CARTESIAN_POINT ( 'NONE',  ( -0.1265901696524986964, -0.4724409448818899238, -0.5446194225721783244 ) ) ;
#10885=CARTESIAN_POINT ( 'NONE',  ( -0.2867679344610364334, -0.2867679344610367109, -0.05118110236220468900 ) ) ;
#10891=CARTESIAN_POINT ( 'NONE',  ( -0.4724409448818899238, 0.1265901696524986686, -2.314304461942256808 ) ) ;
#10893=CARTESIAN_POINT ( 'NONE',  ( -0.3420746716998662729, 0.1974969037888702206, -2.150262467191601523 ) ) ;
#10916=CARTESIAN_POINT ( 'NONE',  ( -0.1070741851644056997, 0.3996062992125984925, -0.8707349081364830212 ) ) ;
#10917=CARTESIAN_POINT ( 'NONE',  ( -0.3392501089628017219, -0.1958661417322836718, -2.341863517060367439 ) ) ;
#10926=CARTESIAN_POINT ( 'NONE',  ( 0.2925321140481932369, 0.2925321140481932369, -1.316929133858267820 ) ) ;
#10928=CARTESIAN_POINT ( 'NONE',  ( -0.4724409448818917001, 0.1265901696524956710, -2.237532808398950301 ) ) ;
#10929=ORIENTED_EDGE ( 'NONE', *, *, #10612, .F. ) ;
#10933=CARTESIAN_POINT ( 'NONE',  ( 0.3917322834645670104, 2.398668435337828261E-17, -1.462598425196850460 ) ) ;
#10938=CARTESIAN_POINT ( 'NONE',  ( 0.2925321140481931814, 0.2925321140481931814, -2.419291338582677309 ) ) ;
#10940=CARTESIAN_POINT ( 'NONE',  ( -0.3996062992125986035, -0.1070741851644056997, -0.9908136482939633449 ) ) ;
#10941=EDGE_LOOP ( 'NONE', ( #25934, #13972, #37451, #72748 ) ) ;
#10943=CARTESIAN_POINT ( 'NONE',  ( -0.3917322834645669549, -0.1049643490035306603, -2.557742782152230721 ) ) ;
#10953=CARTESIAN_POINT ( 'NONE',  ( -0.1958661417322834497, -0.3392501089628018884, -1.877933440123672471 ) ) ;
#10956=CARTESIAN_POINT ( 'NONE',  ( 0.3917322834645670104, 2.398668435337828261E-17, 0.04724409448818902429 ) ) ;
#10958=EDGE_LOOP ( 'NONE', ( #65709, #73696, #15934, #12428 ) ) ;
#10959=CARTESIAN_POINT ( 'NONE',  ( 0.2891555358219910499, 0.2891555358219910499, -0.2952755905511811885 ) ) ;
#10967=CARTESIAN_POINT ( 'NONE',  ( -0.1958661417322836995, 0.3392501089628017219, -1.112224040191287955 ) ) ;
#10969=CARTESIAN_POINT ( 'NONE',  ( -0.1049643490035302024, -0.3917322834645671215, -2.833989501312335957 ) ) ;
#10974=CARTESIAN_POINT ( 'NONE',  ( 0.3996062992125986035, 2.446882876249141962E-17, -1.062992125984252079 ) ) ;
#10976=CARTESIAN_POINT ( 'NONE',  ( -0.1070741851644051862, -0.3996062992125986590, -0.4639107611548556331 ) ) ;
#10978=CARTESIAN_POINT ( 'NONE',  ( -0.2925321140481932924, 0.2925321140481931814, -2.381889763779527325 ) ) ;
#10982=CARTESIAN_POINT ( 'NONE',  ( -0.4724409448818899238, 0.1265901696524986686, -0.8969816272965877024 ) ) ;
#10985=CARTESIAN_POINT ( 'NONE',  ( -0.3949938075777408852, -0.1058382717557502933, -0.4376640419947507299 ) ) ;
#10991=FACE_OUTER_BOUND ( 'NONE', #6110, .T. ) ;
#10998=LINE ( 'NONE', #36658, #47851 ) ;
#11000=CARTESIAN_POINT ( 'NONE',  ( -0.2925321140481930149, -0.2925321140481933480, -1.710629921259842812 ) ) ;
#11003=CARTESIAN_POINT ( 'NONE',  ( -0.3917322834645670104, -7.196005306013484475E-17, -1.291338582677165503 ) ) ;
#11035=CARTESIAN_POINT ( 'NONE',  ( -0.3917322834645669549, -0.1049643490035306603, -2.242782152230970993 ) ) ;
#11038=CARTESIAN_POINT ( 'NONE',  ( -0.4724409448818895907, -0.1265901696524993070, -0.5183727034120735322 ) ) ;
#11039=CARTESIAN_POINT ( 'NONE',  ( -0.3949938075777411628, 0.1058382717557497937, -2.867454068241469756 ) ) ;
#11042=CARTESIAN_POINT ( 'NONE',  ( -0.1049643490035307020, 0.3917322834645669549, -1.258530183727033958 ) ) ;
#11044=CARTESIAN_POINT ( 'NONE',  ( -0.4091458600556402980, -0.2362204724409451284, -2.257217847769029007 ) ) ;
#11051=CARTESIAN_POINT ( 'NONE',  ( -0.3917322834645670659, 0.1049643490035301607, -0.7427628364491322133 ) ) ;
#11059=CARTESIAN_POINT ( 'NONE',  ( -0.3392501089628017219, -0.1958661417322836995, -1.938995693734595127 ) ) ;
#11065=CARTESIAN_POINT ( 'NONE',  ( 0.2867679344610365999, -0.2867679344610365444, -0.8129921259842518566 ) ) ;
#11077=CARTESIAN_POINT ( 'NONE',  ( 0.2867679344610365999, -0.2867679344610365444, -2.767716535433069946 ) ) ;
#11079=VERTEX_POINT ( 'NONE', #19995 ) ;
#11083=DIRECTION ( 'NONE',  ( 1.000000000000000000, 0.000000000000000000, 0.000000000000000000 ) ) ;
#11084=CARTESIAN_POINT ( 'NONE',  ( -0.3917322834645669549, -0.1049643490035306603, -0.7604986876640419391 ) ) ;
#11085=CARTESIAN_POINT ( 'NONE',  ( -0.4091458600556402980, -0.2362204724409451284, 0.1856955380577427484 ) ) ;
#11087=CARTESIAN_POINT ( 'NONE',  ( 0.2925321140481932369, -0.2925321140481931814, -2.537401574803149984 ) ) ;
#11097=CARTESIAN_POINT ( 'NONE',  ( -0.3460692066303960313, 0.1998031496062989965, -0.5754593175853018883 ) ) ;
#11100=CARTESIAN_POINT ( 'NONE',  ( 0.3392501089628018884, -0.1958661417322834220, -0.2545931758530183275 ) ) ;
#11102=CLOSED_SHELL ( 'NONE', ( #12860, #62457, #37076, #46190, #70542, #41965, #35003, #70263, #56538, #66639, #63049, #23839, #69767, #81565, #42118, #17218, #44095, #74767, #49011, #23364, #46434, #43418, #39387, #3231, #53780, #27008, #73345, #62001, #43832, #63578, #52459, #12985, #49613, #55236, #37297, #48865, #6567, #23820, #42951, #74212, #51683, #19892, #54843, #48134, #20809, #1547, #60902, #223, #57898, #50514 ) ) ;
#11108=CARTESIAN_POINT ( 'NONE',  ( 0.3917322834645668994, 0.1049643490035304522, -1.779508243273278945 ) ) ;
#11117=CARTESIAN_POINT ( 'NONE',  ( 0.1958661417322834775, 0.3392501089628018884, -0.6135363761492932388 ) ) ;
#11121=CARTESIAN_POINT ( 'NONE',  ( 0.4091458600556404646, -0.2362204724409448231, -2.229002624671915900 ) ) ;
#11141=CARTESIAN_POINT ( 'NONE',  ( -0.3996062992125985480, -0.1070741851644057135, -0.04593175853018374027 ) ) ;
#11142=CARTESIAN_POINT ( 'NONE',  ( 0.3996062992125985480, 2.446882876249141654E-17, -2.714566929133858331 ) ) ;
#11148=CARTESIAN_POINT ( 'NONE',  ( -0.1070741851644051862, -0.3996062992125987146, -1.961942257217847763 ) ) ;
#11149=CARTESIAN_POINT ( 'NONE',  ( 0.3949938075777411073, -0.1058382717557499464, -1.371391076115485719 ) ) ;
#11152=CARTESIAN_POINT ( 'NONE',  ( -0.1958661417322836718, 0.3392501089628017219, -0.7926509186351704539 ) ) ;
#11157=CARTESIAN_POINT ( 'NONE',  ( -0.3949938075777411073, 0.1058382717557497660, -2.786745406824147064 ) ) ;
#11161=CARTESIAN_POINT ( 'NONE',  ( 0.4091458600556403535, 0.2362204724409449896, -2.335958005249343827 ) ) ;
#11162=CARTESIAN_POINT ( 'NONE',  ( -0.3996062992125986035, -0.1070741851644056997, -2.250656167979002920 ) ) ;
#11169=CARTESIAN_POINT ( 'NONE',  ( -0.3917322834645668994, -0.1049643490035306742, -2.803130290517373613 ) ) ;
#11177=CARTESIAN_POINT ( 'NONE',  ( -0.2867679344610364334, -0.2867679344610367109, -0.3011811023622048000 ) ) ;
#11178=CARTESIAN_POINT ( 'NONE',  ( 0.1958661417322834775, 0.3392501089628018884, -1.711286089238845287 ) ) ;
#11179=CARTESIAN_POINT ( 'NONE',  ( -0.3917322834645671215, 0.1049643490035301469, -2.229658792650918819 ) ) ;
#11182=CARTESIAN_POINT ( 'NONE',  ( 0.2891555358219910499, 0.2891555358219910499, -2.814960629921259727 ) ) ;
#11186=CARTESIAN_POINT ( 'NONE',  ( -9.787531504996567848E-17, 0.3996062992125986035, -0.9448818897637796255 ) ) ;
#11187=FACE_OUTER_BOUND ( 'NONE', #67586, .T. ) ;
#11191=CARTESIAN_POINT ( 'NONE',  ( 0.1049643490035303689, 0.3917322834645670104, -0.5505249343832020470 ) ) ;
#11192=( BOUNDED_SURFACE ( )  B_SPLINE_SURFACE ( 3, 2, ( 
 ( #54341, #80051, #23184, #42539, #53923, #21953, #29502, #22370, #3427, #42129, #48854, #10576, #2603, #67824, #16900, #10162, #36233, #35828, #61903, #29907, #15655, #9741, #48029, #47196, #61077, #40896, #66577, #8912, #55162, #47611, #74138, #3842, #73730, #41714, #28261, #29090, #80872, #55571, #34587, #73307, #35412, #34999, #74555, #21536, #54760, #28680, #4244, #16068, #66997, #15236, #9329, #60665, #80466, #22776, #74968, #75369, #56404, #6299, #69046, #63962, #24010, #30320, #50491, #31975, #4649, #5884, #17314, #37467, #70273, #76194, #31141, #44580, #56808, #38286, #81279, #5072, #82103, #75782, #11812, #18531, #23595, #37876, #50901, #63140, #49266, #49678, #69462, #36636, #55988, #24416, #12627, #62312, #81699, #17716, #43344, #82507, #24823, #44174, #57214, #11395, #30741, #69867, #18124, #42942, #37052, #62734, #68637, #10976, #50086, #82916, #43756, #5480, #63550, #12219, #31557, #25236, #76601, #18932, #7568, #39542, #46683, #46262, #20186, #27326, #1669, #65657, #58050, #39970, #33240, #13883, #65230, #32387, #39117, #38702, #416, #26072, #8397, #7986, #71535, #64798, #77433, #52986, #58902, #7137, #26499, #1262, #52151, #72376, #77015, #21022, #14725, #78699, #40378, #20610, #51731, #32810, #19347, #44997, #19768, #26910, #45837, #841, #58477, #14310, #25650, #66061, #71957, #77857, #71117, #57635, #51312, #70696, #13049, #52570, #45421, #33650, #16834, #64381, #78278, #6717, #13460, #59313, #60972, #66899, #23084, #54654, #40789, #72783, #53818, #2082, #35310, #27747, #79120, #48751, #3323, #21437, #42026, #10056, #67720, #74450, #79532, #28987, #35719, #60151, #34902, #3738, #61389, #80364, #54235, #34064, #22677, #73628, #53411, #47093, #66474, #16796, #9641, #42433, #15133, #8809, #2503, #48336, #68133, #74033, #9229, #2915, #67306, #28578, #59727, #34485, #80769, #28162, #29402, #21846, #16380, #47510, #41211, #73202, #15552, #60564, #55061, #22265, #79952, #47923, #15970, #41617, #57119, #24730, #30643, #23914, #25137, #4144, #61804, #29809, #82005, #62215, #18439, #76507, #17212, #17618, #18836, #30223, #75275, #37374, #43249, #82813, #31044, #42845, #49163, #55886, #55470, #11718, #81180, #23497, #50806, #63044, #74869, #44081, #69774, #12118, #44481, #81597, #5383, #37776, #36539, #11297, #63451, #5787, #56712, #56308, #10478, #82411, #49989, #68538, #10878, #4553, #36131, #69364, #49579, #68947, #36956, #62633, #50398, #4977, #76095, #43662, #31457, #24319, #75687, #18028, #45739, #7037, #70172, #44892, #25548, #6198, #22054, #19241, #47298, #83227, #32287, #52469, #6616, #76911, #65127, #66686, #26811, #20089, #52051, #60357, #58802, #32707, #41003, #15341, #78177, #70591, #21638, #71435, #26393, #77756, #12945, #51627, #51215, #38603, #64281, #12525, #72987, #736, #77331, #57947, #9021, #314, #19660, #13782, #45322, #2704, #7462, #25968, #71017, #13361, #38186, #39439, #63861, #31876, #28364, #33132, #57536, #34694, #54026, #79737, #39014, #64698, #1160, #58373, #73832, #48546, #17418, #75071, #48962, #67926, #47716, #74662, #3947, #41415, #15763, #54445, #62421, #23291, #30434, #67099, #60766, #16172, #17006, #81803, #42646, #80979, #68343, #23704, #28783, #80572, #10683, #10267, #73414, #22474, #3116, #9430, #35099, #80157, #49375, #48135, #9844, #30016, #67508, #41817, #36338, #43049, #4349, #62012, #29608, #36744, #55680, #35935, #68745, #11087, #81388, #35516, #4758, #56099, #55268, #61179, #3533, #29200, #54866, #22882, #74244, #16586, #42232, #61603, #31252, #43871, #19460, #83024, #56919, #76307, #57330, #18638, #13165, #43458, #70816, #64493, #45110, #38815, #70384, #82210, #82614, #69156, #11507, #69570, #25347, #12326, #50600, #5585, #64078, #75485, #6831, #38399, #44282, #37573, #32500, #17825, #37163, #62843, #37984, #75892, #32085 ),
 ( #76708, #58164, #30843, #57746, #5179, #63659, #24115, #19041, #51009, #49784, #44688, #56508, #24529, #24930, #69972, #6000, #31669, #12740, #50194, #6416, #77126, #108, #18232, #11918, #25762, #63246, #51424, #59016, #72897, #64916, #58591, #26614, #52267, #32926, #7253, #959, #14834, #65766, #1780, #72485, #77972, #20302, #66173, #46375, #46794, #27439, #45951, #71649, #14000, #40494, #40079, #72068, #39658, #59843, #65348, #52684, #1372, #53101, #7685, #78810, #39231, #33353, #53523, #21139, #2195, #77554, #27023, #78392, #27863, #21546, #20723, #14427, #8512, #8098, #33763, #34178, #79231, #47207, #59424, #15248, #40907, #66589, #8924, #34601, #532, #26186, #51847, #19887, #45535, #71233, #13577, #79646, #21963, #47623, #10587, #3023, #29512, #3852, #35422, #80476, #41326, #16495, #36244, #10985, #73319, #15665, #48448, #73742, #55173, #68647, #42139, #41723, #16911, #67417, #35011, #17324, #60266, #80882, #22788, #68252, #42953, #67007, #9750, #2616, #80063, #61087, #23195, #3438, #49276, #48866, #9340, #60675, #22381, #28272, #61506, #53934, #28690, #74979, #74565, #54351, #61913, #4255, #29918, #48040, #16078, #42549, #55581, #29101, #54772, #81292, #23607, #74148, #67834, #10173, #35838, #76205, #30332, #4658, #43356, #51325, #12231, #19361, #55998, #49687, #62747, #63564, #70710, #37888, #69878, #57227, #12639, #17728, #69472, #5898, #56819, #36646, #11405, #75380, #81709, #62321, #69056, #38299, #37062, #82113, #18944, #56414, #5082, #31570, #31988, #76614, #82928, #18543, #25664, #25249, #82517, #6311, #63975, #44592, #30751, #70287, #50914, #44187, #57648, #24427, #18134, #50096, #75792, #43767, #24019, #11, #50502, #11825, #37478, #77029, #45010, #63150, #5491, #31152, #24833, #2095, #32400, #59741, #53425, #8410, #27760, #59326, #71130, #20199, #58063, #430, #58490, #71971, #1275, #39556, #77870, #52999, #64394, #79133, #27341, #33254, #26512, #21450, #6730, #26085, #51745, #26923, #64811, #47107, #77448, #19782, #52583, #52166, #65673, #13062, #78292, #45850, #78712, #71549, #13473, #38716, #45435, #39983, #58916, #39130, #7152, #32823, #13898, #855, #65244, #7582, #20624, #46275, #8000, #14325, #33663, #21037, #1682, #46696, #72389, #14739, #40391, #66074, #34078, #29823, #81196, #79966, #47939, #67321, #3337, #10070, #23511, #29415, #42448, #29001, #72796, #15565, #60988, #28175, #47524, #73642, #61818, #53832, #73215, #41225, #66912, #21859, #79546, #9243, #3751, #54667, #74047, #61402, #34916, #60578, #55074, #35325, #35734, #16395, #2929, #28593, #54250, #80782, #80378, #22691, #22279, #48766, #15984, #41631, #9655, #42041, #48350, #67737, #23098, #74465, #68148, #16812, #10492, #66487, #36146, #4158, #55485, #15146, #40803, #8822, #34499, #60164, #2517, #69789, #50822, #70189, #30239, #44096, #44499, #37791, #63876, #12135, #6215, #57552, #43264, #11733, #24334, #74883, #5397, #68552, #10893, #36553, #82832, #75289, #18453, #76112, #50004, #69379, #55902, #31060, #25154, #81614, #17632, #11311, #63469, #56728, #37388, #68961, #76524, #30659, #18043, #75701, #5803, #56322, #31474, #4568, #36970, #18852, #50412, #12543, #42859, #82021, #43676, #38202, #31891, #23928, #49595, #57135, #63060, #82425, #83243, #49180, #17228, #62650, #62229, #4991, #24745, #40295, #71874, #65976, #33980, #19679, #71451, #752, #51231, #65145, #44910, #70607, #12962, #59227, #51644, #78194, #52486, #26413, #45755, #6631, #7481, #1588, #59641, #38619, #64297, #13799, #39031, #20525, #25565, #33151, #7056, #65570, #32724, #331, #8313, #76930, #46177, #39457, #32303, #19257, #45338, #52066, #57964, #13378, #25985, #77348, #71034, #14223, #64715, #58392, #33565, #77773, #58820, #14639, #39883, #1177, #72293, #26828, #20105, #7904, #27243, #52902, #78616, #20939, #46597 ),
 ( #22182, #1998, #60065, #40704, #21354, #36051, #34397, #61300, #15048, #47424, #67637, #21761, #8727, #80282, #66815, #28905, #34820, #74366, #22595, #2419, #66388, #73115, #53326, #3240, #79035, #47007, #16709, #54567, #72701, #9968, #3658, #35640, #42350, #15467, #48256, #29321, #28076, #2829, #54982, #80690, #73952, #47839, #27660, #16298, #41537, #53734, #79442, #41124, #68048, #60890, #10395, #9148, #60478, #28490, #41941, #54150, #23003, #35226, #48669, #79864, #73545, #15888, #67224, #9556, #61724, #36457, #17131, #81096, #12440, #10797, #37690, #74780, #23830, #43996, #81508, #68459, #56627, #57035, #18353, #11627, #43579, #50724, #50313, #24234, #31370, #5699, #69690, #62131, #12033, #37288, #17943, #69281, #4471, #43167, #42763, #30139, #55802, #4061, #63365, #75604, #68863, #49498, #82730, #62963, #11212, #30559, #5301, #56225, #76422, #23413, #25049, #18751, #44395, #70087, #24646, #75191, #36871, #49080, #17535, #62549, #30960, #49906, #4885, #81923, #29728, #55390, #82327, #76011, #58280, #51540, #52799, #31787, #6115, #57450, #26302, #6534, #46069, #20832, #44806, #45232, #46485, #57861, #13278, #27135, #19155, #12859, #64200, #32204, #70501, #38517, #228, #52377, #19998, #39345, #26723, #25878, #77243, #20417, #645, #1070, #65031, #19573, #70933, #38930, #78085, #77667, #51961, #64610, #14115, #6947, #32618, #45649, #7366, #71344, #33036, #76823, #13691, #7796, #58704, #39768, #83142, #71762, #65463, #33462, #59124, #1481, #78509, #72180, #38100, #63774, #25462, #51129, #35534, #78924, #9447, #9864, #3136, #29218, #60784, #54885, #22897, #8623, #60374, #73007, #40189, #54043, #33873, #59537, #1894, #48155, #40601, #67116, #41433, #15359, #34713, #21246, #79756, #73850, #48565, #27554, #53213, #2722, #27971, #35118, #14538, #22074, #79337, #54464, #21657, #72595, #80590, #65873, #28800, #28383, #46901, #8208, #34294, #41020, #14942, #2310, #66283, #59955, #53629, #80177, #47317, #66706, #22492, #9039, #47733, #3553, #16190, #73431, #61196, #15781, #41837, #67527, #81407, #49395, #68764, #4777, #12651, #442, #32001, #45022, #30453, #74263, #17025, #62440, #29627, #48980, #42249, #10286, #56117, #42664, #23, #58076, #80997, #23724, #26097, #10701, #55699, #17843, #75089, #64407, #38312, #23310, #55287, #36356, #67944, #75504, #35953, #61622, #6742, #44603, #3964, #25676, #51336, #77040, #32414, #62032, #70299, #19372, #68363, #17437, #70723, #13076, #63987, #11108, #16605, #6326, #81823, #74679, #4368, #30036, #43067, #49803, #36764, #24133, #57660, #38730, #78724, #2528, #53011, #1694, #72401, #27772, #32835, #1286, #27352, #71982, #51757, #26525, #7164, #71144, #77460, #867, #53436, #64826, #13911, #34089, #71561, #58503, #46709, #47119, #8421, #21049, #33675, #40815, #40404, #14336, #21461, #79144, #59752, #52179, #2106, #14750, #8011, #59337, #77882, #33268, #20214, #45863, #39568, #19798, #72808, #65684, #58927, #65257, #15157, #66085, #26935, #20635, #66499, #46287, #8833, #13486, #34510, #60175, #45447, #39142, #7594, #52597, #78303, #39996, #47535, #79976, #16405, #54678, #9666, #73653, #29426, #53844, #10502, #55084, #3347, #22289, #61829, #79557, #28603, #67333, #29833, #47950, #4169, #2939, #9255, #10081, #55496, #66923, #80793, #21870, #80390, #36156, #35744, #74059, #28186, #61412, #73226, #15577, #29012, #22701, #42051, #3762, #48776, #41235, #34927, #60589, #23110, #54260, #67747, #42458, #48360, #74475, #16822, #15995, #68158, #41642, #35335, #60999, #52441, #26785, #78152, #34359, #1958, #21314, #8689, #20483, #46137, #2380, #65937, #66350, #46967, #71832, #14181, #65528, #60025, #59603, #8273, #39839, #79404, #1546, #72251, #20900, #72661, #27200, #15009, #58773, #7860, #73077, #40666, #21723, #13758, #52864, #78574, #47386, #41087 ),
 ( #28037, #60441, #28452, #33525, #33938, #46553, #45714, #27620, #39415, #65099, #7436, #53695, #59188, #15426, #66776, #14600, #40254, #1135, #53283, #9109, #54112, #33106, #78994, #34782, #2793, #20061, #71411, #36017, #61264, #36424, #3618, #54529, #36837, #79827, #23378, #42314, #41502, #73505, #3204, #80244, #10764, #61688, #81062, #68424, #28867, #22560, #62097, #68013, #42728, #49046, #48222, #73918, #41905, #4439, #4029, #10357, #16259, #55767, #29284, #48633, #80654, #74743, #54948, #17093, #35190, #67599, #49463, #30105, #81474, #15853, #22967, #74328, #23791, #17502, #9930, #35602, #75157, #16675, #29694, #43134, #68830, #11177, #60851, #62510, #4848, #30523, #22144, #47801, #67187, #9518, #55356, #18720, #31335, #81888, #12408, #75569, #17910, #43546, #6500, #82293, #25429, #83110, #57000, #76387, #37253, #38066, #32170, #6915, #69246, #11593, #44362, #69655, #51094, #64577, #63742, #37653, #12826, #63331, #30926, #13249, #56185, #76792, #70054, #62928, #49870, #50279, #82697, #24199, #43959, #38898, #24612, #5262, #19123, #56593, #75977, #64167, #18317, #6081, #45196, #44772, #31755, #19539, #57417, #11999, #5668, #25016, #50689, #70469, #38483, #57826, #194, #25846, #51506, #77210, #70899, #63589, #38327, #5924, #50940, #6342, #11435, #63177, #31596, #50528, #30359, #5110, #64420, #62776, #32014, #43386, #75821, #12667, #50122, #37090, #25273, #25689, #70312, #57253, #12255, #19386, #18968, #76234, #36, #57674, #64000, #30777, #51350, #82955, #69901, #37912, #56438, #11849, #82141, #24456, #18163, #56028, #77053, #44211, #37502, #43795, #45038, #76637, #5515, #82543, #44617, #24861, #70738, #49716, #13091, #38744, #81736, #24045, #75412, #69500, #31180, #17756, #69087, #56845, #18568, #78319, #33282, #71575, #46722, #58090, #53450, #21062, #26950, #20229, #21475, #455, #26111, #51772, #20650, #58518, #14763, #72824, #13499, #13926, #15174, #26541, #39583, #33690, #65272, #79158, #27365, #39155, #45461, #52194, #77476, #8027, #19812, #71159, #47133, #59351, #64840, #40419, #66100, #8436, #40831, #77898, #1710, #34106, #32849, #7609, #59767, #2122, #53026, #52613, #6755, #78739, #46303, #7178, #882, #45877, #32427, #65697, #58943, #1301, #71997, #14351, #40010, #72414, #27788, #16421, #3779, #42472, #47551, #16010, #42067, #3364, #66516, #41251, #21887, #2542, #29442, #10098, #73243, #9270, #28618, #55101, #22717, #29028, #34941, #68175, #47967, #35351, #67347, #35762, #73668, #61430, #15592, #60604, #36170, #67762, #10516, #60191, #41656, #9680, #61843, #4184, #66938, #2953, #74491, #61013, #48376, #80810, #29847, #55510, #54276, #23125, #81218, #48793, #23534, #16838, #49203, #74905, #79992, #54697, #80405, #8848, #74075, #28200, #53859, #79571, #17253, #22306, #34526, #69810, #18065, #63083, #23948, #82450, #76546, #76955, #4589, #62253, #31083, #56344, #12159, #51253, #24765, #24358, #82857, #50028, #17657, #83267, #42881, #37815, #5421, #30260, #36574, #36993, #55924, #81639, #49616, #50846, #18874, #44523, #31914, #5014, #63491, #70211, #68985, #43699, #12567, #38225, #44118, #56750, #68576, #5825, #50433, #75310, #10917, #43288, #57576, #18476, #25590, #11334, #62673, #30683, #82045, #76135, #63902, #31498, #57157, #6238, #75725, #69403, #25178, #11756, #37411, #77373, #57991, #38643, #53352, #51670, #78641, #32329, #64741, #1611, #39058, #19283, #46204, #58844, #12988, #70631, #26012, #34006, #78219, #2023, #64321, #355, #7079, #32750, #52511, #27267, #20552, #39908, #20964, #19705, #52090, #71898, #39484, #44934, #45363, #71059, #6656, #13403, #58417, #46623, #776, #26438, #52928, #77799, #20131, #14249, #14665, #59254, #65595, #1202, #8340, #7928, #65171, #72319, #40323, #66001, #45779, #59668, #33589, #26852, #27687, #71478, #13825, #7507, #33176 ) ),
 .UNSPECIFIED., .F., .F., .F. ) 
 B_SPLINE_SURFACE_WITH_KNOTS ( ( 4, 4 ),
 ( 3, 2, 2, 2, 2, 2, 2, 2, 2, 2, 2, 2, 2, 2, 2, 2, 2, 2, 2, 2, 2, 2, 2, 2, 2, 2, 2, 2, 2, 2, 2, 2, 2, 2, 2, 2, 2, 2, 2, 2, 2, 2, 2, 2, 2, 2, 2, 2, 2, 2, 2, 2, 2, 2, 2, 2, 2, 2, 2, 2, 2, 2, 2, 2, 2, 2, 2, 2, 2, 2, 2, 2, 2, 2, 2, 2, 2, 2, 2, 2, 2, 2, 2, 2, 2, 2, 2, 2, 2, 2, 2, 2, 2, 2, 2, 2, 2, 2, 2, 2, 2, 2, 2, 2, 2, 2, 2, 2, 2, 2, 2, 2, 2, 2, 2, 2, 2, 2, 2, 2, 2, 2, 2, 2, 2, 2, 2, 2, 2, 2, 2, 2, 2, 2, 2, 2, 2, 2, 2, 2, 2, 2, 2, 2, 2, 2, 2, 2, 2, 2, 2, 2, 2, 2, 2, 2, 2, 2, 2, 2, 2, 2, 2, 2, 2, 2, 2, 2, 2, 2, 2, 2, 2, 2, 2, 2, 2, 2, 2, 2, 2, 2, 2, 2, 2, 2, 2, 2, 2, 2, 2, 2, 2, 2, 2, 2, 2, 2, 2, 2, 2, 2, 2, 2, 2, 2, 2, 2, 2, 2, 2, 2, 2, 2, 2, 2, 2, 2, 2, 2, 2, 2, 2, 2, 2, 2, 2, 2, 2, 2, 2, 2, 2, 2, 2, 2, 2, 3 ),
 ( 0.000000000000000000, 1.000000000000000000 ),
 ( 0.000000000000000000, 0.004166666666666666609, 0.008333333333333333218, 0.01250000000000000069, 0.01666666666666666644, 0.02083333333333333218, 0.02500000000000000139, 0.02916666666666666713, 0.03333333333333333287, 0.03749999999999999861, 0.04166666666666666435, 0.04583333333333333010, 0.05000000000000000278, 0.05416666666666666852, 0.05833333333333333426, 0.06250000000000000000, 0.06666666666666666574, 0.07083333333333333148, 0.07499999999999999722, 0.07916666666666666297, 0.08333333333333332871, 0.08749999999999999445, 0.09166666666666666019, 0.09583333333333333981, 0.1000000000000000056, 0.1041666666666666713, 0.1083333333333333370, 0.1125000000000000028, 0.1166666666666666685, 0.1208333333333333343, 0.1250000000000000000, 0.1291666666666666796, 0.1333333333333333315, 0.1375000000000000111, 0.1416666666666666630, 0.1458333333333333426, 0.1499999999999999944, 0.1541666666666666741, 0.1583333333333333259, 0.1625000000000000056, 0.1666666666666666574, 0.1708333333333333370, 0.1749999999999999889, 0.1791666666666666685, 0.1833333333333333204, 0.1875000000000000000, 0.1916666666666666796, 0.1958333333333333315, 0.2000000000000000111, 0.2041666666666666630, 0.2083333333333333426, 0.2124999999999999944, 0.2166666666666666741, 0.2208333333333333259, 0.2250000000000000056, 0.2291666666666666574, 0.2333333333333333370, 0.2374999999999999889, 0.2416666666666666685, 0.2458333333333333204, 0.2500000000000000000, 0.2541666666666666519, 0.2583333333333333592, 0.2625000000000000111, 0.2666666666666666630, 0.2708333333333333148, 0.2750000000000000222, 0.2791666666666666741, 0.2833333333333333259, 0.2874999999999999778, 0.2916666666666666852, 0.2958333333333333370, 0.2999999999999999889, 0.3041666666666666408, 0.3083333333333333481, 0.3125000000000000000, 0.3166666666666666519, 0.3208333333333333592, 0.3250000000000000111, 0.3291666666666666630, 0.3333333333333333148, 0.3375000000000000222, 0.3416666666666666741, 0.3458333333333333259, 0.3499999999999999778, 0.3541666666666666852, 0.3583333333333333370, 0.3624999999999999889, 0.3666666666666666408, 0.3708333333333333481, 0.3750000000000000000, 0.3791666666666666519, 0.3833333333333333592, 0.3875000000000000111, 0.3916666666666666630, 0.3958333333333333148, 0.4000000000000000222, 0.4041666666666666741, 0.4083333333333333259, 0.4124999999999999778, 0.4166666666666666852, 0.4208333333333333370, 0.4249999999999999889, 0.4291666666666666408, 0.4333333333333333481, 0.4375000000000000000, 0.4416666666666666519, 0.4458333333333333592, 0.4500000000000000111, 0.4541666666666666630, 0.4583333333333333148, 0.4625000000000000222, 0.4666666666666666741, 0.4708333333333333259, 0.4749999999999999778, 0.4791666666666666852, 0.4833333333333333370, 0.4874999999999999889, 0.4916666666666666408, 0.4958333333333333481, 0.5000000000000000000, 0.5041666666666666519, 0.5083333333333333037, 0.5124999999999999556, 0.5166666666666667185, 0.5208333333333333703, 0.5250000000000000222, 0.5291666666666666741, 0.5333333333333333259, 0.5374999999999999778, 0.5416666666666666297, 0.5458333333333332815, 0.5500000000000000444, 0.5541666666666666963, 0.5583333333333333481, 0.5625000000000000000, 0.5666666666666666519, 0.5708333333333333037, 0.5749999999999999556, 0.5791666666666667185, 0.5833333333333333703, 0.5875000000000000222, 0.5916666666666666741, 0.5958333333333333259, 0.5999999999999999778, 0.6041666666666666297, 0.6083333333333332815, 0.6125000000000000444, 0.6166666666666666963, 0.6208333333333333481, 0.6250000000000000000, 0.6291666666666666519, 0.6333333333333333037, 0.6374999999999999556, 0.6416666666666667185, 0.6458333333333333703, 0.6500000000000000222, 0.6541666666666666741, 0.6583333333333333259, 0.6624999999999999778, 0.6666666666666666297, 0.6708333333333332815, 0.6750000000000000444, 0.6791666666666666963, 0.6833333333333333481, 0.6875000000000000000, 0.6916666666666666519, 0.6958333333333333037, 0.6999999999999999556, 0.7041666666666667185, 0.7083333333333333703, 0.7125000000000000222, 0.7166666666666666741, 0.7208333333333333259, 0.7249999999999999778, 0.7291666666666666297, 0.7333333333333332815, 0.7375000000000000444, 0.7416666666666666963, 0.7458333333333333481, 0.7500000000000000000, 0.7541666666666666519, 0.7583333333333333037, 0.7624999999999999556, 0.7666666666666667185, 0.7708333333333333703, 0.7750000000000000222, 0.7791666666666666741, 0.7833333333333333259, 0.7874999999999999778, 0.7916666666666666297, 0.7958333333333332815, 0.8000000000000000444, 0.8041666666666666963, 0.8083333333333333481, 0.8125000000000000000, 0.8166666666666666519, 0.8208333333333333037, 0.8249999999999999556, 0.8291666666666667185, 0.8333333333333333703, 0.8375000000000000222, 0.8416666666666666741, 0.8458333333333333259, 0.8499999999999999778, 0.8541666666666666297, 0.8583333333333332815, 0.8625000000000000444, 0.8666666666666666963, 0.8708333333333333481, 0.8750000000000000000, 0.8791666666666666519, 0.8833333333333333037, 0.8874999999999999556, 0.8916666666666667185, 0.8958333333333333703, 0.9000000000000000222, 0.9041666666666666741, 0.9083333333333333259, 0.9124999999999999778, 0.9166666666666666297, 0.9208333333333332815, 0.9250000000000000444, 0.9291666666666666963, 0.9333333333333333481, 0.9375000000000000000, 0.9416666666666666519, 0.9458333333333333037, 0.9499999999999999556, 0.9541666666666667185, 0.9583333333333333703, 0.9625000000000000222, 0.9666666666666666741, 0.9708333333333333259, 0.9749999999999999778, 0.9791666666666666297, 0.9833333333333332815, 0.9875000000000000444 ),
 .UNSPECIFIED. ) 
 GEOMETRIC_REPRESENTATION_ITEM ( )  RATIONAL_B_SPLINE_SURFACE ( (
 ( 1.000000000000000000, 0.9659258262890683122, 1.000000000000000000, 0.9659258262890683122, 1.000000000000000000, 0.9659258262890683122, 1.000000000000000000, 0.9659258262890683122, 1.000000000000000000, 0.9659258262890683122, 1.000000000000000000, 0.9659258262890683122, 1.000000000000000000, 0.9659258262890683122, 1.000000000000000000, 0.9659258262890683122, 1.000000000000000000, 0.9659258262890683122, 1.000000000000000000, 0.9659258262890683122, 1.000000000000000000, 0.9659258262890683122, 1.000000000000000000, 0.9659258262890683122, 1.000000000000000000, 0.9659258262890683122, 1.000000000000000000, 0.9659258262890683122, 1.000000000000000000, 0.9659258262890683122, 1.000000000000000000, 0.9659258262890683122, 1.000000000000000000, 0.9659258262890683122, 1.000000000000000000, 0.9659258262890683122, 1.000000000000000000, 0.9659258262890683122, 1.000000000000000000, 0.9659258262890683122, 1.000000000000000000, 0.9659258262890683122, 1.000000000000000000, 0.9659258262890683122, 1.000000000000000000, 0.9659258262890683122, 1.000000000000000000, 0.9659258262890683122, 1.000000000000000000, 0.9659258262890683122, 1.000000000000000000, 0.9659258262890683122, 1.000000000000000000, 0.9659258262890683122, 1.000000000000000000, 0.9659258262890683122, 1.000000000000000000, 0.9659258262890683122, 1.000000000000000000, 0.9659258262890683122, 1.000000000000000000, 0.9659258262890683122, 1.000000000000000000, 0.9659258262890683122, 1.000000000000000000, 0.9659258262890683122, 1.000000000000000000, 0.9659258262890683122, 1.000000000000000000, 0.9659258262890683122, 1.000000000000000000, 0.9659258262890683122, 1.000000000000000000, 0.9659258262890683122, 1.000000000000000000, 0.9659258262890683122, 1.000000000000000000, 0.9659258262890683122, 1.000000000000000000, 0.9659258262890683122, 1.000000000000000000, 0.9659258262890683122, 1.000000000000000000, 0.9659258262890683122, 1.000000000000000000, 0.9659258262890683122, 1.000000000000000000, 0.9659258262890683122, 1.000000000000000000, 0.9659258262890683122, 1.000000000000000000, 0.9659258262890683122, 1.000000000000000000, 0.9659258262890683122, 1.000000000000000000, 0.9659258262890683122, 1.000000000000000000, 0.9659258262890683122, 1.000000000000000000, 0.9659258262890683122, 1.000000000000000000, 0.9659258262890683122, 1.000000000000000000, 0.9659258262890683122, 1.000000000000000000, 0.9659258262890683122, 1.000000000000000000, 0.9659258262890683122, 1.000000000000000000, 0.9659258262890683122, 1.000000000000000000, 0.9659258262890683122, 1.000000000000000000, 0.9659258262890683122, 1.000000000000000000, 0.9659258262890683122, 1.000000000000000000, 0.9659258262890683122, 1.000000000000000000, 0.9659258262890683122, 1.000000000000000000, 0.9659258262890683122, 1.000000000000000000, 0.9659258262890683122, 1.000000000000000000, 0.9659258262890683122, 1.000000000000000000, 0.9659258262890683122, 1.000000000000000000, 0.9659258262890683122, 1.000000000000000000, 0.9659258262890683122, 1.000000000000000000, 0.9659258262890683122, 1.000000000000000000, 0.9659258262890683122, 1.000000000000000000, 0.9659258262890683122, 1.000000000000000000, 0.9659258262890683122, 1.000000000000000000, 0.9659258262890683122, 1.000000000000000000, 0.9659258262890683122, 1.000000000000000000, 0.9659258262890683122, 1.000000000000000000, 0.9659258262890683122, 1.000000000000000000, 0.9659258262890683122, 1.000000000000000000, 0.9659258262890683122, 1.000000000000000000, 0.9659258262890683122, 1.000000000000000000, 0.9659258262890683122, 1.000000000000000000, 0.9659258262890683122, 1.000000000000000000, 0.9659258262890683122, 1.000000000000000000, 0.9659258262890683122, 1.000000000000000000, 0.9659258262890683122, 1.000000000000000000, 0.9659258262890683122, 1.000000000000000000, 0.9659258262890683122, 1.000000000000000000, 0.9659258262890683122, 1.000000000000000000, 0.9659258262890683122, 1.000000000000000000, 0.9659258262890683122, 1.000000000000000000, 0.9659258262890683122, 1.000000000000000000, 0.9659258262890683122, 1.000000000000000000, 0.9659258262890683122, 1.000000000000000000, 0.9659258262890683122, 1.000000000000000000, 0.9659258262890683122, 1.000000000000000000, 0.9659258262890683122, 1.000000000000000000, 0.9659258262890683122, 1.000000000000000000, 0.9659258262890683122, 1.000000000000000000, 0.9659258262890683122, 1.000000000000000000, 0.9659258262890683122, 1.000000000000000000, 0.9659258262890683122, 1.000000000000000000, 0.9659258262890683122, 1.000000000000000000, 0.9659258262890683122, 1.000000000000000000, 0.9659258262890683122, 1.000000000000000000, 0.9659258262890683122, 1.000000000000000000, 0.9659258262890683122, 1.000000000000000000, 0.9659258262890683122, 1.000000000000000000, 0.9659258262890683122, 1.000000000000000000, 0.9659258262890683122, 1.000000000000000000, 0.9659258262890683122, 1.000000000000000000, 0.9659258262890683122, 1.000000000000000000, 0.9659258262890683122, 1.000000000000000000, 0.9659258262890683122, 1.000000000000000000, 0.9659258262890683122, 1.000000000000000000, 0.9659258262890683122, 1.000000000000000000, 0.9659258262890683122, 1.000000000000000000, 0.9659258262890683122, 1.000000000000000000, 0.9659258262890683122, 1.000000000000000000, 0.9659258262890683122, 1.000000000000000000, 0.9659258262890683122, 1.000000000000000000, 0.9659258262890683122, 1.000000000000000000, 0.9659258262890683122, 1.000000000000000000, 0.9659258262890683122, 1.000000000000000000, 0.9659258262890683122, 1.000000000000000000, 0.9659258262890683122, 1.000000000000000000, 0.9659258262890683122, 1.000000000000000000, 0.9659258262890683122, 1.000000000000000000, 0.9659258262890683122, 1.000000000000000000, 0.9659258262890683122, 1.000000000000000000, 0.9659258262890683122, 1.000000000000000000, 0.9659258262890683122, 1.000000000000000000, 0.9659258262890683122, 1.000000000000000000, 0.9659258262890683122, 1.000000000000000000, 0.9659258262890683122, 1.000000000000000000, 0.9659258262890683122, 1.000000000000000000, 0.9659258262890683122, 1.000000000000000000, 0.9659258262890683122, 1.000000000000000000, 0.9659258262890683122, 1.000000000000000000, 0.9659258262890683122, 1.000000000000000000, 0.9659258262890683122, 1.000000000000000000, 0.9659258262890683122, 1.000000000000000000, 0.9659258262890683122, 1.000000000000000000, 0.9659258262890683122, 1.000000000000000000, 0.9659258262890683122, 1.000000000000000000, 0.9659258262890683122, 1.000000000000000000, 0.9659258262890683122, 1.000000000000000000, 0.9659258262890683122, 1.000000000000000000, 0.9659258262890683122, 1.000000000000000000, 0.9659258262890683122, 1.000000000000000000, 0.9659258262890683122, 1.000000000000000000, 0.9659258262890683122, 1.000000000000000000, 0.9659258262890683122, 1.000000000000000000, 0.9659258262890683122, 1.000000000000000000, 0.9659258262890683122, 1.000000000000000000, 0.9659258262890683122, 1.000000000000000000, 0.9659258262890683122, 1.000000000000000000, 0.9659258262890683122, 1.000000000000000000, 0.9659258262890683122, 1.000000000000000000, 0.9659258262890683122, 1.000000000000000000, 0.9659258262890683122, 1.000000000000000000, 0.9659258262890683122, 1.000000000000000000, 0.9659258262890683122, 1.000000000000000000, 0.9659258262890683122, 1.000000000000000000, 0.9659258262890683122, 1.000000000000000000, 0.9659258262890683122, 1.000000000000000000, 0.9659258262890683122, 1.000000000000000000, 0.9659258262890683122, 1.000000000000000000, 0.9659258262890683122, 1.000000000000000000, 0.9659258262890683122, 1.000000000000000000, 0.9659258262890683122, 1.000000000000000000, 0.9659258262890683122, 1.000000000000000000, 0.9659258262890683122, 1.000000000000000000, 0.9659258262890683122, 1.000000000000000000, 0.9659258262890683122, 1.000000000000000000, 0.9659258262890683122, 1.000000000000000000, 0.9659258262890683122, 1.000000000000000000, 0.9659258262890683122, 1.000000000000000000, 0.9659258262890683122, 1.000000000000000000, 0.9659258262890683122, 1.000000000000000000, 0.9659258262890683122, 1.000000000000000000, 0.9659258262890683122, 1.000000000000000000, 0.9659258262890683122, 1.000000000000000000, 0.9659258262890683122, 1.000000000000000000, 0.9659258262890683122, 1.000000000000000000, 0.9659258262890683122, 1.000000000000000000, 0.9659258262890683122, 1.000000000000000000, 0.9659258262890683122, 1.000000000000000000, 0.9659258262890683122, 1.000000000000000000, 0.9659258262890683122, 1.000000000000000000, 0.9659258262890683122, 1.000000000000000000, 0.9659258262890683122, 1.000000000000000000, 0.9659258262890683122, 1.000000000000000000, 0.9659258262890683122, 1.000000000000000000, 0.9659258262890683122, 1.000000000000000000, 0.9659258262890683122, 1.000000000000000000, 0.9659258262890683122, 1.000000000000000000, 0.9659258262890683122, 1.000000000000000000, 0.9659258262890683122, 1.000000000000000000, 0.9659258262890683122, 1.000000000000000000, 0.9659258262890683122, 1.000000000000000000, 0.9659258262890683122, 1.000000000000000000, 0.9659258262890683122, 1.000000000000000000, 0.9659258262890683122, 1.000000000000000000, 0.9659258262890683122, 1.000000000000000000, 0.9659258262890683122, 1.000000000000000000, 0.9659258262890683122, 1.000000000000000000, 0.9659258262890683122, 1.000000000000000000, 0.9659258262890683122, 1.000000000000000000, 0.9659258262890683122, 1.000000000000000000, 0.9659258262890683122, 1.000000000000000000, 0.9659258262890683122, 1.000000000000000000, 0.9659258262890683122, 1.000000000000000000, 0.9659258262890683122, 1.000000000000000000, 0.9659258262890683122, 1.000000000000000000, 0.9659258262890683122, 1.000000000000000000, 0.9659258262890683122, 1.000000000000000000, 0.9659258262890683122, 1.000000000000000000, 0.9659258262890683122, 1.000000000000000000, 0.9659258262890683122, 1.000000000000000000, 0.9659258262890683122, 1.000000000000000000, 0.9659258262890683122, 1.000000000000000000, 0.9659258262890683122, 1.000000000000000000, 0.9659258262890683122, 1.000000000000000000, 0.9659258262890683122, 1.000000000000000000, 0.9659258262890683122, 1.000000000000000000, 0.9659258262890683122, 1.000000000000000000, 0.9659258262890683122, 1.000000000000000000, 0.9659258262890683122, 1.000000000000000000, 0.9659258262890683122, 1.000000000000000000, 0.9659258262890683122, 1.000000000000000000, 0.9659258262890683122, 1.000000000000000000, 0.9659258262890683122, 1.000000000000000000, 0.9659258262890683122, 1.000000000000000000, 0.9659258262890683122, 1.000000000000000000, 0.9659258262890683122, 1.000000000000000000, 0.9659258262890683122, 1.000000000000000000, 0.9659258262890683122, 1.000000000000000000, 0.9659258262890683122, 1.000000000000000000, 0.9659258262890683122, 1.000000000000000000, 0.9659258262890683122, 1.000000000000000000),
 ( 0.8047378541243631611, 0.7773170766911672303, 0.8047378541243631611, 0.7773170766911672303, 0.8047378541243631611, 0.7773170766911672303, 0.8047378541243631611, 0.7773170766911672303, 0.8047378541243631611, 0.7773170766911672303, 0.8047378541243631611, 0.7773170766911672303, 0.8047378541243631611, 0.7773170766911672303, 0.8047378541243631611, 0.7773170766911672303, 0.8047378541243631611, 0.7773170766911672303, 0.8047378541243631611, 0.7773170766911672303, 0.8047378541243631611, 0.7773170766911672303, 0.8047378541243631611, 0.7773170766911672303, 0.8047378541243631611, 0.7773170766911672303, 0.8047378541243631611, 0.7773170766911672303, 0.8047378541243631611, 0.7773170766911672303, 0.8047378541243631611, 0.7773170766911672303, 0.8047378541243631611, 0.7773170766911672303, 0.8047378541243631611, 0.7773170766911672303, 0.8047378541243631611, 0.7773170766911672303, 0.8047378541243631611, 0.7773170766911672303, 0.8047378541243631611, 0.7773170766911672303, 0.8047378541243631611, 0.7773170766911672303, 0.8047378541243631611, 0.7773170766911672303, 0.8047378541243631611, 0.7773170766911672303, 0.8047378541243631611, 0.7773170766911672303, 0.8047378541243631611, 0.7773170766911672303, 0.8047378541243631611, 0.7773170766911672303, 0.8047378541243631611, 0.7773170766911672303, 0.8047378541243631611, 0.7773170766911672303, 0.8047378541243631611, 0.7773170766911672303, 0.8047378541243631611, 0.7773170766911672303, 0.8047378541243631611, 0.7773170766911672303, 0.8047378541243631611, 0.7773170766911672303, 0.8047378541243631611, 0.7773170766911672303, 0.8047378541243631611, 0.7773170766911672303, 0.8047378541243631611, 0.7773170766911672303, 0.8047378541243631611, 0.7773170766911672303, 0.8047378541243631611, 0.7773170766911672303, 0.8047378541243631611, 0.7773170766911672303, 0.8047378541243631611, 0.7773170766911672303, 0.8047378541243631611, 0.7773170766911672303, 0.8047378541243631611, 0.7773170766911672303, 0.8047378541243631611, 0.7773170766911672303, 0.8047378541243631611, 0.7773170766911672303, 0.8047378541243631611, 0.7773170766911672303, 0.8047378541243631611, 0.7773170766911672303, 0.8047378541243631611, 0.7773170766911672303, 0.8047378541243631611, 0.7773170766911672303, 0.8047378541243631611, 0.7773170766911672303, 0.8047378541243631611, 0.7773170766911672303, 0.8047378541243631611, 0.7773170766911672303, 0.8047378541243631611, 0.7773170766911672303, 0.8047378541243631611, 0.7773170766911672303, 0.8047378541243631611, 0.7773170766911672303, 0.8047378541243631611, 0.7773170766911672303, 0.8047378541243631611, 0.7773170766911672303, 0.8047378541243631611, 0.7773170766911672303, 0.8047378541243631611, 0.7773170766911672303, 0.8047378541243631611, 0.7773170766911672303, 0.8047378541243631611, 0.7773170766911672303, 0.8047378541243631611, 0.7773170766911672303, 0.8047378541243631611, 0.7773170766911672303, 0.8047378541243631611, 0.7773170766911672303, 0.8047378541243631611, 0.7773170766911672303, 0.8047378541243631611, 0.7773170766911672303, 0.8047378541243631611, 0.7773170766911672303, 0.8047378541243631611, 0.7773170766911672303, 0.8047378541243631611, 0.7773170766911672303, 0.8047378541243631611, 0.7773170766911672303, 0.8047378541243631611, 0.7773170766911672303, 0.8047378541243631611, 0.7773170766911672303, 0.8047378541243631611, 0.7773170766911672303, 0.8047378541243631611, 0.7773170766911672303, 0.8047378541243631611, 0.7773170766911672303, 0.8047378541243631611, 0.7773170766911672303, 0.8047378541243631611, 0.7773170766911672303, 0.8047378541243631611, 0.7773170766911672303, 0.8047378541243631611, 0.7773170766911672303, 0.8047378541243631611, 0.7773170766911672303, 0.8047378541243631611, 0.7773170766911672303, 0.8047378541243631611, 0.7773170766911672303, 0.8047378541243631611, 0.7773170766911672303, 0.8047378541243631611, 0.7773170766911672303, 0.8047378541243631611, 0.7773170766911672303, 0.8047378541243631611, 0.7773170766911672303, 0.8047378541243631611, 0.7773170766911672303, 0.8047378541243631611, 0.7773170766911672303, 0.8047378541243631611, 0.7773170766911672303, 0.8047378541243631611, 0.7773170766911672303, 0.8047378541243631611, 0.7773170766911672303, 0.8047378541243631611, 0.7773170766911672303, 0.8047378541243631611, 0.7773170766911672303, 0.8047378541243631611, 0.7773170766911672303, 0.8047378541243631611, 0.7773170766911672303, 0.8047378541243631611, 0.7773170766911672303, 0.8047378541243631611, 0.7773170766911672303, 0.8047378541243631611, 0.7773170766911672303, 0.8047378541243631611, 0.7773170766911672303, 0.8047378541243631611, 0.7773170766911672303, 0.8047378541243631611, 0.7773170766911672303, 0.8047378541243631611, 0.7773170766911672303, 0.8047378541243631611, 0.7773170766911672303, 0.8047378541243631611, 0.7773170766911672303, 0.8047378541243631611, 0.7773170766911672303, 0.8047378541243631611, 0.7773170766911672303, 0.8047378541243631611, 0.7773170766911672303, 0.8047378541243631611, 0.7773170766911672303, 0.8047378541243631611, 0.7773170766911672303, 0.8047378541243631611, 0.7773170766911672303, 0.8047378541243631611, 0.7773170766911672303, 0.8047378541243631611, 0.7773170766911672303, 0.8047378541243631611, 0.7773170766911672303, 0.8047378541243631611, 0.7773170766911672303, 0.8047378541243631611, 0.7773170766911672303, 0.8047378541243631611, 0.7773170766911672303, 0.8047378541243631611, 0.7773170766911672303, 0.8047378541243631611, 0.7773170766911672303, 0.8047378541243631611, 0.7773170766911672303, 0.8047378541243631611, 0.7773170766911672303, 0.8047378541243631611, 0.7773170766911672303, 0.8047378541243631611, 0.7773170766911672303, 0.8047378541243631611, 0.7773170766911672303, 0.8047378541243631611, 0.7773170766911672303, 0.8047378541243631611, 0.7773170766911672303, 0.8047378541243631611, 0.7773170766911672303, 0.8047378541243631611, 0.7773170766911672303, 0.8047378541243631611, 0.7773170766911672303, 0.8047378541243631611, 0.7773170766911672303, 0.8047378541243631611, 0.7773170766911672303, 0.8047378541243631611, 0.7773170766911672303, 0.8047378541243631611, 0.7773170766911672303, 0.8047378541243631611, 0.7773170766911672303, 0.8047378541243631611, 0.7773170766911672303, 0.8047378541243631611, 0.7773170766911672303, 0.8047378541243631611, 0.7773170766911672303, 0.8047378541243631611, 0.7773170766911672303, 0.8047378541243631611, 0.7773170766911672303, 0.8047378541243631611, 0.7773170766911672303, 0.8047378541243631611, 0.7773170766911672303, 0.8047378541243631611, 0.7773170766911672303, 0.8047378541243631611, 0.7773170766911672303, 0.8047378541243631611, 0.7773170766911672303, 0.8047378541243631611, 0.7773170766911672303, 0.8047378541243631611, 0.7773170766911672303, 0.8047378541243631611, 0.7773170766911672303, 0.8047378541243631611, 0.7773170766911672303, 0.8047378541243631611, 0.7773170766911672303, 0.8047378541243631611, 0.7773170766911672303, 0.8047378541243631611, 0.7773170766911672303, 0.8047378541243631611, 0.7773170766911672303, 0.8047378541243631611, 0.7773170766911672303, 0.8047378541243631611, 0.7773170766911672303, 0.8047378541243631611, 0.7773170766911672303, 0.8047378541243631611, 0.7773170766911672303, 0.8047378541243631611, 0.7773170766911672303, 0.8047378541243631611, 0.7773170766911672303, 0.8047378541243631611, 0.7773170766911672303, 0.8047378541243631611, 0.7773170766911672303, 0.8047378541243631611, 0.7773170766911672303, 0.8047378541243631611, 0.7773170766911672303, 0.8047378541243631611, 0.7773170766911672303, 0.8047378541243631611, 0.7773170766911672303, 0.8047378541243631611, 0.7773170766911672303, 0.8047378541243631611, 0.7773170766911672303, 0.8047378541243631611, 0.7773170766911672303, 0.8047378541243631611, 0.7773170766911672303, 0.8047378541243631611, 0.7773170766911672303, 0.8047378541243631611, 0.7773170766911672303, 0.8047378541243631611, 0.7773170766911672303, 0.8047378541243631611, 0.7773170766911672303, 0.8047378541243631611, 0.7773170766911672303, 0.8047378541243631611, 0.7773170766911672303, 0.8047378541243631611, 0.7773170766911672303, 0.8047378541243631611, 0.7773170766911672303, 0.8047378541243631611, 0.7773170766911672303, 0.8047378541243631611, 0.7773170766911672303, 0.8047378541243631611, 0.7773170766911672303, 0.8047378541243631611, 0.7773170766911672303, 0.8047378541243631611, 0.7773170766911672303, 0.8047378541243631611, 0.7773170766911672303, 0.8047378541243631611, 0.7773170766911672303, 0.8047378541243631611, 0.7773170766911672303, 0.8047378541243631611, 0.7773170766911672303, 0.8047378541243631611, 0.7773170766911672303, 0.8047378541243631611, 0.7773170766911672303, 0.8047378541243631611, 0.7773170766911672303, 0.8047378541243631611, 0.7773170766911672303, 0.8047378541243631611, 0.7773170766911672303, 0.8047378541243631611, 0.7773170766911672303, 0.8047378541243631611, 0.7773170766911672303, 0.8047378541243631611, 0.7773170766911672303, 0.8047378541243631611, 0.7773170766911672303, 0.8047378541243631611, 0.7773170766911672303, 0.8047378541243631611, 0.7773170766911672303, 0.8047378541243631611, 0.7773170766911672303, 0.8047378541243631611, 0.7773170766911672303, 0.8047378541243631611, 0.7773170766911672303, 0.8047378541243631611, 0.7773170766911672303, 0.8047378541243631611, 0.7773170766911672303, 0.8047378541243631611, 0.7773170766911672303, 0.8047378541243631611, 0.7773170766911672303, 0.8047378541243631611, 0.7773170766911672303, 0.8047378541243631611, 0.7773170766911672303, 0.8047378541243631611, 0.7773170766911672303, 0.8047378541243631611, 0.7773170766911672303, 0.8047378541243631611, 0.7773170766911672303, 0.8047378541243631611, 0.7773170766911672303, 0.8047378541243631611, 0.7773170766911672303, 0.8047378541243631611, 0.7773170766911672303, 0.8047378541243631611, 0.7773170766911672303, 0.8047378541243631611, 0.7773170766911672303, 0.8047378541243631611, 0.7773170766911672303, 0.8047378541243631611, 0.7773170766911672303, 0.8047378541243631611, 0.7773170766911672303, 0.8047378541243631611, 0.7773170766911672303, 0.8047378541243631611, 0.7773170766911672303, 0.8047378541243631611, 0.7773170766911672303, 0.8047378541243631611, 0.7773170766911672303, 0.8047378541243631611, 0.7773170766911672303, 0.8047378541243631611, 0.7773170766911672303, 0.8047378541243631611, 0.7773170766911672303, 0.8047378541243631611, 0.7773170766911672303, 0.8047378541243631611, 0.7773170766911672303, 0.8047378541243631611, 0.7773170766911672303, 0.8047378541243631611, 0.7773170766911672303, 0.8047378541243631611, 0.7773170766911672303, 0.8047378541243631611, 0.7773170766911672303, 0.8047378541243631611, 0.7773170766911672303, 0.8047378541243631611, 0.7773170766911672303, 0.8047378541243631611, 0.7773170766911672303, 0.8047378541243631611, 0.7773170766911672303, 0.8047378541243631611, 0.7773170766911672303, 0.8047378541243631611, 0.7773170766911672303, 0.8047378541243631611, 0.7773170766911672303, 0.8047378541243631611, 0.7773170766911672303, 0.8047378541243631611, 0.7773170766911672303, 0.8047378541243631611, 0.7773170766911672303, 0.8047378541243631611),
 ( 0.8047378541243631611, 0.7773170766911672303, 0.8047378541243631611, 0.7773170766911672303, 0.8047378541243631611, 0.7773170766911672303, 0.8047378541243631611, 0.7773170766911672303, 0.8047378541243631611, 0.7773170766911672303, 0.8047378541243631611, 0.7773170766911672303, 0.8047378541243631611, 0.7773170766911672303, 0.8047378541243631611, 0.7773170766911672303, 0.8047378541243631611, 0.7773170766911672303, 0.8047378541243631611, 0.7773170766911672303, 0.8047378541243631611, 0.7773170766911672303, 0.8047378541243631611, 0.7773170766911672303, 0.8047378541243631611, 0.7773170766911672303, 0.8047378541243631611, 0.7773170766911672303, 0.8047378541243631611, 0.7773170766911672303, 0.8047378541243631611, 0.7773170766911672303, 0.8047378541243631611, 0.7773170766911672303, 0.8047378541243631611, 0.7773170766911672303, 0.8047378541243631611, 0.7773170766911672303, 0.8047378541243631611, 0.7773170766911672303, 0.8047378541243631611, 0.7773170766911672303, 0.8047378541243631611, 0.7773170766911672303, 0.8047378541243631611, 0.7773170766911672303, 0.8047378541243631611, 0.7773170766911672303, 0.8047378541243631611, 0.7773170766911672303, 0.8047378541243631611, 0.7773170766911672303, 0.8047378541243631611, 0.7773170766911672303, 0.8047378541243631611, 0.7773170766911672303, 0.8047378541243631611, 0.7773170766911672303, 0.8047378541243631611, 0.7773170766911672303, 0.8047378541243631611, 0.7773170766911672303, 0.8047378541243631611, 0.7773170766911672303, 0.8047378541243631611, 0.7773170766911672303, 0.8047378541243631611, 0.7773170766911672303, 0.8047378541243631611, 0.7773170766911672303, 0.8047378541243631611, 0.7773170766911672303, 0.8047378541243631611, 0.7773170766911672303, 0.8047378541243631611, 0.7773170766911672303, 0.8047378541243631611, 0.7773170766911672303, 0.8047378541243631611, 0.7773170766911672303, 0.8047378541243631611, 0.7773170766911672303, 0.8047378541243631611, 0.7773170766911672303, 0.8047378541243631611, 0.7773170766911672303, 0.8047378541243631611, 0.7773170766911672303, 0.8047378541243631611, 0.7773170766911672303, 0.8047378541243631611, 0.7773170766911672303, 0.8047378541243631611, 0.7773170766911672303, 0.8047378541243631611, 0.7773170766911672303, 0.8047378541243631611, 0.7773170766911672303, 0.8047378541243631611, 0.7773170766911672303, 0.8047378541243631611, 0.7773170766911672303, 0.8047378541243631611, 0.7773170766911672303, 0.8047378541243631611, 0.7773170766911672303, 0.8047378541243631611, 0.7773170766911672303, 0.8047378541243631611, 0.7773170766911672303, 0.8047378541243631611, 0.7773170766911672303, 0.8047378541243631611, 0.7773170766911672303, 0.8047378541243631611, 0.7773170766911672303, 0.8047378541243631611, 0.7773170766911672303, 0.8047378541243631611, 0.7773170766911672303, 0.8047378541243631611, 0.7773170766911672303, 0.8047378541243631611, 0.7773170766911672303, 0.8047378541243631611, 0.7773170766911672303, 0.8047378541243631611, 0.7773170766911672303, 0.8047378541243631611, 0.7773170766911672303, 0.8047378541243631611, 0.7773170766911672303, 0.8047378541243631611, 0.7773170766911672303, 0.8047378541243631611, 0.7773170766911672303, 0.8047378541243631611, 0.7773170766911672303, 0.8047378541243631611, 0.7773170766911672303, 0.8047378541243631611, 0.7773170766911672303, 0.8047378541243631611, 0.7773170766911672303, 0.8047378541243631611, 0.7773170766911672303, 0.8047378541243631611, 0.7773170766911672303, 0.8047378541243631611, 0.7773170766911672303, 0.8047378541243631611, 0.7773170766911672303, 0.8047378541243631611, 0.7773170766911672303, 0.8047378541243631611, 0.7773170766911672303, 0.8047378541243631611, 0.7773170766911672303, 0.8047378541243631611, 0.7773170766911672303, 0.8047378541243631611, 0.7773170766911672303, 0.8047378541243631611, 0.7773170766911672303, 0.8047378541243631611, 0.7773170766911672303, 0.8047378541243631611, 0.7773170766911672303, 0.8047378541243631611, 0.7773170766911672303, 0.8047378541243631611, 0.7773170766911672303, 0.8047378541243631611, 0.7773170766911672303, 0.8047378541243631611, 0.7773170766911672303, 0.8047378541243631611, 0.7773170766911672303, 0.8047378541243631611, 0.7773170766911672303, 0.8047378541243631611, 0.7773170766911672303, 0.8047378541243631611, 0.7773170766911672303, 0.8047378541243631611, 0.7773170766911672303, 0.8047378541243631611, 0.7773170766911672303, 0.8047378541243631611, 0.7773170766911672303, 0.8047378541243631611, 0.7773170766911672303, 0.8047378541243631611, 0.7773170766911672303, 0.8047378541243631611, 0.7773170766911672303, 0.8047378541243631611, 0.7773170766911672303, 0.8047378541243631611, 0.7773170766911672303, 0.8047378541243631611, 0.7773170766911672303, 0.8047378541243631611, 0.7773170766911672303, 0.8047378541243631611, 0.7773170766911672303, 0.8047378541243631611, 0.7773170766911672303, 0.8047378541243631611, 0.7773170766911672303, 0.8047378541243631611, 0.7773170766911672303, 0.8047378541243631611, 0.7773170766911672303, 0.8047378541243631611, 0.7773170766911672303, 0.8047378541243631611, 0.7773170766911672303, 0.8047378541243631611, 0.7773170766911672303, 0.8047378541243631611, 0.7773170766911672303, 0.8047378541243631611, 0.7773170766911672303, 0.8047378541243631611, 0.7773170766911672303, 0.8047378541243631611, 0.7773170766911672303, 0.8047378541243631611, 0.7773170766911672303, 0.8047378541243631611, 0.7773170766911672303, 0.8047378541243631611, 0.7773170766911672303, 0.8047378541243631611, 0.7773170766911672303, 0.8047378541243631611, 0.7773170766911672303, 0.8047378541243631611, 0.7773170766911672303, 0.8047378541243631611, 0.7773170766911672303, 0.8047378541243631611, 0.7773170766911672303, 0.8047378541243631611, 0.7773170766911672303, 0.8047378541243631611, 0.7773170766911672303, 0.8047378541243631611, 0.7773170766911672303, 0.8047378541243631611, 0.7773170766911672303, 0.8047378541243631611, 0.7773170766911672303, 0.8047378541243631611, 0.7773170766911672303, 0.8047378541243631611, 0.7773170766911672303, 0.8047378541243631611, 0.7773170766911672303, 0.8047378541243631611, 0.7773170766911672303, 0.8047378541243631611, 0.7773170766911672303, 0.8047378541243631611, 0.7773170766911672303, 0.8047378541243631611, 0.7773170766911672303, 0.8047378541243631611, 0.7773170766911672303, 0.8047378541243631611, 0.7773170766911672303, 0.8047378541243631611, 0.7773170766911672303, 0.8047378541243631611, 0.7773170766911672303, 0.8047378541243631611, 0.7773170766911672303, 0.8047378541243631611, 0.7773170766911672303, 0.8047378541243631611, 0.7773170766911672303, 0.8047378541243631611, 0.7773170766911672303, 0.8047378541243631611, 0.7773170766911672303, 0.8047378541243631611, 0.7773170766911672303, 0.8047378541243631611, 0.7773170766911672303, 0.8047378541243631611, 0.7773170766911672303, 0.8047378541243631611, 0.7773170766911672303, 0.8047378541243631611, 0.7773170766911672303, 0.8047378541243631611, 0.7773170766911672303, 0.8047378541243631611, 0.7773170766911672303, 0.8047378541243631611, 0.7773170766911672303, 0.8047378541243631611, 0.7773170766911672303, 0.8047378541243631611, 0.7773170766911672303, 0.8047378541243631611, 0.7773170766911672303, 0.8047378541243631611, 0.7773170766911672303, 0.8047378541243631611, 0.7773170766911672303, 0.8047378541243631611, 0.7773170766911672303, 0.8047378541243631611, 0.7773170766911672303, 0.8047378541243631611, 0.7773170766911672303, 0.8047378541243631611, 0.7773170766911672303, 0.8047378541243631611, 0.7773170766911672303, 0.8047378541243631611, 0.7773170766911672303, 0.8047378541243631611, 0.7773170766911672303, 0.8047378541243631611, 0.7773170766911672303, 0.8047378541243631611, 0.7773170766911672303, 0.8047378541243631611, 0.7773170766911672303, 0.8047378541243631611, 0.7773170766911672303, 0.8047378541243631611, 0.7773170766911672303, 0.8047378541243631611, 0.7773170766911672303, 0.8047378541243631611, 0.7773170766911672303, 0.8047378541243631611, 0.7773170766911672303, 0.8047378541243631611, 0.7773170766911672303, 0.8047378541243631611, 0.7773170766911672303, 0.8047378541243631611, 0.7773170766911672303, 0.8047378541243631611, 0.7773170766911672303, 0.8047378541243631611, 0.7773170766911672303, 0.8047378541243631611, 0.7773170766911672303, 0.8047378541243631611, 0.7773170766911672303, 0.8047378541243631611, 0.7773170766911672303, 0.8047378541243631611, 0.7773170766911672303, 0.8047378541243631611, 0.7773170766911672303, 0.8047378541243631611, 0.7773170766911672303, 0.8047378541243631611, 0.7773170766911672303, 0.8047378541243631611, 0.7773170766911672303, 0.8047378541243631611, 0.7773170766911672303, 0.8047378541243631611, 0.7773170766911672303, 0.8047378541243631611, 0.7773170766911672303, 0.8047378541243631611, 0.7773170766911672303, 0.8047378541243631611, 0.7773170766911672303, 0.8047378541243631611, 0.7773170766911672303, 0.8047378541243631611, 0.7773170766911672303, 0.8047378541243631611, 0.7773170766911672303, 0.8047378541243631611, 0.7773170766911672303, 0.8047378541243631611, 0.7773170766911672303, 0.8047378541243631611, 0.7773170766911672303, 0.8047378541243631611, 0.7773170766911672303, 0.8047378541243631611, 0.7773170766911672303, 0.8047378541243631611, 0.7773170766911672303, 0.8047378541243631611, 0.7773170766911672303, 0.8047378541243631611, 0.7773170766911672303, 0.8047378541243631611, 0.7773170766911672303, 0.8047378541243631611, 0.7773170766911672303, 0.8047378541243631611, 0.7773170766911672303, 0.8047378541243631611, 0.7773170766911672303, 0.8047378541243631611, 0.7773170766911672303, 0.8047378541243631611, 0.7773170766911672303, 0.8047378541243631611, 0.7773170766911672303, 0.8047378541243631611, 0.7773170766911672303, 0.8047378541243631611, 0.7773170766911672303, 0.8047378541243631611, 0.7773170766911672303, 0.8047378541243631611, 0.7773170766911672303, 0.8047378541243631611, 0.7773170766911672303, 0.8047378541243631611, 0.7773170766911672303, 0.8047378541243631611, 0.7773170766911672303, 0.8047378541243631611, 0.7773170766911672303, 0.8047378541243631611, 0.7773170766911672303, 0.8047378541243631611, 0.7773170766911672303, 0.8047378541243631611, 0.7773170766911672303, 0.8047378541243631611, 0.7773170766911672303, 0.8047378541243631611, 0.7773170766911672303, 0.8047378541243631611, 0.7773170766911672303, 0.8047378541243631611, 0.7773170766911672303, 0.8047378541243631611, 0.7773170766911672303, 0.8047378541243631611, 0.7773170766911672303, 0.8047378541243631611, 0.7773170766911672303, 0.8047378541243631611, 0.7773170766911672303, 0.8047378541243631611, 0.7773170766911672303, 0.8047378541243631611, 0.7773170766911672303, 0.8047378541243631611, 0.7773170766911672303, 0.8047378541243631611, 0.7773170766911672303, 0.8047378541243631611, 0.7773170766911672303, 0.8047378541243631611, 0.7773170766911672303, 0.8047378541243631611, 0.7773170766911672303, 0.8047378541243631611, 0.7773170766911672303, 0.8047378541243631611, 0.7773170766911672303, 0.8047378541243631611, 0.7773170766911672303, 0.8047378541243631611, 0.7773170766911672303, 0.8047378541243631611),
 ( 1.000000000000000000, 0.9659258262890683122, 1.000000000000000000, 0.9659258262890683122, 1.000000000000000000, 0.9659258262890683122, 1.000000000000000000, 0.9659258262890683122, 1.000000000000000000, 0.9659258262890683122, 1.000000000000000000, 0.9659258262890683122, 1.000000000000000000, 0.9659258262890683122, 1.000000000000000000, 0.9659258262890683122, 1.000000000000000000, 0.9659258262890683122, 1.000000000000000000, 0.9659258262890683122, 1.000000000000000000, 0.9659258262890683122, 1.000000000000000000, 0.9659258262890683122, 1.000000000000000000, 0.9659258262890683122, 1.000000000000000000, 0.9659258262890683122, 1.000000000000000000, 0.9659258262890683122, 1.000000000000000000, 0.9659258262890683122, 1.000000000000000000, 0.9659258262890683122, 1.000000000000000000, 0.9659258262890683122, 1.000000000000000000, 0.9659258262890683122, 1.000000000000000000, 0.9659258262890683122, 1.000000000000000000, 0.9659258262890683122, 1.000000000000000000, 0.9659258262890683122, 1.000000000000000000, 0.9659258262890683122, 1.000000000000000000, 0.9659258262890683122, 1.000000000000000000, 0.9659258262890683122, 1.000000000000000000, 0.9659258262890683122, 1.000000000000000000, 0.9659258262890683122, 1.000000000000000000, 0.9659258262890683122, 1.000000000000000000, 0.9659258262890683122, 1.000000000000000000, 0.9659258262890683122, 1.000000000000000000, 0.9659258262890683122, 1.000000000000000000, 0.9659258262890683122, 1.000000000000000000, 0.9659258262890683122, 1.000000000000000000, 0.9659258262890683122, 1.000000000000000000, 0.9659258262890683122, 1.000000000000000000, 0.9659258262890683122, 1.000000000000000000, 0.9659258262890683122, 1.000000000000000000, 0.9659258262890683122, 1.000000000000000000, 0.9659258262890683122, 1.000000000000000000, 0.9659258262890683122, 1.000000000000000000, 0.9659258262890683122, 1.000000000000000000, 0.9659258262890683122, 1.000000000000000000, 0.9659258262890683122, 1.000000000000000000, 0.9659258262890683122, 1.000000000000000000, 0.9659258262890683122, 1.000000000000000000, 0.9659258262890683122, 1.000000000000000000, 0.9659258262890683122, 1.000000000000000000, 0.9659258262890683122, 1.000000000000000000, 0.9659258262890683122, 1.000000000000000000, 0.9659258262890683122, 1.000000000000000000, 0.9659258262890683122, 1.000000000000000000, 0.9659258262890683122, 1.000000000000000000, 0.9659258262890683122, 1.000000000000000000, 0.9659258262890683122, 1.000000000000000000, 0.9659258262890683122, 1.000000000000000000, 0.9659258262890683122, 1.000000000000000000, 0.9659258262890683122, 1.000000000000000000, 0.9659258262890683122, 1.000000000000000000, 0.9659258262890683122, 1.000000000000000000, 0.9659258262890683122, 1.000000000000000000, 0.9659258262890683122, 1.000000000000000000, 0.9659258262890683122, 1.000000000000000000, 0.9659258262890683122, 1.000000000000000000, 0.9659258262890683122, 1.000000000000000000, 0.9659258262890683122, 1.000000000000000000, 0.9659258262890683122, 1.000000000000000000, 0.9659258262890683122, 1.000000000000000000, 0.9659258262890683122, 1.000000000000000000, 0.9659258262890683122, 1.000000000000000000, 0.9659258262890683122, 1.000000000000000000, 0.9659258262890683122, 1.000000000000000000, 0.9659258262890683122, 1.000000000000000000, 0.9659258262890683122, 1.000000000000000000, 0.9659258262890683122, 1.000000000000000000, 0.9659258262890683122, 1.000000000000000000, 0.9659258262890683122, 1.000000000000000000, 0.9659258262890683122, 1.000000000000000000, 0.9659258262890683122, 1.000000000000000000, 0.9659258262890683122, 1.000000000000000000, 0.9659258262890683122, 1.000000000000000000, 0.9659258262890683122, 1.000000000000000000, 0.9659258262890683122, 1.000000000000000000, 0.9659258262890683122, 1.000000000000000000, 0.9659258262890683122, 1.000000000000000000, 0.9659258262890683122, 1.000000000000000000, 0.9659258262890683122, 1.000000000000000000, 0.9659258262890683122, 1.000000000000000000, 0.9659258262890683122, 1.000000000000000000, 0.9659258262890683122, 1.000000000000000000, 0.9659258262890683122, 1.000000000000000000, 0.9659258262890683122, 1.000000000000000000, 0.9659258262890683122, 1.000000000000000000, 0.9659258262890683122, 1.000000000000000000, 0.9659258262890683122, 1.000000000000000000, 0.9659258262890683122, 1.000000000000000000, 0.9659258262890683122, 1.000000000000000000, 0.9659258262890683122, 1.000000000000000000, 0.9659258262890683122, 1.000000000000000000, 0.9659258262890683122, 1.000000000000000000, 0.9659258262890683122, 1.000000000000000000, 0.9659258262890683122, 1.000000000000000000, 0.9659258262890683122, 1.000000000000000000, 0.9659258262890683122, 1.000000000000000000, 0.9659258262890683122, 1.000000000000000000, 0.9659258262890683122, 1.000000000000000000, 0.9659258262890683122, 1.000000000000000000, 0.9659258262890683122, 1.000000000000000000, 0.9659258262890683122, 1.000000000000000000, 0.9659258262890683122, 1.000000000000000000, 0.9659258262890683122, 1.000000000000000000, 0.9659258262890683122, 1.000000000000000000, 0.9659258262890683122, 1.000000000000000000, 0.9659258262890683122, 1.000000000000000000, 0.9659258262890683122, 1.000000000000000000, 0.9659258262890683122, 1.000000000000000000, 0.9659258262890683122, 1.000000000000000000, 0.9659258262890683122, 1.000000000000000000, 0.9659258262890683122, 1.000000000000000000, 0.9659258262890683122, 1.000000000000000000, 0.9659258262890683122, 1.000000000000000000, 0.9659258262890683122, 1.000000000000000000, 0.9659258262890683122, 1.000000000000000000, 0.9659258262890683122, 1.000000000000000000, 0.9659258262890683122, 1.000000000000000000, 0.9659258262890683122, 1.000000000000000000, 0.9659258262890683122, 1.000000000000000000, 0.9659258262890683122, 1.000000000000000000, 0.9659258262890683122, 1.000000000000000000, 0.9659258262890683122, 1.000000000000000000, 0.9659258262890683122, 1.000000000000000000, 0.9659258262890683122, 1.000000000000000000, 0.9659258262890683122, 1.000000000000000000, 0.9659258262890683122, 1.000000000000000000, 0.9659258262890683122, 1.000000000000000000, 0.9659258262890683122, 1.000000000000000000, 0.9659258262890683122, 1.000000000000000000, 0.9659258262890683122, 1.000000000000000000, 0.9659258262890683122, 1.000000000000000000, 0.9659258262890683122, 1.000000000000000000, 0.9659258262890683122, 1.000000000000000000, 0.9659258262890683122, 1.000000000000000000, 0.9659258262890683122, 1.000000000000000000, 0.9659258262890683122, 1.000000000000000000, 0.9659258262890683122, 1.000000000000000000, 0.9659258262890683122, 1.000000000000000000, 0.9659258262890683122, 1.000000000000000000, 0.9659258262890683122, 1.000000000000000000, 0.9659258262890683122, 1.000000000000000000, 0.9659258262890683122, 1.000000000000000000, 0.9659258262890683122, 1.000000000000000000, 0.9659258262890683122, 1.000000000000000000, 0.9659258262890683122, 1.000000000000000000, 0.9659258262890683122, 1.000000000000000000, 0.9659258262890683122, 1.000000000000000000, 0.9659258262890683122, 1.000000000000000000, 0.9659258262890683122, 1.000000000000000000, 0.9659258262890683122, 1.000000000000000000, 0.9659258262890683122, 1.000000000000000000, 0.9659258262890683122, 1.000000000000000000, 0.9659258262890683122, 1.000000000000000000, 0.9659258262890683122, 1.000000000000000000, 0.9659258262890683122, 1.000000000000000000, 0.9659258262890683122, 1.000000000000000000, 0.9659258262890683122, 1.000000000000000000, 0.9659258262890683122, 1.000000000000000000, 0.9659258262890683122, 1.000000000000000000, 0.9659258262890683122, 1.000000000000000000, 0.9659258262890683122, 1.000000000000000000, 0.9659258262890683122, 1.000000000000000000, 0.9659258262890683122, 1.000000000000000000, 0.9659258262890683122, 1.000000000000000000, 0.9659258262890683122, 1.000000000000000000, 0.9659258262890683122, 1.000000000000000000, 0.9659258262890683122, 1.000000000000000000, 0.9659258262890683122, 1.000000000000000000, 0.9659258262890683122, 1.000000000000000000, 0.9659258262890683122, 1.000000000000000000, 0.9659258262890683122, 1.000000000000000000, 0.9659258262890683122, 1.000000000000000000, 0.9659258262890683122, 1.000000000000000000, 0.9659258262890683122, 1.000000000000000000, 0.9659258262890683122, 1.000000000000000000, 0.9659258262890683122, 1.000000000000000000, 0.9659258262890683122, 1.000000000000000000, 0.9659258262890683122, 1.000000000000000000, 0.9659258262890683122, 1.000000000000000000, 0.9659258262890683122, 1.000000000000000000, 0.9659258262890683122, 1.000000000000000000, 0.9659258262890683122, 1.000000000000000000, 0.9659258262890683122, 1.000000000000000000, 0.9659258262890683122, 1.000000000000000000, 0.9659258262890683122, 1.000000000000000000, 0.9659258262890683122, 1.000000000000000000, 0.9659258262890683122, 1.000000000000000000, 0.9659258262890683122, 1.000000000000000000, 0.9659258262890683122, 1.000000000000000000, 0.9659258262890683122, 1.000000000000000000, 0.9659258262890683122, 1.000000000000000000, 0.9659258262890683122, 1.000000000000000000, 0.9659258262890683122, 1.000000000000000000, 0.9659258262890683122, 1.000000000000000000, 0.9659258262890683122, 1.000000000000000000, 0.9659258262890683122, 1.000000000000000000, 0.9659258262890683122, 1.000000000000000000, 0.9659258262890683122, 1.000000000000000000, 0.9659258262890683122, 1.000000000000000000, 0.9659258262890683122, 1.000000000000000000, 0.9659258262890683122, 1.000000000000000000, 0.9659258262890683122, 1.000000000000000000, 0.9659258262890683122, 1.000000000000000000, 0.9659258262890683122, 1.000000000000000000, 0.9659258262890683122, 1.000000000000000000, 0.9659258262890683122, 1.000000000000000000, 0.9659258262890683122, 1.000000000000000000, 0.9659258262890683122, 1.000000000000000000, 0.9659258262890683122, 1.000000000000000000, 0.9659258262890683122, 1.000000000000000000, 0.9659258262890683122, 1.000000000000000000, 0.9659258262890683122, 1.000000000000000000, 0.9659258262890683122, 1.000000000000000000, 0.9659258262890683122, 1.000000000000000000, 0.9659258262890683122, 1.000000000000000000, 0.9659258262890683122, 1.000000000000000000, 0.9659258262890683122, 1.000000000000000000, 0.9659258262890683122, 1.000000000000000000, 0.9659258262890683122, 1.000000000000000000, 0.9659258262890683122, 1.000000000000000000, 0.9659258262890683122, 1.000000000000000000, 0.9659258262890683122, 1.000000000000000000, 0.9659258262890683122, 1.000000000000000000, 0.9659258262890683122, 1.000000000000000000, 0.9659258262890683122, 1.000000000000000000, 0.9659258262890683122, 1.000000000000000000, 0.9659258262890683122, 1.000000000000000000, 0.9659258262890683122, 1.000000000000000000, 0.9659258262890683122, 1.000000000000000000, 0.9659258262890683122, 1.000000000000000000) ) ) 
 REPRESENTATION_ITEM ( '' )  SURFACE ( )  );
#11198=CARTESIAN_POINT ( 'NONE',  ( 0.2867679344610365999, -0.2867679344610365444, -0.2480314960629920740 ) ) ;
#11203=CARTESIAN_POINT ( 'NONE',  ( 5.785732909357575061E-17, -0.4724409448818898682, -1.811023622047244208 ) ) ;
#11205=CARTESIAN_POINT ( 'NONE',  ( -0.4091458600556405756, 0.2362204724409446288, -0.9711286089238845287 ) ) ;
#11209=CARTESIAN_POINT ( 'NONE',  ( 0.3458507752293908943, -0.3458507752293908943, -1.988188976377952777 ) ) ;
#11212=CARTESIAN_POINT ( 'NONE',  ( -0.3392501089628018329, -0.1958661417322836440, -0.4474872458979509138 ) ) ;
#11214=CARTESIAN_POINT ( 'NONE',  ( 0.1958661417322834775, 0.3392501089628018884, -1.016404199475065662 ) ) ;
#11219=CARTESIAN_POINT ( 'NONE',  ( -9.594673741351313045E-17, 0.3917322834645670104, -2.196850393700787496 ) ) ;
#11222=CARTESIAN_POINT ( 'NONE',  ( 0.1265901696524989462, 0.4724409448818897572, -0.7001312335958002064 ) ) ;
#11235=CARTESIAN_POINT ( 'NONE',  ( -0.2925321140481930149, -0.2925321140481933480, -2.025590551181101873 ) ) ;
#11243=CARTESIAN_POINT ( 'NONE',  ( -0.1070741851644057135, 0.3996062992125984925, -0.08333333333333335646 ) ) ;
#11244=EDGE_CURVE ( 'NONE', #35624, #32899, #23598, .T. ) ;
#11245=CARTESIAN_POINT ( 'NONE',  ( -0.1998031496062994683, 0.3460692066303958092, -0.6430446194225721834 ) ) ;
#11247=CARTESIAN_POINT ( 'NONE',  ( 0.3420746716998660508, -0.1974969037888703871, -0.2624671916010499206 ) ) ;
#11249=CARTESIAN_POINT ( 'NONE',  ( 0.03143970413924662005, -0.3977953519386796533, -5.548669992249399297E-14 ) ) ;
#11253=CARTESIAN_POINT ( 'NONE',  ( -9.674558042662122972E-17, 0.3949938075777409963, -0.7066929133858269596 ) ) ;
#11258=CARTESIAN_POINT ( 'NONE',  ( 0.4091458600556403535, 0.2362204724409449896, -1.076115485564304475 ) ) ;
#11259=CARTESIAN_POINT ( 'NONE',  ( 0.1070741851644053666, 0.3996062992125986035, -2.513123359580052174 ) ) ;
#11262=CARTESIAN_POINT ( 'NONE',  ( -0.3392501089628019995, 0.1958661417322831999, -0.8103867698500807348 ) ) ;
#11272=CARTESIAN_POINT ( 'NONE',  ( 0.1049643490035304938, -0.3917322834645669549, -0.8648293963254591876 ) ) ;
#11275=CARTESIAN_POINT ( 'NONE',  ( 0.1974969037888706369, -0.3420746716998659953, -1.509186351706036655 ) ) ;
#11280=CARTESIAN_POINT ( 'NONE',  ( -0.3460692066303960868, 0.1998031496062990242, 0.1312335958005249048 ) ) ;
#11287=CARTESIAN_POINT ( 'NONE',  ( -0.3917322834645671215, 0.1049643490035301469, 0.1975065616797899160 ) ) ;
#11294=CARTESIAN_POINT ( 'NONE',  ( 0.3460692066303959757, -0.1998031496062991907, -2.152230971128608950 ) ) ;
#11297=CARTESIAN_POINT ( 'NONE',  ( 0.2925321140481932369, 0.2925321140481932369, -1.631889763779527325 ) ) ;
#11301=CARTESIAN_POINT ( 'NONE',  ( -0.2362204724409451284, 0.4091458600556402425, -0.3280839895013123453 ) ) ;
#11303=CARTESIAN_POINT ( 'NONE',  ( -0.3917322834645670104, -7.196005306013484475E-17, -0.03149606299212594218 ) ) ;
#11309=CARTESIAN_POINT ( 'NONE',  ( -0.2362204724409451284, 0.4091458600556402425, -2.452099737532808188 ) ) ;
#11311=CARTESIAN_POINT ( 'NONE',  ( 0.3949938075777409408, -0.1058382717557499186, -2.235564304461942431 ) ) ;
#11323=CARTESIAN_POINT ( 'NONE',  ( 0.2362204724409449064, 0.4091458600556404646, -1.008530183727034180 ) ) ;
#11332=CARTESIAN_POINT ( 'NONE',  ( -0.2925321140481930149, -0.2925321140481933480, -0.7657480314960628531 ) ) ;
#11334=CARTESIAN_POINT ( 'NONE',  ( 0.1049643490035304938, -0.3917322834645669549, -2.374671916010498762 ) ) ;
#11352=CARTESIAN_POINT ( 'NONE',  ( -9.594673741351313045E-17, 0.3917322834645670104, -1.501968503937008093 ) ) ;
#11353=CARTESIAN_POINT ( 'NONE',  ( -0.1188761721681626526, 0.3738583250858228402, -1.220472440944881942 ) ) ;
#11357=CARTESIAN_POINT ( 'NONE',  ( 0.3996062992125985480, -0.1070741851644052972, -2.393044619422572072 ) ) ;
#11359=CARTESIAN_POINT ( 'NONE',  ( -0.3996062992125986035, -7.340648628747425578E-17, -0.8267716535433070613 ) ) ;
#11363=CARTESIAN_POINT ( 'NONE',  ( -0.2867679344610364334, -0.2867679344610367109, -2.728346456692912536 ) ) ;
#11375=CARTESIAN_POINT ( 'NONE',  ( 4.797336870675656522E-17, -0.3917322834645670104, -2.840551181102362044 ) ) ;
#11378=CARTESIAN_POINT ( 'NONE',  ( 0.3420746716998659953, 0.1974969037888705536, -0.1312335958005249881 ) ) ;
#11382=CARTESIAN_POINT ( 'NONE',  ( 0.4091458600556403535, 0.2362204724409449896, -0.1312335958005249326 ) ) ;
#11386=CARTESIAN_POINT ( 'NONE',  ( 0.3917322834645670659, -0.1049643490035303273, -1.210649237041681703 ) ) ;
#11388=CARTESIAN_POINT ( 'NONE',  ( -0.1958661417322836718, 0.3392501089628017219, -2.459973753280839670 ) ) ;
#11393=CARTESIAN_POINT ( 'NONE',  ( -0.1070741851644056997, 0.3996062992125986035, -0.7939632545931758489 ) ) ;
#11395=CARTESIAN_POINT ( 'NONE',  ( -0.2925321140481932369, 0.2925321140481931259, -0.4114173228346455491 ) ) ;
#11397=CARTESIAN_POINT ( 'NONE',  ( 0.1070741851644054915, -0.3996062992125986035, -2.447506561679789527 ) ) ;
#11398=CARTESIAN_POINT ( 'NONE',  ( -0.1049643490035302024, -0.3917322834645671215, -1.574146981627296604 ) ) ;
#11402=CARTESIAN_POINT ( 'NONE',  ( 5.785732909357575061E-17, -0.4724409448818898682, -1.257874015748031260 ) ) ;
#11405=CARTESIAN_POINT ( 'NONE',  ( -0.3420746716998660508, -0.1974969037888706924, -0.9166666666666668517 ) ) ;
#11419=CARTESIAN_POINT ( 'NONE',  ( 0.1998031496062992463, 0.3460692066303959202, -1.638451443569554078 ) ) ;
#11421=CARTESIAN_POINT ( 'NONE',  ( 0.1958661417322836440, -0.3392501089628017219, -1.501312335958005173 ) ) ;
#11435=CARTESIAN_POINT ( 'NONE',  ( 0.3392501089628018884, -0.1958661417322834220, -0.8195538057742782767 ) ) ;
#11451=CARTESIAN_POINT ( 'NONE',  ( -0.1070741851644051862, -0.3996062992125986590, -1.017060367454068137 ) ) ;
#11453=PLANE ( 'NONE',  #67790 ) ;
#11456=CARTESIAN_POINT ( 'NONE',  ( 0.1265901696524990294, -0.4724409448818896462, -0.2427821522309711322 ) ) ;
#11457=CARTESIAN_POINT ( 'NONE',  ( 0.3949938075777409963, 2.418639510665530435E-17, -2.952755905511811108 ) ) ;
#11460=CARTESIAN_POINT ( 'NONE',  ( 0.1049643490035304938, -0.3917322834645669549, -1.337270341207349000 ) ) ;
#11462=CARTESIAN_POINT ( 'NONE',  ( -0.4724409448818895907, -0.1265901696524993070, -2.408136482939632561 ) ) ;
#11469=CARTESIAN_POINT ( 'NONE',  ( 0.2867679344610365999, -0.2867679344610365999, -0.6508993193887645523 ) ) ;
#11478=CARTESIAN_POINT ( 'NONE',  ( -0.3917322834645671770, 0.1049643490035302024, -1.919310654364516200 ) ) ;
#11486=CARTESIAN_POINT ( 'NONE',  ( -9.594673741351313045E-17, 0.3917322834645670104, -1.344488188976378007 ) ) ;
#11496=CARTESIAN_POINT ( 'NONE',  ( -0.3917322834645671215, 0.1049643490035301469, -2.859580052493438274 ) ) ;
#11504=CARTESIAN_POINT ( 'NONE',  ( -0.3917322834645669549, -0.1049643490035306603, -1.075459317585301777 ) ) ;
#11505=CARTESIAN_POINT ( 'NONE',  ( 0.1265901696524989462, 0.4724409448818897572, 0.08727034120734905587 ) ) ;
#11507=CARTESIAN_POINT ( 'NONE',  ( -9.787531504996566615E-17, 0.3996062992125985480, -2.753937007874015741 ) ) ;
#11516=CARTESIAN_POINT ( 'NONE',  ( 0.1998031496062994128, -0.3460692066303957537, -0.4835958005249343938 ) ) ;
#11518=CARTESIAN_POINT ( 'NONE',  ( -0.2867679344610364334, -0.2867679344610367109, -0.3661417322834645827 ) ) ;
#11533=CARTESIAN_POINT ( 'NONE',  ( -0.1958661417322836995, 0.3392501089628017219, -0.9547437252306580913 ) ) ;
#11537=CARTESIAN_POINT ( 'NONE',  ( 0.1265901696524989462, 0.4724409448818897572, -1.959973753280839892 ) ) ;
#11558=CARTESIAN_POINT ( 'NONE',  ( -0.3460692066303960868, 0.1998031496062990242, -0.02624671916010500733 ) ) ;
#11559=CARTESIAN_POINT ( 'NONE',  ( -0.3460692066303960313, 0.1998031496062989965, -2.780183727034120977 ) ) ;
#11564=CARTESIAN_POINT ( 'NONE',  ( -0.3996062992125986035, -7.340648628747425578E-17, -2.086614173228346303 ) ) ;
#11565=CARTESIAN_POINT ( 'NONE',  ( 0.3949938075777409963, 2.418639510665530435E-17, -1.535433070866141447 ) ) ;
#11566=CARTESIAN_POINT ( 'NONE',  ( 0.3996062992125986590, -0.1070741851644053111, -2.788713910761154047 ) ) ;
#11568=CARTESIAN_POINT ( 'NONE',  ( 0.2867679344610366554, -0.2867679344610365444, -0.4055118110236220486 ) ) ;
#11572=CARTESIAN_POINT ( 'NONE',  ( 0.3949938075777408852, 0.1058382717557500435, -2.563648293963254776 ) ) ;
#11576=CARTESIAN_POINT ( 'NONE',  ( -0.4724409448818895907, -0.1265901696524993070, -2.723097112860892288 ) ) ;
#11578=CARTESIAN_POINT ( 'NONE',  ( -0.3460692066303958092, -0.1998031496062994683, -2.257217847769029007 ) ) ;
#11586=CARTESIAN_POINT ( 'NONE',  ( -0.1049643490035302024, -0.3917322834645671215, -0.1568241469816273603 ) ) ;
#11593=CARTESIAN_POINT ( 'NONE',  ( 0.1049643490035304938, -0.3917322834645669549, -0.4849081364829396779 ) ) ;
#11594=CARTESIAN_POINT ( 'NONE',  ( -0.3917322834645671215, 0.1049643490035301469, -1.442257217847769057 ) ) ;
#11595=CARTESIAN_POINT ( 'NONE',  ( 0.1958661417322836440, -0.3392501089628017219, -2.918635170603674389 ) ) ;
#11598=CARTESIAN_POINT ( 'NONE',  ( 0.1974969037888704704, 0.3420746716998660508, -2.664041994750656173 ) ) ;
#11603=CARTESIAN_POINT ( 'NONE',  ( 0.3996062992125986035, 0.1070741851644054776, -1.384514435695537671 ) ) ;
#11608=CARTESIAN_POINT ( 'NONE',  ( 0.3392501089628018884, -0.1958661417322834220, -0.5045931758530184386 ) ) ;
#11616=CARTESIAN_POINT ( 'NONE',  ( -1.157146581871515012E-16, 0.4724409448818898682, -2.204724409448818978 ) ) ;
#11622=CARTESIAN_POINT ( 'NONE',  ( -0.4724409448818880364, -0.1265901696525023323, -2.250656167979002920 ) ) ;
#11627=CARTESIAN_POINT ( 'NONE',  ( -0.3917322834645668994, -0.1049643490035306742, -0.2834452511472947966 ) ) ;
#11629=CARTESIAN_POINT ( 'NONE',  ( -0.3392501089628017219, -0.1958661417322836718, -0.7670603674540683592 ) ) ;
#11635=CARTESIAN_POINT ( 'NONE',  ( 0.3917322834645669549, 0.1049643490035304660, -2.636482939632545985 ) ) ;
#11637=VECTOR ( 'NONE', #58811, 39.37007874015748143 ) ;
#11640=CARTESIAN_POINT ( 'NONE',  ( -0.4091458600556405756, 0.2362204724409446288, -0.5754593175853018883 ) ) ;
#11649=CARTESIAN_POINT ( 'NONE',  ( 0.4724409448818897017, 0.1265901696524990294, -0.2821522309711286258 ) ) ;
#11653=CARTESIAN_POINT ( 'NONE',  ( 4.893765752498283308E-17, -0.3996062992125985480, -1.887795275590550936 ) ) ;
#11662=CARTESIAN_POINT ( 'NONE',  ( -0.3996062992125986035, 0.1070741851644051584, -0.5820209973753279753 ) ) ;
#11663=CARTESIAN_POINT ( 'NONE',  ( 0.2925321140481932369, 0.2925321140481932369, -1.082677165354330562 ) ) ;
#11665=CARTESIAN_POINT ( 'NONE',  ( -0.3949938075777409963, -7.255918531996591613E-17, -0.3543307086614174151 ) ) ;
#11671=CARTESIAN_POINT ( 'NONE',  ( -0.3949938075777409963, -7.255918531996591613E-17, -1.218503937007874072 ) ) ;
#11676=CARTESIAN_POINT ( 'NONE',  ( 0.4724409448818898682, 2.892866454678787531E-17, -1.377952755905511806 ) ) ;
#11677=CARTESIAN_POINT ( 'NONE',  ( -0.1998031496062994683, 0.3460692066303958092, -2.532808398950130879 ) ) ;
#11679=( BOUNDED_CURVE ( )  B_SPLINE_CURVE ( 2, ( #59803, #2988, #53894, #60226, #2157, #48003, #53484, #40869, #72860, #54313, #79194, #22343, #27402 ),
 .UNSPECIFIED., .F., .F. ) 
 B_SPLINE_CURVE_WITH_KNOTS ( ( 3, 2, 2, 2, 2, 2, 3 ),
 ( 0.7124999999999999112, 0.7166666666666665630, 0.7208333333333332149, 0.7249999999999998668, 0.7291666666666665186, 0.7333333333333331705, 0.7374999999999999334 ),
 .UNSPECIFIED. ) 
 CURVE ( )  GEOMETRIC_REPRESENTATION_ITEM ( )  RATIONAL_B_SPLINE_CURVE ( ( 1.000000000000000888, 0.9659258262890674240, 1.000000000000000000, 0.9659258262890683122, 1.000000000000000000, 0.9659258262890683122, 1.000000000000000000, 0.9659258262890683122, 1.000000000000000000, 0.9659258262890683122, 1.000000000000000000, 0.9659258262890692004, 0.9999999999999991118 ) ) 
 REPRESENTATION_ITEM ( '' )  );
#11681=ORIENTED_EDGE ( 'NONE', *, *, #41165, .T. ) ;
#11690=VECTOR ( 'NONE', #22114, 39.37007874015748143 ) ;
#11691=CARTESIAN_POINT ( 'NONE',  ( 0.3917322834645669549, 0.1049643490035304660, -1.061679790026246462 ) ) ;
#11694=CARTESIAN_POINT ( 'NONE',  ( 0.2891555358219910499, 0.2891555358219910499, -1.555118110236220375 ) ) ;
#11702=CARTESIAN_POINT ( 'NONE',  ( -0.1998031496062991907, -0.3460692066303959757, -0.3805774278215223183 ) ) ;
#11709=CARTESIAN_POINT ( 'NONE',  ( 0.3917322834645670104, 2.398668435337828261E-17, 0.1122047244094487306 ) ) ;
#11715=CARTESIAN_POINT ( 'NONE',  ( -0.3996062992125986035, -7.340648628747425578E-17, -2.244094488188976388 ) ) ;
#11718=CARTESIAN_POINT ( 'NONE',  ( -0.3996062992125984925, -0.1070741851644056858, -1.540026246719159886 ) ) ;
#11722=CARTESIAN_POINT ( 'NONE',  ( -0.2362204724409447953, -0.4091458600556404646, -0.5380577427821522374 ) ) ;
#11724=CARTESIAN_POINT ( 'NONE',  ( -0.1958661417322836718, 0.3392501089628017219, -2.774934383202099841 ) ) ;
#11730=CARTESIAN_POINT ( 'NONE',  ( -0.4091458600556405756, 0.2362204724409446288, -2.150262467191601079 ) ) ;
#11733=CARTESIAN_POINT ( 'NONE',  ( 0.1058382717557499880, 0.3949938075777409408, -2.117454068241470200 ) ) ;
#11746=DIRECTION ( 'NONE',  ( 1.000000000000000000, 0.000000000000000000, 0.000000000000000000 ) ) ;
#11754=CARTESIAN_POINT ( 'NONE',  ( 0.1998031496062994128, -0.3460692066303957537, -0.6410761154855643129 ) ) ;
#11756=CARTESIAN_POINT ( 'NONE',  ( -0.1049643490035307020, 0.3917322834645669549, -2.453412073490813139 ) ) ;
#11773=CARTESIAN_POINT ( 'NONE',  ( -0.3392501089628017219, -0.1958661417322836718, -1.869422572178477848 ) ) ;
#11777=CARTESIAN_POINT ( 'NONE',  ( -0.3458507752293909498, 0.3458507752293908388, -0.4921259842519684624 ) ) ;
#11778=CARTESIAN_POINT ( 'NONE',  ( 0.1070741851644053527, 0.3996062992125985480, -2.589895013123359568 ) ) ;
#11780=CARTESIAN_POINT ( 'NONE',  ( 0.1998031496062992740, 0.3460692066303959757, -1.089238845144356871 ) ) ;
#11781=ORIENTED_EDGE ( 'NONE', *, *, #79349, .T. ) ;
#11782=CARTESIAN_POINT ( 'NONE',  ( 0.1049643490035303689, 0.3917322834645670104, -2.662729658792650778 ) ) ;
#11789=CYLINDRICAL_SURFACE ( 'NONE', #50718, 0.4724409448818898682 ) ;
#11794=CARTESIAN_POINT ( 'NONE',  ( -0.1958661417322836718, 0.3392501089628017219, -2.617454068241469756 ) ) ;
#11797=CARTESIAN_POINT ( 'NONE',  ( -0.1058382717557497937, -0.3949938075777411628, -0.3871391076115485719 ) ) ;
#11798=ORIENTED_EDGE ( 'NONE', *, *, #58932, .T. ) ;
#11803=CARTESIAN_POINT ( 'NONE',  ( 0.1958661417322836718, -0.3392501089628017219, -1.663405142553492810 ) ) ;
#11805=CARTESIAN_POINT ( 'NONE',  ( 0.1049643490035303689, 0.3917322834645670104, -2.755249343832020248 ) ) ;
#11810=CARTESIAN_POINT ( 'NONE',  ( 4.893765752498283924E-17, -0.3996062992125986035, -1.023622047244094446 ) ) ;
#11812=CARTESIAN_POINT ( 'NONE',  ( -0.3996062992125985480, -7.340648628747423112E-17, -0.2736220472440945017 ) ) ;
#11814=CARTESIAN_POINT ( 'NONE',  ( -0.2925321140481932924, 0.2925321140481931814, -2.224409448818897239 ) ) ;
#11816=( BOUNDED_CURVE ( )  B_SPLINE_CURVE ( 2, ( #44683, #64912, #44277, #64073, #19882, #45105, #6410, #77550, #69566, #58160, #50596, #31664, #69967 ),
 .UNSPECIFIED., .F., .F. ) 
 B_SPLINE_CURVE_WITH_KNOTS ( ( 3, 2, 2, 2, 2, 2, 3 ),
 ( 0.1625000000000000056, 0.1666666666666666574, 0.1708333333333333370, 0.1749999999999999889, 0.1791666666666666685, 0.1833333333333333204, 0.1875000000000000000 ),
 .UNSPECIFIED. ) 
 CURVE ( )  GEOMETRIC_REPRESENTATION_ITEM ( )  RATIONAL_B_SPLINE_CURVE ( ( 1.000000000000000000, 0.9659258262890683122, 1.000000000000000000, 0.9659258262890683122, 1.000000000000000000, 0.9659258262890683122, 1.000000000000000000, 0.9659258262890683122, 1.000000000000000000, 0.9659258262890683122, 1.000000000000000000, 0.9659258262890683122, 1.000000000000000000 ) ) 
 REPRESENTATION_ITEM ( '' )  );
#11817=CARTESIAN_POINT ( 'NONE',  ( 0.1958661417322836440, -0.3392501089628017219, -1.593832020997375531 ) ) ;
#11822=CARTESIAN_POINT ( 'NONE',  ( 0.4091458600556403535, 0.2362204724409449896, -1.152887139107611425 ) ) ;
#11825=CARTESIAN_POINT ( 'NONE',  ( 0.3949938075777408852, 0.1058382717557500435, -1.146325459317585338 ) ) ;
#11829=FACE_OUTER_BOUND ( 'NONE', #33927, .T. ) ;
#11835=CARTESIAN_POINT ( 'NONE',  ( -0.2925321140481932369, 0.2925321140481931259, -1.671259842519685179 ) ) ;
#11849=CARTESIAN_POINT ( 'NONE',  ( 0.1049643490035303689, 0.3917322834645670104, -1.022965879265091749 ) ) ;
#11864=CARTESIAN_POINT ( 'NONE',  ( 0.4091458600556404646, -0.2362204724409448231, -0.5774278215223097588 ) ) ;
#11868=CARTESIAN_POINT ( 'NONE',  ( -0.2867679344610366554, 0.2867679344610365444, -2.216535433070866201 ) ) ;
#11872=CARTESIAN_POINT ( 'NONE',  ( 0.1265901696524989462, 0.4724409448818897572, -0.1509186351706036378 ) ) ;
#11873=CARTESIAN_POINT ( 'NONE',  ( -0.3420746716998659953, -0.1974969037888706647, -2.887139107611548461 ) ) ;
#11876=CARTESIAN_POINT ( 'NONE',  ( 0.3917322834645670104, 2.398668435337828261E-17, -1.212598425196850238 ) ) ;
#11878=CARTESIAN_POINT ( 'NONE',  ( 0.2362204724409449064, 0.4091458600556404646, -2.821522309711286258 ) ) ;
#11885=CARTESIAN_POINT ( 'NONE',  ( -0.3392501089628019439, 0.1958661417322832554, -0.7362011566591059042 ) ) ;
#11890=DIRECTION ( 'NONE',  ( -1.000000000000000000, 0.000000000000000000, 0.000000000000000000 ) ) ;
#11892=CARTESIAN_POINT ( 'NONE',  ( -9.594673741351313045E-17, 0.3917322834645670659, -2.201462885335645048 ) ) ;
#11899=CARTESIAN_POINT ( 'NONE',  ( 0.3392501089628018329, 0.1958661417322835607, -1.475721784776902856 ) ) ;
#11908=CARTESIAN_POINT ( 'NONE',  ( -0.1049643490035307020, 0.3917322834645669549, -2.833333333333333037 ) ) ;
#11910=ORIENTED_EDGE ( 'NONE', *, *, #21817, .F. ) ;
#11914=PLANE ( 'NONE',  #58567 ) ;
#11915=CARTESIAN_POINT ( 'NONE',  ( -0.1049643490035307020, 0.3917322834645669549, -1.351049868766404538 ) ) ;
#11916=CARTESIAN_POINT ( 'NONE',  ( -0.2362204724409451284, 0.4091458600556402425, 0.06758530183727033680 ) ) ;
#11918=CARTESIAN_POINT ( 'NONE',  ( 0.1058382717557499880, 0.3949938075777409408, 0.08727034120734906975 ) ) ;
#11927=CARTESIAN_POINT ( 'NONE',  ( 0.1070741851644053388, 0.3996062992125986035, -0.3851706036745406458 ) ) ;
#11929=CARTESIAN_POINT ( 'NONE',  ( 0.3917322834645669549, 0.1049643490035304660, -0.1167979002624671692 ) ) ;
#11931=PLANE ( 'NONE',  #56012 ) ;
#11944=CARTESIAN_POINT ( 'NONE',  ( -0.2867679344610365444, -0.2867679344610367664, -0.8431951688002119472 ) ) ;
#11946=CARTESIAN_POINT ( 'NONE',  ( 0.2017716535433070613, 0.2017716535433070613, -0.3937007874015748254 ) ) ;
#11948=CARTESIAN_POINT ( 'NONE',  ( -0.1265901696524993347, 0.4724409448818895907, -2.288057742782152015 ) ) ;
#11967=CARTESIAN_POINT ( 'NONE',  ( -0.1998031496062991907, -0.3460692066303959757, -0.5380577427821522374 ) ) ;
#11968=CARTESIAN_POINT ( 'NONE',  ( -0.3996062992125986590, 0.1070741851644051723, -2.786745406824146620 ) ) ;
#11973=CARTESIAN_POINT ( 'NONE',  ( -0.3996062992125986035, -0.1070741851644056997, -2.093175853018372834 ) ) ;
#11974=CARTESIAN_POINT ( 'NONE',  ( -0.2891555358219908833, -0.2891555358219912164, -1.476377952755905332 ) ) ;
#11976=CARTESIAN_POINT ( 'NONE',  ( -0.4724409448818898682, -8.678599364036362592E-17, -2.559055118110236560 ) ) ;
#11977=CARTESIAN_POINT ( 'NONE',  ( 0.3917322834645670104, -0.1049643490035303273, -0.7335958005249343383 ) ) ;
#11981=CARTESIAN_POINT ( 'NONE',  ( 0.1974969037888706092, -0.3420746716998660508, -2.530839895013123453 ) ) ;
#11986=CARTESIAN_POINT ( 'NONE',  ( 0.1070741851644053527, 0.3996062992125986590, -2.355643044619422533 ) ) ;
#11992=CARTESIAN_POINT ( 'NONE',  ( 0.3917322834645669549, 0.1049643490035304660, -0.2093175853018373611 ) ) ;
#11999=CARTESIAN_POINT ( 'NONE',  ( 0.1049643490035303689, 0.3917322834645670104, -0.7080052493438320216 ) ) ;
#12000=CARTESIAN_POINT ( 'NONE',  ( 0.1049643490035304938, -0.3917322834645669549, -1.652230971128608505 ) ) ;
#12001=CARTESIAN_POINT ( 'NONE',  ( 0.1049643490035304938, -0.3917322834645669549, -2.597112860892388131 ) ) ;
#12004=CARTESIAN_POINT ( 'NONE',  ( -0.3420746716998659953, -0.1974969037888706647, -2.729658792650918819 ) ) ;
#12008=CARTESIAN_POINT ( 'NONE',  ( 0.3996062992125986035, 2.446882876249141962E-17, -1.535433070866141669 ) ) ;
#12013=CARTESIAN_POINT ( 'NONE',  ( -0.1958661417322834220, -0.3392501089628018884, -0.4652230971128609727 ) ) ;
#12023=CARTESIAN_POINT ( 'NONE',  ( 0.2362204724409449064, 0.4091458600556404646, -2.034120734908136718 ) ) ;
#12029=CARTESIAN_POINT ( 'NONE',  ( -0.4724409448818898682, -8.678599364036362592E-17, -2.478346456692913868 ) ) ;
#12033=CARTESIAN_POINT ( 'NONE',  ( 0.3392501089628018329, -0.1958661417322834497, -0.3425003692575309677 ) ) ;
#12035=CARTESIAN_POINT ( 'NONE',  ( 0.1049643490035304799, -0.3917322834645669549, -0.9573490813648293241 ) ) ;
#12041=CARTESIAN_POINT ( 'NONE',  ( 0.3392501089628018884, -0.1958661417322834220, -2.774278215223096922 ) ) ;
#12044=CARTESIAN_POINT ( 'NONE',  ( 0.1265901696524990294, -0.4724409448818896462, -0.6345144356955381149 ) ) ;
#12057=CARTESIAN_POINT ( 'NONE',  ( -0.1070741851644056997, 0.3996062992125984925, -1.973097112860892510 ) ) ;
#12063=CARTESIAN_POINT ( 'NONE',  ( -0.3458507752293906723, -0.3458507752293910609, -0.05905511811023621271 ) ) ;
#12065=CARTESIAN_POINT ( 'NONE',  ( -0.3996062992125985480, -7.340648628747423112E-17, -0.7460629921259841479 ) ) ;
#12066=CARTESIAN_POINT ( 'NONE',  ( 0.3996062992125986035, 0.1070741851644054776, -0.9120734908136483021 ) ) ;
#12067=CARTESIAN_POINT ( 'NONE',  ( 0.2891555358219910499, -0.2891555358219909944, -0.4133858267716535861 ) ) ;
#12074=CARTESIAN_POINT ( 'NONE',  ( -0.2891555358219911054, 0.2891555358219909388, -1.356299212598425230 ) ) ;
#12079=CARTESIAN_POINT ( 'NONE',  ( 0.4091458600556403535, 0.2362204724409449896, -1.548556430446194287 ) ) ;
#12080=CARTESIAN_POINT ( 'NONE',  ( -0.2925321140481930704, -0.2925321140481933480, -2.578740157480315265 ) ) ;
#12094=CARTESIAN_POINT ( 'NONE',  ( -0.1049643490035302024, -0.3917322834645671215, -1.324146981627296826 ) ) ;
#12097=CARTESIAN_POINT ( 'NONE',  ( -0.1974969037888706647, 0.3420746716998658843, -1.430446194225722056 ) ) ;
#12098=EDGE_LOOP ( 'NONE', ( #48182, #39828, #41598, #2062 ) ) ;
#12102=CARTESIAN_POINT ( 'NONE',  ( -0.2925321140481932924, 0.2925321140481931814, -0.1771653543307086520 ) ) ;
#12109=CARTESIAN_POINT ( 'NONE',  ( -0.3917322834645670104, -7.196005306013484475E-17, 0.03346456692913377107 ) ) ;
#12114=ORIENTED_EDGE ( 'NONE', *, *, #1376, .F. ) ;
#12115=CARTESIAN_POINT ( 'NONE',  ( 0.1070741851644053527, 0.3996062992125986590, -2.040682414698162361 ) ) ;
#12118=CARTESIAN_POINT ( 'NONE',  ( 0.2925321140481932369, -0.2925321140481931814, -1.592519685039370358 ) ) ;
#12123=CARTESIAN_POINT ( 'NONE',  ( 0.3458507752293908943, -0.3458507752293908943, -0.7283464566929134243 ) ) ;
#12126=CARTESIAN_POINT ( 'NONE',  ( 0.3392501089628018329, 0.1958661417322835607, 0.03412073490813653104 ) ) ;
#12128=CARTESIAN_POINT ( 'NONE',  ( -0.1049643490035307020, 0.3917322834645669549, -2.138451443569553412 ) ) ;
#12132=CARTESIAN_POINT ( 'NONE',  ( -0.4091458600556402980, -0.2362204724409451284, -2.648950131233595684 ) ) ;
#12135=CARTESIAN_POINT ( 'NONE',  ( 0.3949938075777408852, 0.1058382717557500435, -2.091207349081364519 ) ) ;
#12140=CARTESIAN_POINT ( 'NONE',  ( 0.3458507752293908943, -0.3458507752293908943, -2.222440944881889813 ) ) ;
#12158=CARTESIAN_POINT ( 'NONE',  ( 0.3996062992125985480, 2.446882876249141654E-17, -0.6673228346456693272 ) ) ;
#12159=CARTESIAN_POINT ( 'NONE',  ( 0.1958661417322834775, 0.3392501089628018884, -2.118766404199475151 ) ) ;
#12169=CARTESIAN_POINT ( 'NONE',  ( -0.2867679344610367109, 0.2867679344610365444, -1.906187294784464026 ) ) ;
#12175=CARTESIAN_POINT ( 'NONE',  ( -0.3917322834645669549, -0.1049643490035306603, -1.862860892388451761 ) ) ;
#12179=CARTESIAN_POINT ( 'NONE',  ( -0.4091458600556405756, 0.2362204724409446288, -0.4986876640419947715 ) ) ;
#12183=CARTESIAN_POINT ( 'NONE',  ( -0.1070741851644056997, 0.3996062992125986035, -0.7939632545931758489 ) ) ;
#12185=CARTESIAN_POINT ( 'NONE',  ( -9.594673741351313045E-17, 0.3917322834645670104, -2.511811023622047223 ) ) ;
#12198=CARTESIAN_POINT ( 'NONE',  ( 0.1049643490035303689, 0.3917322834645670104, -0.1430446194225721002 ) ) ;
#12201=CARTESIAN_POINT ( 'NONE',  ( 0.1058382717557500713, -0.3949938075777409408, -0.4002624671916010235 ) ) ;
#12209=CARTESIAN_POINT ( 'NONE',  ( 0.3917322834645670104, 0.1049643490035304660, -1.853693856464253997 ) ) ;
#12211=CARTESIAN_POINT ( 'NONE',  ( 0.2867679344610365999, 0.2867679344610365999, -2.584645669291338876 ) ) ;
#12217=CARTESIAN_POINT ( 'NONE',  ( -0.3996062992125986035, -7.340648628747425578E-17, -0.6692913385826770867 ) ) ;
#12219=CARTESIAN_POINT ( 'NONE',  ( 0.3996062992125986035, -0.1070741851644052972, -0.5032808398950130435 ) ) ;
#12220=CARTESIAN_POINT ( 'NONE',  ( -0.2925321140481932369, 0.2925321140481931259, -0.09645669291338584972 ) ) ;
#12222=CARTESIAN_POINT ( 'NONE',  ( -0.3996062992125986035, -7.340648628747425578E-17, -2.874015748031495843 ) ) ;
#12223=CARTESIAN_POINT ( 'NONE',  ( -0.3917322834645669549, -0.1049643490035306603, -1.705380577427821898 ) ) ;
#12228=CARTESIAN_POINT ( 'NONE',  ( -0.4724409448818895907, -0.1265901696524993070, -1.697506561679789971 ) ) ;
#12231=CARTESIAN_POINT ( 'NONE',  ( 0.3420746716998660508, -0.1974969037888704149, -0.8116797900262466836 ) ) ;
#12241=CARTESIAN_POINT ( 'NONE',  ( 0.1998031496062994128, -0.3460692066303957537, -1.900918635170603999 ) ) ;
#12255=CARTESIAN_POINT ( 'NONE',  ( -0.1958661417322834220, -0.3392501089628018884, -0.9376640419947508409 ) ) ;
#12263=DIRECTION ( 'NONE',  ( 0.000000000000000000, 0.000000000000000000, 1.000000000000000000 ) ) ;
#12274=CARTESIAN_POINT ( 'NONE',  ( -0.3392501089628019995, 0.1958661417322832277, -2.065616797900262647 ) ) ;
#12278=CARTESIAN_POINT ( 'NONE',  ( -0.3458507752293906723, -0.3458507752293910609, -0.2165354330708661734 ) ) ;
#12280=CARTESIAN_POINT ( 'NONE',  ( -9.674558042662121740E-17, 0.3949938075777409963, -2.677165354330708347 ) ) ;
#12281=ORIENTED_EDGE ( 'NONE', *, *, #17250, .T. ) ;
#12283=CARTESIAN_POINT ( 'NONE',  ( 0.1958661417322836440, -0.3392501089628017219, -1.501312335958005173 ) ) ;
#12285=CARTESIAN_POINT ( 'NONE',  ( 0.009287274676459343278, 0.3937527723457945328, -2.755905511811026276 ) ) ;
#12292=CARTESIAN_POINT ( 'NONE',  ( -0.3392501089628018329, -0.1958661417322836440, -0.9199281907798407820 ) ) ;
#12297=PLANE ( 'NONE',  #48961 ) ;
#12299=CARTESIAN_POINT ( 'NONE',  ( -0.2867679344610365444, -0.2867679344610367664, -1.945557373524620992 ) ) ;
#12306=CARTESIAN_POINT ( 'NONE',  ( 0.3917322834645670104, -0.1049643490035303411, -1.298556430446194510 ) ) ;
#12311=CARTESIAN_POINT ( 'NONE',  ( -5.237264738830231135E-17, 0.3992723400743281581, -1.920830620545185538E-17 ) ) ;
#12315=CARTESIAN_POINT ( 'NONE',  ( 0.3917322834645670104, -0.1049643490035303411, -2.623359580052493367 ) ) ;
#12322=CARTESIAN_POINT ( 'NONE',  ( 0.2867679344610365999, 0.2867679344610365999, -1.009842519685039353 ) ) ;
#12326=CARTESIAN_POINT ( 'NONE',  ( -0.2925321140481932369, 0.2925321140481931259, -2.773622047244094002 ) ) ;
#12337=CARTESIAN_POINT ( 'NONE',  ( 0.3460692066303958092, 0.1998031496062993018, -0.6804461942257218343 ) ) ;
#12339=CARTESIAN_POINT ( 'NONE',  ( 0.1958661417322836440, -0.3392501089628017219, -0.2414698162729658204 ) ) ;
#12341=DIRECTION ( 'NONE',  ( 0.000000000000000000, 0.000000000000000000, 1.000000000000000000 ) ) ;
#12353=CARTESIAN_POINT ( 'NONE',  ( 0.3917322834645670104, 0.1049643490035304660, -0.7513316517398445082 ) ) ;
#12357=CARTESIAN_POINT ( 'NONE',  ( -0.4091458600556402980, -0.2362204724409451284, -2.333989501312335957 ) ) ;
#12375=CARTESIAN_POINT ( 'NONE',  ( 0.1070741851644054915, -0.3996062992125985480, -0.4002624671916010235 ) ) ;
#12376=CARTESIAN_POINT ( 'NONE',  ( -9.787531504996566615E-17, 0.3996062992125985480, -2.438976377952756014 ) ) ;
#12381=CARTESIAN_POINT ( 'NONE',  ( 0.3996062992125986035, 2.446882876249141962E-17, -2.322834645669291209 ) ) ;
#12382=CARTESIAN_POINT ( 'NONE',  ( -0.3420746716998661618, 0.1974969037888702206, -1.443569553805774230 ) ) ;
#12383=CARTESIAN_POINT ( 'NONE',  ( -0.2925321140481930704, -0.2925321140481933480, -2.736220472440944018 ) ) ;
#12385=CARTESIAN_POINT ( 'NONE',  ( 0.3392501089628018884, -0.1958661417322834220, -0.7270341207349080292 ) ) ;
#12389=CARTESIAN_POINT ( 'NONE',  ( -0.3420746716998660508, -0.1974969037888706924, -2.491469816272965598 ) ) ;
#12393=CARTESIAN_POINT ( 'NONE',  ( 0.2362204724409449064, 0.4091458600556404646, -2.821522309711286258 ) ) ;
#12394=CARTESIAN_POINT ( 'NONE',  ( 0.2925321140481932369, -0.2925321140481932369, -2.145669291338581974 ) ) ;
#12400=CARTESIAN_POINT ( 'NONE',  ( 0.3392501089628018329, 0.1958661417322835607, -0.2158792650918636147 ) ) ;
#12408=CARTESIAN_POINT ( 'NONE',  ( 0.1958661417322834775, 0.3392501089628018884, -0.3864829396325459854 ) ) ;
#12409=CARTESIAN_POINT ( 'NONE',  ( 0.3917322834645669549, 0.1049643490035304660, -1.534120734908136052 ) ) ;
#12410=CARTESIAN_POINT ( 'NONE',  ( -9.594673741351313045E-17, 0.3917322834645670104, -2.511811023622047223 ) ) ;
#12412=CARTESIAN_POINT ( 'NONE',  ( -0.3460692066303960868, 0.1998031496062990242, -0.1837270341207349333 ) ) ;
#12416=CARTESIAN_POINT ( 'NONE',  ( 0.3460692066303959202, 0.1998031496062993295, -1.391076115485564424 ) ) ;
#12422=CARTESIAN_POINT ( 'NONE',  ( -0.2867679344610365999, 0.2867679344610364889, -0.8917322834645667884 ) ) ;
#12428=ORIENTED_EDGE ( 'NONE', *, *, #64537, .F. ) ;
#12430=CARTESIAN_POINT ( 'NONE',  ( 0.2362204724409451007, -0.4091458600556402980, -1.981627296587926690 ) ) ;
#12435=ORIENTED_EDGE ( 'NONE', *, *, #63766, .F. ) ;
#12440=CARTESIAN_POINT ( 'NONE',  ( 0.3392501089628018329, 0.1958661417322835052, -0.2112667734570061184 ) ) ;
#12443=CARTESIAN_POINT ( 'NONE',  ( -0.2867679344610364334, -0.2867679344610367109, -0.7736220472440945573 ) ) ;
#12448=CARTESIAN_POINT ( 'NONE',  ( -0.2867679344610365999, 0.2867679344610364889, -2.846456692913385655 ) ) ;
#12451=CARTESIAN_POINT ( 'NONE',  ( 0.4091458600556403535, 0.2362204724409449896, -0.9954068241469815614 ) ) ;
#12463=CARTESIAN_POINT ( 'NONE',  ( -0.1070741851644056997, 0.3996062992125984925, -2.288057742782152015 ) ) ;
#12467=CARTESIAN_POINT ( 'NONE',  ( 4.893765752498283308E-17, -0.3996062992125985480, -1.257874015748031482 ) ) ;
#12473=CARTESIAN_POINT ( 'NONE',  ( 0.2925321140481931814, -0.2925321140481931259, -0.8051181102362204856 ) ) ;
#12474=CARTESIAN_POINT ( 'NONE',  ( 0.2925321140481932369, 0.2925321140481932369, -0.9251968503937008093 ) ) ;
#12475=CARTESIAN_POINT ( 'NONE',  ( 0.1974969037888706369, -0.3420746716998659953, -0.09186351706036749443 ) ) ;
#12481=CARTESIAN_POINT ( 'NONE',  ( 0.3949938075777408852, 0.1058382717557500435, -1.303805774278215424 ) ) ;
#12486=CARTESIAN_POINT ( 'NONE',  ( -0.4091458600556402980, -0.2362204724409451284, -1.627296587926509330 ) ) ;
#12487=CARTESIAN_POINT ( 'NONE',  ( -0.2925321140481932369, 0.2925321140481931814, -2.539370078740157410 ) ) ;
#12489=ORIENTED_EDGE ( 'NONE', *, *, #53092, .T. ) ;
#12495=CARTESIAN_POINT ( 'NONE',  ( 0.3917322834645668994, 0.1049643490035304522, -2.094468873194538450 ) ) ;
#12503=CARTESIAN_POINT ( 'NONE',  ( 0.2867679344610365999, -0.2867679344610365444, -1.350393700787401619 ) ) ;
#12506=CARTESIAN_POINT ( 'NONE',  ( -0.1974969037888703871, -0.3420746716998661063, -1.955380577427821454 ) ) ;
#12511=CARTESIAN_POINT ( 'NONE',  ( 0.1070741851644054915, -0.3996062992125986035, -0.2427821522309711322 ) ) ;
#12518=CARTESIAN_POINT ( 'NONE',  ( -0.3917322834645669549, -0.1049643490035306603, 0.1843832020997374643 ) ) ;
#12523=ORIENTED_EDGE ( 'NONE', *, *, #60460, .F. ) ;
#12525=CARTESIAN_POINT ( 'NONE',  ( -0.2925321140481930149, -0.2925321140481933480, -2.025590551181101873 ) ) ;
#12530=CARTESIAN_POINT ( 'NONE',  ( 0.4091458600556403535, 0.2362204724409449896, -0.9186351706036745002 ) ) ;
#12533=CARTESIAN_POINT ( 'NONE',  ( 0.2867679344610365999, -0.2867679344610365444, -0.09055118110236216877 ) ) ;
#12535=CARTESIAN_POINT ( 'NONE',  ( 0.1049643490035303689, 0.3917322834645670104, -2.125328083989501238 ) ) ;
#12539=CARTESIAN_POINT ( 'NONE',  ( -0.4724409448818899238, 0.1265901696524986686, -2.786745406824146620 ) ) ;
#12543=CARTESIAN_POINT ( 'NONE',  ( -0.2891555358219909388, -0.2891555358219912164, -2.340551181102362488 ) ) ;
#12553=CARTESIAN_POINT ( 'NONE',  ( -0.4724409448818895907, -0.1265901696524993070, -0.1227034120734908362 ) ) ;
#12566=CARTESIAN_POINT ( 'NONE',  ( 0.1070741851644053388, 0.3996062992125986035, -1.172572178477690352 ) ) ;
#12567=CARTESIAN_POINT ( 'NONE',  ( -9.594673741351313045E-17, 0.3917322834645670104, -2.289370078740157410 ) ) ;
#12578=CARTESIAN_POINT ( 'NONE',  ( -0.2867679344610367109, 0.2867679344610365444, -2.063667609745093667 ) ) ;
#12585=CARTESIAN_POINT ( 'NONE',  ( -9.594673741351313045E-17, 0.3917322834645670104, -1.816929133858267820 ) ) ;
#12590=CARTESIAN_POINT ( 'NONE',  ( -0.2925321140481932369, 0.2925321140481930704, -2.616141732283464361 ) ) ;
#12592=CARTESIAN_POINT ( 'NONE',  ( 0.3996062992125986035, 0.1070741851644054776, -1.227034120734908029 ) ) ;
#12594=CARTESIAN_POINT ( 'NONE',  ( -9.594673741351313045E-17, 0.3917322834645670659, 0.1607418390738039049 ) ) ;
#12608=CARTESIAN_POINT ( 'NONE',  ( 0.2867679344610365999, -0.2867679344610365444, -0.09055118110236216877 ) ) ;
#12611=CARTESIAN_POINT ( 'NONE',  ( 0.1058382717557500713, -0.3949938075777409408, -0.7152230971128611392 ) ) ;
#12619=CARTESIAN_POINT ( 'NONE',  ( -0.1958661417322833942, -0.3392501089628018884, -1.794638738354017660 ) ) ;
#12621=CARTESIAN_POINT ( 'NONE',  ( -0.2867679344610364334, -0.2867679344610367109, -2.820866141732283339 ) ) ;
#12625=CARTESIAN_POINT ( 'NONE',  ( -0.2925321140481930704, -0.2925321140481933480, -0.8464566929133857665 ) ) ;
#12627=CARTESIAN_POINT ( 'NONE',  ( 0.3996062992125985480, 2.446882876249141654E-17, -0.3523622047244094335 ) ) ;
#12628=CARTESIAN_POINT ( 'NONE',  ( 0.2925321140481932369, 0.2925321140481932369, -0.2145669291338583029 ) ) ;
#12630=CARTESIAN_POINT ( 'NONE',  ( 0.1070741851644053527, 0.3996062992125986590, -2.828083989501312345 ) ) ;
#12631=CARTESIAN_POINT ( 'NONE',  ( 0.3917322834645670104, -0.1049643490035303411, -1.613517060367454237 ) ) ;
#12636=CARTESIAN_POINT ( 'NONE',  ( -0.4724409448818895907, -0.1265901696524993070, -1.540026246719159886 ) ) ;
#12639=CARTESIAN_POINT ( 'NONE',  ( -0.1974969037888706924, 0.3420746716998658843, -0.8772965879265093303 ) ) ;
#12642=DIRECTION ( 'NONE',  ( 0.000000000000000000, 0.000000000000000000, 1.000000000000000000 ) ) ;
#12649=CARTESIAN_POINT ( 'NONE',  ( 0.3996062992125984925, 0.1070741851644054637, -2.248687664041995049 ) ) ;
#12651=CARTESIAN_POINT ( 'NONE',  ( 0.3392501089628018329, 0.1958661417322835052, -1.471109293142045304 ) ) ;
#12667=CARTESIAN_POINT ( 'NONE',  ( -0.2867679344610365999, 0.2867679344610364889, -0.8917322834645667884 ) ) ;
#12689=CARTESIAN_POINT ( 'NONE',  ( 0.3392501089628018884, -0.1958661417322834220, -2.144356955380577467 ) ) ;
#12692=CARTESIAN_POINT ( 'NONE',  ( 0.2362204724409449064, 0.4091458600556404646, -0.3018372703412073310 ) ) ;
#12693=CARTESIAN_POINT ( 'NONE',  ( -0.2925321140481930704, -0.2925321140481933480, -0.05905511811023622659 ) ) ;
#12696=CARTESIAN_POINT ( 'NONE',  ( 0.1049643490035303689, 0.3917322834645670104, -1.875328083989501460 ) ) ;
#12698=CARTESIAN_POINT ( 'NONE',  ( -1.157146581871515012E-16, 0.4724409448818898682, -2.834645669291338432 ) ) ;
#12705=CARTESIAN_POINT ( 'NONE',  ( 0.3917322834645668994, -0.1049643490035303134, -0.8215029939294470340 ) ) ;
#12712=CARTESIAN_POINT ( 'NONE',  ( 0.3392501089628018329, 0.1958661417322835607, -2.017735851214910170 ) ) ;
#12719=CARTESIAN_POINT ( 'NONE',  ( -0.2867679344610364334, -0.2867679344610367109, -1.246062992125984481 ) ) ;
#12724=CARTESIAN_POINT ( 'NONE',  ( -0.01218835185196217967, 0.3960428127060656167, -1.229201864173550318E-17 ) ) ;
#12734=CARTESIAN_POINT ( 'NONE',  ( 0.000000000000000000, 0.000000000000000000, -1.929133858267716661 ) ) ;
#12735=CARTESIAN_POINT ( 'NONE',  ( -0.3392501089628019995, 0.1958661417322832277, -1.055774278215223294 ) ) ;
#12736=CARTESIAN_POINT ( 'NONE',  ( -0.2362204724409451284, 0.4091458600556402425, -0.08989501312335958227 ) ) ;
#12740=CARTESIAN_POINT ( 'NONE',  ( 0.3949938075777409408, -0.1058382717557499186, 0.1266404199475065773 ) ) ;
#12745=CARTESIAN_POINT ( 'NONE',  ( 0.3420746716998660508, 0.1974969037888705814, -0.2080052493438320771 ) ) ;
#12749=CARTESIAN_POINT ( 'NONE',  ( 0.3917322834645670104, 2.398668435337828261E-17, -2.722440944881889369 ) ) ;
#12753=CARTESIAN_POINT ( 'NONE',  ( 0.2925321140481932369, 0.2925321140481932369, -1.001968503937007871 ) ) ;
#12755=CARTESIAN_POINT ( 'NONE',  ( -0.1049643490035302024, -0.3917322834645671215, -0.2217847769028870319 ) ) ;
#12769=CARTESIAN_POINT ( 'NONE',  ( 0.1958661417322834775, 0.3392501089628018884, -0.7710166911099232134 ) ) ;
#12773=CARTESIAN_POINT ( 'NONE',  ( 0.4091458600556403535, 0.2362204724409449896, -2.412729658792650778 ) ) ;
#12791=CARTESIAN_POINT ( 'NONE',  ( -0.2925321140481930704, -0.2925321140481933480, -0.5314960629921260393 ) ) ;
#12792=CARTESIAN_POINT ( 'NONE',  ( -0.3996062992125986590, 0.1070741851644051723, -2.471784776902887337 ) ) ;
#12797=CARTESIAN_POINT ( 'NONE',  ( -0.1998031496062994683, 0.3460692066303958092, -2.060367454068241511 ) ) ;
#12799=CARTESIAN_POINT ( 'NONE',  ( 4.837279021331060870E-17, -0.3949938075777409963, -1.653543307086614123 ) ) ;
#12800=CARTESIAN_POINT ( 'NONE',  ( 0.3996062992125986035, 2.446882876249141962E-17, -2.795275590551181022 ) ) ;
#12801=CARTESIAN_POINT ( 'NONE',  ( 0.1265901696524989184, 0.4724409448818898127, -2.513123359580052174 ) ) ;
#12802=CARTESIAN_POINT ( 'NONE',  ( -0.3392501089628017219, -0.1958661417322836718, -1.146981627296587813 ) ) ;
#12806=CARTESIAN_POINT ( 'NONE',  ( 0.3949938075777409963, 2.418639510665530743E-17, -2.557086614173228689 ) ) ;
#12811=CARTESIAN_POINT ( 'NONE',  ( 0.3996062992125986035, 2.446882876249141962E-17, -2.007874015748031482 ) ) ;
#12812=CARTESIAN_POINT ( 'NONE',  ( -0.1049643490035302301, -0.3917322834645671770, -0.8563185283802644543 ) ) ;
#12818=CARTESIAN_POINT ( 'NONE',  ( -0.2867679344610365999, 0.2867679344610364889, 0.05314960629921249707 ) ) ;
#12826=CARTESIAN_POINT ( 'NONE',  ( 0.3392501089628018329, 0.1958661417322835607, -0.5308398950131234528 ) ) ;
#12827=CARTESIAN_POINT ( 'NONE',  ( 0.3917322834645670104, 2.398668435337828261E-17, -1.685039370078740051 ) ) ;
#12828=CARTESIAN_POINT ( 'NONE',  ( -0.3392501089628017219, -0.1958661417322836718, -2.721784776902886893 ) ) ;
#12829=VERTEX_POINT ( 'NONE', #32518 ) ;
#12830=CARTESIAN_POINT ( 'NONE',  ( -0.3460692066303958092, -0.1998031496062994683, -0.2099737532808399199 ) ) ;
#12834=CARTESIAN_POINT ( 'NONE',  ( 0.3460692066303959202, 0.1998031496062993295, -1.548556430446194287 ) ) ;
#12839=CARTESIAN_POINT ( 'NONE',  ( 0.3917322834645669549, 0.1049643490035304660, -0.9967191601049870675 ) ) ;
#12848=CARTESIAN_POINT ( 'NONE',  ( 0.1265901696524989462, 0.4724409448818897572, -2.040682414698162361 ) ) ;
#12859=CARTESIAN_POINT ( 'NONE',  ( -0.1049643490035306742, 0.3917322834645668994, -0.7165161172890270880 ) ) ;
#12860=ADVANCED_FACE ( 'NONE', ( #24545 ), #44705, .T. ) ;
#12862=CARTESIAN_POINT ( 'NONE',  ( -0.2867679344610366554, 0.2867679344610365444, -0.8917322834645667884 ) ) ;
#12867=CARTESIAN_POINT ( 'NONE',  ( 0.3392501089628018329, 0.1958661417322835607, -2.800524934383201714 ) ) ;
#12870=CARTESIAN_POINT ( 'NONE',  ( -0.4091458600556402980, -0.2362204724409451284, -1.231627296587926468 ) ) ;
#12882=CARTESIAN_POINT ( 'NONE',  ( 0.1070741851644053388, 0.3996062992125986035, -2.274934383202099397 ) ) ;
#12886=CARTESIAN_POINT ( 'NONE',  ( -0.3996062992125984925, -0.1070741851644056858, -1.225065616797899937 ) ) ;
#12893=CARTESIAN_POINT ( 'NONE',  ( 0.3996062992125985480, 2.446882876249141654E-17, -0.6673228346456693272 ) ) ;
#12894=CARTESIAN_POINT ( 'NONE',  ( 0.1998031496062992740, 0.3460692066303959757, -0.7742782152230971437 ) ) ;
#12895=CARTESIAN_POINT ( 'NONE',  ( -0.2891555358219911054, 0.2891555358219909388, -0.3346456692913387099 ) ) ;
#12901=CARTESIAN_POINT ( 'NONE',  ( 0.1974969037888706092, -0.3420746716998660508, -1.270997375328083878 ) ) ;
#12906=CARTESIAN_POINT ( 'NONE',  ( 0.2362204724409451007, -0.4091458600556402980, -1.666666666666666741 ) ) ;
#12907=CARTESIAN_POINT ( 'NONE',  ( -0.3996062992125986035, -7.340648628747425578E-17, -2.559055118110236560 ) ) ;
#12908=AXIS2_PLACEMENT_3D ( 'NONE', #12734, #51004, #19036 ) ;
#12910=ORIENTED_EDGE ( 'NONE', *, *, #71814, .T. ) ;
#12916=CARTESIAN_POINT ( 'NONE',  ( 0.1049643490035304522, -0.3917322834645668994, -1.897618479493751398 ) ) ;
#12917=CARTESIAN_POINT ( 'NONE',  ( 0.1070741851644053388, 0.3996062992125986035, -2.747375328083988766 ) ) ;
#12922=CARTESIAN_POINT ( 'NONE',  ( -0.1958661417322834220, -0.3392501089628018884, -1.632545931758530244 ) ) ;
#12924=ORIENTED_EDGE ( 'NONE', *, *, #33021, .T. ) ;
#12925=CARTESIAN_POINT ( 'NONE',  ( -0.1058382717557503211, 0.3949938075777409408, -1.896325459317585116 ) ) ;
#12930=CARTESIAN_POINT ( 'NONE',  ( -0.3460692066303958092, -0.1998031496062994683, -0.2099737532808398921 ) ) ;
#12933=( CONVERSION_BASED_UNIT ( 'INCH', #26382 ) LENGTH_UNIT ( ) NAMED_UNIT ( #56145 ) );
#12938=CARTESIAN_POINT ( 'NONE',  ( -0.3917322834645671215, 0.1049643490035301469, -0.4324146981627298159 ) ) ;
#12945=CARTESIAN_POINT ( 'NONE',  ( -0.3460692066303960313, 0.1998031496062989965, -1.992782152230971437 ) ) ;
#12950=CARTESIAN_POINT ( 'NONE',  ( 0.1265901696524990294, -0.4724409448818896462, -0.8727034120734907807 ) ) ;
#12952=CARTESIAN_POINT ( 'NONE',  ( -0.2867679344610364334, -0.2867679344610367109, -0.5236220472440944462 ) ) ;
#12958=CARTESIAN_POINT ( 'NONE',  ( 0.4724409448818897572, -0.1265901696524988906, -2.865485564304462329 ) ) ;
#12962=CARTESIAN_POINT ( 'NONE',  ( 0.1974969037888706092, -0.3420746716998660508, -2.530839895013123453 ) ) ;
#12970=CARTESIAN_POINT ( 'NONE',  ( 0.3917322834645670104, 2.398668435337828261E-17, -1.685039370078740051 ) ) ;
#12974=CARTESIAN_POINT ( 'NONE',  ( -0.4091458600556402980, -0.2362204724409451284, -0.1292650918635170620 ) ) ;
#12985=ADVANCED_FACE ( 'NONE', ( #75500 ), #11931, .F. ) ;
#12987=CARTESIAN_POINT ( 'NONE',  ( 0.1998031496062992463, 0.3460692066303959202, -1.323490813648294129 ) ) ;
#12988=CARTESIAN_POINT ( 'NONE',  ( 0.3392501089628018884, -0.1958661417322834220, -2.551837270341207109 ) ) ;
#12998=CARTESIAN_POINT ( 'NONE',  ( 0.3458507752293908943, -0.3458507752293908943, -0.7283464566929134243 ) ) ;
#12999=CARTESIAN_POINT ( 'NONE',  ( -0.3917322834645670104, -0.1049643490035307020, -2.089914328905198904 ) ) ;
#13000=ORIENTED_EDGE ( 'NONE', *, *, #52169, .F. ) ;
#13005=CARTESIAN_POINT ( 'NONE',  ( -0.3917322834645671215, 0.1049643490035301469, -2.164698162729658648 ) ) ;
#13010=CYLINDRICAL_SURFACE ( 'NONE', #36887, 0.4724409448818898682 ) ;
#13014=CARTESIAN_POINT ( 'NONE',  ( 0.1070741851644054915, -0.3996062992125986035, -1.345144356955380704 ) ) ;
#13016=CARTESIAN_POINT ( 'NONE',  ( -0.2867679344610367109, 0.2867679344610365444, 0.1410567997037251442 ) ) ;
#13029=( BOUNDED_CURVE ( )  B_SPLINE_CURVE ( 2, ( #20420, #27974, #648, #26726, #27557, #1897, #46488, #77671, #78512, #58708, #39349, #52380, #14541 ),
 .UNSPECIFIED., .F., .F. ) 
 B_SPLINE_CURVE_WITH_KNOTS ( ( 3, 2, 2, 2, 2, 2, 3 ),
 ( 0.2875000000000000333, 0.2916666666666667407, 0.2958333333333333925, 0.3000000000000000444, 0.3041666666666666408, 0.3083333333333333481, 0.3125000000000000000 ),
 .UNSPECIFIED. ) 
 CURVE ( )  GEOMETRIC_REPRESENTATION_ITEM ( )  RATIONAL_B_SPLINE_CURVE ( ( 0.9999999999999995559, 0.9659258262890687563, 1.000000000000000000, 0.9659258262890683122, 1.000000000000000000, 0.9659258262890683122, 1.000000000000000000, 0.9659258262890683122, 1.000000000000000000, 0.9659258262890683122, 1.000000000000000000, 0.9659258262890683122, 1.000000000000000000 ) ) 
 REPRESENTATION_ITEM ( '' )  );
#13031=CARTESIAN_POINT ( 'NONE',  ( -0.3917322834645670104, -7.196005306013484475E-17, -0.3464566929133857665 ) ) ;
#13034=CARTESIAN_POINT ( 'NONE',  ( 0.1058382717557499880, 0.3949938075777411073, -0.4658792650918635592 ) ) ;
#13041=CARTESIAN_POINT ( 'NONE',  ( -0.2867679344610367109, 0.2867679344610365444, -1.748706979823833718 ) ) ;
#13047=CARTESIAN_POINT ( 'NONE',  ( -0.1998031496062994683, 0.3460692066303958092, -1.430446194225721834 ) ) ;
#13049=CARTESIAN_POINT ( 'NONE',  ( -0.3460692066303960313, 0.1998031496062989965, -0.8904199475065617264 ) ) ;
#13050=CARTESIAN_POINT ( 'NONE',  ( -0.3996062992125984925, -0.1070741851644056858, -0.2801837270341207553 ) ) ;
#13052=CARTESIAN_POINT ( 'NONE',  ( 0.2925321140481932369, 0.2925321140481932369, -2.657480314960630530 ) ) ;
#13053=CARTESIAN_POINT ( 'NONE',  ( 0.1958661417322834775, 0.3392501089628018884, -1.488845144356955252 ) ) ;
#13059=CARTESIAN_POINT ( 'NONE',  ( 0.4724409448818897572, -0.1265901696524988906, -1.605643044619422977 ) ) ;
#13062=CARTESIAN_POINT ( 'NONE',  ( 0.1058382717557500852, -0.3949938075777408852, -1.421916010498688099 ) ) ;
#13072=CIRCLE ( 'NONE', #19793, 0.4724409448818898682 ) ;
#13073=CARTESIAN_POINT ( 'NONE',  ( -0.1998031496062994405, 0.3460692066303957537, -2.137139107611548905 ) ) ;
#13076=CARTESIAN_POINT ( 'NONE',  ( 0.3917322834645668994, -0.1049643490035303134, -1.766384883693226771 ) ) ;
#13085=CARTESIAN_POINT ( 'NONE',  ( 0.4724409448818898682, 2.892866454678787531E-17, -2.322834645669291209 ) ) ;
#13089=CARTESIAN_POINT ( 'NONE',  ( -9.787531504996566615E-17, 0.3996062992125985480, 0.2381889763779527491 ) ) ;
#13091=CARTESIAN_POINT ( 'NONE',  ( 0.3392501089628018884, -0.1958661417322834220, -1.134514435695538115 ) ) ;
#13110=CARTESIAN_POINT ( 'NONE',  ( 0.3392501089628018329, 0.1958661417322835607, -2.328083989501312345 ) ) ;
#13114=CARTESIAN_POINT ( 'NONE',  ( -0.1265901696524993347, 0.4724409448818895907, -0.9514435695538056015 ) ) ;
#13115=CARTESIAN_POINT ( 'NONE',  ( 0.2925321140481932369, 0.2925321140481932369, -0.1377952755905512139 ) ) ;
#13118=CARTESIAN_POINT ( 'NONE',  ( -0.3392501089628017219, -0.1958661417322836718, -1.619422572178477848 ) ) ;
#13123=CARTESIAN_POINT ( 'NONE',  ( 0.1265901696524989462, 0.4724409448818897572, -2.828083989501312345 ) ) ;
#13130=CARTESIAN_POINT ( 'NONE',  ( -0.3392501089628019439, 0.1958661417322832554, -1.208642101540995606 ) ) ;
#13137=CARTESIAN_POINT ( 'NONE',  ( -0.1958661417322833942, -0.3392501089628018884, -2.267079683235907694 ) ) ;
#13146=CARTESIAN_POINT ( 'NONE',  ( -0.1958661417322834220, -0.3392501089628018884, -1.252624671916010568 ) ) ;
#13162=CARTESIAN_POINT ( 'NONE',  ( 0.4724409448818896462, 0.1265901696524990294, -0.04396325459317586282 ) ) ;
#13165=CARTESIAN_POINT ( 'NONE',  ( 0.1998031496062994128, -0.3460692066303957537, -2.688320209973753538 ) ) ;
#13170=CARTESIAN_POINT ( 'NONE',  ( -0.3949938075777411073, 0.1058382717557497660, 0.04790026246719160385 ) ) ;
#13177=EDGE_CURVE ( 'NONE', #2851, #51988, #5888, .T. ) ;
#13178=CARTESIAN_POINT ( 'NONE',  ( 0.3460692066303959202, -0.1998031496062991630, -0.9691601049868766582 ) ) ;
#13180=CARTESIAN_POINT ( 'NONE',  ( 0.3917322834645670104, 2.398668435337828261E-17, -0.7401574803149605364 ) ) ;
#13198=CARTESIAN_POINT ( 'NONE',  ( -0.3458507752293906723, -0.3458507752293910609, -2.498031496062992574 ) ) ;
#13215=CARTESIAN_POINT ( 'NONE',  ( 0.3996062992125985480, 0.1070741851644054637, -0.4396325459317584894 ) ) ;
#13221=CARTESIAN_POINT ( 'NONE',  ( -0.3996062992125986035, -0.1070741851644056997, -2.723097112860892288 ) ) ;
#13222=CARTESIAN_POINT ( 'NONE',  ( -0.3949938075777411628, 0.1058382717557497937, -1.765091863517060267 ) ) ;
#13223=CARTESIAN_POINT ( 'NONE',  ( -0.3917322834645669549, -0.1049643490035306603, -0.5104986876640419391 ) ) ;
#13225=CARTESIAN_POINT ( 'NONE',  ( 0.3917322834645670104, -0.1049643490035303273, -0.8910761154855640909 ) ) ;
#13228=CARTESIAN_POINT ( 'NONE',  ( -0.3917322834645670659, 0.1049643490035301607, 0.2021190533146474677 ) ) ;
#13232=CARTESIAN_POINT ( 'NONE',  ( 0.4724409448818896462, 0.1265901696524990294, -2.801837270341207553 ) ) ;
#13233=CARTESIAN_POINT ( 'NONE',  ( 0.1998031496062992740, 0.3460692066303959757, -2.664041994750656173 ) ) ;
#13234=CARTESIAN_POINT ( 'NONE',  ( -9.594673741351313045E-17, 0.3917322834645670659, -1.099100680611235559 ) ) ;
#13241=CARTESIAN_POINT ( 'NONE',  ( 0.1049643490035304938, -0.3917322834645669549, -0.01246719160104995359 ) ) ;
#13249=CARTESIAN_POINT ( 'NONE',  ( 0.1049643490035303689, 0.3917322834645670104, -0.5505249343832020470 ) ) ;
#13250=CARTESIAN_POINT ( 'NONE',  ( -0.1958661417322834220, -0.3392501089628018884, -1.947506561679789971 ) ) ;
#13251=CARTESIAN_POINT ( 'NONE',  ( -0.1049643490035302024, -0.3917322834645671215, -2.898950131233595684 ) ) ;
#13253=CARTESIAN_POINT ( 'NONE',  ( 0.1998031496062992740, 0.3460692066303959757, 0.01312335958005247417 ) ) ;
#13257=CARTESIAN_POINT ( 'NONE',  ( -0.2925321140481930704, -0.2925321140481933480, -1.633858267716534973 ) ) ;
#13261=CARTESIAN_POINT ( 'NONE',  ( -9.594673741351313045E-17, 0.3917322834645670104, -0.7145669291338584417 ) ) ;
#13269=CARTESIAN_POINT ( 'NONE',  ( 0.000000000000000000, 0.000000000000000000, -2.755905511811024056 ) ) ;
#13273=ORIENTED_EDGE ( 'NONE', *, *, #74631, .T. ) ;
#13274=CARTESIAN_POINT ( 'NONE',  ( 0.4724409448818898682, 2.892866454678787531E-17, -2.557086614173228689 ) ) ;
#13278=CARTESIAN_POINT ( 'NONE',  ( 0.1958661417322834497, 0.3392501089628018329, -0.6968310779189482718 ) ) ;
#13281=CARTESIAN_POINT ( 'NONE',  ( -0.2867679344610364334, -0.2867679344610367109, -1.088582677165354173 ) ) ;
#13286=CARTESIAN_POINT ( 'NONE',  ( 0.2867679344610365999, 0.2867679344610365999, -2.807086614173227357 ) ) ;
#13289=CARTESIAN_POINT ( 'NONE',  ( 0.4724409448818896462, 0.1265901696524990294, -1.303805774278215202 ) ) ;
#13301=CARTESIAN_POINT ( 'NONE',  ( -0.3996062992125986590, 0.1070741851644051723, -2.471784776902887337 ) ) ;
#13305=CARTESIAN_POINT ( 'NONE',  ( 0.1070741851644054776, -0.3996062992125984925, -1.421916010498687877 ) ) ;
#13311=CARTESIAN_POINT ( 'NONE',  ( 0.1998031496062992463, 0.3460692066303959202, -0.8510498687664042050 ) ) ;
#13312=CARTESIAN_POINT ( 'NONE',  ( 0.2925321140481932369, 0.2925321140481932369, -0.7677165354330709457 ) ) ;
#13313=CARTESIAN_POINT ( 'NONE',  ( 0.3949938075777409408, 0.1058382717557500574, -0.7545931758530185496 ) ) ;
#13319=CARTESIAN_POINT ( 'NONE',  ( -0.1058382717557503072, 0.3949938075777408852, -1.343175853018372834 ) ) ;
#13324=CARTESIAN_POINT ( 'NONE',  ( 0.4091458600556404646, -0.2362204724409448231, -1.522309711286089273 ) ) ;
#13327=ORIENTED_EDGE ( 'NONE', *, *, #59249, .T. ) ;
#13332=CARTESIAN_POINT ( 'NONE',  ( -0.1049643490035306742, 0.3917322834645668994, -1.818878322013436355 ) ) ;
#13338=CARTESIAN_POINT ( 'NONE',  ( -0.2867679344610364334, -0.2867679344610367109, -1.311023622047244430 ) ) ;
#13341=CARTESIAN_POINT ( 'NONE',  ( 0.3949938075777411073, -0.1058382717557499464, -2.001312335958005395 ) ) ;
#13346=CARTESIAN_POINT ( 'NONE',  ( 0.3996062992125986590, -0.1070741851644053111, -0.1115485564304461857 ) ) ;
#13354=CARTESIAN_POINT ( 'NONE',  ( -0.3917322834645669549, -0.1049643490035306603, -0.2880577427821523484 ) ) ;
#13361=CARTESIAN_POINT ( 'NONE',  ( 0.1070741851644053388, 0.3996062992125986035, -2.117454068241469756 ) ) ;
#13366=CARTESIAN_POINT ( 'NONE',  ( -0.4091458600556405756, 0.2362204724409446288, -0.8136482939632546652 ) ) ;
#13368=CARTESIAN_POINT ( 'NONE',  ( 0.1958661417322836440, -0.3392501089628017219, -0.2414698162729658204 ) ) ;
#13369=CARTESIAN_POINT ( 'NONE',  ( -0.3392501089628017219, -0.1958661417322836718, -2.184383202099737797 ) ) ;
#13373=CARTESIAN_POINT ( 'NONE',  ( -9.787531504996566615E-17, 0.3996062992125985480, 0.2381889763779527491 ) ) ;
#13378=CARTESIAN_POINT ( 'NONE',  ( 0.2891555358219910499, 0.2891555358219910499, -2.734251968503936592 ) ) ;
#13385=UNCERTAINTY_MEASURE_WITH_UNIT (LENGTH_MEASURE( 1.000000000000000082E-05 ), #28477, 'distance_accuracy_value', 'NONE');
#13387=CARTESIAN_POINT ( 'NONE',  ( -9.594673741351313045E-17, 0.3917322834645670104, -1.409448818897637734 ) ) ;
#13390=CARTESIAN_POINT ( 'NONE',  ( -0.3458507752293909498, 0.3458507752293907833, 0.2185039370078740162 ) ) ;
#13402=CARTESIAN_POINT ( 'NONE',  ( -0.3996062992125986590, 0.1070741851644051723, -1.054461942257217899 ) ) ;
#13403=CARTESIAN_POINT ( 'NONE',  ( 0.2867679344610365999, -0.2867679344610365444, -2.702755905511810663 ) ) ;
#13412=CARTESIAN_POINT ( 'NONE',  ( -0.4091458600556402980, -0.2362204724409451284, -0.6824146981627295938 ) ) ;
#13413=CARTESIAN_POINT ( 'NONE',  ( 0.3392501089628018884, -0.1958661417322833942, -2.148969447015434575 ) ) ;
#13419=CARTESIAN_POINT ( 'NONE',  ( 0.1958661417322834775, 0.3392501089628018884, -1.961286089238845287 ) ) ;
#13425=CARTESIAN_POINT ( 'NONE',  ( 0.2925321140481931814, 0.2925321140481931814, -2.734251968503936592 ) ) ;
#13427=CARTESIAN_POINT ( 'NONE',  ( -0.3460692066303960868, 0.1998031496062990242, -1.128608923884514503 ) ) ;
#13429=CARTESIAN_POINT ( 'NONE',  ( 0.3392501089628018329, 0.1958661417322835607, 0.02950824327327895152 ) ) ;
#13442=CARTESIAN_POINT ( 'NONE',  ( -0.1049643490035307020, 0.3917322834645669549, -0.1561679790026246351 ) ) ;
#13445=CARTESIAN_POINT ( 'NONE',  ( 0.3949938075777411073, -0.1058382717557499464, -0.7414698162729659314 ) ) ;
#13448=CARTESIAN_POINT ( 'NONE',  ( -0.4724409448818898682, -8.678599364036362592E-17, -0.1968503937007874127 ) ) ;
#13452=CARTESIAN_POINT ( 'NONE',  ( 0.3392501089628018329, 0.1958661417322835607, -1.545294906333020135 ) ) ;
#13458=CARTESIAN_POINT ( 'NONE',  ( 0.3996062992125986035, 0.1070741851644054776, -1.384514435695537671 ) ) ;
#13460=CARTESIAN_POINT ( 'NONE',  ( 4.893765752498283308E-17, -0.3996062992125985480, -0.9429133858267716439 ) ) ;
#13461=CARTESIAN_POINT ( 'NONE',  ( 4.893765752498283308E-17, -0.3996062992125985480, -0.3129921259842520231 ) ) ;
#13463=CARTESIAN_POINT ( 'NONE',  ( -0.2925321140481932924, 0.2925321140481931814, -2.539370078740157410 ) ) ;
#13464=CARTESIAN_POINT ( 'NONE',  ( 0.1958661417322836440, -0.3392501089628017219, -1.908792650918635259 ) ) ;
#13470=CARTESIAN_POINT ( 'NONE',  ( 0.3458507752293908943, -0.3458507752293908943, -1.435039370078740051 ) ) ;
#13473=CARTESIAN_POINT ( 'NONE',  ( 0.3949938075777409963, 2.418639510665530743E-17, -1.454724409448818756 ) ) ;
#13483=CARTESIAN_POINT ( 'NONE',  ( 0.1070741851644053388, 0.3996062992125986035, -2.117454068241469756 ) ) ;
#13486=CARTESIAN_POINT ( 'NONE',  ( 0.2867679344610365999, -0.2867679344610365999, -2.225702468995064187 ) ) ;
#13494=CARTESIAN_POINT ( 'NONE',  ( -0.4724409448818899238, 0.1265901696524986964, -2.395013123359579943 ) ) ;
#13497=CARTESIAN_POINT ( 'NONE',  ( 0.3996062992125986035, -0.1070741851644052972, 0.1266404199475065218 ) ) ;
#13499=CARTESIAN_POINT ( 'NONE',  ( 0.3392501089628018329, 0.1958661417322835607, -1.318241469816273215 ) ) ;
#13521=CARTESIAN_POINT ( 'NONE',  ( -0.3917322834645671215, 0.1049643490035301469, -2.544619422572177658 ) ) ;
#13524=CARTESIAN_POINT ( 'NONE',  ( -0.2362204724409451284, 0.4091458600556402425, -0.9580052493438320216 ) ) ;
#13525=CARTESIAN_POINT ( 'NONE',  ( -0.2925321140481932924, 0.2925321140481931814, -0.1771653543307087075 ) ) ;
#13528=CARTESIAN_POINT ( 'NONE',  ( -0.3917322834645670104, -7.196005306013484475E-17, -1.921259842519684957 ) ) ;
#13532=CARTESIAN_POINT ( 'NONE',  ( -0.4091458600556405756, 0.2362204724409446288, -2.860892388451443669 ) ) ;
#13540=CARTESIAN_POINT ( 'NONE',  ( -0.3917322834645668994, -0.1049643490035306742, -1.228327140911074089 ) ) ;
#13547=CARTESIAN_POINT ( 'NONE',  ( 0.2867679344610366554, -0.2867679344610365999, -2.457368397146668659 ) ) ;
#13555=CARTESIAN_POINT ( 'NONE',  ( 0.2867679344610365999, -0.2867679344610365444, -1.757874015748031260 ) ) ;
#13566=CARTESIAN_POINT ( 'NONE',  ( -0.4724409448818898682, 5.785732909357575061E-17, -2.755905511811024056 ) ) ;
#13574=CARTESIAN_POINT ( 'NONE',  ( -0.4724409448818898682, -8.678599364036362592E-17, -0.4311023622047244208 ) ) ;
#13577=CARTESIAN_POINT ( 'NONE',  ( 0.3949938075777409963, 2.418639510665530743E-17, -0.3523622047244094335 ) ) ;
#13582=CARTESIAN_POINT ( 'NONE',  ( -0.1058382717557497660, -0.3949938075777411073, 0.008530183727034110208 ) ) ;
#13589=CARTESIAN_POINT ( 'NONE',  ( 0.3996062992125985480, 2.446882876249141654E-17, -0.9822834645669291653 ) ) ;
#13592=CARTESIAN_POINT ( 'NONE',  ( -0.3917322834645669549, -0.1049643490035306603, -0.5104986876640419391 ) ) ;
#13593=EDGE_CURVE ( 'NONE', #2797, #5054, #49294, .T. ) ;
#13608=CARTESIAN_POINT ( 'NONE',  ( -0.2362204724409451284, 0.4091458600556402425, -2.609580052493438274 ) ) ;
#13626=CARTESIAN_POINT ( 'NONE',  ( 0.1070741851644054915, -0.3996062992125985480, -0.5577427821522309426 ) ) ;
#13627=CARTESIAN_POINT ( 'NONE',  ( -1.157146581871515012E-16, 0.4724409448818898682, -1.179133858267716661 ) ) ;
#13631=CARTESIAN_POINT ( 'NONE',  ( -0.1998031496062994683, 0.3460692066303958092, -2.690288713910760965 ) ) ;
#13632=CARTESIAN_POINT ( 'NONE',  ( -0.1058382717557503211, 0.3949938075777409408, -1.738845144356955696 ) ) ;
#13633=CARTESIAN_POINT ( 'NONE',  ( -0.1958661417322834220, -0.3392501089628018884, -0.5301837270341206443 ) ) ;
#13635=CARTESIAN_POINT ( 'NONE',  ( 0.1049643490035304799, -0.3917322834645669549, -1.179790026246718915 ) ) ;
#13637=CARTESIAN_POINT ( 'NONE',  ( -0.2867679344610365999, 0.2867679344610364889, -1.114173228346456712 ) ) ;
#13639=CARTESIAN_POINT ( 'NONE',  ( 0.1058382717557500852, -0.3949938075777408852, -2.839238845144357093 ) ) ;
#13640=EDGE_CURVE ( 'NONE', #23562, #14913, #77783, .T. ) ;
#13646=CARTESIAN_POINT ( 'NONE',  ( -0.3460692066303960868, 0.1998031496062990242, -2.703412073490813583 ) ) ;
#13647=CARTESIAN_POINT ( 'NONE',  ( 0.3917322834645670104, 0.1049643490035304660, -1.381252911582363962 ) ) ;
#13652=CARTESIAN_POINT ( 'NONE',  ( 0.3392501089628018884, -0.1958661417322834220, -0.3471128608923885195 ) ) ;
#13661=CARTESIAN_POINT ( 'NONE',  ( -0.2579773093923122262, -0.2955417804225481393, -1.929133858267716439 ) ) ;
#13662=CARTESIAN_POINT ( 'NONE',  ( 0.1958661417322834775, 0.3392501089628018884, -2.026246719160105236 ) ) ;
#13666=CARTESIAN_POINT ( 'NONE',  ( 0.2925321140481932369, 0.2925321140481932369, 0.01968503937007872254 ) ) ;
#13672=CARTESIAN_POINT ( 'NONE',  ( 0.1265901696524990572, -0.4724409448818897017, -1.187664041994750619 ) ) ;
#13673=CARTESIAN_POINT ( 'NONE',  ( 0.1958661417322834775, 0.3392501089628018884, -1.016404199475065662 ) ) ;
#13682=DIRECTION ( 'NONE',  ( 0.000000000000000000, 1.000000000000000000, 0.000000000000000000 ) ) ;
#13691=CARTESIAN_POINT ( 'NONE',  ( -0.3392501089628018329, -0.1958661417322836440, -0.9199281907798407820 ) ) ;
#13694=CARTESIAN_POINT ( 'NONE',  ( -0.4724409448818898682, -8.678599364036362592E-17, -0.03937007874015747977 ) ) ;
#13700=CARTESIAN_POINT ( 'NONE',  ( -0.3392501089628017219, -0.1958661417322836995, -0.04923191420703601495 ) ) ;
#13702=( BOUNDED_CURVE ( )  B_SPLINE_CURVE ( 2, ( #21470, #66094, #47959, #21881, #2116, #8430, #73235, #22712, #15586, #2948, #54270, #73663, #40824 ),
 .UNSPECIFIED., .F., .F. ) 
 B_SPLINE_CURVE_WITH_KNOTS ( ( 3, 2, 2, 2, 2, 2, 3 ),
 ( 0.3125000000000000000, 0.3166666666666666519, 0.3208333333333333592, 0.3250000000000000111, 0.3291666666666666630, 0.3333333333333333148, 0.3375000000000000222 ),
 .UNSPECIFIED. ) 
 CURVE ( )  GEOMETRIC_REPRESENTATION_ITEM ( )  RATIONAL_B_SPLINE_CURVE ( ( 1.000000000000000000, 0.9659258262890683122, 1.000000000000000000, 0.9659258262890683122, 1.000000000000000000, 0.9659258262890683122, 1.000000000000000000, 0.9659258262890683122, 1.000000000000000000, 0.9659258262890683122, 1.000000000000000000, 0.9659258262890683122, 1.000000000000000000 ) ) 
 REPRESENTATION_ITEM ( '' )  );
#13704=CARTESIAN_POINT ( 'NONE',  ( 0.4724409448818896462, 0.1265901696524990294, -1.146325459317585116 ) ) ;
#13714=CARTESIAN_POINT ( 'NONE',  ( 0.000000000000000000, 0.000000000000000000, -2.755905511811024056 ) ) ;
#13721=CARTESIAN_POINT ( 'NONE',  ( 0.3460692066303959202, -0.1998031496062991630, -2.229002624671915900 ) ) ;
#13725=CARTESIAN_POINT ( 'NONE',  ( 0.3460692066303959202, -0.1998031496062991630, -1.599081364829396446 ) ) ;
#13731=CARTESIAN_POINT ( 'NONE',  ( -0.1998031496062991630, -0.3460692066303959202, -1.087270341207349000 ) ) ;
#13732=CARTESIAN_POINT ( 'NONE',  ( -0.1070741851644056997, 0.3996062992125986035, -1.266404199475065440 ) ) ;
#13733=CARTESIAN_POINT ( 'NONE',  ( -0.1058382717557503211, 0.3949938075777409408, -0.6364829396325458744 ) ) ;
#13739=CARTESIAN_POINT ( 'NONE',  ( -0.3949938075777408852, -0.1058382717557502933, -1.854986876640420501 ) ) ;
#13744=CARTESIAN_POINT ( 'NONE',  ( -0.4724409448818898682, -8.678599364036362592E-17, -1.771653543307086576 ) ) ;
#13752=CARTESIAN_POINT ( 'NONE',  ( 0.1049643490035304522, -0.3917322834645668994, -2.212579109415011569 ) ) ;
#13758=CARTESIAN_POINT ( 'NONE',  ( 0.1958661417322836162, -0.3392501089628018329, -2.849062049047557998 ) ) ;
#13760=CARTESIAN_POINT ( 'NONE',  ( -0.3392501089628017219, -0.1958661417322836718, -1.619422572178477848 ) ) ;
#13763=CARTESIAN_POINT ( 'NONE',  ( 0.3949938075777411073, -0.1058382717557499464, -1.843832020997375309 ) ) ;
#13768=CARTESIAN_POINT ( 'NONE',  ( -0.1070741851644051862, -0.3996062992125987146, -0.5446194225721783244 ) ) ;
#13775=CARTESIAN_POINT ( 'NONE',  ( 0.1958661417322836440, -0.3392501089628017219, -0.1765091863517061210 ) ) ;
#13780=ORIENTED_EDGE ( 'NONE', *, *, #24858, .F. ) ;
#13782=CARTESIAN_POINT ( 'NONE',  ( 0.3996062992125986035, -0.1070741851644052972, -2.078083989501312345 ) ) ;
#13787=CARTESIAN_POINT ( 'NONE',  ( 0.1265901696524990294, -0.4724409448818896462, -0.7152230971128609172 ) ) ;
#13789=CARTESIAN_POINT ( 'NONE',  ( -0.3392501089628017219, -0.1958661417322836718, -0.2020997375328083545 ) ) ;
#13790=CARTESIAN_POINT ( 'NONE',  ( -9.594673741351313045E-17, 0.3917322834645670104, -1.974409448818897683 ) ) ;
#13794=CARTESIAN_POINT ( 'NONE',  ( -0.3460692066303957537, -0.1998031496062994405, 0.1856955380577427484 ) ) ;
#13799=CARTESIAN_POINT ( 'NONE',  ( -0.2891555358219911054, 0.2891555358219909388, -2.616141732283464805 ) ) ;
#13802=CARTESIAN_POINT ( 'NONE',  ( 0.2867679344610366554, -0.2867679344610365444, -0.1830708661417323746 ) ) ;
#13807=CARTESIAN_POINT ( 'NONE',  ( 0.1958661417322834775, 0.3392501089628018884, -1.868766404199474929 ) ) ;
#13810=CARTESIAN_POINT ( 'NONE',  ( -0.2362204724409447953, -0.4091458600556404646, 0.01509186351706036204 ) ) ;
#13815=CARTESIAN_POINT ( 'NONE',  ( 0.3458507752293908943, 0.3458507752293908943, -0.6870078740157479213 ) ) ;
#13824=CARTESIAN_POINT ( 'NONE',  ( 0.1998031496062992463, 0.3460692066303959202, -1.008530183727034180 ) ) ;
#13825=CARTESIAN_POINT ( 'NONE',  ( 0.3392501089628018884, -0.1958661417322834220, -2.866797900262466836 ) ) ;
#13834=CARTESIAN_POINT ( 'NONE',  ( 0.2925321140481932369, 0.2925321140481932369, -0.2952755905511811330 ) ) ;
#13836=CARTESIAN_POINT ( 'NONE',  ( 0.1958661417322836718, -0.3392501089628017219, -2.608287032317271770 ) ) ;
#13838=CARTESIAN_POINT ( 'NONE',  ( 0.02578378529929631693, -0.3963884504522709462, -2.713666019656065720E-16 ) ) ;
#13842=CARTESIAN_POINT ( 'NONE',  ( 0.1958661417322836440, -0.3392501089628017219, -2.223753280839895208 ) ) ;
#13847=CARTESIAN_POINT ( 'NONE',  ( -0.3460692066303957537, -0.1998031496062994405, -2.648950131233595684 ) ) ;
#13849=CARTESIAN_POINT ( 'NONE',  ( 0.2925321140481932369, -0.2925321140481932369, -1.358267716535433101 ) ) ;
#13851=CARTESIAN_POINT ( 'NONE',  ( -0.3917322834645670104, -0.1049643490035307020, 0.1148100805436201299 ) ) ;
#13862=CARTESIAN_POINT ( 'NONE',  ( 0.3917322834645669549, 0.1049643490035304660, -0.1167979002624671414 ) ) ;
#13865=CARTESIAN_POINT ( 'NONE',  ( -0.3420746716998659953, -0.1974969037888706647, -0.5249343832020998413 ) ) ;
#13875=DIRECTION ( 'NONE',  ( 1.000000000000000000, 0.000000000000000000, 0.000000000000000000 ) ) ;
#13881=CARTESIAN_POINT ( 'NONE',  ( -0.3996062992125986035, -7.340648628747425578E-17, -1.456692913385826849 ) ) ;
#13883=CARTESIAN_POINT ( 'NONE',  ( -0.2925321140481930149, -0.2925321140481933480, -0.6082677165354329896 ) ) ;
#13884=CARTESIAN_POINT ( 'NONE',  ( -0.3460692066303960313, 0.1998031496062989965, 0.05446194225721782967 ) ) ;
#13886=CARTESIAN_POINT ( 'NONE',  ( -9.787531504996567848E-17, 0.3996062992125986035, -2.677165354330708347 ) ) ;
#13887=CARTESIAN_POINT ( 'NONE',  ( 0.1049643490035304938, -0.3917322834645669549, -2.059711286089238591 ) ) ;
#13893=CARTESIAN_POINT ( 'NONE',  ( -0.4724409448818895907, -0.1265901696524993070, -1.382545931758530022 ) ) ;
#13898=CARTESIAN_POINT ( 'NONE',  ( -0.1974969037888706924, 0.3420746716998658843, -1.507217847769029007 ) ) ;
#13908=CARTESIAN_POINT ( 'NONE',  ( -0.3996062992125984925, -0.1070741851644056858, -2.327427821522309870 ) ) ;
#13910=EDGE_CURVE ( 'NONE', #15221, #32199, #20096, .T. ) ;
#13911=CARTESIAN_POINT ( 'NONE',  ( -0.1958661417322836440, 0.3392501089628016664, -1.982920316764092306 ) ) ;
#13924=CARTESIAN_POINT ( 'NONE',  ( -0.3996062992125985480, -7.340648628747423112E-17, 0.1988188976377952832 ) ) ;
#13926=CARTESIAN_POINT ( 'NONE',  ( 0.2867679344610365999, 0.2867679344610365999, -1.324803149606299302 ) ) ;
#13948=CARTESIAN_POINT ( 'NONE',  ( 4.797336870675656522E-17, -0.3917322834645670104, -2.433070866141732402 ) ) ;
#13951=CARTESIAN_POINT ( 'NONE',  ( 0.4724409448818897572, -0.1265901696524988906, -0.5839895013123358458 ) ) ;
#13952=CARTESIAN_POINT ( 'NONE',  ( -0.1998031496062994683, 0.3460692066303958092, -0.01312335958005251234 ) ) ;
#13953=VERTEX_POINT ( 'NONE', #77340 ) ;
#13956=CARTESIAN_POINT ( 'NONE',  ( -9.594673741351313045E-17, 0.3917322834645670104, -1.724409448818897683 ) ) ;
#13967=CARTESIAN_POINT ( 'NONE',  ( -0.1958661417322836440, 0.3392501089628016664, -1.038038427000312902 ) ) ;
#13972=ORIENTED_EDGE ( 'NONE', *, *, #66038, .T. ) ;
#13973=CARTESIAN_POINT ( 'NONE',  ( 0.3917322834645670104, 0.1049643490035304660, -2.641095431267403537 ) ) ;
#13980=EDGE_CURVE ( 'NONE', #69925, #78139, #73535, .T. ) ;
#13982=CARTESIAN_POINT ( 'NONE',  ( -0.3392501089628019995, 0.1958661417322832277, -1.685695538057742970 ) ) ;
#13997=CARTESIAN_POINT ( 'NONE',  ( -0.4724409448818898682, -8.678599364036362592E-17, -0.2736220472440945017 ) ) ;
#14000=CARTESIAN_POINT ( 'NONE',  ( -9.674558042662122972E-17, 0.3949938075777409963, -0.07677165354330710290 ) ) ;
#14006=CARTESIAN_POINT ( 'NONE',  ( -0.2891555358219911054, 0.2891555358219909388, -0.09645669291338582196 ) ) ;
#14013=CARTESIAN_POINT ( 'NONE',  ( -0.3996062992125986590, 0.1070741851644051723, -0.8969816272965877024 ) ) ;
#14015=CARTESIAN_POINT ( 'NONE',  ( -0.1049643490035302024, -0.3917322834645671215, -0.8517060367454066805 ) ) ;
#14031=CARTESIAN_POINT ( 'NONE',  ( -0.3996062992125984925, -0.1070741851644056858, 0.1922572178477689464 ) ) ;
#14038=CARTESIAN_POINT ( 'NONE',  ( 0.3458507752293908943, 0.3458507752293908943, -2.027559055118109743 ) ) ;
#14046=EDGE_CURVE ( 'NONE', #18027, #57846, #17238, .T. ) ;
#14050=CARTESIAN_POINT ( 'NONE',  ( 0.1070741851644053666, 0.3996062992125986035, -0.7808398950131233418 ) ) ;
#14055=CARTESIAN_POINT ( 'NONE',  ( 0.1070741851644054915, -0.3996062992125986035, -2.762467191601049255 ) ) ;
#14056=CARTESIAN_POINT ( 'NONE',  ( -0.1058382717557503211, 0.3949938075777409408, -1.896325459317585116 ) ) ;
#14057=CARTESIAN_POINT ( 'NONE',  ( 0.3917322834645669549, 0.1049643490035304660, -0.4317585301837270628 ) ) ;
#14059=CARTESIAN_POINT ( 'NONE',  ( 0.3917322834645670104, -0.1049643490035303273, -1.206036745406823929 ) ) ;
#14061=CARTESIAN_POINT ( 'NONE',  ( 0.1049643490035303689, 0.3917322834645670104, -1.245406824146981561 ) ) ;
#14063=CARTESIAN_POINT ( 'NONE',  ( -0.2867679344610364334, -0.2867679344610368219, 0.01839201919391258294 ) ) ;
#14069=CARTESIAN_POINT ( 'NONE',  ( -0.4724409448818899238, 0.1265901696524986964, -0.1095800524934383291 ) ) ;
#14070=CARTESIAN_POINT ( 'NONE',  ( 4.893765752498283924E-17, -0.3996062992125986035, -2.755905511811023612 ) ) ;
#14071=CARTESIAN_POINT ( 'NONE',  ( 0.2867679344610366554, 0.2867679344610366554, -1.079415641241156854 ) ) ;
#14078=CARTESIAN_POINT ( 'NONE',  ( 0.1049643490035303689, 0.3917322834645670104, -0.5505249343832020470 ) ) ;
#14086=CARTESIAN_POINT ( 'NONE',  ( 0.3808816823641231752, -0.09156050430092187165, -1.929133858267716661 ) ) ;
#14087=CARTESIAN_POINT ( 'NONE',  ( 0.1958661417322836440, -0.3392501089628017219, -1.973753280839895208 ) ) ;
#14089=CARTESIAN_POINT ( 'NONE',  ( -0.1070741851644051862, -0.3996062992125987146, -0.5446194225721783244 ) ) ;
#14096=CARTESIAN_POINT ( 'NONE',  ( -0.3392501089628019995, 0.1958661417322832277, -1.055774278215223294 ) ) ;
#14101=VERTEX_POINT ( 'NONE', #3233 ) ;
#14111=CARTESIAN_POINT ( 'NONE',  ( -0.4091458600556402980, -0.2362204724409451284, -2.491469816272966042 ) ) ;
#14115=CARTESIAN_POINT ( 'NONE',  ( -9.594673741351310580E-17, 0.3917322834645669549, -0.8674347524596309755 ) ) ;
#14125=CARTESIAN_POINT ( 'NONE',  ( -0.3917322834645670104, -0.1049643490035307020, -0.2001505493776396805 ) ) ;
#14129=CARTESIAN_POINT ( 'NONE',  ( 0.4724409448818896462, 0.1265901696524990294, -1.461286089238844843 ) ) ;
#14145=CARTESIAN_POINT ( 'NONE',  ( -0.1070741851644051862, -0.3996062992125986590, -2.196194225721784576 ) ) ;
#14149=CARTESIAN_POINT ( 'NONE',  ( -0.2925321140481932369, 0.2925321140481931259, -1.828740157480315265 ) ) ;
#14155=CARTESIAN_POINT ( 'NONE',  ( -0.2925321140481932369, 0.2925321140481930704, -1.198818897637795367 ) ) ;
#14156=CARTESIAN_POINT ( 'NONE',  ( 0.1998031496062994405, -0.3460692066303958092, -1.509186351706036655 ) ) ;
#14157=CARTESIAN_POINT ( 'NONE',  ( -0.1974969037888703871, -0.3420746716998661063, -0.6955380577427822120 ) ) ;
#14163=CARTESIAN_POINT ( 'NONE',  ( -0.3420746716998660508, -0.1974969037888706924, -1.546587926509186417 ) ) ;
#14168=CARTESIAN_POINT ( 'NONE',  ( 5.785732909357575061E-17, -0.4724409448818898682, -1.968503937007873850 ) ) ;
#14175=CARTESIAN_POINT ( 'NONE',  ( -0.3917322834645670659, 0.1049643490035301607, -2.317565986055430738 ) ) ;
#14181=CARTESIAN_POINT ( 'NONE',  ( 0.3392501089628018329, 0.1958661417322835052, -2.730951812827084435 ) ) ;
#14183=CARTESIAN_POINT ( 'NONE',  ( 0.1049643490035304938, -0.3917322834645669549, -1.809711286089239035 ) ) ;
#14186=CARTESIAN_POINT ( 'NONE',  ( 0.3949938075777409963, 2.418639510665530435E-17, -1.692913385826771533 ) ) ;
#14189=VECTOR ( 'NONE', #29537, 39.37007874015748143 ) ;
#14192=CARTESIAN_POINT ( 'NONE',  ( 0.3460692066303959757, -0.1998031496062991907, -0.5774278215223097588 ) ) ;
#14199=DIRECTION ( 'NONE',  ( 1.000000000000000000, 0.000000000000000000, 0.000000000000000000 ) ) ;
#14200=CARTESIAN_POINT ( 'NONE',  ( -0.2867679344610365999, 0.2867679344610364889, -0.2618110236220473341 ) ) ;
#14203=EDGE_CURVE ( 'NONE', #28644, #59098, #66630, .T. ) ;
#14211=CARTESIAN_POINT ( 'NONE',  ( -0.2362204724409451284, 0.4091458600556402425, -1.272965879265091749 ) ) ;
#14213=CARTESIAN_POINT ( 'NONE',  ( -0.1049643490035307020, 0.3917322834645669549, -0.1561679790026246351 ) ) ;
#14214=CARTESIAN_POINT ( 'NONE',  ( -0.3917322834645669549, -0.1049643490035306603, -2.335301837270341352 ) ) ;
#14218=CARTESIAN_POINT ( 'NONE',  ( 0.3996062992125986035, -0.1070741851644052972, -0.03083989501312338344 ) ) ;
#14223=CARTESIAN_POINT ( 'NONE',  ( -0.1058382717557503072, 0.3949938075777408852, -2.760498687664042716 ) ) ;
#14230=CARTESIAN_POINT ( 'NONE',  ( 0.3392501089628018884, -0.1958661417322834220, -1.986876640419947604 ) ) ;
#14234=CARTESIAN_POINT ( 'NONE',  ( 5.785732909357575061E-17, -0.4724409448818898682, 0.001968503937007862279 ) ) ;
#14248=CARTESIAN_POINT ( 'NONE',  ( 0.1070741851644053388, 0.3996062992125986035, -1.015091863517060267 ) ) ;
#14249=CARTESIAN_POINT ( 'NONE',  ( 0.1049643490035303689, 0.3917322834645670104, -2.755249343832020248 ) ) ;
#14259=CARTESIAN_POINT ( 'NONE',  ( -0.1070741851644056997, 0.3996062992125986035, -0.006561679790026256169 ) ) ;
#14260=CARTESIAN_POINT ( 'NONE',  ( 0.3392501089628018329, 0.1958661417322835607, -2.332696481136169453 ) ) ;
#14266=CARTESIAN_POINT ( 'NONE',  ( -0.2867679344610365999, 0.2867679344610364889, -2.466535433070865757 ) ) ;
#14271=CARTESIAN_POINT ( 'NONE',  ( -0.3460692066303960868, 0.1998031496062990242, -2.073490813648294129 ) ) ;
#14273=CARTESIAN_POINT ( 'NONE',  ( -0.3460692066303958092, -0.1998031496062994683, -1.154855643044619518 ) ) ;
#14275=CARTESIAN_POINT ( 'NONE',  ( 0.3917322834645670659, 2.398668435337828261E-17, 0.04263160285333144478 ) ) ;
#14286=CARTESIAN_POINT ( 'NONE',  ( -0.3917322834645671215, 0.1049643490035301469, -0.4973753280839895430 ) ) ;
#14289=CARTESIAN_POINT ( 'NONE',  ( -0.1058382717557503211, 0.3949938075777409408, -0.7939632545931760710 ) ) ;
#14308=CARTESIAN_POINT ( 'NONE',  ( -0.3996062992125986035, -7.340648628747425578E-17, -1.299212598425196985 ) ) ;
#14310=CARTESIAN_POINT ( 'NONE',  ( 0.3996062992125984925, 0.1070741851644054637, -0.8313648293963252778 ) ) ;
#14311=CARTESIAN_POINT ( 'NONE',  ( -0.3996062992125986590, 0.1070741851644051723, -0.4245406824146981672 ) ) ;
#14313=CARTESIAN_POINT ( 'NONE',  ( -0.4091458600556405756, 0.2362204724409446288, -0.02624671916010498651 ) ) ;
#14315=CARTESIAN_POINT ( 'NONE',  ( -0.1049643490035307020, 0.3917322834645669549, -1.980971128608924214 ) ) ;
#14318=VECTOR ( 'NONE', #28066, 39.37007874015748143 ) ;
#14322=CARTESIAN_POINT ( 'NONE',  ( 0.4724409448818896462, 0.1265901696524990294, -1.933727034120735100 ) ) ;
#14325=CARTESIAN_POINT ( 'NONE',  ( -0.2891555358219909388, -0.2891555358219912164, -1.553149606299212504 ) ) ;
#14335=CARTESIAN_POINT ( 'NONE',  ( 0.1998031496062992463, 0.3460692066303959202, -2.110892388451443669 ) ) ;
#14336=CARTESIAN_POINT ( 'NONE',  ( 0.1049643490035304522, -0.3917322834645668994, -2.055098794454381927 ) ) ;
#14351=CARTESIAN_POINT ( 'NONE',  ( 0.2867679344610365999, -0.2867679344610365444, -1.600393700787401619 ) ) ;
#14374=CARTESIAN_POINT ( 'NONE',  ( -0.3917322834645669549, -0.1049643490035306603, -2.400262467191600635 ) ) ;
#14377=CARTESIAN_POINT ( 'NONE',  ( 0.3460692066303959202, 0.1998031496062993295, 0.02624671916010496570 ) ) ;
#14380=CARTESIAN_POINT ( 'NONE',  ( 0.2867679344610365999, -0.2867679344610365444, -1.665354330708661124 ) ) ;
#14391=CARTESIAN_POINT ( 'NONE',  ( 0.3917322834645668994, -0.1049643490035303134, -1.293943938811336958 ) ) ;
#14397=ORIENTED_EDGE ( 'NONE', *, *, #47459, .F. ) ;
#14398=CARTESIAN_POINT ( 'NONE',  ( 0.3917322834645670659, 2.398668435337828261E-17, -2.477053436516747364 ) ) ;
#14408=CARTESIAN_POINT ( 'NONE',  ( -0.1049643490035307020, 0.3917322834645669549, -1.823490813648294129 ) ) ;
#14424=CARTESIAN_POINT ( 'NONE',  ( -0.4724409448818899238, 0.1265901696524986686, -0.7395013123359580609 ) ) ;
#14427=CARTESIAN_POINT ( 'NONE',  ( 0.1058382717557499880, 0.3949938075777409408, -0.2276902887139107823 ) ) ;
#14432=CARTESIAN_POINT ( 'NONE',  ( 0.1974969037888706092, -0.3420746716998660508, 0.1463254593175853102 ) ) ;
#14439=CARTESIAN_POINT ( 'NONE',  ( 0.1070741851644053388, 0.3996062992125986035, -0.8576115485564304031 ) ) ;
#14441=CARTESIAN_POINT ( 'NONE',  ( -0.3917322834645670104, -7.196005306013484475E-17, -0.6614173228346454936 ) ) ;
#14453=CARTESIAN_POINT ( 'NONE',  ( -0.3980111619244106058, -0.03175677952934882753, -1.220472440944883719 ) ) ;
#14455=CARTESIAN_POINT ( 'NONE',  ( -0.4724409448818895907, -0.1265901696524993070, -2.799868766404198794 ) ) ;
#14471=CARTESIAN_POINT ( 'NONE',  ( -0.1070741851644057135, 0.3996062992125985480, -0.6364829396325458744 ) ) ;
#14477=CARTESIAN_POINT ( 'NONE',  ( 0.2925321140481932369, 0.2925321140481932369, -2.657480314960630530 ) ) ;
#14478=CARTESIAN_POINT ( 'NONE',  ( -0.3949938075777411628, 0.1058382717557497937, -1.922572178477690130 ) ) ;
#14479=CARTESIAN_POINT ( 'NONE',  ( 4.797336870675656522E-17, -0.3917322834645670104, -0.3858267716535432879 ) ) ;
#14480=CARTESIAN_POINT ( 'NONE',  ( 0.2867679344610366554, 0.2867679344610366554, -0.9173228346456692162 ) ) ;
#14482=CARTESIAN_POINT ( 'NONE',  ( -0.2867679344610364334, -0.2867679344610367109, -0.9960629921259842590 ) ) ;
#14484=CARTESIAN_POINT ( 'NONE',  ( 0.2867679344610365999, 0.2867679344610365999, -0.06034813828640239741 ) ) ;
#14491=CARTESIAN_POINT ( 'NONE',  ( 4.893765752498283924E-17, -0.3996062992125986035, -2.598425196850393970 ) ) ;
#14492=CARTESIAN_POINT ( 'NONE',  ( 0.1049643490035303967, 0.3917322834645670659, -1.092539000821209250 ) ) ;
#14498=CARTESIAN_POINT ( 'NONE',  ( -0.3917322834645669549, -0.1049643490035306603, -0.7604986876640419391 ) ) ;
#14506=CARTESIAN_POINT ( 'NONE',  ( -0.3594585737333946263, -0.1614515132150200205, -1.929133858267715773 ) ) ;
#14507=CARTESIAN_POINT ( 'NONE',  ( 4.797336870675656522E-17, -0.3917322834645670104, -1.960629921259842368 ) ) ;
#14509=CARTESIAN_POINT ( 'NONE',  ( 0.3996062992125986035, 2.446882876249141962E-17, -0.5905511811023621549 ) ) ;
#14515=CARTESIAN_POINT ( 'NONE',  ( 0.4724409448818898682, 2.892866454678787531E-17, -1.220472440944881942 ) ) ;
#14516=CARTESIAN_POINT ( 'NONE',  ( 4.797336870675656522E-17, -0.3917322834645670104, -1.108267716535433101 ) ) ;
#14538=CARTESIAN_POINT ( 'NONE',  ( -0.3392501089628018329, -0.1958661417322836440, -1.234888820701100398 ) ) ;
#14541=CARTESIAN_POINT ( 'NONE',  ( -0.4724409448818898682, -8.678599364036362592E-17, -0.8267716535433070613 ) ) ;
#14547=CARTESIAN_POINT ( 'NONE',  ( -0.3392501089628017219, -0.1958661417322836995, 0.1082484007535938902 ) ) ;
#14551=CARTESIAN_POINT ( 'NONE',  ( -0.2362204724409447953, -0.4091458600556404646, -1.717191601049868677 ) ) ;
#14566=CARTESIAN_POINT ( 'NONE',  ( 0.3996062992125986035, -0.1070741851644052972, -2.708005249343832688 ) ) ;
#14571=CARTESIAN_POINT ( 'NONE',  ( -0.1998031496062994405, 0.3460692066303957537, -1.664698162729658870 ) ) ;
#14577=CARTESIAN_POINT ( 'NONE',  ( -0.1998031496062994683, 0.3460692066303958092, -1.272965879265091749 ) ) ;
#14578=CARTESIAN_POINT ( 'NONE',  ( 4.837279021331060870E-17, -0.3949938075777409963, -0.8661417322834645827 ) ) ;
#14582=CARTESIAN_POINT ( 'NONE',  ( 4.837279021331061486E-17, -0.3949938075777409963, -1.887795275590550936 ) ) ;
#14587=CARTESIAN_POINT ( 'NONE',  ( -1.157146581871515012E-16, 0.4724409448818898682, -1.889763779527559251 ) ) ;
#14588=CARTESIAN_POINT ( 'NONE',  ( 0.3436793299028388926, -0.1882840440723189401, -2.755905511811023612 ) ) ;
#14594=CARTESIAN_POINT ( 'NONE',  ( 0.1049643490035303689, 0.3917322834645668994, -2.435676222275903857 ) ) ;
#14595=CARTESIAN_POINT ( 'NONE',  ( 0.3996062992125985480, 2.446882876249141654E-17, -2.872047244094488416 ) ) ;
#14600=CARTESIAN_POINT ( 'NONE',  ( 0.2867679344610365999, -0.2867679344610365444, 0.1318897637795274913 ) ) ;
#14602=CARTESIAN_POINT ( 'NONE',  ( 4.797336870675656522E-17, -0.3917322834645670104, -1.803149606299212726 ) ) ;
#14605=CARTESIAN_POINT ( 'NONE',  ( -0.1974969037888706647, 0.3420746716998658843, -2.217847769028871596 ) ) ;
#14606=ORIENTED_EDGE ( 'NONE', *, *, #37682, .T. ) ;
#14610=CARTESIAN_POINT ( 'NONE',  ( 0.2925321140481932369, 0.2925321140481932369, -0.7677165354330709457 ) ) ;
#14617=CARTESIAN_POINT ( 'NONE',  ( -0.1958661417322836718, 0.3392501089628017219, -0.2552493438320210806 ) ) ;
#14622=CARTESIAN_POINT ( 'NONE',  ( -0.3392501089628017219, -0.1958661417322836718, 0.1128608923884514836 ) ) ;
#14623=EDGE_LOOP ( 'NONE', ( #41172, #35927, #24633, #61887 ) ) ;
#14628=CARTESIAN_POINT ( 'NONE',  ( 0.1265901696524990294, -0.4724409448818896462, -1.345144356955380704 ) ) ;
#14630=CARTESIAN_POINT ( 'NONE',  ( 0.3917322834645669549, 0.1049643490035304660, -0.1167979002624671414 ) ) ;
#14631=CARTESIAN_POINT ( 'NONE',  ( 0.1049643490035303689, 0.3917322834645670104, -2.440288713910760521 ) ) ;
#14634=CARTESIAN_POINT ( 'NONE',  ( -0.1998031496062991630, -0.3460692066303959202, 0.01509186351706034469 ) ) ;
#14639=CARTESIAN_POINT ( 'NONE',  ( -0.3949938075777408852, -0.1058382717557502933, -2.799868766404199683 ) ) ;
#14641=CARTESIAN_POINT ( 'NONE',  ( -0.1958661417322836718, 0.3392501089628017219, -0.09776902887139117537 ) ) ;
#14646=CARTESIAN_POINT ( 'NONE',  ( 0.1958661417322836440, -0.3392501089628017219, -1.816272965879265122 ) ) ;
#14650=CARTESIAN_POINT ( 'NONE',  ( 0.2362204724409451007, -0.4091458600556402980, -0.3261154855643044748 ) ) ;
#14661=CARTESIAN_POINT ( 'NONE',  ( -0.4091458600556405756, 0.2362204724409446288, -1.992782152230971437 ) ) ;
#14664=CARTESIAN_POINT ( 'NONE',  ( -0.3996062992125984925, -0.1070741851644056858, -1.382545931758530022 ) ) ;
#14665=CARTESIAN_POINT ( 'NONE',  ( -9.594673741351313045E-17, 0.3917322834645670104, -2.761811023622046779 ) ) ;
#14674=CARTESIAN_POINT ( 'NONE',  ( 0.1070741851644054915, -0.3996062992125986035, 0.07217847769028869209 ) ) ;
#14675=CARTESIAN_POINT ( 'NONE',  ( 0.3917322834645670659, 2.398668435337828261E-17, -2.634533751477377450 ) ) ;
#14681=CARTESIAN_POINT ( 'NONE',  ( -9.594673741351313045E-17, 0.3917322834645670104, -2.604330708661416693 ) ) ;
#14686=CARTESIAN_POINT ( 'NONE',  ( 0.3996062992125986035, 2.446882876249141962E-17, -2.007874015748031482 ) ) ;
#14689=CARTESIAN_POINT ( 'NONE',  ( 0.3996062992125986035, 2.446882876249141962E-17, -1.850393700787401619 ) ) ;
#14691=CARTESIAN_POINT ( 'NONE',  ( 0.1049643490035303967, 0.3917322834645670659, -0.3051374260180596543 ) ) ;
#14704=CARTESIAN_POINT ( 'NONE',  ( 0.3392501089628018884, -0.1958661417322834220, -0.5695538057742781657 ) ) ;
#14707=CARTESIAN_POINT ( 'NONE',  ( 0.1058382717557500713, -0.3949938075777409408, -1.187664041994750619 ) ) ;
#14723=CARTESIAN_POINT ( 'NONE',  ( 0.3996062992125986035, 0.1070741851644054776, -1.069553805774278166 ) ) ;
#14725=CARTESIAN_POINT ( 'NONE',  ( -0.3996062992125985480, -7.340648628747423112E-17, -0.7460629921259841479 ) ) ;
#14726=CARTESIAN_POINT ( 'NONE',  ( -0.3460692066303957537, -0.1998031496062994405, -0.6017060367454067915 ) ) ;
#14728=CARTESIAN_POINT ( 'NONE',  ( -0.1265901696524986964, -0.4724409448818899238, -0.07217847769028870597 ) ) ;
#14730=CARTESIAN_POINT ( 'NONE',  ( 0.1958661417322836440, -0.3392501089628017219, -2.066272965879265122 ) ) ;
#14736=CARTESIAN_POINT ( 'NONE',  ( 0.3458507752293908943, 0.3458507752293908943, -2.104330708661417138 ) ) ;
#14739=CARTESIAN_POINT ( 'NONE',  ( 0.2891555358219910499, -0.2891555358219909944, -1.592519685039370581 ) ) ;
#14742=FACE_OUTER_BOUND ( 'NONE', #40242, .T. ) ;
#14749=CARTESIAN_POINT ( 'NONE',  ( 0.1070741851644054776, -0.3996062992125984925, -2.524278215223096478 ) ) ;
#14750=CARTESIAN_POINT ( 'NONE',  ( 0.3917322834645668994, 0.1049643490035304522, -2.094468873194538450 ) ) ;
#14761=CARTESIAN_POINT ( 'NONE',  ( -0.1998031496062991630, -0.3460692066303959202, 0.1725721784776902690 ) ) ;
#14763=CARTESIAN_POINT ( 'NONE',  ( 0.3917322834645670104, 2.398668435337828261E-17, -1.305118110236220375 ) ) ;
#14771=EDGE_CURVE ( 'NONE', #64662, #56613, #34424, .T. ) ;
#14773=CARTESIAN_POINT ( 'NONE',  ( -0.2925321140481932369, 0.2925321140481931259, -0.8838582677165351953 ) ) ;
#14786=CARTESIAN_POINT ( 'NONE',  ( 0.1049643490035304799, -0.3917322834645669549, -2.282152230971128404 ) ) ;
#14789=CARTESIAN_POINT ( 'NONE',  ( -0.3460692066303960868, 0.1998031496062990242, -0.6561679790026246906 ) ) ;
#14792=CARTESIAN_POINT ( 'NONE',  ( 0.1958661417322836440, -0.3392501089628017219, -2.288713910761154935 ) ) ;
#14803=CARTESIAN_POINT ( 'NONE',  ( 0.3917322834645668994, 0.1049643490035304522, -1.149586983430759490 ) ) ;
#14809=CARTESIAN_POINT ( 'NONE',  ( 0.1049643490035303967, 0.3917322834645670659, -2.509861835466878244 ) ) ;
#14818=CARTESIAN_POINT ( 'NONE',  ( -0.3917322834645669549, -0.1049643490035306603, -2.020341207349081181 ) ) ;
#14826=CARTESIAN_POINT ( 'NONE',  ( -9.787531504996567848E-17, 0.3996062992125986035, -1.732283464566929165 ) ) ;
#14831=CARTESIAN_POINT ( 'NONE',  ( 5.785732909357575061E-17, -0.4724409448818898682, -0.7854330708661416693 ) ) ;
#14834=CARTESIAN_POINT ( 'NONE',  ( 4.837279021331061486E-17, -0.3949938075777409963, 0.001968503937007861845 ) ) ;
#14839=CARTESIAN_POINT ( 'NONE',  ( 0.3949938075777408852, 0.1058382717557500435, -0.6738845144356955252 ) ) ;
#14846=CARTESIAN_POINT ( 'NONE',  ( 0.1070741851644054776, -0.3996062992125984925, -1.421916010498687877 ) ) ;
#14848=CARTESIAN_POINT ( 'NONE',  ( 0.1049643490035303689, 0.3917322834645670104, -0.6154855643044617741 ) ) ;
#14860=CARTESIAN_POINT ( 'NONE',  ( -0.3808816823641234528, 0.09156050430092053938, -1.220472440944881942 ) ) ;
#14862=CARTESIAN_POINT ( 'NONE',  ( 0.3460692066303959202, -0.1998031496062991630, 0.1332020997375328031 ) ) ;
#14880=CARTESIAN_POINT ( 'NONE',  ( 0.2925321140481932369, -0.2925321140481931814, -0.8858267716535431768 ) ) ;
#14884=CARTESIAN_POINT ( 'NONE',  ( 0.1998031496062992740, 0.3460692066303959757, -2.664041994750656173 ) ) ;
#14885=CARTESIAN_POINT ( 'NONE',  ( 0.1974969037888706369, -0.3420746716998659953, -1.981627296587926690 ) ) ;
#14886=CARTESIAN_POINT ( 'NONE',  ( 0.3392501089628018329, 0.1958661417322835607, -0.5958005249343831800 ) ) ;
#14889=CARTESIAN_POINT ( 'NONE',  ( 0.2867679344610365999, 0.2867679344610365999, -0.9173228346456693272 ) ) ;
#14891=CARTESIAN_POINT ( 'NONE',  ( -0.1958661417322836440, 0.3392501089628016664, -0.09315653723653360974 ) ) ;
#14897=CARTESIAN_POINT ( 'NONE',  ( 0.1998031496062994405, -0.3460692066303958092, -2.454068241469816058 ) ) ;
#14898=CARTESIAN_POINT ( 'NONE',  ( -9.594673741351313045E-17, 0.3917322834645670659, -1.256580995571865200 ) ) ;
#14903=CARTESIAN_POINT ( 'NONE',  ( 0.3392501089628018884, -0.1958661417322834220, -0.5045931758530184386 ) ) ;
#14911=CARTESIAN_POINT ( 'NONE',  ( 0.4724409448818898682, 0.000000000000000000, -2.755905511811024056 ) ) ;
#14912=CARTESIAN_POINT ( 'NONE',  ( -0.3917322834645669549, -0.1049643490035306603, -1.770341207349081181 ) ) ;
#14913=VERTEX_POINT ( 'NONE', #29111 ) ;
#14914=CARTESIAN_POINT ( 'NONE',  ( 0.3460692066303959202, 0.1998031496062993295, -0.6036745406824146620 ) ) ;
#14921=CARTESIAN_POINT ( 'NONE',  ( -0.1049643490035302024, -0.3917322834645671215, -1.101706036745407014 ) ) ;
#14942=CARTESIAN_POINT ( 'NONE',  ( 0.1958661417322834497, 0.3392501089628018329, -1.326752337761467837 ) ) ;
#14952=CARTESIAN_POINT ( 'NONE',  ( -0.2867679344610367109, 0.2867679344610365444, -0.01642351525690478181 ) ) ;
#14956=CARTESIAN_POINT ( 'NONE',  ( -0.4724409448818899238, 0.1265901696524986686, -1.526902887139107490 ) ) ;
#14971=CARTESIAN_POINT ( 'NONE',  ( -0.3420746716998662729, 0.1974969037888702206, 0.2119422572178478181 ) ) ;
#14976=CARTESIAN_POINT ( 'NONE',  ( -0.1070741851644051862, -0.3996062992125986590, -1.723753280839895208 ) ) ;
#14981=CARTESIAN_POINT ( 'NONE',  ( 0.1070741851644053527, 0.3996062992125985480, -1.015091863517060267 ) ) ;
#14982=CARTESIAN_POINT ( 'NONE',  ( 0.3996062992125986035, 0.1070741851644054776, -1.227034120734908029 ) ) ;
#14983=CARTESIAN_POINT ( 'NONE',  ( -9.674558042662121740E-17, 0.3949938075777409963, -0.4724409448818898127 ) ) ;
#14984=CARTESIAN_POINT ( 'NONE',  ( 0.2867679344610366554, -0.2867679344610365444, -0.09055118110236216877 ) ) ;
#14990=CARTESIAN_POINT ( 'NONE',  ( 0.3420746716998660508, -0.1974969037888704149, -1.599081364829396223 ) ) ;
#14994=CARTESIAN_POINT ( 'NONE',  ( 0.3458507752293908943, -0.3458507752293908943, -1.830708661417322913 ) ) ;
#14995=CARTESIAN_POINT ( 'NONE',  ( 0.2749078412854595865, 0.2798680777847445400, -2.755905511811024500 ) ) ;
#15002=CARTESIAN_POINT ( 'NONE',  ( -9.594673741351310580E-17, 0.3917322834645669549, -2.442237902065930388 ) ) ;
#15009=CARTESIAN_POINT ( 'NONE',  ( -0.3392501089628018329, -0.1958661417322836440, -2.809691970307399700 ) ) ;
#15011=( BOUNDED_CURVE ( )  B_SPLINE_CURVE ( 2, ( #61297, #48253, #80279, #75187, #43164, #3655, #30135, #74363, #73949, #11209, #4058, #29725, #28901 ),
 .UNSPECIFIED., .F., .F. ) 
 B_SPLINE_CURVE_WITH_KNOTS ( ( 3, 2, 2, 2, 2, 2, 3 ),
 ( 0.6624999999999999778, 0.6666666666666666297, 0.6708333333333332815, 0.6750000000000000444, 0.6791666666666666963, 0.6833333333333333481, 0.6875000000000000000 ),
 .UNSPECIFIED. ) 
 CURVE ( )  GEOMETRIC_REPRESENTATION_ITEM ( )  RATIONAL_B_SPLINE_CURVE ( ( 1.000000000000000000, 0.9659258262890683122, 1.000000000000000000, 0.9659258262890683122, 1.000000000000000000, 0.9659258262890683122, 1.000000000000000000, 0.9659258262890683122, 1.000000000000000000, 0.9659258262890683122, 1.000000000000000000, 0.9659258262890683122, 1.000000000000000000 ) ) 
 REPRESENTATION_ITEM ( '' )  );
#15012=CARTESIAN_POINT ( 'NONE',  ( -0.3392501089628017219, -0.1958661417322836718, -1.776902887139107490 ) ) ;
#15015=CARTESIAN_POINT ( 'NONE',  ( -0.3949938075777411628, 0.1058382717557497937, -2.237532808398950301 ) ) ;
#15016=ORIENTED_EDGE ( 'NONE', *, *, #42744, .T. ) ;
#15020=CARTESIAN_POINT ( 'NONE',  ( -0.1998031496062994683, 0.3460692066303958092, -0.8005249343832020470 ) ) ;
#15022=CARTESIAN_POINT ( 'NONE',  ( -0.4724409448818898682, 5.785732909357575061E-17, -2.755905511811024056 ) ) ;
#15025=CARTESIAN_POINT ( 'NONE',  ( -0.3392501089628019995, 0.1958661417322832277, -0.1108923884514436548 ) ) ;
#15037=CARTESIAN_POINT ( 'NONE',  ( -0.1265901696524986964, -0.4724409448818899238, -1.174540682414698001 ) ) ;
#15039=CARTESIAN_POINT ( 'NONE',  ( -0.3392501089628017219, -0.1958661417322836718, -0.8320209973753279753 ) ) ;
#15040=CARTESIAN_POINT ( 'NONE',  ( 0.2867679344610366554, 0.2867679344610366554, -2.269685039370078705 ) ) ;
#15043=CARTESIAN_POINT ( 'NONE',  ( -0.3996062992125986590, 0.1070741851644051723, -0.2670603674540683037 ) ) ;
#15048=CARTESIAN_POINT ( 'NONE',  ( -0.3392501089628018329, -0.1958661417322836440, 0.1824340139445687625 ) ) ;
#15050=CARTESIAN_POINT ( 'NONE',  ( -0.04642319063763892389, -0.3917322834645671215, -0.003003439681892647057 ) ) ;
#15055=CARTESIAN_POINT ( 'NONE',  ( -0.2867679344610365999, 0.2867679344610364889, -2.059055118110236116 ) ) ;
#15059=CARTESIAN_POINT ( 'NONE',  ( -0.3458507752293906723, -0.3458507752293910609, -0.4507874015748031815 ) ) ;
#15069=DIRECTION ( 'NONE',  ( 0.000000000000000000, 0.000000000000000000, 1.000000000000000000 ) ) ;
#15072=CARTESIAN_POINT ( 'NONE',  ( 0.3996062992125986035, -0.1070741851644052972, -1.448162729658792669 ) ) ;
#15079=CARTESIAN_POINT ( 'NONE',  ( 0.3460692066303959202, -0.1998031496062991630, -0.02427821522309713681 ) ) ;
#15081=CARTESIAN_POINT ( 'NONE',  ( 4.893765752498283924E-17, -0.3996062992125986035, -0.2362204724409449064 ) ) ;
#15082=CARTESIAN_POINT ( 'NONE',  ( -0.1958661417322833942, -0.3392501089628018884, -2.424559998196537336 ) ) ;
#15088=CARTESIAN_POINT ( 'NONE',  ( 0.3917322834645669549, 0.1049643490035304660, -2.571522309711286258 ) ) ;
#15097=CARTESIAN_POINT ( 'NONE',  ( 0.1958661417322834775, 0.3392501089628018884, -0.4560560611886632087 ) ) ;
#15113=CARTESIAN_POINT ( 'NONE',  ( -0.3392501089628019995, 0.1958661417322832277, -0.8057742782152230721 ) ) ;
#15116=CARTESIAN_POINT ( 'NONE',  ( -0.1058382717557503211, 0.3949938075777409408, -1.108923884514435798 ) ) ;
#15131=CARTESIAN_POINT ( 'NONE',  ( 0.3996062992125986035, 2.446882876249141962E-17, -1.692913385826771533 ) ) ;
#15133=CARTESIAN_POINT ( 'NONE',  ( -0.1998031496062994405, 0.3460692066303957537, -1.192257217847769057 ) ) ;
#15134=CARTESIAN_POINT ( 'NONE',  ( 0.2925321140481932369, 0.2925321140481932369, -0.5295275590551181688 ) ) ;
#15136=CARTESIAN_POINT ( 'NONE',  ( 0.1265901696524989462, 0.4724409448818897572, -0.1509186351706036378 ) ) ;
#15137=CARTESIAN_POINT ( 'NONE',  ( -0.2867679344610365999, 0.2867679344610364889, -2.309055118110235671 ) ) ;
#15143=CARTESIAN_POINT ( 'NONE',  ( -0.4091458600556402980, -0.2362204724409451284, -2.019028871391076230 ) ) ;
#15146=CARTESIAN_POINT ( 'NONE',  ( -0.3949938075777411073, 0.1058382717557497660, -1.999343832020997747 ) ) ;
#15156=CARTESIAN_POINT ( 'NONE',  ( -0.1998031496062994405, 0.3460692066303957537, -2.452099737532808188 ) ) ;
#15157=CARTESIAN_POINT ( 'NONE',  ( -0.3392501089628018329, -0.1958661417322836440, -2.179770710464879802 ) ) ;
#15172=CARTESIAN_POINT ( 'NONE',  ( 0.2925321140481932369, -0.2925321140481931814, -0.1751968503937007537 ) ) ;
#15174=CARTESIAN_POINT ( 'NONE',  ( 0.1958661417322834775, 0.3392501089628018884, -1.331364829396325611 ) ) ;
#15183=CARTESIAN_POINT ( 'NONE',  ( 0.3460692066303958092, 0.1998031496062993018, -1.152887139107611425 ) ) ;
#15189=CARTESIAN_POINT ( 'NONE',  ( 0.3974711515625343194, 0.004548682155565822449, -1.220472440944882164 ) ) ;
#15198=CARTESIAN_POINT ( 'NONE',  ( 0.3460692066303959202, 0.1998031496062993295, -0.2887139107611548794 ) ) ;
#15201=CARTESIAN_POINT ( 'NONE',  ( -0.1958661417322836718, 0.3392501089628017219, -2.052493438320210029 ) ) ;
#15213=CARTESIAN_POINT ( 'NONE',  ( -0.1958661417322834497, -0.3392501089628018884, -1.405492495241783102 ) ) ;
#15219=CARTESIAN_POINT ( 'NONE',  ( -0.1958661417322836995, 0.3392501089628017219, -2.844507504758217120 ) ) ;
#15221=VERTEX_POINT ( 'NONE', #65679 ) ;
#15229=CARTESIAN_POINT ( 'NONE',  ( 4.797336870675656522E-17, -0.3917322834645670104, -2.210629921259842590 ) ) ;
#15236=CARTESIAN_POINT ( 'NONE',  ( -0.1070741851644056997, 0.3996062992125984925, -0.08333333333333335646 ) ) ;
#15238=CARTESIAN_POINT ( 'NONE',  ( 0.3460692066303959202, 0.1998031496062993295, -1.706036745406824151 ) ) ;
#15244=CARTESIAN_POINT ( 'NONE',  ( -0.3458507752293909498, 0.3458507752293907833, -0.7263779527559056648 ) ) ;
#15248=CARTESIAN_POINT ( 'NONE',  ( -0.3949938075777408852, -0.1058382717557502933, -0.2801837270341207553 ) ) ;
#15253=EDGE_CURVE ( 'NONE', #14101, #28644, #19367, .T. ) ;
#15254=CARTESIAN_POINT ( 'NONE',  ( -9.674558042662122972E-17, 0.3949938075777409963, -0.3917322834645669549 ) ) ;
#15260=CARTESIAN_POINT ( 'NONE',  ( 5.785732909357575061E-17, -0.4724409448818898682, -2.755905511811023612 ) ) ;
#15261=CARTESIAN_POINT ( 'NONE',  ( -0.2925321140481932369, 0.2925321140481931259, -1.198818897637795367 ) ) ;
#15263=CARTESIAN_POINT ( 'NONE',  ( 0.3917322834645670104, -0.1049643490035303411, -0.8910761154855640909 ) ) ;
#15276=CARTESIAN_POINT ( 'NONE',  ( 0.4724409448818898682, 2.892866454678787531E-17, -2.872047244094488416 ) ) ;
#15293=CARTESIAN_POINT ( 'NONE',  ( -0.3996062992125985480, -0.1070741851644057135, -0.8333333333333332593 ) ) ;
#15297=CARTESIAN_POINT ( 'NONE',  ( 0.4091458600556403535, 0.2362204724409449896, -0.1312335958005249326 ) ) ;
#15298=CARTESIAN_POINT ( 'NONE',  ( 0.3949938075777411073, -0.1058382717557499464, -2.316272965879265122 ) ) ;
#15300=CARTESIAN_POINT ( 'NONE',  ( -0.3392501089628017219, -0.1958661417322836718, -0.9895013123359579499 ) ) ;
#15306=CARTESIAN_POINT ( 'NONE',  ( -0.1049643490035301746, -0.3917322834645670659, -0.4671722852680298410 ) ) ;
#15312=CARTESIAN_POINT ( 'NONE',  ( 0.3458507752293908943, 0.3458507752293908943, -1.082677165354330562 ) ) ;
#15313=CARTESIAN_POINT ( 'NONE',  ( 0.1958661417322836718, -0.3392501089628017219, -1.663405142553492810 ) ) ;
#15319=CARTESIAN_POINT ( 'NONE',  ( 0.3917322834645669549, 0.1049643490035304660, -0.6817585301837268963 ) ) ;
#15328=CARTESIAN_POINT ( 'NONE',  ( -0.2155943732389342393, -0.3272402980651248905, -1.929133858267717105 ) ) ;
#15329=CARTESIAN_POINT ( 'NONE',  ( -0.3917322834645669549, -0.1049643490035306603, -2.242782152230970993 ) ) ;
#15331=CARTESIAN_POINT ( 'NONE',  ( 0.3996062992125986035, 2.446882876249141962E-17, -0.4330708661417322913 ) ) ;
#15332=ORIENTED_EDGE ( 'NONE', *, *, #21932, .T. ) ;
#15338=CARTESIAN_POINT ( 'NONE',  ( 0.1049643490035303689, 0.3917322834645670104, -1.337926509186352142 ) ) ;
#15341=CARTESIAN_POINT ( 'NONE',  ( 0.2925321140481932369, 0.2925321140481932369, -1.946850393700787274 ) ) ;
#15351=CARTESIAN_POINT ( 'NONE',  ( 0.3917322834645670104, -0.1049643490035303411, 0.05380577427821527092 ) ) ;
#15359=CARTESIAN_POINT ( 'NONE',  ( 0.2867679344610365999, 0.2867679344610365999, -1.162710343010812108 ) ) ;
#15368=CARTESIAN_POINT ( 'NONE',  ( -9.594673741351313045E-17, 0.3917322834645670659, 0.003261524113173961108 ) ) ;
#15370=CARTESIAN_POINT ( 'NONE',  ( 0.3458507752293908943, -0.3458507752293908943, -0.2559055118110235560 ) ) ;
#15371=CARTESIAN_POINT ( 'NONE',  ( 0.3458507752293908943, 0.3458507752293908943, -1.631889763779527325 ) ) ;
#15386=CARTESIAN_POINT ( 'NONE',  ( -0.3996062992125984925, -0.1070741851644056858, -2.642388451443570041 ) ) ;
#15391=CARTESIAN_POINT ( 'NONE',  ( 0.3460692066303958092, 0.1998031496062993018, -1.782808398950131323 ) ) ;
#15396=CARTESIAN_POINT ( 'NONE',  ( 4.893765752498283308E-17, -0.3996062992125985480, -0.9429133858267716439 ) ) ;
#15397=CARTESIAN_POINT ( 'NONE',  ( 0.3460692066303959202, 0.1998031496062993295, -1.391076115485564424 ) ) ;
#15399=CARTESIAN_POINT ( 'NONE',  ( 0.3949938075777409963, 2.418639510665530435E-17, -1.062992125984251857 ) ) ;
#15400=CARTESIAN_POINT ( 'NONE',  ( 0.3996062992125986035, 2.446882876249141962E-17, -2.322834645669291209 ) ) ;
#15403=CARTESIAN_POINT ( 'NONE',  ( -0.1049643490035307020, 0.3917322834645669549, -0.3136482939632545541 ) ) ;
#15407=CARTESIAN_POINT ( 'NONE',  ( 0.2891555358219910499, 0.2891555358219910499, -1.631889763779527991 ) ) ;
#15411=CARTESIAN_POINT ( 'NONE',  ( -0.4091458600556405756, 0.2362204724409446288, -1.916010498687664043 ) ) ;
#15419=CARTESIAN_POINT ( 'NONE',  ( 0.3392501089628018329, -0.1958661417322834497, -2.389744463745719916 ) ) ;
#15426=CARTESIAN_POINT ( 'NONE',  ( 0.1049643490035304938, -0.3917322834645669549, 0.1450131233595799429 ) ) ;
#15429=CARTESIAN_POINT ( 'NONE',  ( -0.1958661417322836718, 0.3392501089628017219, -1.737532808398950079 ) ) ;
#15432=CARTESIAN_POINT ( 'NONE',  ( -9.674558042662121740E-17, 0.3949938075777409963, -2.362204724409449064 ) ) ;
#15437=CARTESIAN_POINT ( 'NONE',  ( 4.893765752498283924E-17, -0.3996062992125986035, -0.5511811023622047445 ) ) ;
#15442=CARTESIAN_POINT ( 'NONE',  ( 0.1049643490035303689, 0.3917322834645670104, -0.07808398950131241467 ) ) ;
#15450=CARTESIAN_POINT ( 'NONE',  ( -0.3917322834645670104, -7.196005306013484475E-17, -0.03149606299212594218 ) ) ;
#15455=CARTESIAN_POINT ( 'NONE',  ( -0.3458507752293909498, 0.3458507752293907833, -1.437007874015747921 ) ) ;
#15457=CARTESIAN_POINT ( 'NONE',  ( 0.2867679344610365999, 0.2867679344610365999, -0.6023622047244093780 ) ) ;
#15458=CARTESIAN_POINT ( 'NONE',  ( -0.1049643490035307020, 0.3917322834645669549, -2.453412073490813583 ) ) ;
#15461=CARTESIAN_POINT ( 'NONE',  ( 0.3460692066303958092, 0.1998031496062993018, 0.1069553805774277888 ) ) ;
#15467=CARTESIAN_POINT ( 'NONE',  ( -0.2867679344610364334, -0.2867679344610368219, 0.01839201919391258294 ) ) ;
#15469=CARTESIAN_POINT ( 'NONE',  ( -0.1049643490035301885, -0.3917322834645671215, -0.1568241469816273326 ) ) ;
#15474=CARTESIAN_POINT ( 'NONE',  ( -0.1958661417322834220, -0.3392501089628018884, -2.104986876640420057 ) ) ;
#15479=CARTESIAN_POINT ( 'NONE',  ( 0.4724409448818897572, -0.1265901696524988906, -0.3458005249343831244 ) ) ;
#15488=CARTESIAN_POINT ( 'NONE',  ( -0.4724409448818898682, -8.678599364036362592E-17, -2.005905511811023612 ) ) ;
#15490=CARTESIAN_POINT ( 'NONE',  ( -0.3996062992125986590, 0.1070741851644051723, -1.684383202099737353 ) ) ;
#15498=FACE_OUTER_BOUND ( 'NONE', #42007, .T. ) ;
#15499=CARTESIAN_POINT ( 'NONE',  ( 0.3460692066303959202, 0.1998031496062993295, -0.2887139107611548794 ) ) ;
#15500=CARTESIAN_POINT ( 'NONE',  ( -9.674558042662121740E-17, 0.3949938075777409963, -5.756223643949423463E-17 ) ) ;
#15505=CARTESIAN_POINT ( 'NONE',  ( 0.1958661417322834775, 0.3392501089628018884, -2.276246719160105236 ) ) ;
#15510=CARTESIAN_POINT ( 'NONE',  ( -0.2362204724409447953, -0.4091458600556404646, -0.8530183727034120755 ) ) ;
#15516=CARTESIAN_POINT ( 'NONE',  ( -0.1958661417322833942, -0.3392501089628018884, -0.3773159037083483325 ) ) ;
#15529=CARTESIAN_POINT ( 'NONE',  ( 0.2867679344610365999, 0.2867679344610365999, -0.6023622047244093780 ) ) ;
#15532=CARTESIAN_POINT ( 'NONE',  ( 0.1974969037888706369, -0.3420746716998659953, -1.194225721784776928 ) ) ;
#15549=CARTESIAN_POINT ( 'NONE',  ( 0.1998031496062994405, -0.3460692066303958092, -1.666666666666666741 ) ) ;
#15552=CARTESIAN_POINT ( 'NONE',  ( 0.1998031496062992463, 0.3460692066303959202, -1.323490813648294129 ) ) ;
#15553=CARTESIAN_POINT ( 'NONE',  ( -0.1070741851644051862, -0.3996062992125986590, -0.4639107611548556331 ) ) ;
#15555=CARTESIAN_POINT ( 'NONE',  ( -0.4724409448818895907, -0.1265901696524993070, -0.04593175853018372640 ) ) ;
#15556=CARTESIAN_POINT ( 'NONE',  ( -0.3392501089628017219, -0.1958661417322836718, -2.499343832020997080 ) ) ;
#15562=CARTESIAN_POINT ( 'NONE',  ( -0.4724409448818895907, -0.1265901696524993070, -1.854986876640420057 ) ) ;
#15565=CARTESIAN_POINT ( 'NONE',  ( -0.3949938075777408852, -0.1058382717557502933, -1.697506561679790194 ) ) ;
#15576=CARTESIAN_POINT ( 'NONE',  ( -0.3460692066303960313, 0.1998031496062989965, -2.465223097112860806 ) ) ;
#15577=CARTESIAN_POINT ( 'NONE',  ( -0.2867679344610364334, -0.2867679344610368219, -2.501293020176166504 ) ) ;
#15586=CARTESIAN_POINT ( 'NONE',  ( 0.2362204724409451007, -0.4091458600556402980, -0.8792650918635170898 ) ) ;
#15590=CARTESIAN_POINT ( 'NONE',  ( -0.3996062992125984925, -0.1070741851644056858, -0.2801837270341207553 ) ) ;
#15592=CARTESIAN_POINT ( 'NONE',  ( 0.1958661417322834775, 0.3392501089628018884, -1.803805774278215202 ) ) ;
#15601=CARTESIAN_POINT ( 'NONE',  ( -0.1998031496062991630, -0.3460692066303959202, -0.9297900262467192478 ) ) ;
#15614=AXIS2_PLACEMENT_3D ( 'NONE', #5411, #31487, #11746 ) ;
#15618=CARTESIAN_POINT ( 'NONE',  ( 0.1070741851644053527, 0.3996062992125986590, -0.3083989501312335846 ) ) ;
#15621=CARTESIAN_POINT ( 'NONE',  ( 0.3917322834645670104, 2.398668435337828261E-17, -2.314960629921259727 ) ) ;
#15632=CARTESIAN_POINT ( 'NONE',  ( -0.3392501089628019439, 0.1958661417322832554, -1.523602731462254889 ) ) ;
#15638=CARTESIAN_POINT ( 'NONE',  ( -0.3420746716998659953, -0.1974969037888706647, 0.1049868766404198905 ) ) ;
#15648=CARTESIAN_POINT ( 'NONE',  ( -0.2867679344610365999, 0.2867679344610364889, -2.151574803149605586 ) ) ;
#15655=CARTESIAN_POINT ( 'NONE',  ( 0.3460692066303958092, 0.1998031496062993018, 0.1069553805774278027 ) ) ;
#15657=CARTESIAN_POINT ( 'NONE',  ( 0.3460692066303959202, 0.1998031496062993295, -1.863517060367454015 ) ) ;
#15662=CARTESIAN_POINT ( 'NONE',  ( -0.4724409448818898682, -8.678599364036362592E-17, -0.7460629921259841479 ) ) ;
#15665=CARTESIAN_POINT ( 'NONE',  ( -0.2891555358219909388, -0.2891555358219912164, -0.4507874015748032925 ) ) ;
#15670=CARTESIAN_POINT ( 'NONE',  ( 0.2891555358219910499, -0.2891555358219909944, -0.4901574803149606474 ) ) ;
#15671=EDGE_CURVE ( 'NONE', #25317, #63931, #1005, .T. ) ;
#15678=CARTESIAN_POINT ( 'NONE',  ( 0.2925321140481932369, 0.2925321140481932369, -1.474409448818897905 ) ) ;
#15681=CARTESIAN_POINT ( 'NONE',  ( 0.3917322834645669549, 0.1049643490035304660, -0.9041994750656167090 ) ) ;
#15693=CARTESIAN_POINT ( 'NONE',  ( -0.4724409448818899238, 0.1265901696524986964, -0.2670603674540682482 ) ) ;
#15711=CARTESIAN_POINT ( 'NONE',  ( -0.3460692066303960868, 0.1998031496062990242, -0.8136482939632546652 ) ) ;
#15716=CARTESIAN_POINT ( 'NONE',  ( 0.2362204724409451007, -0.4091458600556402980, 0.06561679790026246628 ) ) ;
#15717=CARTESIAN_POINT ( 'NONE',  ( 0.3949938075777409963, 2.418639510665530435E-17, -2.322834645669291209 ) ) ;
#15720=CARTESIAN_POINT ( 'NONE',  ( -9.594673741351313045E-17, 0.3917322834645670104, -1.094488188976378007 ) ) ;
#15727=CARTESIAN_POINT ( 'NONE',  ( -0.1958661417322836440, 0.3392501089628016664, -0.4081171671577935034 ) ) ;
#15734=CARTESIAN_POINT ( 'NONE',  ( -9.787531504996567848E-17, 0.3996062992125986035, -2.834645669291338432 ) ) ;
#15735=CARTESIAN_POINT ( 'NONE',  ( 4.797336870675656522E-17, -0.3917322834645670659, -1.492801468012810329 ) ) ;
#15742=CARTESIAN_POINT ( 'NONE',  ( -0.3392501089628019995, 0.1958661417322832277, -1.055774278215223294 ) ) ;
#15752=CARTESIAN_POINT ( 'NONE',  ( -0.3392501089628017219, -0.1958661417322836718, -2.249343832020997525 ) ) ;
#15753=ORIENTED_EDGE ( 'NONE', *, *, #59403, .F. ) ;
#15761=CARTESIAN_POINT ( 'NONE',  ( 0.1958661417322836440, -0.3392501089628017219, -1.278871391076115582 ) ) ;
#15762=EDGE_CURVE ( 'NONE', #25718, #2797, #52089, .T. ) ;
#15763=CARTESIAN_POINT ( 'NONE',  ( -9.787531504996566615E-17, 0.3996062992125985480, -2.281496062992125928 ) ) ;
#15772=CARTESIAN_POINT ( 'NONE',  ( -0.3996062992125985480, -7.340648628747423112E-17, -2.005905511811023612 ) ) ;
#15781=CARTESIAN_POINT ( 'NONE',  ( 0.1049643490035304522, -0.3917322834645668994, -1.425177534611861585 ) ) ;
#15790=CARTESIAN_POINT ( 'NONE',  ( -0.2867679344610367109, 0.2867679344610365444, -0.3313841451781647240 ) ) ;
#15793=CARTESIAN_POINT ( 'NONE',  ( 0.4724409448818898127, -0.1265901696524988629, -0.2690288713910760632 ) ) ;
#15795=CARTESIAN_POINT ( 'NONE',  ( -0.4724409448818899238, 0.1265901696524986686, -1.684383202099737353 ) ) ;
#15814=CARTESIAN_POINT ( 'NONE',  ( -0.3949938075777411073, 0.1058382717557497660, 0.2053805774278214813 ) ) ;
#15819=CARTESIAN_POINT ( 'NONE',  ( -0.3996062992125986590, 0.1070741851644051723, -2.314304461942256808 ) ) ;
#15826=CARTESIAN_POINT ( 'NONE',  ( -0.1070741851644056997, 0.3996062992125986035, -1.896325459317584894 ) ) ;
#15827=CARTESIAN_POINT ( 'NONE',  ( 0.3949938075777411073, -0.1058382717557499464, -1.213910761154855633 ) ) ;
#15828=CARTESIAN_POINT ( 'NONE',  ( -0.3996062992125987146, 0.1070741851644051862, -2.552493438320210029 ) ) ;
#15830=CARTESIAN_POINT ( 'NONE',  ( -0.2867679344610364334, -0.2867679344610367109, -0.3661417322834645272 ) ) ;
#15834=CARTESIAN_POINT ( 'NONE',  ( 0.3420746716998660508, -0.1974969037888704149, -2.229002624671915900 ) ) ;
#15838=CARTESIAN_POINT ( 'NONE',  ( -0.4724409448818898682, -8.678599364036362592E-17, -2.244094488188976388 ) ) ;
#15846=CARTESIAN_POINT ( 'NONE',  ( -0.1049643490035301746, -0.3917322834645670659, -2.829377009677478405 ) ) ;
#15849=CARTESIAN_POINT ( 'NONE',  ( 0.4091458600556404646, -0.2362204724409448231, -2.467191601049868677 ) ) ;
#15853=CARTESIAN_POINT ( 'NONE',  ( 0.2867679344610365999, 0.2867679344610365999, -0.2224409448818898127 ) ) ;
#15855=CARTESIAN_POINT ( 'NONE',  ( 0.1049643490035303689, 0.3917322834645670104, -2.347769028871391050 ) ) ;
#15858=CARTESIAN_POINT ( 'NONE',  ( -0.3420746716998659953, -0.1974969037888706647, -2.099737532808398921 ) ) ;
#15863=CARTESIAN_POINT ( 'NONE',  ( 0.3460692066303959757, -0.1998031496062991907, -0.8923884514435694859 ) ) ;
#15868=CARTESIAN_POINT ( 'NONE',  ( 0.3392501089628018329, 0.1958661417322835607, 0.09908136482939623735 ) ) ;
#15878=CARTESIAN_POINT ( 'NONE',  ( 0.3458507752293908943, -0.3458507752293908943, -1.200787401574803015 ) ) ;
#15880=CARTESIAN_POINT ( 'NONE',  ( -0.1958661417322834220, -0.3392501089628018884, -0.8451443569553805935 ) ) ;
#15881=CARTESIAN_POINT ( 'NONE',  ( -0.3917322834645671215, 0.1049643490035301469, -2.479658792650918375 ) ) ;
#15884=CARTESIAN_POINT ( 'NONE',  ( -0.1070741851644051862, -0.3996062992125986590, -0.3064304461942257141 ) ) ;
#15888=CARTESIAN_POINT ( 'NONE',  ( 0.1049643490035304522, -0.3917322834645668994, -0.1653350149268222880 ) ) ;
#15890=CARTESIAN_POINT ( 'NONE',  ( 0.1958661417322834775, 0.3392501089628018884, -0.3864829396325459854 ) ) ;
#15896=CARTESIAN_POINT ( 'NONE',  ( -0.1049643490035302024, -0.3917322834645671215, -2.426509186351705427 ) ) ;
#15899=CARTESIAN_POINT ( 'NONE',  ( -0.2362204724409447953, -0.4091458600556404646, -0.2998687664041995160 ) ) ;
#15909=CARTESIAN_POINT ( 'NONE',  ( 0.2925321140481932369, -0.2925321140481931814, -1.592519685039370358 ) ) ;
#15918=CARTESIAN_POINT ( 'NONE',  ( -0.1998031496062994405, 0.3460692066303957537, -0.2473753280839895152 ) ) ;
#15920=CARTESIAN_POINT ( 'NONE',  ( 0.3996062992125986035, 0.1070741851644054776, -0.4396325459317584339 ) ) ;
#15921=CARTESIAN_POINT ( 'NONE',  ( 0.3917322834645670659, 2.398668435337828261E-17, -2.792014066438007092 ) ) ;
#15926=CARTESIAN_POINT ( 'NONE',  ( 0.3949938075777408852, 0.1058382717557500435, -0.8313648293963256108 ) ) ;
#15931=CARTESIAN_POINT ( 'NONE',  ( -0.3458507752293906723, -0.3458507752293910609, -0.8464566929133857665 ) ) ;
#15932=CARTESIAN_POINT ( 'NONE',  ( -0.2925321140481930704, -0.2925321140481933480, -2.263779527559055094 ) ) ;
#15934=ORIENTED_EDGE ( 'NONE', *, *, #17054, .F. ) ;
#15935=CARTESIAN_POINT ( 'NONE',  ( -0.3392501089628017219, -0.1958661417322836995, -0.3641925441282957698 ) ) ;
#15948=CARTESIAN_POINT ( 'NONE',  ( -0.2867679344610364334, -0.2867679344610367109, -0.5236220472440944462 ) ) ;
#15951=CARTESIAN_POINT ( 'NONE',  ( -0.3420746716998659953, -0.1974969037888706647, -0.9973753280839895430 ) ) ;
#15955=CARTESIAN_POINT ( 'NONE',  ( 0.3996062992125986035, 2.446882876249141962E-17, 0.03937007874015747283 ) ) ;
#15967=CARTESIAN_POINT ( 'NONE',  ( 0.1070741851644053527, 0.3996062992125986590, -1.568241469816272993 ) ) ;
#15970=CARTESIAN_POINT ( 'NONE',  ( -0.3460692066303960313, 0.1998031496062989965, -1.362860892388451539 ) ) ;
#15971=CARTESIAN_POINT ( 'NONE',  ( 0.2925321140481932369, 0.2925321140481932369, -0.6870078740157479213 ) ) ;
#15974=CARTESIAN_POINT ( 'NONE',  ( 0.3458507752293908943, -0.3458507752293908943, -0.09842519685039372024 ) ) ;
#15975=CARTESIAN_POINT ( 'NONE',  ( 0.1958661417322836440, -0.3392501089628017219, -2.538713910761154491 ) ) ;
#15981=CARTESIAN_POINT ( 'NONE',  ( -0.3458507752293909498, 0.3458507752293907833, -1.986220472440944906 ) ) ;
#15984=CARTESIAN_POINT ( 'NONE',  ( 0.1974969037888706092, -0.3420746716998660508, -1.900918635170603554 ) ) ;
#15987=DIRECTION ( 'NONE',  ( 1.000000000000000000, 0.000000000000000000, 0.000000000000000000 ) ) ;
#15993=CARTESIAN_POINT ( 'NONE',  ( 0.2925321140481932369, -0.2925321140481931814, -2.537401574803149984 ) ) ;
#15995=CARTESIAN_POINT ( 'NONE',  ( -0.1049643490035306742, 0.3917322834645668994, -2.606279896816586117 ) ) ;
#16007=CARTESIAN_POINT ( 'NONE',  ( -0.3460692066303960313, 0.1998031496062989965, -0.1030183727034120617 ) ) ;
#16010=CARTESIAN_POINT ( 'NONE',  ( 0.1049643490035303689, 0.3917322834645670104, -1.652887139107611425 ) ) ;
#16019=CARTESIAN_POINT ( 'NONE',  ( 0.3460692066303959202, -0.1998031496062991630, -0.8116797900262466836 ) ) ;
#16032=CARTESIAN_POINT ( 'NONE',  ( 0.2925321140481932369, 0.2925321140481932369, -0.2952755905511811885 ) ) ;
#16035=CARTESIAN_POINT ( 'NONE',  ( -0.3917322834645669549, -0.1049643490035306603, -2.085301837270341352 ) ) ;
#16045=CARTESIAN_POINT ( 'NONE',  ( 0.3917322834645668994, 0.1049643490035304522, -1.622027928312648859 ) ) ;
#16051=CARTESIAN_POINT ( 'NONE',  ( -0.3392501089628019995, 0.1958661417322831999, -2.857630864338269738 ) ) ;
#16059=CARTESIAN_POINT ( 'NONE',  ( -0.3392501089628017219, -0.1958661417322836995, -1.309074433892075451 ) ) ;
#16061=CARTESIAN_POINT ( 'NONE',  ( 0.1958661417322834775, 0.3392501089628018884, -2.118766404199475151 ) ) ;
#16068=CARTESIAN_POINT ( 'NONE',  ( 0.1070741851644053388, 0.3996062992125986035, -0.07020997375328083545 ) ) ;
#16070=CARTESIAN_POINT ( 'NONE',  ( -0.1998031496062994683, 0.3460692066303958092, -1.745406824146981561 ) ) ;
#16074=CARTESIAN_POINT ( 'NONE',  ( 0.4091458600556403535, 0.2362204724409449896, -0.6804461942257218343 ) ) ;
#16078=CARTESIAN_POINT ( 'NONE',  ( -9.674558042662122972E-17, 0.3949938075777409963, -0.7066929133858269596 ) ) ;
#16083=CARTESIAN_POINT ( 'NONE',  ( 0.3949938075777409963, 2.418639510665530743E-17, -0.3523622047244094335 ) ) ;
#16087=CARTESIAN_POINT ( 'NONE',  ( 0.3458507752293908943, -0.3458507752293908943, -0.1751968503937007537 ) ) ;
#16090=CARTESIAN_POINT ( 'NONE',  ( 0.3460692066303958092, 0.1998031496062993018, -1.310367454068241733 ) ) ;
#16092=CARTESIAN_POINT ( 'NONE',  ( 0.3917322834645670104, 2.398668435337828261E-17, -0.8976377952755905110 ) ) ;
#16094=CARTESIAN_POINT ( 'NONE',  ( -0.3814249188612186536, 0.08989863709126630353, -1.138966262901370454E-17 ) ) ;
#16102=CARTESIAN_POINT ( 'NONE',  ( -1.157146581871515012E-16, 0.4724409448818898682, -0.2342519685039370358 ) ) ;
#16120=CARTESIAN_POINT ( 'NONE',  ( 0.1070741851644053666, 0.3996062992125986035, -1.095800524934382958 ) ) ;
#16124=CARTESIAN_POINT ( 'NONE',  ( 0.2362204724409449064, 0.4091458600556404646, 0.01312335958005249326 ) ) ;
#16125=CARTESIAN_POINT ( 'NONE',  ( 0.2891555358219910499, 0.2891555358219910499, -2.500000000000000444 ) ) ;
#16128=CARTESIAN_POINT ( 'NONE',  ( -9.594673741351313045E-17, 0.3917322834645670104, -0.7795275590551180578 ) ) ;
#16136=CARTESIAN_POINT ( 'NONE',  ( -0.2867679344610364334, -0.2867679344610368219, -0.2965686107273473038 ) ) ;
#16143=CARTESIAN_POINT ( 'NONE',  ( -0.3460692066303960868, 0.1998031496062990242, -2.860892388451443669 ) ) ;
#16144=CARTESIAN_POINT ( 'NONE',  ( -0.1049643490035307158, 0.3917322834645670104, -1.735583620243781322 ) ) ;
#16150=CARTESIAN_POINT ( 'NONE',  ( -0.3917322834645670104, -7.196005306013484475E-17, -1.068897637795275690 ) ) ;
#16159=CARTESIAN_POINT ( 'NONE',  ( 4.797336870675656522E-17, -0.3917322834645670104, -2.275590551181102317 ) ) ;
#16162=EDGE_LOOP ( 'NONE', ( #54711, #22758, #25100, #74953 ) ) ;
#16166=DIRECTION ( 'NONE',  ( 0.000000000000000000, 0.000000000000000000, 1.000000000000000000 ) ) ;
#16167=CARTESIAN_POINT ( 'NONE',  ( 4.797336870675656522E-17, -0.3917322834645670104, -0.6358267716535433989 ) ) ;
#16169=CARTESIAN_POINT ( 'NONE',  ( 0.3458507752293908943, -0.3458507752293908943, -0.01771653543307087630 ) ) ;
#16171=CARTESIAN_POINT ( 'NONE',  ( 0.2867679344610365999, -0.2867679344610365444, -1.285433070866141669 ) ) ;
#16172=CARTESIAN_POINT ( 'NONE',  ( -0.3996062992125984925, -0.1070741851644056858, -2.327427821522309426 ) ) ;
#16181=CARTESIAN_POINT ( 'NONE',  ( 0.2925321140481931814, -0.2925321140481931259, -2.064960629921259727 ) ) ;
#16183=CARTESIAN_POINT ( 'NONE',  ( -0.3917322834645671215, 0.1049643490035301469, 0.1325459317585302166 ) ) ;
#16190=CARTESIAN_POINT ( 'NONE',  ( -0.1958661417322834497, -0.3392501089628018884, -1.405492495241783102 ) ) ;
#16200=CARTESIAN_POINT ( 'NONE',  ( 0.3392501089628018884, -0.1958661417322833942, -0.5741662974091357174 ) ) ;
#16203=CARTESIAN_POINT ( 'NONE',  ( -0.4724409448818895907, -0.1265901696524993070, -2.012467191601049699 ) ) ;
#16224=CARTESIAN_POINT ( 'NONE',  ( -0.3460692066303960313, 0.1998031496062989965, -2.150262467191601079 ) ) ;
#16229=CARTESIAN_POINT ( 'NONE',  ( -0.3460692066303960868, 0.1998031496062990242, -1.916010498687664043 ) ) ;
#16230=CARTESIAN_POINT ( 'NONE',  ( 0.3949938075777409963, 2.418639510665530435E-17, -0.9055118110236219930 ) ) ;
#16231=CARTESIAN_POINT ( 'NONE',  ( 0.3460692066303959757, -0.1998031496062991907, -2.467191601049868677 ) ) ;
#16233=CARTESIAN_POINT ( 'NONE',  ( 0.1958661417322836440, -0.3392501089628017219, -0.2414698162729658204 ) ) ;
#16237=CARTESIAN_POINT ( 'NONE',  ( -0.1974969037888706924, 0.3420746716998658843, -2.294619422572178102 ) ) ;
#16242=CARTESIAN_POINT ( 'NONE',  ( -0.3458507752293906723, -0.3458507752293910609, -2.421259842519684735 ) ) ;
#16243=CARTESIAN_POINT ( 'NONE',  ( 0.3996062992125986035, 0.1070741851644054776, -1.856955380577427928 ) ) ;
#16245=ORIENTED_EDGE ( 'NONE', *, *, #24858, .T. ) ;
#16246=ORIENTED_EDGE ( 'NONE', *, *, #52589, .T. ) ;
#16251=CARTESIAN_POINT ( 'NONE',  ( -0.3392501089628018329, -0.1958661417322836440, -2.809691970307399700 ) ) ;
#16254=CARTESIAN_POINT ( 'NONE',  ( 0.2362204724409451007, -0.4091458600556402980, -2.454068241469816058 ) ) ;
#16259=CARTESIAN_POINT ( 'NONE',  ( -0.3392501089628017219, -0.1958661417322836718, -0.1371391076115486551 ) ) ;
#16261=CARTESIAN_POINT ( 'NONE',  ( -0.1049643490035307020, 0.3917322834645669549, -2.203412073490814027 ) ) ;
#16265=CARTESIAN_POINT ( 'NONE',  ( 0.1058382717557500713, -0.3949938075777409408, -2.132545931758530244 ) ) ;
#16269=CARTESIAN_POINT ( 'NONE',  ( 0.2925321140481932369, -0.2925321140481932369, -1.200787401574803015 ) ) ;
#16275=CARTESIAN_POINT ( 'NONE',  ( -0.3392501089628017219, -0.1958661417322836718, 0.02034120734908127781 ) ) ;
#16287=CARTESIAN_POINT ( 'NONE',  ( 0.4724409448818896462, 0.1265901696524990294, -1.541994750656167978 ) ) ;
#16289=CARTESIAN_POINT ( 'NONE',  ( -0.2867679344610365999, 0.2867679344610364889, -0.7992125984251968740 ) ) ;
#16290=CARTESIAN_POINT ( 'NONE',  ( -0.2362204724409451284, 0.4091458600556402425, -0.9580052493438320216 ) ) ;
#16294=LINE ( 'NONE', #3237, #73466 ) ;
#16298=CARTESIAN_POINT ( 'NONE',  ( 0.3917322834645668994, 0.1049643490035304522, -0.04722477870634988334 ) ) ;
#16300=CARTESIAN_POINT ( 'NONE',  ( -0.1049643490035307020, 0.3917322834645669549, -0.5636482939632546652 ) ) ;
#16306=CARTESIAN_POINT ( 'NONE',  ( -0.1958661417322836718, 0.3392501089628017219, -2.367454068241469756 ) ) ;
#16309=CARTESIAN_POINT ( 'NONE',  ( -0.3458507752293906723, -0.3458507752293910609, -0.2933070866141732069 ) ) ;
#16320=CARTESIAN_POINT ( 'NONE',  ( -9.787531504996566615E-17, 0.3996062992125985480, -1.651574803149606474 ) ) ;
#16329=CARTESIAN_POINT ( 'NONE',  ( -0.1070741851644051862, -0.3996062992125986035, -0.1489501312335957672 ) ) ;
#16330=CARTESIAN_POINT ( 'NONE',  ( 0.3996062992125986035, 2.446882876249141962E-17, -0.4330708661417322913 ) ) ;
#16331=CARTESIAN_POINT ( 'NONE',  ( -0.1958661417322833942, -0.3392501089628018884, -2.897000943078426705 ) ) ;
#16338=CARTESIAN_POINT ( 'NONE',  ( -0.3949938075777409963, -7.255918531996591613E-17, -0.9035433070866141225 ) ) ;
#16343=CARTESIAN_POINT ( 'NONE',  ( -0.1265901696524986964, -0.4724409448818899238, -1.174540682414698001 ) ) ;
#16344=CARTESIAN_POINT ( 'NONE',  ( -0.3996062992125986035, -7.340648628747425578E-17, -2.244094488188976388 ) ) ;
#16347=CARTESIAN_POINT ( 'NONE',  ( -0.3392501089628019995, 0.1958661417322831999, -0.1804655100075609198 ) ) ;
#16358=CARTESIAN_POINT ( 'NONE',  ( 0.3392501089628018884, -0.1958661417322834220, -0.8845144356955378928 ) ) ;
#16361=CARTESIAN_POINT ( 'NONE',  ( -0.3949938075777409963, -7.255918531996591613E-17, -0.9842519685039369248 ) ) ;
#16370=CARTESIAN_POINT ( 'NONE',  ( 0.1265901696524990572, -0.4724409448818897017, -1.030183727034120533 ) ) ;
#16377=CARTESIAN_POINT ( 'NONE',  ( -0.3996062992125987146, 0.1070741851644051862, -1.607611548556430403 ) ) ;
#16380=CARTESIAN_POINT ( 'NONE',  ( 0.3996062992125985480, 2.446882876249141654E-17, -1.297244094488188670 ) ) ;
#16384=CARTESIAN_POINT ( 'NONE',  ( -1.157146581871515012E-16, 0.4724409448818898682, -0.6299212598425196763 ) ) ;
#16385=CARTESIAN_POINT ( 'NONE',  ( -0.1049643490035307020, 0.3917322834645669549, -2.610892388451443225 ) ) ;
#16391=CARTESIAN_POINT ( 'NONE',  ( 0.1265901696524989462, 0.4724409448818897572, -2.274934383202099397 ) ) ;
#16395=CARTESIAN_POINT ( 'NONE',  ( -0.3949938075777411073, 0.1058382717557497660, -1.841863517060367661 ) ) ;
#16405=CARTESIAN_POINT ( 'NONE',  ( -0.1958661417322836440, 0.3392501089628016664, -2.297880946685352033 ) ) ;
#16419=CARTESIAN_POINT ( 'NONE',  ( 0.1070741851644053388, 0.3996062992125986035, -0.2276902887139107545 ) ) ;
#16421=CARTESIAN_POINT ( 'NONE',  ( 0.3917322834645669549, 0.1049643490035304660, -1.626640419947506411 ) ) ;
#16430=CARTESIAN_POINT ( 'NONE',  ( 0.1070741851644054776, -0.3996062992125984925, -0.7919947506561679784 ) ) ;
#16432=CARTESIAN_POINT ( 'NONE',  ( -0.4091458600556405756, 0.2362204724409446288, -2.622703412073490892 ) ) ;
#16439=CARTESIAN_POINT ( 'NONE',  ( 0.1049643490035303689, 0.3917322834645670104, -1.495406824146981117 ) ) ;
#16444=CARTESIAN_POINT ( 'NONE',  ( 0.3460692066303958092, 0.1998031496062993018, -2.570209973753280863 ) ) ;
#16446=CARTESIAN_POINT ( 'NONE',  ( -0.3996062992125986035, -7.340648628747425578E-17, -0.5118110236220472231 ) ) ;
#16449=CARTESIAN_POINT ( 'NONE',  ( -9.594673741351313045E-17, 0.3917322834645670104, -2.196850393700787496 ) ) ;
#16459=CARTESIAN_POINT ( 'NONE',  ( 0.1958661417322834497, 0.3392501089628018329, -1.484232652722097923 ) ) ;
#16463=CARTESIAN_POINT ( 'NONE',  ( 0.2867679344610365999, -0.2867679344610365444, -2.860236220472440749 ) ) ;
#16465=ORIENTED_EDGE ( 'NONE', *, *, #63766, .T. ) ;
#16466=CARTESIAN_POINT ( 'NONE',  ( -0.1974969037888706647, 0.3420746716998658843, 0.1443569553805773842 ) ) ;
#16474=CARTESIAN_POINT ( 'NONE',  ( 0.3392501089628018329, 0.1958661417322835607, -1.072853961451130544 ) ) ;
#16476=CARTESIAN_POINT ( 'NONE',  ( -0.1958661417322836718, 0.3392501089628017219, -2.145013123359580387 ) ) ;
#16484=CARTESIAN_POINT ( 'NONE',  ( -0.2925321140481932924, 0.2925321140481931814, -1.909448818897637512 ) ) ;
#16490=CARTESIAN_POINT ( 'NONE',  ( 0.3458507752293908943, -0.3458507752293908943, -1.120078740157480324 ) ) ;
#16495=CARTESIAN_POINT ( 'NONE',  ( -0.3949938075777411073, 0.1058382717557497660, -0.4245406824146981672 ) ) ;
#16500=CARTESIAN_POINT ( 'NONE',  ( -0.3949938075777408852, -0.1058382717557502933, -0.4376640419947507299 ) ) ;
#16509=CARTESIAN_POINT ( 'NONE',  ( 0.3996062992125984925, 0.1070741851644054637, -1.303805774278215202 ) ) ;
#16511=CARTESIAN_POINT ( 'NONE',  ( 0.2867679344610365999, 0.2867679344610365999, -0.9173228346456693272 ) ) ;
#16513=CARTESIAN_POINT ( 'NONE',  ( -0.3486222174624316050, 0.1789624963018554005, -1.599317578742253179E-17 ) ) ;
#16521=CARTESIAN_POINT ( 'NONE',  ( -0.1265901696524993347, 0.4724409448818896462, -0.2408136482939632061 ) ) ;
#16526=CARTESIAN_POINT ( 'NONE',  ( -0.3458507752293906723, -0.3458507752293910609, -0.2933070866141732624 ) ) ;
#16536=DIRECTION ( 'NONE',  ( 1.000000000000000000, 8.462065736472231082E-17, 0.000000000000000000 ) ) ;
#16537=CARTESIAN_POINT ( 'NONE',  ( -0.4724409448818898682, 5.785732909357575061E-17, -2.755905511811024056 ) ) ;
#16538=CARTESIAN_POINT ( 'NONE',  ( -0.1998031496062991907, -0.3460692066303959757, -1.010498687664042050 ) ) ;
#16542=CARTESIAN_POINT ( 'NONE',  ( -0.3458507752293909498, 0.3458507752293907833, 0.1377952755905511861 ) ) ;
#16543=CARTESIAN_POINT ( 'NONE',  ( 0.1058382717557500713, -0.3949938075777409408, -2.447506561679789971 ) ) ;
#16544=ORIENTED_EDGE ( 'NONE', *, *, #11244, .F. ) ;
#16546=CARTESIAN_POINT ( 'NONE',  ( 0.3917322834645669549, 0.1049643490035304660, -1.061679790026246462 ) ) ;
#16549=CARTESIAN_POINT ( 'NONE',  ( 0.4091458600556403535, 0.2362204724409449896, -2.493438320209973469 ) ) ;
#16555=CARTESIAN_POINT ( 'NONE',  ( -0.3392501089628019439, 0.1958661417322832554, -0.4212405267378459550 ) ) ;
#16561=CARTESIAN_POINT ( 'NONE',  ( -0.3460692066303958092, -0.1998031496062994683, -2.887139107611548461 ) ) ;
#16562=CARTESIAN_POINT ( 'NONE',  ( 0.1958661417322834775, 0.3392501089628018884, -1.558418265913072309 ) ) ;
#16568=CARTESIAN_POINT ( 'NONE',  ( 0.1049643490035304938, -0.3917322834645669549, -0.7998687664041995715 ) ) ;
#16576=CARTESIAN_POINT ( 'NONE',  ( 5.785732909357575061E-17, -0.4724409448818898682, -0.9429133858267716439 ) ) ;
#16577=CARTESIAN_POINT ( 'NONE',  ( 0.3917322834645670104, 2.398668435337828261E-17, -2.314960629921259727 ) ) ;
#16584=CARTESIAN_POINT ( 'NONE',  ( -0.3917322834645669549, -0.1049643490035306603, -0.6030183727034120755 ) ) ;
#16586=CARTESIAN_POINT ( 'NONE',  ( -0.2925321140481932369, 0.2925321140481931259, -2.616141732283464805 ) ) ;
#16595=CARTESIAN_POINT ( 'NONE',  ( -0.1998031496062991630, -0.3460692066303959202, -2.032152230971128848 ) ) ;
#16597=CARTESIAN_POINT ( 'NONE',  ( 0.3392501089628018884, -0.1958661417322834220, 0.06036745406824151755 ) ) ;
#16605=CARTESIAN_POINT ( 'NONE',  ( 0.3392501089628018329, 0.1958661417322835052, -1.786069923063305032 ) ) ;
#16615=CARTESIAN_POINT ( 'NONE',  ( -0.3917322834645670104, -0.1049643490035307020, -0.5151111792988996019 ) ) ;
#16619=CARTESIAN_POINT ( 'NONE',  ( -0.3458507752293909498, 0.3458507752293907833, -2.143700787401574548 ) ) ;
#16629=CARTESIAN_POINT ( 'NONE',  ( -0.4091458600556405756, 0.2362204724409446288, -2.150262467191601079 ) ) ;
#16641=CARTESIAN_POINT ( 'NONE',  ( 0.3460692066303958092, 0.1998031496062993018, -2.255249343832021136 ) ) ;
#16646=CARTESIAN_POINT ( 'NONE',  ( 0.1070741851644053527, 0.3996062992125986590, -1.883202099737532276 ) ) ;
#16647=CARTESIAN_POINT ( 'NONE',  ( 0.1058382717557500713, -0.3949938075777409408, -1.030183727034120755 ) ) ;
#16648=CARTESIAN_POINT ( 'NONE',  ( -0.1998031496062991907, -0.3460692066303959757, -2.427821522309711266 ) ) ;
#16651=CARTESIAN_POINT ( 'NONE',  ( -0.1601112597053892528, 0.3598931997258726923, -0.002668403679490424611 ) ) ;
#16655=CARTESIAN_POINT ( 'NONE',  ( -0.1974969037888704149, -0.3420746716998661063, -2.189632545931758489 ) ) ;
#16659=CARTESIAN_POINT ( 'NONE',  ( 0.4091458600556404646, -0.2362204724409448231, -2.309711286089239035 ) ) ;
#16660=CARTESIAN_POINT ( 'NONE',  ( -0.3460692066303958092, -0.1998031496062994683, -1.627296587926509330 ) ) ;
#16661=LINE ( 'NONE', #35176, #46591 ) ;
#16668=CARTESIAN_POINT ( 'NONE',  ( 0.3917322834645670104, 2.398668435337828261E-17, 0.1122047244094487306 ) ) ;
#16675=CARTESIAN_POINT ( 'NONE',  ( -0.3917322834645671215, 0.1049643490035301469, -0.2749343832020998413 ) ) ;
#16677=CARTESIAN_POINT ( 'NONE',  ( 0.3917322834645670104, 2.398668435337828261E-17, -2.314960629921259727 ) ) ;
#16680=CARTESIAN_POINT ( 'NONE',  ( -0.1974969037888703871, -0.3420746716998661063, -2.742782152230970993 ) ) ;
#16684=CARTESIAN_POINT ( 'NONE',  ( 0.1070741851644053527, 0.3996062992125986590, -0.9383202099737533164 ) ) ;
#16689=CARTESIAN_POINT ( 'NONE',  ( 0.2867679344610365999, -0.2867679344610365444, -0.02559055118110245899 ) ) ;
#16695=CARTESIAN_POINT ( 'NONE',  ( -0.3917322834645671215, 0.1049643490035301469, -0.1824146981627296216 ) ) ;
#16698=DIRECTION ( 'NONE',  ( 1.000000000000000000, 0.000000000000000000, -0.000000000000000000 ) ) ;
#16699=CARTESIAN_POINT ( 'NONE',  ( 0.1265901696524989462, 0.4724409448818897572, -1.725721784776903078 ) ) ;
#16700=EDGE_CURVE ( 'NONE', #7865, #25718, #68832, .T. ) ;
#16709=CARTESIAN_POINT ( 'NONE',  ( -0.1958661417322836440, 0.3392501089628016664, 0.06432377772409630934 ) ) ;
#16711=CARTESIAN_POINT ( 'NONE',  ( -0.3917322834645671215, 0.1049643490035301469, -0.4324146981627297603 ) ) ;
#16717=CARTESIAN_POINT ( 'NONE',  ( 0.2867679344610365999, 0.2867679344610365999, -2.492125984251968518 ) ) ;
#16720=CARTESIAN_POINT ( 'NONE',  ( -0.1265901696524986964, -0.4724409448818899238, -0.7788713910761155823 ) ) ;
#16732=CARTESIAN_POINT ( 'NONE',  ( -0.3460692066303960313, 0.1998031496062989965, -2.150262467191601079 ) ) ;
#16741=CARTESIAN_POINT ( 'NONE',  ( 0.2925321140481931814, -0.2925321140481931259, -0.3326771653543306728 ) ) ;
#16742=CARTESIAN_POINT ( 'NONE',  ( -0.1998031496062994683, 0.3460692066303958092, -0.4855643044619422644 ) ) ;
#16743=CARTESIAN_POINT ( 'NONE',  ( 0.3392501089628018884, -0.1958661417322833942, -2.778890706857954473 ) ) ;
#16745=CARTESIAN_POINT ( 'NONE',  ( 0.03087045868620516900, -0.3974833285012868700, -5.548669992249399928E-14 ) ) ;
#16750=CARTESIAN_POINT ( 'NONE',  ( -0.2891555358219909388, -0.2891555358219912164, -0.7657480314960630752 ) ) ;
#16755=CARTESIAN_POINT ( 'NONE',  ( -0.2362204724409447953, -0.4091458600556404646, -1.010498687664042050 ) ) ;
#16756=CARTESIAN_POINT ( 'NONE',  ( 0.3996062992125986035, -0.1070741851644053111, -2.316272965879265122 ) ) ;
#16760=CARTESIAN_POINT ( 'NONE',  ( 0.3392501089628018329, 0.1958661417322835607, -0.9153736464905005699 ) ) ;
#16773=CARTESIAN_POINT ( 'NONE',  ( 0.1049643490035304938, -0.3917322834645669549, -1.022309711286088829 ) ) ;
#16776=CARTESIAN_POINT ( 'NONE',  ( 0.1058382717557499880, 0.3949938075777411073, -1.410761154855643351 ) ) ;
#16780=CARTESIAN_POINT ( 'NONE',  ( -0.1998031496062994683, 0.3460692066303958092, 0.1443569553805774119 ) ) ;
#16785=VECTOR ( 'NONE', #55692, 39.37007874015748143 ) ;
#16787=CARTESIAN_POINT ( 'NONE',  ( -0.4724409448818896462, -0.1265901696524993070, -0.9908136482939633449 ) ) ;
#16788=CARTESIAN_POINT ( 'NONE',  ( 0.1265901696524990572, -0.4724409448818897017, -0.6345144356955381149 ) ) ;
#16793=CARTESIAN_POINT ( 'NONE',  ( 0.2925321140481932369, -0.2925321140481932369, -1.515748031496062742 ) ) ;
#16796=CARTESIAN_POINT ( 'NONE',  ( 0.1070741851644053388, 0.3996062992125986035, -1.172572178477690352 ) ) ;
#16800=CARTESIAN_POINT ( 'NONE',  ( 0.4091458600556403535, 0.2362204724409449896, -0.4461942257217847430 ) ) ;
#16803=CARTESIAN_POINT ( 'NONE',  ( -0.1958661417322834220, -0.3392501089628018884, -2.512467191601049699 ) ) ;
#16809=CARTESIAN_POINT ( 'NONE',  ( -0.2362204724409451284, 0.4091458600556402425, -2.294619422572178102 ) ) ;
#16812=CARTESIAN_POINT ( 'NONE',  ( 0.1058382717557499880, 0.3949938075777409408, -1.959973753280839670 ) ) ;
#16822=CARTESIAN_POINT ( 'NONE',  ( -9.594673741351310580E-17, 0.3917322834645669549, -2.599718217026559586 ) ) ;
#16834=CARTESIAN_POINT ( 'NONE',  ( -0.3460692066303957537, -0.1998031496062994405, -0.9166666666666666297 ) ) ;
#16836=CARTESIAN_POINT ( 'NONE',  ( -0.3996062992125984925, -0.1070741851644056858, -0.4376640419947506744 ) ) ;
#16838=CARTESIAN_POINT ( 'NONE',  ( 0.2867679344610365999, 0.2867679344610365999, -1.954724409448818978 ) ) ;
#16848=CARTESIAN_POINT ( 'NONE',  ( 0.2925321140481932369, -0.2925321140481931814, -1.435039370078740495 ) ) ;
#16855=CARTESIAN_POINT ( 'NONE',  ( 4.797336870675656522E-17, -0.3917322834645670104, -1.423228346456693050 ) ) ;
#16860=CARTESIAN_POINT ( 'NONE',  ( -9.787531504996566615E-17, 0.3996062992125985480, -2.438976377952756014 ) ) ;
#16863=CARTESIAN_POINT ( 'NONE',  ( 0.3460692066303959202, 0.1998031496062993295, -0.7611548556430446366 ) ) ;
#16866=CARTESIAN_POINT ( 'NONE',  ( -0.1958661417322836718, 0.3392501089628017219, -2.839895013123359568 ) ) ;
#16876=CARTESIAN_POINT ( 'NONE',  ( -0.3392501089628019439, 0.1958661417322832554, -1.681083046422885197 ) ) ;
#16880=CARTESIAN_POINT ( 'NONE',  ( -0.1958661417322836718, 0.3392501089628017219, -2.774934383202099841 ) ) ;
#16883=CARTESIAN_POINT ( 'NONE',  ( -0.1958661417322836995, 0.3392501089628017219, -2.687027189797587035 ) ) ;
#16891=CARTESIAN_POINT ( 'NONE',  ( -0.3917322834645670104, -0.1049643490035307020, -1.145032439141419500 ) ) ;
#16893=CARTESIAN_POINT ( 'NONE',  ( -0.1049643490035302024, -0.3917322834645671215, -2.361548556430446144 ) ) ;
#16898=CARTESIAN_POINT ( 'NONE',  ( -0.1070741851644056997, 0.3996062992125986035, -0.4790026246719158998 ) ) ;
#16900=CARTESIAN_POINT ( 'NONE',  ( 0.1998031496062994128, -0.3460692066303957537, 0.1463254593175852825 ) ) ;
#16902=CARTESIAN_POINT ( 'NONE',  ( 0.2925321140481932369, -0.2925321140481932369, -2.145669291338581974 ) ) ;
#16908=CARTESIAN_POINT ( 'NONE',  ( -0.2362204724409447953, -0.4091458600556404646, -1.087270341207349000 ) ) ;
#16911=CARTESIAN_POINT ( 'NONE',  ( 0.3420746716998660508, -0.1974969037888704149, -0.4967191601049869010 ) ) ;
#16924=CARTESIAN_POINT ( 'NONE',  ( 0.2925321140481932369, 0.2925321140481932369, -1.946850393700787496 ) ) ;
#16926=CARTESIAN_POINT ( 'NONE',  ( 0.1958661417322834775, 0.3392501089628018884, -1.238845144356955252 ) ) ;
#16940=CARTESIAN_POINT ( 'NONE',  ( 0.4724409448818898127, -0.1265901696524988629, -0.3458005249343831244 ) ) ;
#16947=CARTESIAN_POINT ( 'NONE',  ( -0.1958661417322836995, 0.3392501089628017219, -2.214586244915697222 ) ) ;
#16959=CARTESIAN_POINT ( 'NONE',  ( -0.1265901696524986964, -0.4724409448818899238, -0.07217847769028870597 ) ) ;
#16960=CARTESIAN_POINT ( 'NONE',  ( 4.837279021331060870E-17, -0.3949938075777409963, -2.755905511811023167 ) ) ;
#16963=CARTESIAN_POINT ( 'NONE',  ( 4.797336870675656522E-17, -0.3917322834645670104, -0.8582677165354329896 ) ) ;
#16965=CARTESIAN_POINT ( 'NONE',  ( 5.785732909357575061E-17, -0.4724409448818898682, -2.598425196850393970 ) ) ;
#16971=CARTESIAN_POINT ( 'NONE',  ( -0.2867679344610364334, -0.2867679344610368219, -0.4540489256879772784 ) ) ;
#16978=CARTESIAN_POINT ( 'NONE',  ( -0.3917322834645671770, 0.1049643490035302024, -1.761830339403886336 ) ) ;
#16984=CARTESIAN_POINT ( 'NONE',  ( 0.3392501089628018329, 0.1958661417322835607, -1.160761154855643129 ) ) ;
#16993=CARTESIAN_POINT ( 'NONE',  ( -9.594673741351313045E-17, 0.3917322834645670104, -2.196850393700787496 ) ) ;
#16994=ORIENTED_EDGE ( 'NONE', *, *, #49705, .T. ) ;
#16995=ORIENTED_EDGE ( 'NONE', *, *, #79349, .F. ) ;
#17003=CARTESIAN_POINT ( 'NONE',  ( -0.2867679344610365999, 0.2867679344610364889, -0.8917322834645667884 ) ) ;
#17006=CARTESIAN_POINT ( 'NONE',  ( -0.3460692066303957537, -0.1998031496062994405, -2.333989501312335957 ) ) ;
#17017=CARTESIAN_POINT ( 'NONE',  ( -0.2867679344610364334, -0.2867679344610367109, 0.1062992125984252439 ) ) ;
#17025=CARTESIAN_POINT ( 'NONE',  ( -0.1958661417322836440, 0.3392501089628016664, -1.510479371882202937 ) ) ;
#17034=CARTESIAN_POINT ( 'NONE',  ( 0.3917322834645670104, 0.1049643490035304660, -0.5938513367792144226 ) ) ;
#17037=CARTESIAN_POINT ( 'NONE',  ( -0.3458507752293906723, -0.3458507752293910609, -2.183070866141731958 ) ) ;
#17054=EDGE_CURVE ( 'NONE', #5751, #65743, #75230, .T. ) ;
#17059=CARTESIAN_POINT ( 'NONE',  ( -0.3996062992125986590, 0.1070741851644051723, -2.156824146981627166 ) ) ;
#17066=CARTESIAN_POINT ( 'NONE',  ( -0.1998031496062994683, 0.3460692066303958092, -1.745406824146981561 ) ) ;
#17067=CARTESIAN_POINT ( 'NONE',  ( -0.1974969037888703871, -0.3420746716998661063, -1.010498687664042050 ) ) ;
#17068=CARTESIAN_POINT ( 'NONE',  ( 0.1070741851644054915, -0.3996062992125986035, -2.290026246719159442 ) ) ;
#17070=CARTESIAN_POINT ( 'NONE',  ( 0.1958661417322834775, 0.3392501089628018884, -0.6089238845144356871 ) ) ;
#17074=CARTESIAN_POINT ( 'NONE',  ( -0.2891555358219909388, -0.2891555358219912164, -2.340551181102362488 ) ) ;
#17077=CARTESIAN_POINT ( 'NONE',  ( 0.2362204724409451007, -0.4091458600556402980, -2.454068241469816058 ) ) ;
#17078=CARTESIAN_POINT ( 'NONE',  ( 4.893765752498283924E-17, -0.3996062992125986035, -1.653543307086614123 ) ) ;
#17084=CARTESIAN_POINT ( 'NONE',  ( 0.2867679344610365999, 0.2867679344610365999, -2.737513492617110522 ) ) ;
#17093=CARTESIAN_POINT ( 'NONE',  ( 0.2867679344610365999, -0.2867679344610365444, -0.1830708661417323746 ) ) ;
#17095=CARTESIAN_POINT ( 'NONE',  ( 0.1049643490035304938, -0.3917322834645669549, -2.282152230971128404 ) ) ;
#17098=CARTESIAN_POINT ( 'NONE',  ( -0.2891555358219911054, 0.2891555358219909388, -2.696850393700787496 ) ) ;
#17102=CARTESIAN_POINT ( 'NONE',  ( -0.3996062992125987146, 0.1070741851644051862, -0.8202099737532806412 ) ) ;
#17105=DIRECTION ( 'NONE',  ( 0.000000000000000000, 0.000000000000000000, 1.000000000000000000 ) ) ;
#17107=CARTESIAN_POINT ( 'NONE',  ( -0.1958661417322836718, 0.3392501089628017219, -0.5702099737532808632 ) ) ;
#17108=( BOUNDED_SURFACE ( )  B_SPLINE_SURFACE ( 1, 2, ( 
 ( #49782, #23702, #49373, #36742, #50598, #75069, #17417, #68743, #11085, #4756, #30432, #56097, #75889, #69154, #5177, #50192, #81802, #24113, #69568, #75482, #24526, #82208, #17823, #11505, #37161, #18230, #11916, #37570, #63244, #5584, #82612, #24929, #76306, #18635, #44279, #69969, #61600, #3946, #55266, #23289, #48959, #74660, #70812, #13162, #39654, #59013, #70381, #38395, #45948, #38813, #12736, #32922, #105, #45107, #19038, #58588, #33350, #26611, #52681, #956, #78389, #46371, #32082, #529, #64490, #63656, #77551, #57327, #83021, #25344, #71646, #64075, #7250, #64913, #6828, #77123, #19883, #27020, #13997, #72065, #51006, #76705, #26182, #51421, #52263, #37981, #45532, #19456, #77969, #32497, #6412, #20720, #5995, #20299, #65345, #57743, #44685, #25759, #58161, #31666, #51844, #71230, #13574, #39228, #7682, #1368, #54348, #65762, #61084, #28687, #34598, #73739, #67413, #8095, #2612, #33759, #28269, #66169, #22377, #80473, #21136, #21543, #22785, #34175, #79227, #41323, #47204, #3435, #35007, #46791, #53097, #60672, #40075, #3020, #9747, #59421, #29097, #67004, #1777, #48037, #16074, #41720, #54769, #59839, #9336, #35419, #40491, #15244, #48445, #14424, #15662, #80059, #8509, #27435, #78807, #72482, #14831, #2192, #27860, #73315, #53520, #72894, #40904, #66585, #8921, #60263, #53931, #47619, #79643, #21960, #55170, #23604, #49684, #10982, #74145, #48862, #29509, #10170, #24830, #23191, #50093, #3849, #36240, #56411, #10583, #80879, #69053, #69469, #30748, #24016, #55994, #63147, #62743, #36642, #43764, #18131, #82110, #74562, #24423, #75376, #30328, #81706, #16908, #55578, #42546, #68249, #61910, #16490, #75789, #4655, #81288, #4252, #11822, #17725, #49273, #43351, #37474, #5488, #35835, #61502, #31149, #56815, #82514, #42136, #37059, #29914, #74976, #17321, #11402, #42949, #68643, #62318, #5079, #67831, #38295, #33251, #76611, #82925, #19778, #1272, #57224, #58487, #44183, #6727, #39552, #45432, #426, #13893, #71127, #51322, #70707, #71546, #25660, #45007, #64391, #13470, #58913, #7147, #20196, #32397, #50499, #18941, #38713, #5894, #25246, #77025, #65241, #31566, #50910, #44589, #70283, #12636, #63972, #6308, #64808, #58060, #51742, #39127, #31985, #57645, #32820, #13059, #852, #77445, #8, #19358, #26082, #26509, #52163, #77867, #45847, #7579, #76202, #18540, #69875, #12228, #37885, #63560, #65670, #52996, #79963, #28172, #28590, #20620, #59738, #2092, #54246, #47936, #59323, #27336, #34912, #27757, #1679, #21856, #72386, #34074, #7996, #47520, #22276, #15562, #41628, #73212, #67317, #35321, #21033, #72793, #53421, #52580, #66484, #46272, #71967, #14322, #60575, #78709, #79543, #53829, #79130, #66071, #8819, #15981, #2926, #60984, #39980, #33660, #15143, #40388, #41222, #26920, #34496, #8407, #66909, #21447, #46693, #9652, #78289, #9240, #47104, #14736, #73639, #40799, #60161, #2513, #49592, #43674, #11730, #80780, #49177, #61816, #28998, #42857, #22688, #48347, #74044, #36968, #29413, #55900, #30236, #4156, #42446, #68550, #75699, #62647, #37386, #16391, #42038, #74881, #16809, #81611, #3334, #10891, #68145, #43262, #10490, #61400, #69377, #54664, #23926, #75287, #23096, #67732, #48763, #29821, #80375, #74462, #10067, #55072, #35730, #17630, #3749, #36144, #11309, #55483, #36551, #18040, #68959, #62227, #50002, #4989, #81192, #23509, #24332, #17225, #4565, #30656, #56320, #82018, #19675, #32719, #76925, #63057, #5800, #51227, #18451, #37789, #38198, #52062, #44093, #63466, #31470, #57132, #12132, #69787, #82829, #77344, #44905, #64293, #51639, #25151, #50819, #45334, #25560, #25981, #6627, #76520, #18849, #44495, #71029, #19253, #70603, #70186, #39026, #12539, #31888, #63873, #32299, #6212, #57959, #57548, #83239, #58386, #327, #64710, #56726, #12958, #38615 ),
 ( #13373, #7050, #747, #26408, #77768, #20100, #45751, #71446, #13794, #5395, #31057, #82423, #24742, #50410, #76110, #1583, #2413, #79030, #1992, #65565, #15461, #20933, #8308, #40290, #66384, #46592, #34392, #78189, #7899, #9143, #40699, #41119, #33146, #72288, #14634, #66810, #60473, #71868, #39878, #47419, #65971, #14218, #60060, #27238, #33975, #20520, #28071, #34814, #53729, #54145, #79437, #79859, #47834, #33560, #27655, #59636, #65139, #21349, #58815, #1172, #26823, #73110, #59222, #8721, #21756, #53320, #78610, #47002, #28485, #2824, #73540, #52481, #46172, #72696, #52897, #22176, #39451, #15043, #7475, #56929, #81813, #75080, #57340, #15884, #43882, #69580, #36755, #4359, #62430, #75495, #25359, #4768, #83035, #43058, #49385, #11927, #51022, #23714, #24939, #9551, #56517, #6010, #37582, #50204, #63669, #63255, #17834, #37172, #37993, #43468, #11516, #30853, #5596, #41532, #82625, #69982, #82220, #67218, #68755, #5188, #55690, #17427, #69165, #31680, #11097, #62852, #35221, #81398, #30443, #56108, #24124, #49793, #24539, #75901, #31262, #18241, #50610, #76317, #18647, #44291, #12337, #60885, #30027, #20314, #120, #19472, #38827, #39670, #32938, #39245, #45122, #52697, #58176, #45548, #77566, #45965, #545, #71662, #32097, #70830, #46387, #77985, #78405, #70397, #26198, #51859, #20736, #14439, #25775, #77139, #1383, #19900, #51436, #14013, #64505, #71245, #57758, #65360, #72080, #7698, #8110, #33365, #33776, #1792, #13178, #64928, #13589, #19053, #58603, #12753, #38410, #64092, #27036, #6844, #59028, #40091, #7266, #32514, #972, #65778, #59439, #27452, #6428, #26626, #52280, #76721, #44700, #61520, #9352, #34613, #9763, #60278, #27875, #10186, #53113, #80076, #22394, #72909, #40506, #15261, #28284, #3866, #40921, #35851, #79243, #2207, #48053, #78822, #59855, #61099, #46806, #35023, #42152, #73754, #3037, #16509, #16090, #53946, #73332, #74161, #79659, #47637, #67019, #41735, #21151, #35434, #22803, #60687, #72497, #21558, #41339, #8524, #3450, #14846, #28702, #67847, #67429, #54364, #66188, #29114, #21975, #15678, #34191, #54785, #80488, #48461, #53535, #47220, #66602, #8935, #2628, #29525, #55594, #17741, #68265, #4269, #4671, #18552, #10601, #29931, #81306, #23620, #61927, #36258, #49289, #43780, #11419, #30763, #18146, #74992, #17337, #11835, #75395, #75804, #56425, #42967, #68662, #11000, #69483, #69069, #43369, #36659, #5501, #62334, #81721, #30344, #82125, #56010, #24440, #24030, #49699, #82528, #50108, #31163, #23208, #37074, #62760, #56830, #50512, #5095, #37488, #63163, #24845, #76217, #44197, #69887, #12241, #37897, #63573, #55187, #80895, #48879, #74579, #16924, #42561, #20, #51755, #64404, #31581, #45445, #25259, #50923, #76623, #39566, #31998, #58501, #32833, #6740, #45020, #71141, #78302, #65255, #39993, #18954, #44601, #77458, #19370, #865, #14335, #13483, #70720, #45861, #13073, #63985, #46285, #5908, #26522, #52177, #25674, #70296, #51334, #32411, #57236, #77038, #71981, #57658, #38310, #77880, #82938, #12649, #38727, #6322, #58074, #440, #20211, #71559, #26095, #19794, #39140, #64822, #7162, #13908, #7592, #33264, #58926, #1285, #26934, #52595, #20634, #33674, #34509, #73651, #73225, #28185, #47949, #47534, #21460, #40813, #22288, #47118, #15156, #60172, #15576, #67331, #9253, #54259, #2527, #65683, #66084, #53843, #21047, #14749, #72807, #15993, #46706, #40403, #8420, #34088, #72400, #59751, #2105, #34925, #79556, #21869, #41234, #27770, #53435, #60588, #8832, #66921, #2938, #79143, #66498, #28602, #79975, #41640, #9664, #8010, #59336, #1693, #27351, #53009, #78722, #38986, #52436, #12917, #285, #27195, #58767, #59183, #51185, #7008, #32676, #1540, #78569, #6589, #57921, #65523, #58342, #32260, #78146, #19632, #76883, #20895, #14595 ) ),
 .UNSPECIFIED., .F., .F., .F. ) 
 B_SPLINE_SURFACE_WITH_KNOTS ( ( 2, 2 ),
 ( 3, 2, 2, 2, 2, 2, 2, 2, 2, 2, 2, 2, 2, 2, 2, 2, 2, 2, 2, 2, 2, 2, 2, 2, 2, 2, 2, 2, 2, 2, 2, 2, 2, 2, 2, 2, 2, 2, 2, 2, 2, 2, 2, 2, 2, 2, 2, 2, 2, 2, 2, 2, 2, 2, 2, 2, 2, 2, 2, 2, 2, 2, 2, 2, 2, 2, 2, 2, 2, 2, 2, 2, 2, 2, 2, 2, 2, 2, 2, 2, 2, 2, 2, 2, 2, 2, 2, 2, 2, 2, 2, 2, 2, 2, 2, 2, 2, 2, 2, 2, 2, 2, 2, 2, 2, 2, 2, 2, 2, 2, 2, 2, 2, 2, 2, 2, 2, 2, 2, 2, 2, 2, 2, 2, 2, 2, 2, 2, 2, 2, 2, 2, 2, 2, 2, 2, 2, 2, 2, 2, 2, 2, 2, 2, 2, 2, 2, 2, 2, 2, 2, 2, 2, 2, 2, 2, 2, 2, 2, 2, 2, 2, 2, 2, 2, 2, 2, 2, 2, 2, 2, 2, 2, 2, 2, 2, 2, 2, 2, 2, 2, 2, 2, 2, 2, 2, 2, 2, 2, 2, 2, 2, 2, 2, 2, 2, 2, 2, 2, 2, 2, 2, 2, 2, 2, 2, 2, 2, 2, 2, 2, 2, 2, 2, 2, 2, 2, 2, 2, 2, 2, 2, 2, 2, 2, 2, 2, 2, 2, 2, 2, 2, 2, 2, 2, 2, 2, 3 ),
 ( 0.000000000000000000, 1.000000000000000000 ),
 ( 0.000000000000000000, 0.004166666666666666609, 0.008333333333333333218, 0.01250000000000000069, 0.01666666666666666644, 0.02083333333333333218, 0.02500000000000000139, 0.02916666666666666713, 0.03333333333333333287, 0.03749999999999999861, 0.04166666666666666435, 0.04583333333333333010, 0.05000000000000000278, 0.05416666666666666852, 0.05833333333333333426, 0.06250000000000000000, 0.06666666666666666574, 0.07083333333333333148, 0.07499999999999999722, 0.07916666666666666297, 0.08333333333333332871, 0.08749999999999999445, 0.09166666666666666019, 0.09583333333333333981, 0.1000000000000000056, 0.1041666666666666713, 0.1083333333333333370, 0.1125000000000000028, 0.1166666666666666685, 0.1208333333333333343, 0.1250000000000000000, 0.1291666666666666796, 0.1333333333333333315, 0.1375000000000000111, 0.1416666666666666630, 0.1458333333333333426, 0.1499999999999999944, 0.1541666666666666741, 0.1583333333333333259, 0.1625000000000000056, 0.1666666666666666574, 0.1708333333333333370, 0.1749999999999999889, 0.1791666666666666685, 0.1833333333333333204, 0.1875000000000000000, 0.1916666666666666796, 0.1958333333333333315, 0.2000000000000000111, 0.2041666666666666630, 0.2083333333333333426, 0.2124999999999999944, 0.2166666666666666741, 0.2208333333333333259, 0.2250000000000000056, 0.2291666666666666574, 0.2333333333333333370, 0.2374999999999999889, 0.2416666666666666685, 0.2458333333333333204, 0.2500000000000000000, 0.2541666666666666519, 0.2583333333333333592, 0.2625000000000000111, 0.2666666666666666630, 0.2708333333333333148, 0.2750000000000000222, 0.2791666666666666741, 0.2833333333333333259, 0.2874999999999999778, 0.2916666666666666852, 0.2958333333333333370, 0.2999999999999999889, 0.3041666666666666408, 0.3083333333333333481, 0.3125000000000000000, 0.3166666666666666519, 0.3208333333333333592, 0.3250000000000000111, 0.3291666666666666630, 0.3333333333333333148, 0.3375000000000000222, 0.3416666666666666741, 0.3458333333333333259, 0.3499999999999999778, 0.3541666666666666852, 0.3583333333333333370, 0.3624999999999999889, 0.3666666666666666408, 0.3708333333333333481, 0.3750000000000000000, 0.3791666666666666519, 0.3833333333333333592, 0.3875000000000000111, 0.3916666666666666630, 0.3958333333333333148, 0.4000000000000000222, 0.4041666666666666741, 0.4083333333333333259, 0.4124999999999999778, 0.4166666666666666852, 0.4208333333333333370, 0.4249999999999999889, 0.4291666666666666408, 0.4333333333333333481, 0.4375000000000000000, 0.4416666666666666519, 0.4458333333333333592, 0.4500000000000000111, 0.4541666666666666630, 0.4583333333333333148, 0.4625000000000000222, 0.4666666666666666741, 0.4708333333333333259, 0.4749999999999999778, 0.4791666666666666852, 0.4833333333333333370, 0.4874999999999999889, 0.4916666666666666408, 0.4958333333333333481, 0.5000000000000000000, 0.5041666666666666519, 0.5083333333333333037, 0.5124999999999999556, 0.5166666666666667185, 0.5208333333333333703, 0.5250000000000000222, 0.5291666666666666741, 0.5333333333333333259, 0.5374999999999999778, 0.5416666666666666297, 0.5458333333333332815, 0.5500000000000000444, 0.5541666666666666963, 0.5583333333333333481, 0.5625000000000000000, 0.5666666666666666519, 0.5708333333333333037, 0.5749999999999999556, 0.5791666666666667185, 0.5833333333333333703, 0.5875000000000000222, 0.5916666666666666741, 0.5958333333333333259, 0.5999999999999999778, 0.6041666666666666297, 0.6083333333333332815, 0.6125000000000000444, 0.6166666666666666963, 0.6208333333333333481, 0.6250000000000000000, 0.6291666666666666519, 0.6333333333333333037, 0.6374999999999999556, 0.6416666666666667185, 0.6458333333333333703, 0.6500000000000000222, 0.6541666666666666741, 0.6583333333333333259, 0.6624999999999999778, 0.6666666666666666297, 0.6708333333333332815, 0.6750000000000000444, 0.6791666666666666963, 0.6833333333333333481, 0.6875000000000000000, 0.6916666666666666519, 0.6958333333333333037, 0.6999999999999999556, 0.7041666666666667185, 0.7083333333333333703, 0.7125000000000000222, 0.7166666666666666741, 0.7208333333333333259, 0.7249999999999999778, 0.7291666666666666297, 0.7333333333333332815, 0.7375000000000000444, 0.7416666666666666963, 0.7458333333333333481, 0.7500000000000000000, 0.7541666666666666519, 0.7583333333333333037, 0.7624999999999999556, 0.7666666666666667185, 0.7708333333333333703, 0.7750000000000000222, 0.7791666666666666741, 0.7833333333333333259, 0.7874999999999999778, 0.7916666666666666297, 0.7958333333333332815, 0.8000000000000000444, 0.8041666666666666963, 0.8083333333333333481, 0.8125000000000000000, 0.8166666666666666519, 0.8208333333333333037, 0.8249999999999999556, 0.8291666666666667185, 0.8333333333333333703, 0.8375000000000000222, 0.8416666666666666741, 0.8458333333333333259, 0.8499999999999999778, 0.8541666666666666297, 0.8583333333333332815, 0.8625000000000000444, 0.8666666666666666963, 0.8708333333333333481, 0.8750000000000000000, 0.8791666666666666519, 0.8833333333333333037, 0.8874999999999999556, 0.8916666666666667185, 0.8958333333333333703, 0.9000000000000000222, 0.9041666666666666741, 0.9083333333333333259, 0.9124999999999999778, 0.9166666666666666297, 0.9208333333333332815, 0.9250000000000000444, 0.9291666666666666963, 0.9333333333333333481, 0.9375000000000000000, 0.9416666666666666519, 0.9458333333333333037, 0.9499999999999999556, 0.9541666666666667185, 0.9583333333333333703, 0.9625000000000000222, 0.9666666666666666741, 0.9708333333333333259, 0.9749999999999999778, 0.9791666666666666297, 0.9833333333333332815, 0.9875000000000000444 ),
 .UNSPECIFIED. ) 
 GEOMETRIC_REPRESENTATION_ITEM ( )  RATIONAL_B_SPLINE_SURFACE ( (
 ( 1.000000000000000000, 0.9659258262890683122, 1.000000000000000000, 0.9659258262890683122, 1.000000000000000000, 0.9659258262890683122, 1.000000000000000000, 0.9659258262890683122, 1.000000000000000000, 0.9659258262890683122, 1.000000000000000000, 0.9659258262890683122, 1.000000000000000000, 0.9659258262890683122, 1.000000000000000000, 0.9659258262890683122, 1.000000000000000000, 0.9659258262890683122, 1.000000000000000000, 0.9659258262890683122, 1.000000000000000000, 0.9659258262890683122, 1.000000000000000000, 0.9659258262890683122, 1.000000000000000000, 0.9659258262890683122, 1.000000000000000000, 0.9659258262890683122, 1.000000000000000000, 0.9659258262890683122, 1.000000000000000000, 0.9659258262890683122, 1.000000000000000000, 0.9659258262890683122, 1.000000000000000000, 0.9659258262890683122, 1.000000000000000000, 0.9659258262890683122, 1.000000000000000000, 0.9659258262890683122, 1.000000000000000000, 0.9659258262890683122, 1.000000000000000000, 0.9659258262890683122, 1.000000000000000000, 0.9659258262890683122, 1.000000000000000000, 0.9659258262890683122, 1.000000000000000000, 0.9659258262890683122, 1.000000000000000000, 0.9659258262890683122, 1.000000000000000000, 0.9659258262890683122, 1.000000000000000000, 0.9659258262890683122, 1.000000000000000000, 0.9659258262890683122, 1.000000000000000000, 0.9659258262890683122, 1.000000000000000000, 0.9659258262890683122, 1.000000000000000000, 0.9659258262890683122, 1.000000000000000000, 0.9659258262890683122, 1.000000000000000000, 0.9659258262890683122, 1.000000000000000000, 0.9659258262890683122, 1.000000000000000000, 0.9659258262890683122, 1.000000000000000000, 0.9659258262890683122, 1.000000000000000000, 0.9659258262890683122, 1.000000000000000000, 0.9659258262890683122, 1.000000000000000000, 0.9659258262890683122, 1.000000000000000000, 0.9659258262890683122, 1.000000000000000000, 0.9659258262890683122, 1.000000000000000000, 0.9659258262890683122, 1.000000000000000000, 0.9659258262890683122, 1.000000000000000000, 0.9659258262890683122, 1.000000000000000000, 0.9659258262890683122, 1.000000000000000000, 0.9659258262890683122, 1.000000000000000000, 0.9659258262890683122, 1.000000000000000000, 0.9659258262890683122, 1.000000000000000000, 0.9659258262890683122, 1.000000000000000000, 0.9659258262890683122, 1.000000000000000000, 0.9659258262890683122, 1.000000000000000000, 0.9659258262890683122, 1.000000000000000000, 0.9659258262890683122, 1.000000000000000000, 0.9659258262890683122, 1.000000000000000000, 0.9659258262890683122, 1.000000000000000000, 0.9659258262890683122, 1.000000000000000000, 0.9659258262890683122, 1.000000000000000000, 0.9659258262890683122, 1.000000000000000000, 0.9659258262890683122, 1.000000000000000000, 0.9659258262890683122, 1.000000000000000000, 0.9659258262890683122, 1.000000000000000000, 0.9659258262890683122, 1.000000000000000000, 0.9659258262890683122, 1.000000000000000000, 0.9659258262890683122, 1.000000000000000000, 0.9659258262890683122, 1.000000000000000000, 0.9659258262890683122, 1.000000000000000000, 0.9659258262890683122, 1.000000000000000000, 0.9659258262890683122, 1.000000000000000000, 0.9659258262890683122, 1.000000000000000000, 0.9659258262890683122, 1.000000000000000000, 0.9659258262890683122, 1.000000000000000000, 0.9659258262890683122, 1.000000000000000000, 0.9659258262890683122, 1.000000000000000000, 0.9659258262890683122, 1.000000000000000000, 0.9659258262890683122, 1.000000000000000000, 0.9659258262890683122, 1.000000000000000000, 0.9659258262890683122, 1.000000000000000000, 0.9659258262890683122, 1.000000000000000000, 0.9659258262890683122, 1.000000000000000000, 0.9659258262890683122, 1.000000000000000000, 0.9659258262890683122, 1.000000000000000000, 0.9659258262890683122, 1.000000000000000000, 0.9659258262890683122, 1.000000000000000000, 0.9659258262890683122, 1.000000000000000000, 0.9659258262890683122, 1.000000000000000000, 0.9659258262890683122, 1.000000000000000000, 0.9659258262890683122, 1.000000000000000000, 0.9659258262890683122, 1.000000000000000000, 0.9659258262890683122, 1.000000000000000000, 0.9659258262890683122, 1.000000000000000000, 0.9659258262890683122, 1.000000000000000000, 0.9659258262890683122, 1.000000000000000000, 0.9659258262890683122, 1.000000000000000000, 0.9659258262890683122, 1.000000000000000000, 0.9659258262890683122, 1.000000000000000000, 0.9659258262890683122, 1.000000000000000000, 0.9659258262890683122, 1.000000000000000000, 0.9659258262890683122, 1.000000000000000000, 0.9659258262890683122, 1.000000000000000000, 0.9659258262890683122, 1.000000000000000000, 0.9659258262890683122, 1.000000000000000000, 0.9659258262890683122, 1.000000000000000000, 0.9659258262890683122, 1.000000000000000000, 0.9659258262890683122, 1.000000000000000000, 0.9659258262890683122, 1.000000000000000000, 0.9659258262890683122, 1.000000000000000000, 0.9659258262890683122, 1.000000000000000000, 0.9659258262890683122, 1.000000000000000000, 0.9659258262890683122, 1.000000000000000000, 0.9659258262890683122, 1.000000000000000000, 0.9659258262890683122, 1.000000000000000000, 0.9659258262890683122, 1.000000000000000000, 0.9659258262890683122, 1.000000000000000000, 0.9659258262890683122, 1.000000000000000000, 0.9659258262890683122, 1.000000000000000000, 0.9659258262890683122, 1.000000000000000000, 0.9659258262890683122, 1.000000000000000000, 0.9659258262890683122, 1.000000000000000000, 0.9659258262890683122, 1.000000000000000000, 0.9659258262890683122, 1.000000000000000000, 0.9659258262890683122, 1.000000000000000000, 0.9659258262890683122, 1.000000000000000000, 0.9659258262890683122, 1.000000000000000000, 0.9659258262890683122, 1.000000000000000000, 0.9659258262890683122, 1.000000000000000000, 0.9659258262890683122, 1.000000000000000000, 0.9659258262890683122, 1.000000000000000000, 0.9659258262890683122, 1.000000000000000000, 0.9659258262890683122, 1.000000000000000000, 0.9659258262890683122, 1.000000000000000000, 0.9659258262890683122, 1.000000000000000000, 0.9659258262890683122, 1.000000000000000000, 0.9659258262890683122, 1.000000000000000000, 0.9659258262890683122, 1.000000000000000000, 0.9659258262890683122, 1.000000000000000000, 0.9659258262890683122, 1.000000000000000000, 0.9659258262890683122, 1.000000000000000000, 0.9659258262890683122, 1.000000000000000000, 0.9659258262890683122, 1.000000000000000000, 0.9659258262890683122, 1.000000000000000000, 0.9659258262890683122, 1.000000000000000000, 0.9659258262890683122, 1.000000000000000000, 0.9659258262890683122, 1.000000000000000000, 0.9659258262890683122, 1.000000000000000000, 0.9659258262890683122, 1.000000000000000000, 0.9659258262890683122, 1.000000000000000000, 0.9659258262890683122, 1.000000000000000000, 0.9659258262890683122, 1.000000000000000000, 0.9659258262890683122, 1.000000000000000000, 0.9659258262890683122, 1.000000000000000000, 0.9659258262890683122, 1.000000000000000000, 0.9659258262890683122, 1.000000000000000000, 0.9659258262890683122, 1.000000000000000000, 0.9659258262890683122, 1.000000000000000000, 0.9659258262890683122, 1.000000000000000000, 0.9659258262890683122, 1.000000000000000000, 0.9659258262890683122, 1.000000000000000000, 0.9659258262890683122, 1.000000000000000000, 0.9659258262890683122, 1.000000000000000000, 0.9659258262890683122, 1.000000000000000000, 0.9659258262890683122, 1.000000000000000000, 0.9659258262890683122, 1.000000000000000000, 0.9659258262890683122, 1.000000000000000000, 0.9659258262890683122, 1.000000000000000000, 0.9659258262890683122, 1.000000000000000000, 0.9659258262890683122, 1.000000000000000000, 0.9659258262890683122, 1.000000000000000000, 0.9659258262890683122, 1.000000000000000000, 0.9659258262890683122, 1.000000000000000000, 0.9659258262890683122, 1.000000000000000000, 0.9659258262890683122, 1.000000000000000000, 0.9659258262890683122, 1.000000000000000000, 0.9659258262890683122, 1.000000000000000000, 0.9659258262890683122, 1.000000000000000000, 0.9659258262890683122, 1.000000000000000000, 0.9659258262890683122, 1.000000000000000000, 0.9659258262890683122, 1.000000000000000000, 0.9659258262890683122, 1.000000000000000000, 0.9659258262890683122, 1.000000000000000000, 0.9659258262890683122, 1.000000000000000000, 0.9659258262890683122, 1.000000000000000000, 0.9659258262890683122, 1.000000000000000000, 0.9659258262890683122, 1.000000000000000000, 0.9659258262890683122, 1.000000000000000000, 0.9659258262890683122, 1.000000000000000000, 0.9659258262890683122, 1.000000000000000000, 0.9659258262890683122, 1.000000000000000000, 0.9659258262890683122, 1.000000000000000000, 0.9659258262890683122, 1.000000000000000000, 0.9659258262890683122, 1.000000000000000000, 0.9659258262890683122, 1.000000000000000000, 0.9659258262890683122, 1.000000000000000000, 0.9659258262890683122, 1.000000000000000000, 0.9659258262890683122, 1.000000000000000000, 0.9659258262890683122, 1.000000000000000000, 0.9659258262890683122, 1.000000000000000000, 0.9659258262890683122, 1.000000000000000000, 0.9659258262890683122, 1.000000000000000000, 0.9659258262890683122, 1.000000000000000000, 0.9659258262890683122, 1.000000000000000000, 0.9659258262890683122, 1.000000000000000000, 0.9659258262890683122, 1.000000000000000000, 0.9659258262890683122, 1.000000000000000000, 0.9659258262890683122, 1.000000000000000000, 0.9659258262890683122, 1.000000000000000000, 0.9659258262890683122, 1.000000000000000000, 0.9659258262890683122, 1.000000000000000000, 0.9659258262890683122, 1.000000000000000000, 0.9659258262890683122, 1.000000000000000000, 0.9659258262890683122, 1.000000000000000000, 0.9659258262890683122, 1.000000000000000000, 0.9659258262890683122, 1.000000000000000000, 0.9659258262890683122, 1.000000000000000000, 0.9659258262890683122, 1.000000000000000000, 0.9659258262890683122, 1.000000000000000000, 0.9659258262890683122, 1.000000000000000000, 0.9659258262890683122, 1.000000000000000000, 0.9659258262890683122, 1.000000000000000000, 0.9659258262890683122, 1.000000000000000000, 0.9659258262890683122, 1.000000000000000000, 0.9659258262890683122, 1.000000000000000000, 0.9659258262890683122, 1.000000000000000000, 0.9659258262890683122, 1.000000000000000000, 0.9659258262890683122, 1.000000000000000000, 0.9659258262890683122, 1.000000000000000000, 0.9659258262890683122, 1.000000000000000000, 0.9659258262890683122, 1.000000000000000000, 0.9659258262890683122, 1.000000000000000000, 0.9659258262890683122, 1.000000000000000000, 0.9659258262890683122, 1.000000000000000000, 0.9659258262890683122, 1.000000000000000000, 0.9659258262890683122, 1.000000000000000000, 0.9659258262890683122, 1.000000000000000000, 0.9659258262890683122, 1.000000000000000000, 0.9659258262890683122, 1.000000000000000000, 0.9659258262890683122, 1.000000000000000000),
 ( 1.000000000000000000, 0.9659258262890683122, 1.000000000000000000, 0.9659258262890683122, 1.000000000000000000, 0.9659258262890683122, 1.000000000000000000, 0.9659258262890683122, 1.000000000000000000, 0.9659258262890683122, 1.000000000000000000, 0.9659258262890683122, 1.000000000000000000, 0.9659258262890683122, 1.000000000000000000, 0.9659258262890683122, 1.000000000000000000, 0.9659258262890683122, 1.000000000000000000, 0.9659258262890683122, 1.000000000000000000, 0.9659258262890683122, 1.000000000000000000, 0.9659258262890683122, 1.000000000000000000, 0.9659258262890683122, 1.000000000000000000, 0.9659258262890683122, 1.000000000000000000, 0.9659258262890683122, 1.000000000000000000, 0.9659258262890683122, 1.000000000000000000, 0.9659258262890683122, 1.000000000000000000, 0.9659258262890683122, 1.000000000000000000, 0.9659258262890683122, 1.000000000000000000, 0.9659258262890683122, 1.000000000000000000, 0.9659258262890683122, 1.000000000000000000, 0.9659258262890683122, 1.000000000000000000, 0.9659258262890683122, 1.000000000000000000, 0.9659258262890683122, 1.000000000000000000, 0.9659258262890683122, 1.000000000000000000, 0.9659258262890683122, 1.000000000000000000, 0.9659258262890683122, 1.000000000000000000, 0.9659258262890683122, 1.000000000000000000, 0.9659258262890683122, 1.000000000000000000, 0.9659258262890683122, 1.000000000000000000, 0.9659258262890683122, 1.000000000000000000, 0.9659258262890683122, 1.000000000000000000, 0.9659258262890683122, 1.000000000000000000, 0.9659258262890683122, 1.000000000000000000, 0.9659258262890683122, 1.000000000000000000, 0.9659258262890683122, 1.000000000000000000, 0.9659258262890683122, 1.000000000000000000, 0.9659258262890683122, 1.000000000000000000, 0.9659258262890683122, 1.000000000000000000, 0.9659258262890683122, 1.000000000000000000, 0.9659258262890683122, 1.000000000000000000, 0.9659258262890683122, 1.000000000000000000, 0.9659258262890683122, 1.000000000000000000, 0.9659258262890683122, 1.000000000000000000, 0.9659258262890683122, 1.000000000000000000, 0.9659258262890683122, 1.000000000000000000, 0.9659258262890683122, 1.000000000000000000, 0.9659258262890683122, 1.000000000000000000, 0.9659258262890683122, 1.000000000000000000, 0.9659258262890683122, 1.000000000000000000, 0.9659258262890683122, 1.000000000000000000, 0.9659258262890683122, 1.000000000000000000, 0.9659258262890683122, 1.000000000000000000, 0.9659258262890683122, 1.000000000000000000, 0.9659258262890683122, 1.000000000000000000, 0.9659258262890683122, 1.000000000000000000, 0.9659258262890683122, 1.000000000000000000, 0.9659258262890683122, 1.000000000000000000, 0.9659258262890683122, 1.000000000000000000, 0.9659258262890683122, 1.000000000000000000, 0.9659258262890683122, 1.000000000000000000, 0.9659258262890683122, 1.000000000000000000, 0.9659258262890683122, 1.000000000000000000, 0.9659258262890683122, 1.000000000000000000, 0.9659258262890683122, 1.000000000000000000, 0.9659258262890683122, 1.000000000000000000, 0.9659258262890683122, 1.000000000000000000, 0.9659258262890683122, 1.000000000000000000, 0.9659258262890683122, 1.000000000000000000, 0.9659258262890683122, 1.000000000000000000, 0.9659258262890683122, 1.000000000000000000, 0.9659258262890683122, 1.000000000000000000, 0.9659258262890683122, 1.000000000000000000, 0.9659258262890683122, 1.000000000000000000, 0.9659258262890683122, 1.000000000000000000, 0.9659258262890683122, 1.000000000000000000, 0.9659258262890683122, 1.000000000000000000, 0.9659258262890683122, 1.000000000000000000, 0.9659258262890683122, 1.000000000000000000, 0.9659258262890683122, 1.000000000000000000, 0.9659258262890683122, 1.000000000000000000, 0.9659258262890683122, 1.000000000000000000, 0.9659258262890683122, 1.000000000000000000, 0.9659258262890683122, 1.000000000000000000, 0.9659258262890683122, 1.000000000000000000, 0.9659258262890683122, 1.000000000000000000, 0.9659258262890683122, 1.000000000000000000, 0.9659258262890683122, 1.000000000000000000, 0.9659258262890683122, 1.000000000000000000, 0.9659258262890683122, 1.000000000000000000, 0.9659258262890683122, 1.000000000000000000, 0.9659258262890683122, 1.000000000000000000, 0.9659258262890683122, 1.000000000000000000, 0.9659258262890683122, 1.000000000000000000, 0.9659258262890683122, 1.000000000000000000, 0.9659258262890683122, 1.000000000000000000, 0.9659258262890683122, 1.000000000000000000, 0.9659258262890683122, 1.000000000000000000, 0.9659258262890683122, 1.000000000000000000, 0.9659258262890683122, 1.000000000000000000, 0.9659258262890683122, 1.000000000000000000, 0.9659258262890683122, 1.000000000000000000, 0.9659258262890683122, 1.000000000000000000, 0.9659258262890683122, 1.000000000000000000, 0.9659258262890683122, 1.000000000000000000, 0.9659258262890683122, 1.000000000000000000, 0.9659258262890683122, 1.000000000000000000, 0.9659258262890683122, 1.000000000000000000, 0.9659258262890683122, 1.000000000000000000, 0.9659258262890683122, 1.000000000000000000, 0.9659258262890683122, 1.000000000000000000, 0.9659258262890683122, 1.000000000000000000, 0.9659258262890683122, 1.000000000000000000, 0.9659258262890683122, 1.000000000000000000, 0.9659258262890683122, 1.000000000000000000, 0.9659258262890683122, 1.000000000000000000, 0.9659258262890683122, 1.000000000000000000, 0.9659258262890683122, 1.000000000000000000, 0.9659258262890683122, 1.000000000000000000, 0.9659258262890683122, 1.000000000000000000, 0.9659258262890683122, 1.000000000000000000, 0.9659258262890683122, 1.000000000000000000, 0.9659258262890683122, 1.000000000000000000, 0.9659258262890683122, 1.000000000000000000, 0.9659258262890683122, 1.000000000000000000, 0.9659258262890683122, 1.000000000000000000, 0.9659258262890683122, 1.000000000000000000, 0.9659258262890683122, 1.000000000000000000, 0.9659258262890683122, 1.000000000000000000, 0.9659258262890683122, 1.000000000000000000, 0.9659258262890683122, 1.000000000000000000, 0.9659258262890683122, 1.000000000000000000, 0.9659258262890683122, 1.000000000000000000, 0.9659258262890683122, 1.000000000000000000, 0.9659258262890683122, 1.000000000000000000, 0.9659258262890683122, 1.000000000000000000, 0.9659258262890683122, 1.000000000000000000, 0.9659258262890683122, 1.000000000000000000, 0.9659258262890683122, 1.000000000000000000, 0.9659258262890683122, 1.000000000000000000, 0.9659258262890683122, 1.000000000000000000, 0.9659258262890683122, 1.000000000000000000, 0.9659258262890683122, 1.000000000000000000, 0.9659258262890683122, 1.000000000000000000, 0.9659258262890683122, 1.000000000000000000, 0.9659258262890683122, 1.000000000000000000, 0.9659258262890683122, 1.000000000000000000, 0.9659258262890683122, 1.000000000000000000, 0.9659258262890683122, 1.000000000000000000, 0.9659258262890683122, 1.000000000000000000, 0.9659258262890683122, 1.000000000000000000, 0.9659258262890683122, 1.000000000000000000, 0.9659258262890683122, 1.000000000000000000, 0.9659258262890683122, 1.000000000000000000, 0.9659258262890683122, 1.000000000000000000, 0.9659258262890683122, 1.000000000000000000, 0.9659258262890683122, 1.000000000000000000, 0.9659258262890683122, 1.000000000000000000, 0.9659258262890683122, 1.000000000000000000, 0.9659258262890683122, 1.000000000000000000, 0.9659258262890683122, 1.000000000000000000, 0.9659258262890683122, 1.000000000000000000, 0.9659258262890683122, 1.000000000000000000, 0.9659258262890683122, 1.000000000000000000, 0.9659258262890683122, 1.000000000000000000, 0.9659258262890683122, 1.000000000000000000, 0.9659258262890683122, 1.000000000000000000, 0.9659258262890683122, 1.000000000000000000, 0.9659258262890683122, 1.000000000000000000, 0.9659258262890683122, 1.000000000000000000, 0.9659258262890683122, 1.000000000000000000, 0.9659258262890683122, 1.000000000000000000, 0.9659258262890683122, 1.000000000000000000, 0.9659258262890683122, 1.000000000000000000, 0.9659258262890683122, 1.000000000000000000, 0.9659258262890683122, 1.000000000000000000, 0.9659258262890683122, 1.000000000000000000, 0.9659258262890683122, 1.000000000000000000, 0.9659258262890683122, 1.000000000000000000, 0.9659258262890683122, 1.000000000000000000, 0.9659258262890683122, 1.000000000000000000, 0.9659258262890683122, 1.000000000000000000, 0.9659258262890683122, 1.000000000000000000, 0.9659258262890683122, 1.000000000000000000, 0.9659258262890683122, 1.000000000000000000, 0.9659258262890683122, 1.000000000000000000, 0.9659258262890683122, 1.000000000000000000, 0.9659258262890683122, 1.000000000000000000, 0.9659258262890683122, 1.000000000000000000, 0.9659258262890683122, 1.000000000000000000, 0.9659258262890683122, 1.000000000000000000, 0.9659258262890683122, 1.000000000000000000, 0.9659258262890683122, 1.000000000000000000, 0.9659258262890683122, 1.000000000000000000, 0.9659258262890683122, 1.000000000000000000, 0.9659258262890683122, 1.000000000000000000, 0.9659258262890683122, 1.000000000000000000, 0.9659258262890683122, 1.000000000000000000, 0.9659258262890683122, 1.000000000000000000, 0.9659258262890683122, 1.000000000000000000, 0.9659258262890683122, 1.000000000000000000, 0.9659258262890683122, 1.000000000000000000, 0.9659258262890683122, 1.000000000000000000, 0.9659258262890683122, 1.000000000000000000, 0.9659258262890683122, 1.000000000000000000, 0.9659258262890683122, 1.000000000000000000, 0.9659258262890683122, 1.000000000000000000, 0.9659258262890683122, 1.000000000000000000, 0.9659258262890683122, 1.000000000000000000, 0.9659258262890683122, 1.000000000000000000, 0.9659258262890683122, 1.000000000000000000, 0.9659258262890683122, 1.000000000000000000, 0.9659258262890683122, 1.000000000000000000, 0.9659258262890683122, 1.000000000000000000, 0.9659258262890683122, 1.000000000000000000, 0.9659258262890683122, 1.000000000000000000, 0.9659258262890683122, 1.000000000000000000, 0.9659258262890683122, 1.000000000000000000, 0.9659258262890683122, 1.000000000000000000, 0.9659258262890683122, 1.000000000000000000, 0.9659258262890683122, 1.000000000000000000, 0.9659258262890683122, 1.000000000000000000, 0.9659258262890683122, 1.000000000000000000, 0.9659258262890683122, 1.000000000000000000, 0.9659258262890683122, 1.000000000000000000, 0.9659258262890683122, 1.000000000000000000, 0.9659258262890683122, 1.000000000000000000, 0.9659258262890683122, 1.000000000000000000, 0.9659258262890683122, 1.000000000000000000, 0.9659258262890683122, 1.000000000000000000, 0.9659258262890683122, 1.000000000000000000, 0.9659258262890683122, 1.000000000000000000, 0.9659258262890683122, 1.000000000000000000, 0.9659258262890683122, 1.000000000000000000, 0.9659258262890683122, 1.000000000000000000, 0.9659258262890683122, 1.000000000000000000, 0.9659258262890683122, 1.000000000000000000) ) ) 
 REPRESENTATION_ITEM ( '' )  SURFACE ( )  );
#17114=CARTESIAN_POINT ( 'NONE',  ( 0.2867679344610365999, 0.2867679344610365999, -0.2874015748031494843 ) ) ;
#17118=CARTESIAN_POINT ( 'NONE',  ( -0.3458507752293906723, -0.3458507752293910609, -1.791338582677165059 ) ) ;
#17131=CARTESIAN_POINT ( 'NONE',  ( 0.3917322834645669549, 2.398668435337827645E-17, -0.1981434138769535558 ) ) ;
#17133=CARTESIAN_POINT ( 'NONE',  ( -0.1958661417322836718, 0.3392501089628017219, -0.2552493438320210806 ) ) ;
#17138=CARTESIAN_POINT ( 'NONE',  ( -0.2867679344610365999, 0.2867679344610364889, -2.531496062992125484 ) ) ;
#17141=CARTESIAN_POINT ( 'NONE',  ( -0.3458507752293906723, -0.3458507752293910609, -0.6082677165354329896 ) ) ;
#17152=CARTESIAN_POINT ( 'NONE',  ( 0.1998031496062992463, 0.3460692066303959202, -1.953412073490813805 ) ) ;
#17160=CARTESIAN_POINT ( 'NONE',  ( 0.3460692066303959202, -0.1998031496062991630, -0.1817585301837270351 ) ) ;
#17161=CARTESIAN_POINT ( 'NONE',  ( -0.3460692066303960868, 0.1998031496062990242, -0.6561679790026246906 ) ) ;
#17162=CARTESIAN_POINT ( 'NONE',  ( -0.3420746716998661618, 0.1974969037888702206, 0.1312335958005248771 ) ) ;
#17167=CARTESIAN_POINT ( 'NONE',  ( -0.3420746716998662729, 0.1974969037888702206, -0.8904199475065616154 ) ) ;
#17172=CARTESIAN_POINT ( 'NONE',  ( -0.4724409448818895907, -0.1265901696524993070, -1.305774278215223072 ) ) ;
#17174=CARTESIAN_POINT ( 'NONE',  ( -0.1070741851644051862, -0.3996062992125986590, -2.434383202099737353 ) ) ;
#17177=CARTESIAN_POINT ( 'NONE',  ( 4.797336870675656522E-17, -0.3917322834645670659, -0.8628802081702905413 ) ) ;
#17189=CARTESIAN_POINT ( 'NONE',  ( -0.3917322834645671215, 0.1049643490035301469, -0.9698162729658791337 ) ) ;
#17191=ORIENTED_EDGE ( 'NONE', *, *, #48857, .F. ) ;
#17192=CARTESIAN_POINT ( 'NONE',  ( 0.1058382717557499880, 0.3949938075777411073, -1.568241469816272993 ) ) ;
#17196=CARTESIAN_POINT ( 'NONE',  ( -0.1070741851644056997, 0.3996062992125986035, 0.1509186351706036100 ) ) ;
#17203=CARTESIAN_POINT ( 'NONE',  ( 0.2867679344610365999, 0.2867679344610365999, 0.09251968503937001154 ) ) ;
#17209=CARTESIAN_POINT ( 'NONE',  ( 0.3996062992125986035, 2.446882876249141962E-17, -2.007874015748031482 ) ) ;
#17212=CARTESIAN_POINT ( 'NONE',  ( 0.3996062992125985480, 2.446882876249141654E-17, -1.454724409448818756 ) ) ;
#17216=CARTESIAN_POINT ( 'NONE',  ( 0.4724409448818897572, -0.1265901696524988906, -0.2690288713910760632 ) ) ;
#17218=ADVANCED_FACE ( 'NONE', ( #55914 ), #81627, .T. ) ;
#17219=CARTESIAN_POINT ( 'NONE',  ( 4.797336870675656522E-17, -0.3917322834645670104, -2.368110236220472675 ) ) ;
#17225=CARTESIAN_POINT ( 'NONE',  ( 0.1265901696524990294, -0.4724409448818896462, -2.524278215223096478 ) ) ;
#17226=EDGE_CURVE ( 'NONE', #18415, #17964, #30672, .T. ) ;
#17228=CARTESIAN_POINT ( 'NONE',  ( 0.1974969037888704704, 0.3420746716998660508, -2.425853018372703396 ) ) ;
#17238=( BOUNDED_CURVE ( )  B_SPLINE_CURVE ( 2, ( #323, #71025, #71442, #32715, #57128, #70182, #19669, #7046, #13790, #50406, #58382, #24738, #76516, #63462, #51223, #57544, #25556, #52058, #39447, #64289, #32295, #76921, #33140, #65135, #25147, #76104, #51635, #45330, #50815, #44089, #31466, #12535, #69783, #12128, #5796, #82823, #38194, #19249, #18845, #63869, #13369, #6207, #39022, #64706, #31884, #70599, #9140, #21753, #78607, #71864, #7895, #67215, #65561, #15040, #34389, #52894, #60055, #22173, #79027, #41529, #46587, #73536, #54142, #14214, #20930, #47416, #34811, #40696, #53726, #27235, #2410, #73107, #72285, #39872, #33556, #9548, #59219, #66381, #28068, #14631, #79434, #15458, #1580, #40287, #65968, #15881, #79856, #8305, #33972, #41116, #60470, #8718, #66806, #59633, #2821, #1989, #46168, #78185, #28482, #47831, #27652, #53315, #20516, #21346, #35218, #46999, #72693, #1168, #26819, #52477, #10790, #29721, #41934, #55383, #76717, #48661, #30131, #68451, #43160, #35632, #81089, #60882, #12749, #22588, #36450, #81501, #36864, #67630, #54975 ),
 .UNSPECIFIED., .F., .F. ) 
 B_SPLINE_CURVE_WITH_KNOTS ( ( 3, 2, 2, 2, 2, 2, 2, 2, 2, 2, 2, 2, 2, 2, 2, 2, 2, 2, 2, 2, 2, 2, 2, 2, 2, 2, 2, 2, 2, 2, 2, 2, 2, 2, 2, 2, 2, 2, 2, 2, 2, 2, 2, 2, 2, 2, 2, 2, 2, 2, 2, 2, 2, 2, 2, 2, 2, 2, 2, 2, 2, 2, 2, 2, 3 ),
 ( 0.6856214849132036271, 0.6875000000000000000, 0.6916666666666666519, 0.6958333333333333037, 0.6999999999999999556, 0.7041666666666667185, 0.7083333333333333703, 0.7125000000000000222, 0.7166666666666666741, 0.7208333333333333259, 0.7249999999999999778, 0.7291666666666666297, 0.7333333333333332815, 0.7375000000000000444, 0.7416666666666666963, 0.7458333333333333481, 0.7500000000000000000, 0.7541666666666666519, 0.7583333333333333037, 0.7624999999999999556, 0.7666666666666667185, 0.7708333333333333703, 0.7750000000000000222, 0.7791666666666666741, 0.7833333333333333259, 0.7874999999999999778, 0.7916666666666666297, 0.7958333333333332815, 0.8000000000000000444, 0.8041666666666666963, 0.8083333333333333481, 0.8125000000000000000, 0.8166666666666666519, 0.8208333333333333037, 0.8249999999999999556, 0.8291666666666667185, 0.8333333333333333703, 0.8375000000000000222, 0.8416666666666666741, 0.8458333333333333259, 0.8499999999999999778, 0.8541666666666666297, 0.8583333333333332815, 0.8625000000000000444, 0.8666666666666666963, 0.8708333333333333481, 0.8750000000000000000, 0.8791666666666666519, 0.8833333333333333037, 0.8874999999999999556, 0.8916666666666667185, 0.8958333333333333703, 0.9000000000000000222, 0.9041666666666666741, 0.9083333333333333259, 0.9124999999999999778, 0.9166666666666666297, 0.9208333333333332815, 0.9250000000000000444, 0.9291666666666666963, 0.9333333333333333481, 0.9375000000000000000, 0.9416666666666666519, 0.9458333333333333037, 0.9481214849132038047 ),
 .UNSPECIFIED. ) 
 CURVE ( )  GEOMETRIC_REPRESENTATION_ITEM ( )  RATIONAL_B_SPLINE_CURVE ( ( 0.9831275833774530959, 0.9846378761473346675, 1.000000000000000000, 0.9659258262890683122, 1.000000000000000000, 0.9659258262890683122, 1.000000000000000000, 0.9659258262890683122, 1.000000000000000000, 0.9659258262890683122, 1.000000000000000000, 0.9659258262890683122, 1.000000000000000000, 0.9659258262890683122, 1.000000000000000000, 0.9659258262890683122, 1.000000000000000000, 0.9659258262890683122, 1.000000000000000000, 0.9659258262890683122, 1.000000000000000000, 0.9659258262890683122, 1.000000000000000000, 0.9659258262890683122, 1.000000000000000000, 0.9659258262890683122, 1.000000000000000000, 0.9659258262890683122, 1.000000000000000000, 0.9659258262890683122, 1.000000000000000000, 0.9659258262890683122, 1.000000000000000000, 0.9659258262890683122, 1.000000000000000000, 0.9659258262890683122, 1.000000000000000000, 0.9659258262890683122, 1.000000000000000000, 0.9659258262890683122, 1.000000000000000000, 0.9659258262890683122, 1.000000000000000000, 0.9659258262890683122, 1.000000000000000000, 0.9659258262890683122, 1.000000000000000000, 0.9659258262890683122, 1.000000000000000000, 0.9659258262890683122, 1.000000000000000000, 0.9659258262890683122, 1.000000000000000000, 0.9659258262890683122, 1.000000000000000000, 0.9659258262890683122, 1.000000000000000000, 0.9659258262890683122, 1.000000000000000000, 0.9659258262890683122, 1.000000000000000000, 0.9659258262890683122, 1.000000000000000000, 0.9659258262890683122, 1.000000000000000000, 0.9659258262890683122, 1.000000000000000000, 0.9659258262890683122, 1.000000000000000000, 0.9659258262890683122, 1.000000000000000000, 0.9659258262890683122, 1.000000000000000000, 0.9659258262890683122, 1.000000000000000000, 0.9659258262890683122, 1.000000000000000000, 0.9659258262890683122, 1.000000000000000000, 0.9659258262890683122, 1.000000000000000000, 0.9659258262890683122, 1.000000000000000000, 0.9659258262890683122, 1.000000000000000000, 0.9659258262890683122, 1.000000000000000000, 0.9659258262890683122, 1.000000000000000000, 0.9659258262890683122, 1.000000000000000000, 0.9659258262890683122, 1.000000000000000000, 0.9659258262890683122, 1.000000000000000000, 0.9659258262890683122, 1.000000000000000000, 0.9659258262890683122, 1.000000000000000000, 0.9659258262890683122, 1.000000000000000000, 0.9659258262890683122, 1.000000000000000000, 0.9659258262890683122, 1.000000000000000000, 0.9659258262890683122, 1.000000000000000000, 0.9659258262890683122, 1.000000000000000000, 0.9659258262890683122, 1.000000000000000000, 0.9659258262890683122, 1.000000000000000000, 0.9659258262890683122, 1.000000000000000000, 0.9659258262890683122, 1.000000000000000000, 0.9659258262890683122, 1.000000000000000000, 0.9659258262890683122, 1.000000000000000000, 0.9659258262890683122, 1.000000000000000000, 0.9659258262890683122, 1.000000000000000000, 0.9659258262890683122, 1.000000000000000000, 0.9812879501417318684, 0.9831275833774535400 ) ) 
 REPRESENTATION_ITEM ( '' )  );
#17250=EDGE_CURVE ( 'NONE', #14101, #59522, #62930, .T. ) ;
#17252=CARTESIAN_POINT ( 'NONE',  ( -0.1998031496062994405, 0.3460692066303957537, -0.5623359580052492701 ) ) ;
#17253=CARTESIAN_POINT ( 'NONE',  ( -0.3392501089628017219, -0.1958661417322836718, -2.026902887139107712 ) ) ;
#17262=CARTESIAN_POINT ( 'NONE',  ( -0.1070741851644051862, -0.3996062992125986590, -1.566272965879265344 ) ) ;
#17264=CARTESIAN_POINT ( 'NONE',  ( 0.4091458600556403535, 0.2362204724409449896, -2.570209973753280863 ) ) ;
#17270=CARTESIAN_POINT ( 'NONE',  ( -0.3917322834645670104, -7.196005306013484475E-17, -1.698818897637795367 ) ) ;
#17275=CARTESIAN_POINT ( 'NONE',  ( 4.893765752498283308E-17, -0.3996062992125985480, -2.202755905511811108 ) ) ;
#17277=CARTESIAN_POINT ( 'NONE',  ( -9.787531504996567848E-17, 0.3996062992125986035, -0.7874015748031496509 ) ) ;
#17280=CARTESIAN_POINT ( 'NONE',  ( 0.1958661417322836440, -0.3392501089628017219, -2.603674540682414218 ) ) ;
#17290=CARTESIAN_POINT ( 'NONE',  ( -0.1049643490035301746, -0.3917322834645670659, -1.884495119913699002 ) ) ;
#17294=CARTESIAN_POINT ( 'NONE',  ( 4.797336870675656522E-17, -0.3917322834645670104, 0.08661417322834651100 ) ) ;
#17297=CARTESIAN_POINT ( 'NONE',  ( -0.1058382717557497937, -0.3949938075777411628, -0.2296587926509187083 ) ) ;
#17305=CARTESIAN_POINT ( 'NONE',  ( -0.3917322834645671770, 0.1049643490035302024, -1.446869709482626831 ) ) ;
#17307=CARTESIAN_POINT ( 'NONE',  ( 0.1049643490035303689, 0.3917322834645670104, -2.597769028871390606 ) ) ;
#17312=CARTESIAN_POINT ( 'NONE',  ( 0.1998031496062994405, -0.3460692066303958092, -0.7217847769028871152 ) ) ;
#17314=CARTESIAN_POINT ( 'NONE',  ( 0.3996062992125985480, 2.446882876249141654E-17, -0.1948818897637795422 ) ) ;
#17316=CARTESIAN_POINT ( 'NONE',  ( 4.893765752498283924E-17, -0.3996062992125986035, -2.125984251968504157 ) ) ;
#17321=CARTESIAN_POINT ( 'NONE',  ( -0.1265901696524986964, -0.4724409448818899238, -1.251312335958005173 ) ) ;
#17324=CARTESIAN_POINT ( 'NONE',  ( 0.3949938075777408852, 0.1058382717557500435, -0.5164041994750657727 ) ) ;
#17330=CYLINDRICAL_SURFACE ( 'NONE', #78942, 0.4724409448818898682 ) ;
#17337=CARTESIAN_POINT ( 'NONE',  ( -0.1998031496062994405, 0.3460692066303957537, -1.664698162729658870 ) ) ;
#17339=CARTESIAN_POINT ( 'NONE',  ( -0.1049643490035307020, 0.3917322834645669549, -1.573490813648293907 ) ) ;
#17341=CARTESIAN_POINT ( 'NONE',  ( -0.3913445824879501211, 0.02733964191758146006, 1.458593243026434070E-17 ) ) ;
#17362=CARTESIAN_POINT ( 'NONE',  ( 4.797336870675656522E-17, -0.3917322834645670659, -2.122722727855329783 ) ) ;
#17370=CARTESIAN_POINT ( 'NONE',  ( 0.2867679344610366554, -0.2867679344610365444, -2.137795275590550936 ) ) ;
#17373=CARTESIAN_POINT ( 'NONE',  ( 0.2362204724409449064, 0.4091458600556404646, -0.4593175853018372501 ) ) ;
#17374=CARTESIAN_POINT ( 'NONE',  ( -0.2891555358219911054, 0.2891555358219909388, -2.854330708661418026 ) ) ;
#17377=CARTESIAN_POINT ( 'NONE',  ( 0.3392501089628018329, 0.1958661417322835607, -1.540682414698162805 ) ) ;
#17379=CARTESIAN_POINT ( 'NONE',  ( 0.3458507752293908943, -0.3458507752293908943, -2.618110236220472675 ) ) ;
#17385=CARTESIAN_POINT ( 'NONE',  ( 0.2867679344610365999, 0.2867679344610365999, -0.5327890831682923212 ) ) ;
#17392=CARTESIAN_POINT ( 'NONE',  ( 0.3917322834645670104, 0.1049643490035304660, -2.168654486385513724 ) ) ;
#17399=CARTESIAN_POINT ( 'NONE',  ( 0.2867679344610365999, 0.2867679344610365999, -1.009842519685039353 ) ) ;
#17409=CARTESIAN_POINT ( 'NONE',  ( -0.1958661417322836718, 0.3392501089628017219, -2.839895013123359568 ) ) ;
#17411=ORIENTED_EDGE ( 'NONE', *, *, #7637, .F. ) ;
#17416=CARTESIAN_POINT ( 'NONE',  ( 0.3392501089628018329, 0.1958661417322835607, -0.8458005249343831800 ) ) ;
#17417=CARTESIAN_POINT ( 'NONE',  ( -0.4724409448818898682, -8.678599364036362592E-17, 0.1988188976377952832 ) ) ;
#17418=CARTESIAN_POINT ( 'NONE',  ( 0.3460692066303959202, -0.1998031496062991630, -2.229002624671915900 ) ) ;
#17427=CARTESIAN_POINT ( 'NONE',  ( -0.1070741851644056997, 0.3996062992125984925, -0.5557742782152230721 ) ) ;
#17429=CARTESIAN_POINT ( 'NONE',  ( 4.797336870675656522E-17, -0.3917322834645670104, -0.07086614173228342195 ) ) ;
#17437=CARTESIAN_POINT ( 'NONE',  ( 0.2867679344610365999, -0.2867679344610365999, -1.753261524113173708 ) ) ;
#17446=CARTESIAN_POINT ( 'NONE',  ( 0.3917322834645670659, 2.398668435337828261E-17, -0.5872896569891882246 ) ) ;
#17450=CARTESIAN_POINT ( 'NONE',  ( 0.2362204724409451007, -0.4091458600556402980, -2.215879265091863726 ) ) ;
#17470=CARTESIAN_POINT ( 'NONE',  ( 4.893765752498283308E-17, -0.3996062992125985480, -2.675196850393700920 ) ) ;
#17475=CARTESIAN_POINT ( 'NONE',  ( 0.1998031496062992740, 0.3460692066303959757, -1.876640419947506411 ) ) ;
#17476=CARTESIAN_POINT ( 'NONE',  ( 0.1058382717557500713, -0.3949938075777409408, -1.345144356955380704 ) ) ;
#17479=CARTESIAN_POINT ( 'NONE',  ( -9.594673741351313045E-17, 0.3917322834645670104, -0.4645669291338582751 ) ) ;
#17483=CARTESIAN_POINT ( 'NONE',  ( -0.3420746716998660508, -0.1974969037888706924, -2.176509186351706759 ) ) ;
#17487=CARTESIAN_POINT ( 'NONE',  ( 0.4091458600556404646, -0.2362204724409448231, -2.467191601049868677 ) ) ;
#17488=CARTESIAN_POINT ( 'NONE',  ( -0.3460692066303958092, -0.1998031496062994683, -1.784776902887138972 ) ) ;
#17489=CARTESIAN_POINT ( 'NONE',  ( 0.4091458600556403535, 0.2362204724409449896, -2.727690288713910949 ) ) ;
#17495=CARTESIAN_POINT ( 'NONE',  ( -0.3917322834645669549, -0.1049643490035306603, 0.1843832020997374643 ) ) ;
#17502=CARTESIAN_POINT ( 'NONE',  ( -0.1049643490035307020, 0.3917322834645669549, -0.2486876640419948270 ) ) ;
#17503=CARTESIAN_POINT ( 'NONE',  ( -0.1958661417322836718, 0.3392501089628017219, -1.422572178477690574 ) ) ;
#17504=CARTESIAN_POINT ( 'NONE',  ( 0.3917322834645669549, 0.1049643490035304660, -2.479002624671915900 ) ) ;
#17507=CARTESIAN_POINT ( 'NONE',  ( -9.674558042662121740E-17, 0.3949938075777409963, -2.519685039370078705 ) ) ;
#17511=CARTESIAN_POINT ( 'NONE',  ( 0.1070741851644053527, 0.3996062992125986590, -1.095800524934382958 ) ) ;
#17516=CARTESIAN_POINT ( 'NONE',  ( -0.2867679344610365999, 0.2867679344610364889, -0.5767716535433071723 ) ) ;
#17521=CARTESIAN_POINT ( 'NONE',  ( 0.1958661417322834775, 0.3392501089628018884, -0.1364829396325459021 ) ) ;
#17526=CARTESIAN_POINT ( 'NONE',  ( -0.2362204724409447953, -0.4091458600556404646, -1.797900262467191590 ) ) ;
#17529=CARTESIAN_POINT ( 'NONE',  ( 0.1265901696524989184, 0.4724409448818898127, -0.9383202099737532054 ) ) ;
#17535=CARTESIAN_POINT ( 'NONE',  ( 0.1958661417322834497, 0.3392501089628018329, -0.5393507629583185192 ) ) ;
#17537=CARTESIAN_POINT ( 'NONE',  ( -9.594673741351313045E-17, 0.3917322834645670104, -0.5570866141732284671 ) ) ;
#17542=CARTESIAN_POINT ( 'NONE',  ( -9.594673741351313045E-17, 0.3917322834645670104, -2.354330708661417138 ) ) ;
#17545=CARTESIAN_POINT ( 'NONE',  ( -0.2362204724409447953, -0.4091458600556404646, -0.6148293963254594097 ) ) ;
#17553=CARTESIAN_POINT ( 'NONE',  ( -0.4091458600556405756, 0.2362204724409446288, -0.3412073490813647969 ) ) ;
#17556=CARTESIAN_POINT ( 'NONE',  ( -0.3460692066303960313, 0.1998031496062989965, -1.992782152230971437 ) ) ;
#17565=CARTESIAN_POINT ( 'NONE',  ( 0.1070741851644053527, 0.3996062992125985480, -0.07020997375328086321 ) ) ;
#17566=CARTESIAN_POINT ( 'NONE',  ( -0.1070741851644056997, 0.3996062992125986035, -0.3215223097112860362 ) ) ;
#17567=CARTESIAN_POINT ( 'NONE',  ( 0.1974969037888704704, 0.3420746716998660508, -0.3018372703412073865 ) ) ;
#17568=CARTESIAN_POINT ( 'NONE',  ( 0.03178304480586199854, -0.3983403474834772418, -9.560572922657961637E-16 ) ) ;
#17572=CARTESIAN_POINT ( 'NONE',  ( 0.2891555358219910499, -0.2891555358219909944, -0.9625984251968502381 ) ) ;
#17577=CARTESIAN_POINT ( 'NONE',  ( -0.4724409448818899238, 0.1265901696524986686, -1.292650918635170454 ) ) ;
#17578=CARTESIAN_POINT ( 'NONE',  ( 0.2925321140481932369, -0.2925321140481931814, -2.460629921259842146 ) ) ;
#17580=( BOUNDED_SURFACE ( )  B_SPLINE_SURFACE ( 3, 2, ( 
 ( #22890, #3544, #54877, #60777, #47309, #16183, #34705, #41830, #72999, #17017, #61189, #54456, #3128, #42657, #48558, #22484, #16597, #15351, #41013, #60367, #2715, #54036, #28793, #48147, #35527, #80584, #42242, #67937, #61615, #3957, #69582, #30445, #19055, #56110, #75082, #43471, #17429, #70399, #37995, #43884, #83037, #76723, #43060, #11929, #68757, #37584, #75497, #31682, #6430, #81816, #30855, #32100, #69167, #56520, #44703, #31264, #63257, #24126, #57342, #12755, #44293, #49387, #12339, #38412, #11100, #64094, #76319, #36757, #25361, #51024, #57760, #23716, #5598, #62433, #82222, #4770, #24542, #49795, #17836, #24941, #56931, #11518, #37174, #62854, #50206, #75904, #5190, #18243, #82627, #50613, #18649, #69984, #63671, #6012, #45550, #7268, #64508, #78408, #78825, #72083, #46808, #72499, #40508, #13592, #52699, #46389, #40093, #66190, #33367, #65780, #6846, #70832, #33778, #26200, #20738, #27038, #58605, #39247, #39672, #14848, #59441, #34193, #45124, #19474, #71664, #64930, #14441, #8526, #122, #25777, #1794, #38830, #32940, #974, #21153, #51438, #8112, #19902, #13180, #71247, #26628, #77141, #52282, #32516, #51861, #58178, #27455, #547, #65363, #77568, #77987, #20316, #45968, #53115, #59030, #14015, #7700, #1385, #59858, #53537, #67431, #15263, #16092, #15681, #68267, #16511, #29527, #73757, #2209, #2630, #48055, #40923, #34615, #35025, #48881, #66604, #60280, #28286, #53948, #8938, #79661, #21977, #74164, #41737, #61101, #48463, #47639, #73334, #42154, #22397, #22806, #3452, #41342, #67021, #9354, #67849, #9765, #35436, #60689, #35854, #3039, #28704, #54366, #29117, #80078, #54787, #80490, #10188, #61522, #3868, #55190, #80897, #23211, #74581, #16926, #42564, #10603, #27877, #79245, #21560, #47222, #72911, #11003, #51652, #19265, #38627, #25995, #42969, #36662, #19688, #83250, #339, #64305, #68664, #62336, #81723, #77357, #76937, #25573, #4674, #13387, #17743, #6222, #38209, #6639, #43372, #32311, #74994, #30346, #57974, #56013, #45346, #71042, #69072, #11421, #39039, #58399, #24032, #49701, #64724, #63884, #75397, #7063, #31898, #57559, #17339, #32732, #759, #26420, #52073, #77780, #20114, #51238, #45761, #71460, #36260, #61929, #70615, #4272, #44918, #23622, #29933, #12970, #55597, #81308, #49292, #52909, #53333, #2836, #47431, #47846, #58827, #33158, #2005, #27250, #66396, #22189, #79872, #54157, #73124, #52493, #46604, #14646, #9155, #65152, #40711, #33572, #1184, #59234, #72300, #13807, #1595, #39466, #39890, #46184, #8734, #7489, #79042, #7911, #26835, #78202, #28499, #34404, #47014, #60486, #20532, #66822, #71881, #14230, #21361, #65577, #72708, #78623, #20947, #53741, #34828, #27667, #40303, #65983, #15055, #8321, #33987, #59649, #60072, #2427, #28083, #15474, #79449, #21769, #41131, #68871, #49087, #23010, #42770, #43174, #55809, #9563, #35234, #36879, #30567, #11219, #80289, #35647, #81516, #23837, #49505, #22603, #36059, #48263, #62557, #73960, #41544, #9978, #67233, #4892, #4478, #10402, #75198, #56232, #60897, #61731, #3249, #4068, #41949, #17542, #81930, #16306, #80697, #24241, #61308, #48678, #73552, #81104, #29735, #67644, #15896, #28912, #10804, #54576, #62139, #3665, #29328, #54989, #68466, #74373, #16717, #42357, #68055, #55398, #23421, #74787, #17138, #36464, #30148, #19581, #77252, #51136, #38107, #32626, #17950, #43587, #76430, #25888, #70941, #69288, #25470, #58289, #11635, #62970, #76018, #76831, #654, #19163, #83150, #70509, #51548, #30967, #82737, #44813, #70094, #49914, #24653, #5308, #37295, #75612, #82335, #45241, #56634, #12041, #32211, #69697, #50321, #12867, #13286, #6541, #38524, #31794, #38938, #64207, #12448, #64619, #6956, #57870, #18360, #236, #44004, #6122, #57457, #37697, #50731, #63372, #5707, #31378, #57043, #25056 ),
 ( #18758, #44402, #63783, #40610, #46494, #2320, #79346, #20007, #14547, #45658, #40199, #78095, #34303, #9048, #33045, #33471, #34723, #46079, #59133, #21667, #33882, #72190, #58714, #59964, #15368, #46910, #51969, #14952, #47326, #71354, #41029, #78933, #13700, #27980, #53639, #73017, #66715, #65882, #39356, #1491, #26311, #27144, #60383, #77677, #27564, #8218, #65040, #7377, #1079, #52808, #26732, #52386, #20426, #1903, #71772, #14125, #39778, #65472, #53223, #7806, #21256, #59548, #72605, #78518, #20842, #66293, #8632, #22906, #2732, #60793, #41442, #22083, #36774, #35129, #62041, #15790, #48164, #68372, #22501, #9456, #81006, #81417, #42673, #35962, #67952, #75098, #74688, #48574, #55708, #30046, #10710, #3146, #36367, #61631, #42257, #10295, #28809, #43076, #54893, #47742, #80598, #28393, #4378, #16615, #9874, #73859, #23733, #3973, #54473, #49404, #80186, #54052, #16200, #79766, #17446, #17034, #74271, #68773, #11117, #73440, #29637, #67126, #55297, #41847, #67537, #35543, #61204, #3561, #29226, #23320, #48990, #51037, #24955, #37598, #43486, #31696, #70413, #69998, #4786, #12353, #76738, #81832, #12769, #18663, #24142, #57355, #83051, #25374, #38426, #31280, #49813, #75919, #62450, #11944, #44716, #19068, #44308, #56945, #30463, #75513, #17852, #63272, #64108, #6443, #69182, #38009, #56126, #62870, #82238, #43900, #11533, #37190, #5206, #30870, #56536, #24557, #5612, #63687, #50223, #18258, #69597, #6025, #82642, #50628, #76333, #3419, #30311, #67398, #16474, #36626, #74129, #61068, #49257, #49669, #10967, #4234, #36224, #43335, #42932, #16891, #24001, #81690, #62303, #54752, #4640, #29898, #10566, #61893, #29082, #11386, #23175, #73720, #48845, #5063, #55979, #68232, #61484, #42121, #75359, #55562, #3833, #23586, #17707, #69036, #16059, #41706, #37043, #62725, #54332, #80458, #67816, #80042, #22361, #48020, #22767, #42530, #48430, #9733, #35404, #74959, #10153, #68627, #35819, #29493, #55152, #17305, #80863, #74546, #81270, #64372, #19760, #44572, #18114, #63542, #30732, #31549, #407, #58042, #31966, #18923, #13452, #82093, #24407, #57206, #6709, #51723, #50077, #6291, #39108, #75773, #43747, #56798, #57627, #64790, #58492, #63954, #51304, #32378, #11803, #5875, #25641, #50893, #56395, #5470, #69453, #37458, #63131, #31132, #26064, #82498, #76185, #13041, #50481, #24814, #77006, #77425, #70688, #19339, #12619, #45413, #44989, #76593, #71109, #18522, #38694, #44165, #69858, #12209, #70264, #38277, #37867, #82907, #25228, #45374, #76966, #12169, #37826, #64332, #367, #10625, #61953, #70643, #63503, #36281, #57588, #23644, #69820, #42589, #83278, #58002, #51264, #26022, #51681, #19715, #75016, #31926, #25601, #19295, #71070, #12578, #44946, #68289, #48903, #12999, #4293, #38655, #6249, #5835, #17362, #18884, #77384, #6669, #13413, #23234, #80919, #50856, #44128, #32340, #61545, #3889, #29549, #55211, #16947, #74604, #29956, #55621, #81330, #31508, #49315, #57168, #82867, #25190, #38235, #76556, #44533, #70223, #63913, #65181, #8349, #66011, #14260, #78229, #78651, #28113, #72736, #73151, #788, #58427, #27278, #52521, #34016, #47457, #21794, #79478, #15082, #77810, #71909, #39918, #34435, #7090, #59677, #58855, #26448, #1212, #65607, #39069, #26862, #64751, #7518, #71488, #2032, #32760, #20973, #33186, #52101, #20140, #53767, #27698, #72328, #2455, #45789, #8760, #13836, #39494, #46632, #20563, #14675, #46214, #7938, #79072, #60101, #52938, #33599, #59264, #40332, #1621, #53362, #21388, #47043, #40741, #66424, #41568, #67257, #47871, #22214, #73575, #29761, #80721, #16743, #4092, #15921, #9590, #81131, #61334, #61755, #42383, #35259, #60924, #3274, #55423, #55012, #3688, #28935, #74817, #80313, #67669, #16331, #68082, #22628, #10426, #54183, #54604, #9180, #36084, #81543 ),
 ( #79896, #23447, #10829, #49111, #17162, #48289, #73985, #41975, #42795, #23035, #29353, #10005, #68490, #35670, #48701, #74400, #36489, #62165, #4505, #30172, #55835, #34852, #23862, #49529, #15500, #41158, #66847, #60514, #2862, #28525, #75637, #83178, #76045, #49939, #70124, #37323, #82361, #56257, #12475, #70539, #63811, #38554, #64234, #32240, #5334, #44430, #38138, #31824, #57899, #25086, #57485, #81953, #62581, #25499, #17976, #6150, #18786, #50347, #30992, #31406, #6569, #51164, #25918, #36905, #11247, #63399, #56660, #76860, #265, #75222, #17567, #19192, #30591, #24680, #18389, #12895, #43200, #44842, #11665, #4923, #62995, #44031, #68895, #69723, #24266, #43613, #69314, #12067, #37725, #57070, #5734, #82764, #50759, #76460, #46528, #1522, #14983, #6987, #21289, #51578, #45272, #59164, #32655, #7835, #7411, #59999, #8249, #46943, #65503, #77280, #77706, #39813, #58322, #26340, #26761, #40642, #684, #52001, #20036, #45687, #71384, #13733, #39388, #65912, #33502, #52839, #40230, #65073, #33081, #33914, #14157, #58748, #72635, #27176, #1110, #20876, #66324, #59578, #70968, #13313, #8664, #34335, #2355, #52416, #78125, #1936, #27598, #53258, #20459, #78551, #46111, #19610, #71806, #38966, #72228, #64649, #14578, #78969, #48194, #4003, #81038, #21697, #16230, #47360, #41877, #79800, #35992, #10740, #34755, #35163, #36397, #47776, #60824, #23350, #35575, #73890, #60415, #61662, #17067, #48606, #53671, #16647, #49022, #73049, #42704, #80628, #15399, #29668, #55329, #74718, #68401, #67571, #41060, #3175, #28011, #28840, #62072, #79378, #29257, #9903, #66749, #9084, #2766, #54502, #28425, #54085, #22116, #3592, #73477, #15827, #41475, #67160, #54921, #9489, #22939, #61237, #74301, #80216, #22532, #42288, #67985, #10330, #4410, #62484, #43107, #23766, #38454, #36807, #63715, #17476, #49843, #70029, #24174, #11149, #82672, #83082, #44338, #37629, #69629, #76767, #76363, #50253, #57391, #31727, #12382, #4818, #38040, #63305, #43935, #11974, #30496, #6056, #37224, #17882, #68803, #30078, #25404, #18290, #11565, #18696, #5643, #31310, #51067, #56159, #81862, #19097, #75951, #50663, #56974, #75542, #43517, #69217, #44746, #24988, #70441, #62901, #12799, #5236, #56567, #30900, #55741, #82268, #81449, #24586, #49437, #75131, #65402, #46843, #78448, #13632, #39284, #65817, #1834, #13222, #64549, #72119, #64971, #38870, #59067, #26241, #71284, #45167, #1422, #59480, #52738, #27494, #53151, #21189, #77608, #33405, #27078, #20774, #72537, #14056, #46428, #70873, #51479, #14478, #6886, #40131, #7739, #7307, #19941, #20355, #78863, #8150, #14885, #25819, #166, #52320, #45591, #33815, #64140, #6473, #32143, #57799, #19514, #32977, #58644, #77182, #32556, #58219, #585, #51901, #1012, #26665, #78026, #46006, #71702, #39711, #72946, #9798, #74616, #22430, #34651, #2246, #27912, #29561, #35470, #73789, #3901, #79280, #10221, #40545, #34232, #48089, #21595, #80112, #79696, #48915, #80525, #35888, #54400, #66225, #66641, #28739, #47257, #15298, #15717, #55223, #40959, #8978, #60315, #2664, #28323, #53984, #22013, #22837, #59894, #53571, #80930, #23245, #61558, #47673, #73368, #48496, #74197, #16543, #41373, #3073, #67054, #8563, #9387, #35057, #60723, #16125, #41771, #54821, #67464, #42188, #61134, #3486, #29152, #67883, #5133, #68698, #24885, #82978, #23657, #24069, #25297, #36697, #49738, #69924, #24481, #37115, #49327, #50554, #5950, #37525, #42599, #5540, #12280, #61966, #31619, #69523, #4305, #76257, #18592, #44235, #57281, #30798, #29968, #75438, #16960, #17777, #37936, #63613, #18186, #56463, #50963, #68301, #10637, #43410, #36292, #55633, #81342, #75844, #75029, #17374, #43004, #11039, #43819, #62372, #11873, #50147, #63200, #4710, #30384, #69109, #31205, #62799, #56050, #81759, #11457 ),
 ( #56872, #82165, #82566, #19411, #52640, #58114, #45486, #77502, #20254, #480, #71600, #32039, #45062, #70338, #77923, #59377, #7638, #26136, #51797, #78344, #14377, #25714, #77078, #1326, #19837, #51374, #13952, #39610, #26566, #40035, #57698, #46328, #76660, #12693, #910, #60, #32875, #32452, #1735, #33308, #72021, #7204, #18993, #70765, #64865, #13115, #38767, #71183, #65721, #64444, #6780, #13525, #39181, #58544, #52220, #45903, #58969, #65299, #26975, #20675, #8053, #33715, #27391, #44642, #38352, #64027, #6367, #79184, #15198, #16032, #9294, #15618, #21500, #29054, #34550, #21913, #53884, #80014, #60216, #47993, #8462, #47158, #46747, #54301, #35788, #67371, #2566, #28225, #54725, #74100, #2147, #53474, #61040, #79598, #27814, #73692, #40857, #47575, #34131, #41678, #48400, #9705, #16446, #42091, #10124, #66541, #22332, #35376, #3390, #61456, #2978, #80430, #59793, #40445, #22740, #72849, #67787, #3804, #73269, #8874, #34964, #53052, #78764, #21088, #14789, #72440, #41275, #66961, #66125, #60627, #28643, #69833, #5445, #68201, #62275, #30284, #24788, #80834, #56369, #49229, #16863, #74932, #4612, #37840, #17277, #12183, #55533, #61866, #82068, #63518, #11359, #23558, #74515, #42500, #18498, #44141, #63107, #29466, #10539, #48816, #17680, #42905, #24381, #55124, #23147, #36196, #31106, #4207, #55950, #81663, #50457, #29871, #50053, #68600, #81242, #10940, #23973, #36597, #49641, #75333, #43310, #69008, #75748, #37017, #62698, #5037, #30706, #18088, #43723, #69427, #11780, #76161, #37433, #82473, #56773, #82883, #13427, #44547, #45387, #44961, #14273, #45804, #58869, #19732, #5848, #31940, #77398, #70237, #63928, #64346, #78244, #12592, #6264, #57601, #83291, #38250, #25614, #51277, #20154, #71084, #7103, #77824, #76980, #19309, #71501, #51695, #52116, #32773, #70658, #13014, #38668, #13849, #39083, #64764, #6683, #65195, #32354, #58015, #380, #58441, #26036, #802, #26465, #39507, #25203, #7532, #71923, #33204, #1227, #26876, #52536, #20576, #46227, #39935, #31524, #57181, #50869, #76569, #18897, #73902, #46647, #61674, #62083, #55342, #30090, #55753, #23778, #80228, #36004, #29679, #23362, #49449, #16660, #49033, #72341, #52950, #17078, #9502, #4015, #10343, #41890, #22544, #22952, #67583, #36408, #10751, #67997, #54933, #75143, #33614, #59277, #9915, #42715, #4424, #1633, #42300, #17488, #27292, #78664, #35175, #81050, #65621, #74729, #68411, #81461, #7952, #14689, #16243, #20985, #3604, #40345, #67173, #60836, #3188, #28852, #54514, #48207, #35587, #61250, #29269, #80640, #48619, #74313, #38466, #83094, #76374, #25001, #32155, #31739, #5655, #12811, #70453, #51079, #43531, #25415, #18707, #82683, #50675, #17894, #19109, #75964, #56579, #81874, #77193, #76777, #56986, #50266, #62915, #64151, #44349, #18302, #12394, #6485, #44757, #62496, #4831, #57811, #178, #25831, #49855, #5248, #51490, #43119, #68816, #75555, #31321, #69230, #11162, #11578, #36821, #30912, #30509, #56171, #57403, #63317, #24186, #37237, #82280, #70040, #24598, #38051, #43946, #69641, #11986, #37640, #63727, #6067, #39299, #52333, #72550, #27090, #39723, #51914, #27508, #8575, #40144, #45179, #8162, #14897, #64562, #34246, #72133, #6899, #53165, #78878, #21201, #59908, #33417, #32570, #78039, #19525, #58232, #53584, #46856, #59079, #26678, #64986, #40557, #78461, #20369, #14491, #66238, #1847, #38883, #599, #2261, #27926, #70884, #26255, #7321, #13233, #77621, #19954, #45604, #65416, #71298, #13646, #32990, #58659, #1025, #46021, #71715, #33827, #7752, #14070, #1434, #52753, #20786, #46442, #65829, #59493, #3918, #61985, #2679, #3091, #4322, #15734, #28755, #48933, #3503, #16143, #28339, #29579, #68317, #16561, #21611, #67901, #74634, #40975, #10654, #48516, #66657, #55242, #80949, #23264 ) ),
 .UNSPECIFIED., .F., .F., .F. ) 
 B_SPLINE_SURFACE_WITH_KNOTS ( ( 4, 4 ),
 ( 3, 2, 2, 2, 2, 2, 2, 2, 2, 2, 2, 2, 2, 2, 2, 2, 2, 2, 2, 2, 2, 2, 2, 2, 2, 2, 2, 2, 2, 2, 2, 2, 2, 2, 2, 2, 2, 2, 2, 2, 2, 2, 2, 2, 2, 2, 2, 2, 2, 2, 2, 2, 2, 2, 2, 2, 2, 2, 2, 2, 2, 2, 2, 2, 2, 2, 2, 2, 2, 2, 2, 2, 2, 2, 2, 2, 2, 2, 2, 2, 2, 2, 2, 2, 2, 2, 2, 2, 2, 2, 2, 2, 2, 2, 2, 2, 2, 2, 2, 2, 2, 2, 2, 2, 2, 2, 2, 2, 2, 2, 2, 2, 2, 2, 2, 2, 2, 2, 2, 2, 2, 2, 2, 2, 2, 2, 2, 2, 2, 2, 2, 2, 2, 2, 2, 2, 2, 2, 2, 2, 2, 2, 2, 2, 2, 2, 2, 2, 2, 2, 2, 2, 2, 2, 2, 2, 2, 2, 2, 2, 2, 2, 2, 2, 2, 2, 2, 2, 2, 2, 2, 2, 2, 2, 2, 2, 2, 2, 2, 2, 2, 2, 2, 2, 2, 2, 2, 2, 2, 2, 2, 2, 2, 2, 2, 2, 2, 2, 2, 2, 2, 2, 2, 2, 2, 2, 2, 2, 2, 2, 2, 2, 2, 2, 2, 2, 2, 2, 2, 2, 2, 2, 2, 2, 2, 2, 2, 2, 2, 2, 2, 2, 2, 2, 2, 2, 2, 3 ),
 ( 0.000000000000000000, 1.000000000000000000 ),
 ( 0.000000000000000000, 0.004166666666666666609, 0.008333333333333333218, 0.01250000000000000069, 0.01666666666666666644, 0.02083333333333333218, 0.02500000000000000139, 0.02916666666666666713, 0.03333333333333333287, 0.03749999999999999861, 0.04166666666666666435, 0.04583333333333333010, 0.05000000000000000278, 0.05416666666666666852, 0.05833333333333333426, 0.06250000000000000000, 0.06666666666666666574, 0.07083333333333333148, 0.07499999999999999722, 0.07916666666666666297, 0.08333333333333332871, 0.08749999999999999445, 0.09166666666666666019, 0.09583333333333333981, 0.1000000000000000056, 0.1041666666666666713, 0.1083333333333333370, 0.1125000000000000028, 0.1166666666666666685, 0.1208333333333333343, 0.1250000000000000000, 0.1291666666666666796, 0.1333333333333333315, 0.1375000000000000111, 0.1416666666666666630, 0.1458333333333333426, 0.1499999999999999944, 0.1541666666666666741, 0.1583333333333333259, 0.1625000000000000056, 0.1666666666666666574, 0.1708333333333333370, 0.1749999999999999889, 0.1791666666666666685, 0.1833333333333333204, 0.1875000000000000000, 0.1916666666666666796, 0.1958333333333333315, 0.2000000000000000111, 0.2041666666666666630, 0.2083333333333333426, 0.2124999999999999944, 0.2166666666666666741, 0.2208333333333333259, 0.2250000000000000056, 0.2291666666666666574, 0.2333333333333333370, 0.2374999999999999889, 0.2416666666666666685, 0.2458333333333333204, 0.2500000000000000000, 0.2541666666666666519, 0.2583333333333333592, 0.2625000000000000111, 0.2666666666666666630, 0.2708333333333333148, 0.2750000000000000222, 0.2791666666666666741, 0.2833333333333333259, 0.2874999999999999778, 0.2916666666666666852, 0.2958333333333333370, 0.2999999999999999889, 0.3041666666666666408, 0.3083333333333333481, 0.3125000000000000000, 0.3166666666666666519, 0.3208333333333333592, 0.3250000000000000111, 0.3291666666666666630, 0.3333333333333333148, 0.3375000000000000222, 0.3416666666666666741, 0.3458333333333333259, 0.3499999999999999778, 0.3541666666666666852, 0.3583333333333333370, 0.3624999999999999889, 0.3666666666666666408, 0.3708333333333333481, 0.3750000000000000000, 0.3791666666666666519, 0.3833333333333333592, 0.3875000000000000111, 0.3916666666666666630, 0.3958333333333333148, 0.4000000000000000222, 0.4041666666666666741, 0.4083333333333333259, 0.4124999999999999778, 0.4166666666666666852, 0.4208333333333333370, 0.4249999999999999889, 0.4291666666666666408, 0.4333333333333333481, 0.4375000000000000000, 0.4416666666666666519, 0.4458333333333333592, 0.4500000000000000111, 0.4541666666666666630, 0.4583333333333333148, 0.4625000000000000222, 0.4666666666666666741, 0.4708333333333333259, 0.4749999999999999778, 0.4791666666666666852, 0.4833333333333333370, 0.4874999999999999889, 0.4916666666666666408, 0.4958333333333333481, 0.5000000000000000000, 0.5041666666666666519, 0.5083333333333333037, 0.5124999999999999556, 0.5166666666666667185, 0.5208333333333333703, 0.5250000000000000222, 0.5291666666666666741, 0.5333333333333333259, 0.5374999999999999778, 0.5416666666666666297, 0.5458333333333332815, 0.5500000000000000444, 0.5541666666666666963, 0.5583333333333333481, 0.5625000000000000000, 0.5666666666666666519, 0.5708333333333333037, 0.5749999999999999556, 0.5791666666666667185, 0.5833333333333333703, 0.5875000000000000222, 0.5916666666666666741, 0.5958333333333333259, 0.5999999999999999778, 0.6041666666666666297, 0.6083333333333332815, 0.6125000000000000444, 0.6166666666666666963, 0.6208333333333333481, 0.6250000000000000000, 0.6291666666666666519, 0.6333333333333333037, 0.6374999999999999556, 0.6416666666666667185, 0.6458333333333333703, 0.6500000000000000222, 0.6541666666666666741, 0.6583333333333333259, 0.6624999999999999778, 0.6666666666666666297, 0.6708333333333332815, 0.6750000000000000444, 0.6791666666666666963, 0.6833333333333333481, 0.6875000000000000000, 0.6916666666666666519, 0.6958333333333333037, 0.6999999999999999556, 0.7041666666666667185, 0.7083333333333333703, 0.7125000000000000222, 0.7166666666666666741, 0.7208333333333333259, 0.7249999999999999778, 0.7291666666666666297, 0.7333333333333332815, 0.7375000000000000444, 0.7416666666666666963, 0.7458333333333333481, 0.7500000000000000000, 0.7541666666666666519, 0.7583333333333333037, 0.7624999999999999556, 0.7666666666666667185, 0.7708333333333333703, 0.7750000000000000222, 0.7791666666666666741, 0.7833333333333333259, 0.7874999999999999778, 0.7916666666666666297, 0.7958333333333332815, 0.8000000000000000444, 0.8041666666666666963, 0.8083333333333333481, 0.8125000000000000000, 0.8166666666666666519, 0.8208333333333333037, 0.8249999999999999556, 0.8291666666666667185, 0.8333333333333333703, 0.8375000000000000222, 0.8416666666666666741, 0.8458333333333333259, 0.8499999999999999778, 0.8541666666666666297, 0.8583333333333332815, 0.8625000000000000444, 0.8666666666666666963, 0.8708333333333333481, 0.8750000000000000000, 0.8791666666666666519, 0.8833333333333333037, 0.8874999999999999556, 0.8916666666666667185, 0.8958333333333333703, 0.9000000000000000222, 0.9041666666666666741, 0.9083333333333333259, 0.9124999999999999778, 0.9166666666666666297, 0.9208333333333332815, 0.9250000000000000444, 0.9291666666666666963, 0.9333333333333333481, 0.9375000000000000000, 0.9416666666666666519, 0.9458333333333333037, 0.9499999999999999556, 0.9541666666666667185, 0.9583333333333333703, 0.9625000000000000222, 0.9666666666666666741, 0.9708333333333333259, 0.9749999999999999778, 0.9791666666666666297, 0.9833333333333332815, 0.9875000000000000444 ),
 .UNSPECIFIED. ) 
 GEOMETRIC_REPRESENTATION_ITEM ( )  RATIONAL_B_SPLINE_SURFACE ( (
 ( 1.000000000000000000, 0.9659258262890683122, 1.000000000000000000, 0.9659258262890683122, 1.000000000000000000, 0.9659258262890683122, 1.000000000000000000, 0.9659258262890683122, 1.000000000000000000, 0.9659258262890683122, 1.000000000000000000, 0.9659258262890683122, 1.000000000000000000, 0.9659258262890683122, 1.000000000000000000, 0.9659258262890683122, 1.000000000000000000, 0.9659258262890683122, 1.000000000000000000, 0.9659258262890683122, 1.000000000000000000, 0.9659258262890683122, 1.000000000000000000, 0.9659258262890683122, 1.000000000000000000, 0.9659258262890683122, 1.000000000000000000, 0.9659258262890683122, 1.000000000000000000, 0.9659258262890683122, 1.000000000000000000, 0.9659258262890683122, 1.000000000000000000, 0.9659258262890683122, 1.000000000000000000, 0.9659258262890683122, 1.000000000000000000, 0.9659258262890683122, 1.000000000000000000, 0.9659258262890683122, 1.000000000000000000, 0.9659258262890683122, 1.000000000000000000, 0.9659258262890683122, 1.000000000000000000, 0.9659258262890683122, 1.000000000000000000, 0.9659258262890683122, 1.000000000000000000, 0.9659258262890683122, 1.000000000000000000, 0.9659258262890683122, 1.000000000000000000, 0.9659258262890683122, 1.000000000000000000, 0.9659258262890683122, 1.000000000000000000, 0.9659258262890683122, 1.000000000000000000, 0.9659258262890683122, 1.000000000000000000, 0.9659258262890683122, 1.000000000000000000, 0.9659258262890683122, 1.000000000000000000, 0.9659258262890683122, 1.000000000000000000, 0.9659258262890683122, 1.000000000000000000, 0.9659258262890683122, 1.000000000000000000, 0.9659258262890683122, 1.000000000000000000, 0.9659258262890683122, 1.000000000000000000, 0.9659258262890683122, 1.000000000000000000, 0.9659258262890683122, 1.000000000000000000, 0.9659258262890683122, 1.000000000000000000, 0.9659258262890683122, 1.000000000000000000, 0.9659258262890683122, 1.000000000000000000, 0.9659258262890683122, 1.000000000000000000, 0.9659258262890683122, 1.000000000000000000, 0.9659258262890683122, 1.000000000000000000, 0.9659258262890683122, 1.000000000000000000, 0.9659258262890683122, 1.000000000000000000, 0.9659258262890683122, 1.000000000000000000, 0.9659258262890683122, 1.000000000000000000, 0.9659258262890683122, 1.000000000000000000, 0.9659258262890683122, 1.000000000000000000, 0.9659258262890683122, 1.000000000000000000, 0.9659258262890683122, 1.000000000000000000, 0.9659258262890683122, 1.000000000000000000, 0.9659258262890683122, 1.000000000000000000, 0.9659258262890683122, 1.000000000000000000, 0.9659258262890683122, 1.000000000000000000, 0.9659258262890683122, 1.000000000000000000, 0.9659258262890683122, 1.000000000000000000, 0.9659258262890683122, 1.000000000000000000, 0.9659258262890683122, 1.000000000000000000, 0.9659258262890683122, 1.000000000000000000, 0.9659258262890683122, 1.000000000000000000, 0.9659258262890683122, 1.000000000000000000, 0.9659258262890683122, 1.000000000000000000, 0.9659258262890683122, 1.000000000000000000, 0.9659258262890683122, 1.000000000000000000, 0.9659258262890683122, 1.000000000000000000, 0.9659258262890683122, 1.000000000000000000, 0.9659258262890683122, 1.000000000000000000, 0.9659258262890683122, 1.000000000000000000, 0.9659258262890683122, 1.000000000000000000, 0.9659258262890683122, 1.000000000000000000, 0.9659258262890683122, 1.000000000000000000, 0.9659258262890683122, 1.000000000000000000, 0.9659258262890683122, 1.000000000000000000, 0.9659258262890683122, 1.000000000000000000, 0.9659258262890683122, 1.000000000000000000, 0.9659258262890683122, 1.000000000000000000, 0.9659258262890683122, 1.000000000000000000, 0.9659258262890683122, 1.000000000000000000, 0.9659258262890683122, 1.000000000000000000, 0.9659258262890683122, 1.000000000000000000, 0.9659258262890683122, 1.000000000000000000, 0.9659258262890683122, 1.000000000000000000, 0.9659258262890683122, 1.000000000000000000, 0.9659258262890683122, 1.000000000000000000, 0.9659258262890683122, 1.000000000000000000, 0.9659258262890683122, 1.000000000000000000, 0.9659258262890683122, 1.000000000000000000, 0.9659258262890683122, 1.000000000000000000, 0.9659258262890683122, 1.000000000000000000, 0.9659258262890683122, 1.000000000000000000, 0.9659258262890683122, 1.000000000000000000, 0.9659258262890683122, 1.000000000000000000, 0.9659258262890683122, 1.000000000000000000, 0.9659258262890683122, 1.000000000000000000, 0.9659258262890683122, 1.000000000000000000, 0.9659258262890683122, 1.000000000000000000, 0.9659258262890683122, 1.000000000000000000, 0.9659258262890683122, 1.000000000000000000, 0.9659258262890683122, 1.000000000000000000, 0.9659258262890683122, 1.000000000000000000, 0.9659258262890683122, 1.000000000000000000, 0.9659258262890683122, 1.000000000000000000, 0.9659258262890683122, 1.000000000000000000, 0.9659258262890683122, 1.000000000000000000, 0.9659258262890683122, 1.000000000000000000, 0.9659258262890683122, 1.000000000000000000, 0.9659258262890683122, 1.000000000000000000, 0.9659258262890683122, 1.000000000000000000, 0.9659258262890683122, 1.000000000000000000, 0.9659258262890683122, 1.000000000000000000, 0.9659258262890683122, 1.000000000000000000, 0.9659258262890683122, 1.000000000000000000, 0.9659258262890683122, 1.000000000000000000, 0.9659258262890683122, 1.000000000000000000, 0.9659258262890683122, 1.000000000000000000, 0.9659258262890683122, 1.000000000000000000, 0.9659258262890683122, 1.000000000000000000, 0.9659258262890683122, 1.000000000000000000, 0.9659258262890683122, 1.000000000000000000, 0.9659258262890683122, 1.000000000000000000, 0.9659258262890683122, 1.000000000000000000, 0.9659258262890683122, 1.000000000000000000, 0.9659258262890683122, 1.000000000000000000, 0.9659258262890683122, 1.000000000000000000, 0.9659258262890683122, 1.000000000000000000, 0.9659258262890683122, 1.000000000000000000, 0.9659258262890683122, 1.000000000000000000, 0.9659258262890683122, 1.000000000000000000, 0.9659258262890683122, 1.000000000000000000, 0.9659258262890683122, 1.000000000000000000, 0.9659258262890683122, 1.000000000000000000, 0.9659258262890683122, 1.000000000000000000, 0.9659258262890683122, 1.000000000000000000, 0.9659258262890683122, 1.000000000000000000, 0.9659258262890683122, 1.000000000000000000, 0.9659258262890683122, 1.000000000000000000, 0.9659258262890683122, 1.000000000000000000, 0.9659258262890683122, 1.000000000000000000, 0.9659258262890683122, 1.000000000000000000, 0.9659258262890683122, 1.000000000000000000, 0.9659258262890683122, 1.000000000000000000, 0.9659258262890683122, 1.000000000000000000, 0.9659258262890683122, 1.000000000000000000, 0.9659258262890683122, 1.000000000000000000, 0.9659258262890683122, 1.000000000000000000, 0.9659258262890683122, 1.000000000000000000, 0.9659258262890683122, 1.000000000000000000, 0.9659258262890683122, 1.000000000000000000, 0.9659258262890683122, 1.000000000000000000, 0.9659258262890683122, 1.000000000000000000, 0.9659258262890683122, 1.000000000000000000, 0.9659258262890683122, 1.000000000000000000, 0.9659258262890683122, 1.000000000000000000, 0.9659258262890683122, 1.000000000000000000, 0.9659258262890683122, 1.000000000000000000, 0.9659258262890683122, 1.000000000000000000, 0.9659258262890683122, 1.000000000000000000, 0.9659258262890683122, 1.000000000000000000, 0.9659258262890683122, 1.000000000000000000, 0.9659258262890683122, 1.000000000000000000, 0.9659258262890683122, 1.000000000000000000, 0.9659258262890683122, 1.000000000000000000, 0.9659258262890683122, 1.000000000000000000, 0.9659258262890683122, 1.000000000000000000, 0.9659258262890683122, 1.000000000000000000, 0.9659258262890683122, 1.000000000000000000, 0.9659258262890683122, 1.000000000000000000, 0.9659258262890683122, 1.000000000000000000, 0.9659258262890683122, 1.000000000000000000, 0.9659258262890683122, 1.000000000000000000, 0.9659258262890683122, 1.000000000000000000, 0.9659258262890683122, 1.000000000000000000, 0.9659258262890683122, 1.000000000000000000, 0.9659258262890683122, 1.000000000000000000, 0.9659258262890683122, 1.000000000000000000, 0.9659258262890683122, 1.000000000000000000, 0.9659258262890683122, 1.000000000000000000, 0.9659258262890683122, 1.000000000000000000, 0.9659258262890683122, 1.000000000000000000, 0.9659258262890683122, 1.000000000000000000, 0.9659258262890683122, 1.000000000000000000, 0.9659258262890683122, 1.000000000000000000, 0.9659258262890683122, 1.000000000000000000, 0.9659258262890683122, 1.000000000000000000, 0.9659258262890683122, 1.000000000000000000, 0.9659258262890683122, 1.000000000000000000, 0.9659258262890683122, 1.000000000000000000, 0.9659258262890683122, 1.000000000000000000, 0.9659258262890683122, 1.000000000000000000, 0.9659258262890683122, 1.000000000000000000, 0.9659258262890683122, 1.000000000000000000, 0.9659258262890683122, 1.000000000000000000, 0.9659258262890683122, 1.000000000000000000, 0.9659258262890683122, 1.000000000000000000, 0.9659258262890683122, 1.000000000000000000, 0.9659258262890683122, 1.000000000000000000, 0.9659258262890683122, 1.000000000000000000, 0.9659258262890683122, 1.000000000000000000, 0.9659258262890683122, 1.000000000000000000, 0.9659258262890683122, 1.000000000000000000, 0.9659258262890683122, 1.000000000000000000, 0.9659258262890683122, 1.000000000000000000, 0.9659258262890683122, 1.000000000000000000, 0.9659258262890683122, 1.000000000000000000, 0.9659258262890683122, 1.000000000000000000, 0.9659258262890683122, 1.000000000000000000, 0.9659258262890683122, 1.000000000000000000, 0.9659258262890683122, 1.000000000000000000, 0.9659258262890683122, 1.000000000000000000, 0.9659258262890683122, 1.000000000000000000, 0.9659258262890683122, 1.000000000000000000, 0.9659258262890683122, 1.000000000000000000, 0.9659258262890683122, 1.000000000000000000, 0.9659258262890683122, 1.000000000000000000, 0.9659258262890683122, 1.000000000000000000, 0.9659258262890683122, 1.000000000000000000, 0.9659258262890683122, 1.000000000000000000, 0.9659258262890683122, 1.000000000000000000, 0.9659258262890683122, 1.000000000000000000, 0.9659258262890683122, 1.000000000000000000, 0.9659258262890683122, 1.000000000000000000, 0.9659258262890683122, 1.000000000000000000, 0.9659258262890683122, 1.000000000000000000, 0.9659258262890683122, 1.000000000000000000, 0.9659258262890683122, 1.000000000000000000, 0.9659258262890683122, 1.000000000000000000, 0.9659258262890683122, 1.000000000000000000, 0.9659258262890683122, 1.000000000000000000, 0.9659258262890683122, 1.000000000000000000, 0.9659258262890683122, 1.000000000000000000, 0.9659258262890683122, 1.000000000000000000, 0.9659258262890683122, 1.000000000000000000, 0.9659258262890683122, 1.000000000000000000, 0.9659258262890683122, 1.000000000000000000),
 ( 0.8047378541243613848, 0.7773170766911654539, 0.8047378541243613848, 0.7773170766911654539, 0.8047378541243613848, 0.7773170766911654539, 0.8047378541243613848, 0.7773170766911654539, 0.8047378541243613848, 0.7773170766911654539, 0.8047378541243613848, 0.7773170766911654539, 0.8047378541243613848, 0.7773170766911654539, 0.8047378541243613848, 0.7773170766911654539, 0.8047378541243613848, 0.7773170766911654539, 0.8047378541243613848, 0.7773170766911654539, 0.8047378541243613848, 0.7773170766911654539, 0.8047378541243613848, 0.7773170766911654539, 0.8047378541243613848, 0.7773170766911654539, 0.8047378541243613848, 0.7773170766911654539, 0.8047378541243613848, 0.7773170766911654539, 0.8047378541243613848, 0.7773170766911654539, 0.8047378541243613848, 0.7773170766911654539, 0.8047378541243613848, 0.7773170766911654539, 0.8047378541243613848, 0.7773170766911654539, 0.8047378541243613848, 0.7773170766911654539, 0.8047378541243613848, 0.7773170766911654539, 0.8047378541243613848, 0.7773170766911654539, 0.8047378541243613848, 0.7773170766911654539, 0.8047378541243613848, 0.7773170766911654539, 0.8047378541243613848, 0.7773170766911654539, 0.8047378541243613848, 0.7773170766911654539, 0.8047378541243613848, 0.7773170766911654539, 0.8047378541243613848, 0.7773170766911654539, 0.8047378541243613848, 0.7773170766911654539, 0.8047378541243613848, 0.7773170766911654539, 0.8047378541243613848, 0.7773170766911654539, 0.8047378541243613848, 0.7773170766911654539, 0.8047378541243613848, 0.7773170766911654539, 0.8047378541243613848, 0.7773170766911654539, 0.8047378541243613848, 0.7773170766911654539, 0.8047378541243613848, 0.7773170766911654539, 0.8047378541243613848, 0.7773170766911654539, 0.8047378541243613848, 0.7773170766911654539, 0.8047378541243613848, 0.7773170766911654539, 0.8047378541243613848, 0.7773170766911654539, 0.8047378541243613848, 0.7773170766911654539, 0.8047378541243613848, 0.7773170766911654539, 0.8047378541243613848, 0.7773170766911654539, 0.8047378541243613848, 0.7773170766911654539, 0.8047378541243613848, 0.7773170766911654539, 0.8047378541243613848, 0.7773170766911654539, 0.8047378541243613848, 0.7773170766911654539, 0.8047378541243613848, 0.7773170766911654539, 0.8047378541243613848, 0.7773170766911654539, 0.8047378541243613848, 0.7773170766911654539, 0.8047378541243613848, 0.7773170766911654539, 0.8047378541243613848, 0.7773170766911654539, 0.8047378541243613848, 0.7773170766911654539, 0.8047378541243613848, 0.7773170766911654539, 0.8047378541243613848, 0.7773170766911654539, 0.8047378541243613848, 0.7773170766911654539, 0.8047378541243613848, 0.7773170766911654539, 0.8047378541243613848, 0.7773170766911654539, 0.8047378541243613848, 0.7773170766911654539, 0.8047378541243613848, 0.7773170766911654539, 0.8047378541243613848, 0.7773170766911654539, 0.8047378541243613848, 0.7773170766911654539, 0.8047378541243613848, 0.7773170766911654539, 0.8047378541243613848, 0.7773170766911654539, 0.8047378541243613848, 0.7773170766911654539, 0.8047378541243613848, 0.7773170766911654539, 0.8047378541243613848, 0.7773170766911654539, 0.8047378541243613848, 0.7773170766911654539, 0.8047378541243613848, 0.7773170766911654539, 0.8047378541243613848, 0.7773170766911654539, 0.8047378541243613848, 0.7773170766911654539, 0.8047378541243613848, 0.7773170766911654539, 0.8047378541243613848, 0.7773170766911654539, 0.8047378541243613848, 0.7773170766911654539, 0.8047378541243613848, 0.7773170766911654539, 0.8047378541243613848, 0.7773170766911654539, 0.8047378541243613848, 0.7773170766911654539, 0.8047378541243613848, 0.7773170766911654539, 0.8047378541243613848, 0.7773170766911654539, 0.8047378541243613848, 0.7773170766911654539, 0.8047378541243613848, 0.7773170766911654539, 0.8047378541243613848, 0.7773170766911654539, 0.8047378541243613848, 0.7773170766911654539, 0.8047378541243613848, 0.7773170766911654539, 0.8047378541243613848, 0.7773170766911654539, 0.8047378541243613848, 0.7773170766911654539, 0.8047378541243613848, 0.7773170766911654539, 0.8047378541243613848, 0.7773170766911654539, 0.8047378541243613848, 0.7773170766911654539, 0.8047378541243613848, 0.7773170766911654539, 0.8047378541243613848, 0.7773170766911654539, 0.8047378541243613848, 0.7773170766911654539, 0.8047378541243613848, 0.7773170766911654539, 0.8047378541243613848, 0.7773170766911654539, 0.8047378541243613848, 0.7773170766911654539, 0.8047378541243613848, 0.7773170766911654539, 0.8047378541243613848, 0.7773170766911654539, 0.8047378541243613848, 0.7773170766911654539, 0.8047378541243613848, 0.7773170766911654539, 0.8047378541243613848, 0.7773170766911654539, 0.8047378541243613848, 0.7773170766911654539, 0.8047378541243613848, 0.7773170766911654539, 0.8047378541243613848, 0.7773170766911654539, 0.8047378541243613848, 0.7773170766911654539, 0.8047378541243613848, 0.7773170766911654539, 0.8047378541243613848, 0.7773170766911654539, 0.8047378541243613848, 0.7773170766911654539, 0.8047378541243613848, 0.7773170766911654539, 0.8047378541243613848, 0.7773170766911654539, 0.8047378541243613848, 0.7773170766911654539, 0.8047378541243613848, 0.7773170766911654539, 0.8047378541243613848, 0.7773170766911654539, 0.8047378541243613848, 0.7773170766911654539, 0.8047378541243613848, 0.7773170766911654539, 0.8047378541243613848, 0.7773170766911654539, 0.8047378541243613848, 0.7773170766911654539, 0.8047378541243613848, 0.7773170766911654539, 0.8047378541243613848, 0.7773170766911654539, 0.8047378541243613848, 0.7773170766911654539, 0.8047378541243613848, 0.7773170766911654539, 0.8047378541243613848, 0.7773170766911654539, 0.8047378541243613848, 0.7773170766911654539, 0.8047378541243613848, 0.7773170766911654539, 0.8047378541243613848, 0.7773170766911654539, 0.8047378541243613848, 0.7773170766911654539, 0.8047378541243613848, 0.7773170766911654539, 0.8047378541243613848, 0.7773170766911654539, 0.8047378541243613848, 0.7773170766911654539, 0.8047378541243613848, 0.7773170766911654539, 0.8047378541243613848, 0.7773170766911654539, 0.8047378541243613848, 0.7773170766911654539, 0.8047378541243613848, 0.7773170766911654539, 0.8047378541243613848, 0.7773170766911654539, 0.8047378541243613848, 0.7773170766911654539, 0.8047378541243613848, 0.7773170766911654539, 0.8047378541243613848, 0.7773170766911654539, 0.8047378541243613848, 0.7773170766911654539, 0.8047378541243613848, 0.7773170766911654539, 0.8047378541243613848, 0.7773170766911654539, 0.8047378541243613848, 0.7773170766911654539, 0.8047378541243613848, 0.7773170766911654539, 0.8047378541243613848, 0.7773170766911654539, 0.8047378541243613848, 0.7773170766911654539, 0.8047378541243613848, 0.7773170766911654539, 0.8047378541243613848, 0.7773170766911654539, 0.8047378541243613848, 0.7773170766911654539, 0.8047378541243613848, 0.7773170766911654539, 0.8047378541243613848, 0.7773170766911654539, 0.8047378541243613848, 0.7773170766911654539, 0.8047378541243613848, 0.7773170766911654539, 0.8047378541243613848, 0.7773170766911654539, 0.8047378541243613848, 0.7773170766911654539, 0.8047378541243613848, 0.7773170766911654539, 0.8047378541243613848, 0.7773170766911654539, 0.8047378541243613848, 0.7773170766911654539, 0.8047378541243613848, 0.7773170766911654539, 0.8047378541243613848, 0.7773170766911654539, 0.8047378541243613848, 0.7773170766911654539, 0.8047378541243613848, 0.7773170766911654539, 0.8047378541243613848, 0.7773170766911654539, 0.8047378541243613848, 0.7773170766911654539, 0.8047378541243613848, 0.7773170766911654539, 0.8047378541243613848, 0.7773170766911654539, 0.8047378541243613848, 0.7773170766911654539, 0.8047378541243613848, 0.7773170766911654539, 0.8047378541243613848, 0.7773170766911654539, 0.8047378541243613848, 0.7773170766911654539, 0.8047378541243613848, 0.7773170766911654539, 0.8047378541243613848, 0.7773170766911654539, 0.8047378541243613848, 0.7773170766911654539, 0.8047378541243613848, 0.7773170766911654539, 0.8047378541243613848, 0.7773170766911654539, 0.8047378541243613848, 0.7773170766911654539, 0.8047378541243613848, 0.7773170766911654539, 0.8047378541243613848, 0.7773170766911654539, 0.8047378541243613848, 0.7773170766911654539, 0.8047378541243613848, 0.7773170766911654539, 0.8047378541243613848, 0.7773170766911654539, 0.8047378541243613848, 0.7773170766911654539, 0.8047378541243613848, 0.7773170766911654539, 0.8047378541243613848, 0.7773170766911654539, 0.8047378541243613848, 0.7773170766911654539, 0.8047378541243613848, 0.7773170766911654539, 0.8047378541243613848, 0.7773170766911654539, 0.8047378541243613848, 0.7773170766911654539, 0.8047378541243613848, 0.7773170766911654539, 0.8047378541243613848, 0.7773170766911654539, 0.8047378541243613848, 0.7773170766911654539, 0.8047378541243613848, 0.7773170766911654539, 0.8047378541243613848, 0.7773170766911654539, 0.8047378541243613848, 0.7773170766911654539, 0.8047378541243613848, 0.7773170766911654539, 0.8047378541243613848, 0.7773170766911654539, 0.8047378541243613848, 0.7773170766911654539, 0.8047378541243613848, 0.7773170766911654539, 0.8047378541243613848, 0.7773170766911654539, 0.8047378541243613848, 0.7773170766911654539, 0.8047378541243613848, 0.7773170766911654539, 0.8047378541243613848, 0.7773170766911654539, 0.8047378541243613848, 0.7773170766911654539, 0.8047378541243613848, 0.7773170766911654539, 0.8047378541243613848, 0.7773170766911654539, 0.8047378541243613848, 0.7773170766911654539, 0.8047378541243613848, 0.7773170766911654539, 0.8047378541243613848, 0.7773170766911654539, 0.8047378541243613848, 0.7773170766911654539, 0.8047378541243613848, 0.7773170766911654539, 0.8047378541243613848, 0.7773170766911654539, 0.8047378541243613848, 0.7773170766911654539, 0.8047378541243613848, 0.7773170766911654539, 0.8047378541243613848, 0.7773170766911654539, 0.8047378541243613848, 0.7773170766911654539, 0.8047378541243613848, 0.7773170766911654539, 0.8047378541243613848, 0.7773170766911654539, 0.8047378541243613848, 0.7773170766911654539, 0.8047378541243613848, 0.7773170766911654539, 0.8047378541243613848, 0.7773170766911654539, 0.8047378541243613848, 0.7773170766911654539, 0.8047378541243613848, 0.7773170766911654539, 0.8047378541243613848, 0.7773170766911654539, 0.8047378541243613848, 0.7773170766911654539, 0.8047378541243613848, 0.7773170766911654539, 0.8047378541243613848, 0.7773170766911654539, 0.8047378541243613848, 0.7773170766911654539, 0.8047378541243613848, 0.7773170766911654539, 0.8047378541243613848, 0.7773170766911654539, 0.8047378541243613848, 0.7773170766911654539, 0.8047378541243613848, 0.7773170766911654539, 0.8047378541243613848, 0.7773170766911654539, 0.8047378541243613848, 0.7773170766911654539, 0.8047378541243613848, 0.7773170766911654539, 0.8047378541243613848, 0.7773170766911654539, 0.8047378541243613848, 0.7773170766911654539, 0.8047378541243613848, 0.7773170766911654539, 0.8047378541243613848, 0.7773170766911654539, 0.8047378541243613848, 0.7773170766911654539, 0.8047378541243613848, 0.7773170766911654539, 0.8047378541243613848),
 ( 0.8047378541243613848, 0.7773170766911654539, 0.8047378541243613848, 0.7773170766911654539, 0.8047378541243613848, 0.7773170766911654539, 0.8047378541243613848, 0.7773170766911654539, 0.8047378541243613848, 0.7773170766911654539, 0.8047378541243613848, 0.7773170766911654539, 0.8047378541243613848, 0.7773170766911654539, 0.8047378541243613848, 0.7773170766911654539, 0.8047378541243613848, 0.7773170766911654539, 0.8047378541243613848, 0.7773170766911654539, 0.8047378541243613848, 0.7773170766911654539, 0.8047378541243613848, 0.7773170766911654539, 0.8047378541243613848, 0.7773170766911654539, 0.8047378541243613848, 0.7773170766911654539, 0.8047378541243613848, 0.7773170766911654539, 0.8047378541243613848, 0.7773170766911654539, 0.8047378541243613848, 0.7773170766911654539, 0.8047378541243613848, 0.7773170766911654539, 0.8047378541243613848, 0.7773170766911654539, 0.8047378541243613848, 0.7773170766911654539, 0.8047378541243613848, 0.7773170766911654539, 0.8047378541243613848, 0.7773170766911654539, 0.8047378541243613848, 0.7773170766911654539, 0.8047378541243613848, 0.7773170766911654539, 0.8047378541243613848, 0.7773170766911654539, 0.8047378541243613848, 0.7773170766911654539, 0.8047378541243613848, 0.7773170766911654539, 0.8047378541243613848, 0.7773170766911654539, 0.8047378541243613848, 0.7773170766911654539, 0.8047378541243613848, 0.7773170766911654539, 0.8047378541243613848, 0.7773170766911654539, 0.8047378541243613848, 0.7773170766911654539, 0.8047378541243613848, 0.7773170766911654539, 0.8047378541243613848, 0.7773170766911654539, 0.8047378541243613848, 0.7773170766911654539, 0.8047378541243613848, 0.7773170766911654539, 0.8047378541243613848, 0.7773170766911654539, 0.8047378541243613848, 0.7773170766911654539, 0.8047378541243613848, 0.7773170766911654539, 0.8047378541243613848, 0.7773170766911654539, 0.8047378541243613848, 0.7773170766911654539, 0.8047378541243613848, 0.7773170766911654539, 0.8047378541243613848, 0.7773170766911654539, 0.8047378541243613848, 0.7773170766911654539, 0.8047378541243613848, 0.7773170766911654539, 0.8047378541243613848, 0.7773170766911654539, 0.8047378541243613848, 0.7773170766911654539, 0.8047378541243613848, 0.7773170766911654539, 0.8047378541243613848, 0.7773170766911654539, 0.8047378541243613848, 0.7773170766911654539, 0.8047378541243613848, 0.7773170766911654539, 0.8047378541243613848, 0.7773170766911654539, 0.8047378541243613848, 0.7773170766911654539, 0.8047378541243613848, 0.7773170766911654539, 0.8047378541243613848, 0.7773170766911654539, 0.8047378541243613848, 0.7773170766911654539, 0.8047378541243613848, 0.7773170766911654539, 0.8047378541243613848, 0.7773170766911654539, 0.8047378541243613848, 0.7773170766911654539, 0.8047378541243613848, 0.7773170766911654539, 0.8047378541243613848, 0.7773170766911654539, 0.8047378541243613848, 0.7773170766911654539, 0.8047378541243613848, 0.7773170766911654539, 0.8047378541243613848, 0.7773170766911654539, 0.8047378541243613848, 0.7773170766911654539, 0.8047378541243613848, 0.7773170766911654539, 0.8047378541243613848, 0.7773170766911654539, 0.8047378541243613848, 0.7773170766911654539, 0.8047378541243613848, 0.7773170766911654539, 0.8047378541243613848, 0.7773170766911654539, 0.8047378541243613848, 0.7773170766911654539, 0.8047378541243613848, 0.7773170766911654539, 0.8047378541243613848, 0.7773170766911654539, 0.8047378541243613848, 0.7773170766911654539, 0.8047378541243613848, 0.7773170766911654539, 0.8047378541243613848, 0.7773170766911654539, 0.8047378541243613848, 0.7773170766911654539, 0.8047378541243613848, 0.7773170766911654539, 0.8047378541243613848, 0.7773170766911654539, 0.8047378541243613848, 0.7773170766911654539, 0.8047378541243613848, 0.7773170766911654539, 0.8047378541243613848, 0.7773170766911654539, 0.8047378541243613848, 0.7773170766911654539, 0.8047378541243613848, 0.7773170766911654539, 0.8047378541243613848, 0.7773170766911654539, 0.8047378541243613848, 0.7773170766911654539, 0.8047378541243613848, 0.7773170766911654539, 0.8047378541243613848, 0.7773170766911654539, 0.8047378541243613848, 0.7773170766911654539, 0.8047378541243613848, 0.7773170766911654539, 0.8047378541243613848, 0.7773170766911654539, 0.8047378541243613848, 0.7773170766911654539, 0.8047378541243613848, 0.7773170766911654539, 0.8047378541243613848, 0.7773170766911654539, 0.8047378541243613848, 0.7773170766911654539, 0.8047378541243613848, 0.7773170766911654539, 0.8047378541243613848, 0.7773170766911654539, 0.8047378541243613848, 0.7773170766911654539, 0.8047378541243613848, 0.7773170766911654539, 0.8047378541243613848, 0.7773170766911654539, 0.8047378541243613848, 0.7773170766911654539, 0.8047378541243613848, 0.7773170766911654539, 0.8047378541243613848, 0.7773170766911654539, 0.8047378541243613848, 0.7773170766911654539, 0.8047378541243613848, 0.7773170766911654539, 0.8047378541243613848, 0.7773170766911654539, 0.8047378541243613848, 0.7773170766911654539, 0.8047378541243613848, 0.7773170766911654539, 0.8047378541243613848, 0.7773170766911654539, 0.8047378541243613848, 0.7773170766911654539, 0.8047378541243613848, 0.7773170766911654539, 0.8047378541243613848, 0.7773170766911654539, 0.8047378541243613848, 0.7773170766911654539, 0.8047378541243613848, 0.7773170766911654539, 0.8047378541243613848, 0.7773170766911654539, 0.8047378541243613848, 0.7773170766911654539, 0.8047378541243613848, 0.7773170766911654539, 0.8047378541243613848, 0.7773170766911654539, 0.8047378541243613848, 0.7773170766911654539, 0.8047378541243613848, 0.7773170766911654539, 0.8047378541243613848, 0.7773170766911654539, 0.8047378541243613848, 0.7773170766911654539, 0.8047378541243613848, 0.7773170766911654539, 0.8047378541243613848, 0.7773170766911654539, 0.8047378541243613848, 0.7773170766911654539, 0.8047378541243613848, 0.7773170766911654539, 0.8047378541243613848, 0.7773170766911654539, 0.8047378541243613848, 0.7773170766911654539, 0.8047378541243613848, 0.7773170766911654539, 0.8047378541243613848, 0.7773170766911654539, 0.8047378541243613848, 0.7773170766911654539, 0.8047378541243613848, 0.7773170766911654539, 0.8047378541243613848, 0.7773170766911654539, 0.8047378541243613848, 0.7773170766911654539, 0.8047378541243613848, 0.7773170766911654539, 0.8047378541243613848, 0.7773170766911654539, 0.8047378541243613848, 0.7773170766911654539, 0.8047378541243613848, 0.7773170766911654539, 0.8047378541243613848, 0.7773170766911654539, 0.8047378541243613848, 0.7773170766911654539, 0.8047378541243613848, 0.7773170766911654539, 0.8047378541243613848, 0.7773170766911654539, 0.8047378541243613848, 0.7773170766911654539, 0.8047378541243613848, 0.7773170766911654539, 0.8047378541243613848, 0.7773170766911654539, 0.8047378541243613848, 0.7773170766911654539, 0.8047378541243613848, 0.7773170766911654539, 0.8047378541243613848, 0.7773170766911654539, 0.8047378541243613848, 0.7773170766911654539, 0.8047378541243613848, 0.7773170766911654539, 0.8047378541243613848, 0.7773170766911654539, 0.8047378541243613848, 0.7773170766911654539, 0.8047378541243613848, 0.7773170766911654539, 0.8047378541243613848, 0.7773170766911654539, 0.8047378541243613848, 0.7773170766911654539, 0.8047378541243613848, 0.7773170766911654539, 0.8047378541243613848, 0.7773170766911654539, 0.8047378541243613848, 0.7773170766911654539, 0.8047378541243613848, 0.7773170766911654539, 0.8047378541243613848, 0.7773170766911654539, 0.8047378541243613848, 0.7773170766911654539, 0.8047378541243613848, 0.7773170766911654539, 0.8047378541243613848, 0.7773170766911654539, 0.8047378541243613848, 0.7773170766911654539, 0.8047378541243613848, 0.7773170766911654539, 0.8047378541243613848, 0.7773170766911654539, 0.8047378541243613848, 0.7773170766911654539, 0.8047378541243613848, 0.7773170766911654539, 0.8047378541243613848, 0.7773170766911654539, 0.8047378541243613848, 0.7773170766911654539, 0.8047378541243613848, 0.7773170766911654539, 0.8047378541243613848, 0.7773170766911654539, 0.8047378541243613848, 0.7773170766911654539, 0.8047378541243613848, 0.7773170766911654539, 0.8047378541243613848, 0.7773170766911654539, 0.8047378541243613848, 0.7773170766911654539, 0.8047378541243613848, 0.7773170766911654539, 0.8047378541243613848, 0.7773170766911654539, 0.8047378541243613848, 0.7773170766911654539, 0.8047378541243613848, 0.7773170766911654539, 0.8047378541243613848, 0.7773170766911654539, 0.8047378541243613848, 0.7773170766911654539, 0.8047378541243613848, 0.7773170766911654539, 0.8047378541243613848, 0.7773170766911654539, 0.8047378541243613848, 0.7773170766911654539, 0.8047378541243613848, 0.7773170766911654539, 0.8047378541243613848, 0.7773170766911654539, 0.8047378541243613848, 0.7773170766911654539, 0.8047378541243613848, 0.7773170766911654539, 0.8047378541243613848, 0.7773170766911654539, 0.8047378541243613848, 0.7773170766911654539, 0.8047378541243613848, 0.7773170766911654539, 0.8047378541243613848, 0.7773170766911654539, 0.8047378541243613848, 0.7773170766911654539, 0.8047378541243613848, 0.7773170766911654539, 0.8047378541243613848, 0.7773170766911654539, 0.8047378541243613848, 0.7773170766911654539, 0.8047378541243613848, 0.7773170766911654539, 0.8047378541243613848, 0.7773170766911654539, 0.8047378541243613848, 0.7773170766911654539, 0.8047378541243613848, 0.7773170766911654539, 0.8047378541243613848, 0.7773170766911654539, 0.8047378541243613848, 0.7773170766911654539, 0.8047378541243613848, 0.7773170766911654539, 0.8047378541243613848, 0.7773170766911654539, 0.8047378541243613848, 0.7773170766911654539, 0.8047378541243613848, 0.7773170766911654539, 0.8047378541243613848, 0.7773170766911654539, 0.8047378541243613848, 0.7773170766911654539, 0.8047378541243613848, 0.7773170766911654539, 0.8047378541243613848, 0.7773170766911654539, 0.8047378541243613848, 0.7773170766911654539, 0.8047378541243613848, 0.7773170766911654539, 0.8047378541243613848, 0.7773170766911654539, 0.8047378541243613848, 0.7773170766911654539, 0.8047378541243613848, 0.7773170766911654539, 0.8047378541243613848, 0.7773170766911654539, 0.8047378541243613848, 0.7773170766911654539, 0.8047378541243613848, 0.7773170766911654539, 0.8047378541243613848, 0.7773170766911654539, 0.8047378541243613848, 0.7773170766911654539, 0.8047378541243613848, 0.7773170766911654539, 0.8047378541243613848, 0.7773170766911654539, 0.8047378541243613848, 0.7773170766911654539, 0.8047378541243613848, 0.7773170766911654539, 0.8047378541243613848, 0.7773170766911654539, 0.8047378541243613848, 0.7773170766911654539, 0.8047378541243613848, 0.7773170766911654539, 0.8047378541243613848, 0.7773170766911654539, 0.8047378541243613848, 0.7773170766911654539, 0.8047378541243613848, 0.7773170766911654539, 0.8047378541243613848, 0.7773170766911654539, 0.8047378541243613848, 0.7773170766911654539, 0.8047378541243613848, 0.7773170766911654539, 0.8047378541243613848, 0.7773170766911654539, 0.8047378541243613848, 0.7773170766911654539, 0.8047378541243613848, 0.7773170766911654539, 0.8047378541243613848),
 ( 1.000000000000000000, 0.9659258262890683122, 1.000000000000000000, 0.9659258262890683122, 1.000000000000000000, 0.9659258262890683122, 1.000000000000000000, 0.9659258262890683122, 1.000000000000000000, 0.9659258262890683122, 1.000000000000000000, 0.9659258262890683122, 1.000000000000000000, 0.9659258262890683122, 1.000000000000000000, 0.9659258262890683122, 1.000000000000000000, 0.9659258262890683122, 1.000000000000000000, 0.9659258262890683122, 1.000000000000000000, 0.9659258262890683122, 1.000000000000000000, 0.9659258262890683122, 1.000000000000000000, 0.9659258262890683122, 1.000000000000000000, 0.9659258262890683122, 1.000000000000000000, 0.9659258262890683122, 1.000000000000000000, 0.9659258262890683122, 1.000000000000000000, 0.9659258262890683122, 1.000000000000000000, 0.9659258262890683122, 1.000000000000000000, 0.9659258262890683122, 1.000000000000000000, 0.9659258262890683122, 1.000000000000000000, 0.9659258262890683122, 1.000000000000000000, 0.9659258262890683122, 1.000000000000000000, 0.9659258262890683122, 1.000000000000000000, 0.9659258262890683122, 1.000000000000000000, 0.9659258262890683122, 1.000000000000000000, 0.9659258262890683122, 1.000000000000000000, 0.9659258262890683122, 1.000000000000000000, 0.9659258262890683122, 1.000000000000000000, 0.9659258262890683122, 1.000000000000000000, 0.9659258262890683122, 1.000000000000000000, 0.9659258262890683122, 1.000000000000000000, 0.9659258262890683122, 1.000000000000000000, 0.9659258262890683122, 1.000000000000000000, 0.9659258262890683122, 1.000000000000000000, 0.9659258262890683122, 1.000000000000000000, 0.9659258262890683122, 1.000000000000000000, 0.9659258262890683122, 1.000000000000000000, 0.9659258262890683122, 1.000000000000000000, 0.9659258262890683122, 1.000000000000000000, 0.9659258262890683122, 1.000000000000000000, 0.9659258262890683122, 1.000000000000000000, 0.9659258262890683122, 1.000000000000000000, 0.9659258262890683122, 1.000000000000000000, 0.9659258262890683122, 1.000000000000000000, 0.9659258262890683122, 1.000000000000000000, 0.9659258262890683122, 1.000000000000000000, 0.9659258262890683122, 1.000000000000000000, 0.9659258262890683122, 1.000000000000000000, 0.9659258262890683122, 1.000000000000000000, 0.9659258262890683122, 1.000000000000000000, 0.9659258262890683122, 1.000000000000000000, 0.9659258262890683122, 1.000000000000000000, 0.9659258262890683122, 1.000000000000000000, 0.9659258262890683122, 1.000000000000000000, 0.9659258262890683122, 1.000000000000000000, 0.9659258262890683122, 1.000000000000000000, 0.9659258262890683122, 1.000000000000000000, 0.9659258262890683122, 1.000000000000000000, 0.9659258262890683122, 1.000000000000000000, 0.9659258262890683122, 1.000000000000000000, 0.9659258262890683122, 1.000000000000000000, 0.9659258262890683122, 1.000000000000000000, 0.9659258262890683122, 1.000000000000000000, 0.9659258262890683122, 1.000000000000000000, 0.9659258262890683122, 1.000000000000000000, 0.9659258262890683122, 1.000000000000000000, 0.9659258262890683122, 1.000000000000000000, 0.9659258262890683122, 1.000000000000000000, 0.9659258262890683122, 1.000000000000000000, 0.9659258262890683122, 1.000000000000000000, 0.9659258262890683122, 1.000000000000000000, 0.9659258262890683122, 1.000000000000000000, 0.9659258262890683122, 1.000000000000000000, 0.9659258262890683122, 1.000000000000000000, 0.9659258262890683122, 1.000000000000000000, 0.9659258262890683122, 1.000000000000000000, 0.9659258262890683122, 1.000000000000000000, 0.9659258262890683122, 1.000000000000000000, 0.9659258262890683122, 1.000000000000000000, 0.9659258262890683122, 1.000000000000000000, 0.9659258262890683122, 1.000000000000000000, 0.9659258262890683122, 1.000000000000000000, 0.9659258262890683122, 1.000000000000000000, 0.9659258262890683122, 1.000000000000000000, 0.9659258262890683122, 1.000000000000000000, 0.9659258262890683122, 1.000000000000000000, 0.9659258262890683122, 1.000000000000000000, 0.9659258262890683122, 1.000000000000000000, 0.9659258262890683122, 1.000000000000000000, 0.9659258262890683122, 1.000000000000000000, 0.9659258262890683122, 1.000000000000000000, 0.9659258262890683122, 1.000000000000000000, 0.9659258262890683122, 1.000000000000000000, 0.9659258262890683122, 1.000000000000000000, 0.9659258262890683122, 1.000000000000000000, 0.9659258262890683122, 1.000000000000000000, 0.9659258262890683122, 1.000000000000000000, 0.9659258262890683122, 1.000000000000000000, 0.9659258262890683122, 1.000000000000000000, 0.9659258262890683122, 1.000000000000000000, 0.9659258262890683122, 1.000000000000000000, 0.9659258262890683122, 1.000000000000000000, 0.9659258262890683122, 1.000000000000000000, 0.9659258262890683122, 1.000000000000000000, 0.9659258262890683122, 1.000000000000000000, 0.9659258262890683122, 1.000000000000000000, 0.9659258262890683122, 1.000000000000000000, 0.9659258262890683122, 1.000000000000000000, 0.9659258262890683122, 1.000000000000000000, 0.9659258262890683122, 1.000000000000000000, 0.9659258262890683122, 1.000000000000000000, 0.9659258262890683122, 1.000000000000000000, 0.9659258262890683122, 1.000000000000000000, 0.9659258262890683122, 1.000000000000000000, 0.9659258262890683122, 1.000000000000000000, 0.9659258262890683122, 1.000000000000000000, 0.9659258262890683122, 1.000000000000000000, 0.9659258262890683122, 1.000000000000000000, 0.9659258262890683122, 1.000000000000000000, 0.9659258262890683122, 1.000000000000000000, 0.9659258262890683122, 1.000000000000000000, 0.9659258262890683122, 1.000000000000000000, 0.9659258262890683122, 1.000000000000000000, 0.9659258262890683122, 1.000000000000000000, 0.9659258262890683122, 1.000000000000000000, 0.9659258262890683122, 1.000000000000000000, 0.9659258262890683122, 1.000000000000000000, 0.9659258262890683122, 1.000000000000000000, 0.9659258262890683122, 1.000000000000000000, 0.9659258262890683122, 1.000000000000000000, 0.9659258262890683122, 1.000000000000000000, 0.9659258262890683122, 1.000000000000000000, 0.9659258262890683122, 1.000000000000000000, 0.9659258262890683122, 1.000000000000000000, 0.9659258262890683122, 1.000000000000000000, 0.9659258262890683122, 1.000000000000000000, 0.9659258262890683122, 1.000000000000000000, 0.9659258262890683122, 1.000000000000000000, 0.9659258262890683122, 1.000000000000000000, 0.9659258262890683122, 1.000000000000000000, 0.9659258262890683122, 1.000000000000000000, 0.9659258262890683122, 1.000000000000000000, 0.9659258262890683122, 1.000000000000000000, 0.9659258262890683122, 1.000000000000000000, 0.9659258262890683122, 1.000000000000000000, 0.9659258262890683122, 1.000000000000000000, 0.9659258262890683122, 1.000000000000000000, 0.9659258262890683122, 1.000000000000000000, 0.9659258262890683122, 1.000000000000000000, 0.9659258262890683122, 1.000000000000000000, 0.9659258262890683122, 1.000000000000000000, 0.9659258262890683122, 1.000000000000000000, 0.9659258262890683122, 1.000000000000000000, 0.9659258262890683122, 1.000000000000000000, 0.9659258262890683122, 1.000000000000000000, 0.9659258262890683122, 1.000000000000000000, 0.9659258262890683122, 1.000000000000000000, 0.9659258262890683122, 1.000000000000000000, 0.9659258262890683122, 1.000000000000000000, 0.9659258262890683122, 1.000000000000000000, 0.9659258262890683122, 1.000000000000000000, 0.9659258262890683122, 1.000000000000000000, 0.9659258262890683122, 1.000000000000000000, 0.9659258262890683122, 1.000000000000000000, 0.9659258262890683122, 1.000000000000000000, 0.9659258262890683122, 1.000000000000000000, 0.9659258262890683122, 1.000000000000000000, 0.9659258262890683122, 1.000000000000000000, 0.9659258262890683122, 1.000000000000000000, 0.9659258262890683122, 1.000000000000000000, 0.9659258262890683122, 1.000000000000000000, 0.9659258262890683122, 1.000000000000000000, 0.9659258262890683122, 1.000000000000000000, 0.9659258262890683122, 1.000000000000000000, 0.9659258262890683122, 1.000000000000000000, 0.9659258262890683122, 1.000000000000000000, 0.9659258262890683122, 1.000000000000000000, 0.9659258262890683122, 1.000000000000000000, 0.9659258262890683122, 1.000000000000000000, 0.9659258262890683122, 1.000000000000000000, 0.9659258262890683122, 1.000000000000000000, 0.9659258262890683122, 1.000000000000000000, 0.9659258262890683122, 1.000000000000000000, 0.9659258262890683122, 1.000000000000000000, 0.9659258262890683122, 1.000000000000000000, 0.9659258262890683122, 1.000000000000000000, 0.9659258262890683122, 1.000000000000000000, 0.9659258262890683122, 1.000000000000000000, 0.9659258262890683122, 1.000000000000000000, 0.9659258262890683122, 1.000000000000000000, 0.9659258262890683122, 1.000000000000000000, 0.9659258262890683122, 1.000000000000000000, 0.9659258262890683122, 1.000000000000000000, 0.9659258262890683122, 1.000000000000000000, 0.9659258262890683122, 1.000000000000000000, 0.9659258262890683122, 1.000000000000000000, 0.9659258262890683122, 1.000000000000000000, 0.9659258262890683122, 1.000000000000000000, 0.9659258262890683122, 1.000000000000000000, 0.9659258262890683122, 1.000000000000000000, 0.9659258262890683122, 1.000000000000000000, 0.9659258262890683122, 1.000000000000000000, 0.9659258262890683122, 1.000000000000000000, 0.9659258262890683122, 1.000000000000000000, 0.9659258262890683122, 1.000000000000000000, 0.9659258262890683122, 1.000000000000000000, 0.9659258262890683122, 1.000000000000000000, 0.9659258262890683122, 1.000000000000000000, 0.9659258262890683122, 1.000000000000000000, 0.9659258262890683122, 1.000000000000000000, 0.9659258262890683122, 1.000000000000000000, 0.9659258262890683122, 1.000000000000000000, 0.9659258262890683122, 1.000000000000000000, 0.9659258262890683122, 1.000000000000000000, 0.9659258262890683122, 1.000000000000000000, 0.9659258262890683122, 1.000000000000000000, 0.9659258262890683122, 1.000000000000000000, 0.9659258262890683122, 1.000000000000000000, 0.9659258262890683122, 1.000000000000000000, 0.9659258262890683122, 1.000000000000000000, 0.9659258262890683122, 1.000000000000000000, 0.9659258262890683122, 1.000000000000000000, 0.9659258262890683122, 1.000000000000000000, 0.9659258262890683122, 1.000000000000000000, 0.9659258262890683122, 1.000000000000000000, 0.9659258262890683122, 1.000000000000000000, 0.9659258262890683122, 1.000000000000000000, 0.9659258262890683122, 1.000000000000000000, 0.9659258262890683122, 1.000000000000000000, 0.9659258262890683122, 1.000000000000000000, 0.9659258262890683122, 1.000000000000000000, 0.9659258262890683122, 1.000000000000000000, 0.9659258262890683122, 1.000000000000000000, 0.9659258262890683122, 1.000000000000000000, 0.9659258262890683122, 1.000000000000000000, 0.9659258262890683122, 1.000000000000000000, 0.9659258262890683122, 1.000000000000000000) ) ) 
 REPRESENTATION_ITEM ( '' )  SURFACE ( )  );
#17582=CARTESIAN_POINT ( 'NONE',  ( 0.1958661417322836718, -0.3392501089628017219, -0.7185232527897132959 ) ) ;
#17594=CARTESIAN_POINT ( 'NONE',  ( 0.1958661417322836440, -0.3392501089628017219, -1.186351706036745446 ) ) ;
#17597=CARTESIAN_POINT ( 'NONE',  ( 0.1058382717557500713, -0.3949938075777409408, -1.660104986876640654 ) ) ;
#17609=CARTESIAN_POINT ( 'NONE',  ( -0.3917322834645670104, -7.196005306013484475E-17, 0.1909448818897636901 ) ) ;
#17615=CARTESIAN_POINT ( 'NONE',  ( 0.1070741851644054915, -0.3996062992125986035, -1.975065616797900381 ) ) ;
#17618=CARTESIAN_POINT ( 'NONE',  ( 0.3996062992125984925, 0.1070741851644054637, -1.461286089238844843 ) ) ;
#17622=CARTESIAN_POINT ( 'NONE',  ( -0.1265901696524986964, -0.4724409448818899238, -0.2296587926509186250 ) ) ;
#17624=CARTESIAN_POINT ( 'NONE',  ( -0.3392501089628017219, -0.1958661417322836718, 0.1128608923884514836 ) ) ;
#17630=CARTESIAN_POINT ( 'NONE',  ( 0.1265901696524989462, 0.4724409448818897572, -2.432414698162729039 ) ) ;
#17632=CARTESIAN_POINT ( 'NONE',  ( 0.3420746716998660508, -0.1974969037888704149, -2.229002624671915900 ) ) ;
#17639=CARTESIAN_POINT ( 'NONE',  ( -0.4091458600556402980, -0.2362204724409451284, -2.176509186351706315 ) ) ;
#17644=CARTESIAN_POINT ( 'NONE',  ( 0.4724409448818898682, 2.892866454678787531E-17, -0.9822834645669291653 ) ) ;
#17646=CYLINDRICAL_SURFACE ( 'NONE', #18304, 0.4724409448818898682 ) ;
#17655=CARTESIAN_POINT ( 'NONE',  ( -0.3460692066303957537, -0.1998031496062994405, -0.6017060367454067915 ) ) ;
#17657=CARTESIAN_POINT ( 'NONE',  ( -0.3392501089628019995, 0.1958661417322832277, -2.158136482939632561 ) ) ;
#17672=CARTESIAN_POINT ( 'NONE',  ( 0.1049643490035304938, -0.3917322834645669549, -1.429790026246719359 ) ) ;
#17673=CARTESIAN_POINT ( 'NONE',  ( -0.2143816077119332086, 0.3285422586334138528, -1.220472440944882386 ) ) ;
#17678=CARTESIAN_POINT ( 'NONE',  ( -0.1998031496062994405, 0.3460692066303957537, -2.452099737532808188 ) ) ;
#17680=CARTESIAN_POINT ( 'NONE',  ( 0.3460692066303959757, -0.1998031496062991907, -0.8923884514435694859 ) ) ;
#17683=CARTESIAN_POINT ( 'NONE',  ( -0.3392501089628017219, -0.1958661417322836718, -2.564304461942256808 ) ) ;
#17696=CARTESIAN_POINT ( 'NONE',  ( 4.797336870675656522E-17, -0.3917322834645670104, -2.683070866141731958 ) ) ;
#17699=CARTESIAN_POINT ( 'NONE',  ( -0.3949938075777409408, -0.1058382717557502933, -0.2034120734908137218 ) ) ;
#17707=CARTESIAN_POINT ( 'NONE',  ( -0.3917322834645670659, -7.196005306013484475E-17, -1.295951074312022833 ) ) ;
#17709=CARTESIAN_POINT ( 'NONE',  ( 0.2867679344610365999, -0.2867679344610365444, -2.702755905511810663 ) ) ;
#17714=CARTESIAN_POINT ( 'NONE',  ( -0.3996062992125986035, -0.1070741851644056997, -0.8333333333333332593 ) ) ;
#17716=CARTESIAN_POINT ( 'NONE',  ( 0.2925321140481932369, 0.2925321140481932369, -0.3720472440944882497 ) ) ;
#17718=CARTESIAN_POINT ( 'NONE',  ( 0.3460692066303959757, -0.1998031496062991907, -2.309711286089239035 ) ) ;
#17719=( BOUNDED_SURFACE ( )  B_SPLINE_SURFACE ( 1, 2, ( 
 ( #82402, #69355, #81588, #49155, #74861, #11287, #17609, #12518, #50799, #38179, #37364, #56299, #68529, #81996, #18828, #75266, #56703, #49570, #11709, #76500, #76086, #17203, #70165, #5778, #57111, #62206, #62624, #44474, #10870, #36947, #12109, #69764, #31035, #37767, #4136, #5374, #24720, #23905, #24310, #29801, #4543, #4967, #63036, #42836, #44072, #82805, #30634, #30214, #55462, #68938, #31447, #49980, #36530, #25129, #81171, #23489, #55876, #75678, #18018, #43653, #58365, #77324, #13775, #71428, #77749, #25961, #39007, #51207, #78592, #19653, #58795, #45315, #6191, #39432, #14617, #14200, #20082, #71010, #57529, #13354, #78170, #7030, #46571, #65548, #64274, #20917, #45732, #1153, #6609, #31869, #70584, #51619, #46155, #71850, #27220, #25541, #64691, #32699, #44884, #39857, #26804, #12938, #72269, #7879, #19234, #728, #33543, #59205, #83220, #52044, #76904, #65118, #32280, #1566, #26386, #38596, #57940, #7455, #33125, #306, #52462, #20501, #52881, #63854, #27638, #61175, #81801, #16584, #68742, #4755, #67505, #42643, #16167, #1974, #72678, #4346, #74240, #36335, #55265, #53300, #42229, #40271, #62009, #8290, #30431, #65954, #75481, #36741, #35932, #30013, #79012, #11084, #61599, #62417, #80975, #23288, #56096, #9840, #46984, #33958, #59620, #21332, #74659, #55676, #17416, #41813, #81385, #48958, #35511, #67924, #24112, #17003, #10679, #3945, #49781, #3529, #29195, #54862, #80567, #22878, #48540, #68340, #10264, #23701, #29604, #49372, #75068, #43046, #69968, #12322, #19455, #50191, #56915, #63243, #37980, #25758, #12735, #45106, #37160, #11504, #30840, #5583, #64074, #24525, #76305, #51420, #69567, #18634, #31249, #82611, #31665, #44278, #50597, #5994, #69153, #57326, #19037, #57742, #24928, #6411, #104, #77122, #32081, #83020, #63655, #18229, #62842, #5176, #25343, #37569, #17822, #43455, #56505, #44684, #51005, #76704, #70380, #82207, #38394, #75888, #43868, #11915, #56362, #81655, #80423, #75740, #69001, #62688, #67779, #68194, #82061, #74093, #16855, #17672, #75326, #36590, #43303, #43716, #10933, #62268, #29459, #42898, #23966, #16439, #11352, #55526, #55940, #4605, #42084, #35779, #55117, #49633, #10117, #68592, #37010, #5030, #30698, #61448, #80826, #30277, #24374, #50045, #35368, #18081, #9698, #3795, #22734, #36187, #42490, #10532, #61033, #3383, #49219, #74925, #17270, #23551, #23140, #61859, #48393, #29045, #48809, #54716, #74508, #4200, #29864, #81235, #19722, #83284, #76562, #63099, #18890, #373, #12585, #52108, #71077, #69826, #795, #51270, #64338, #12175, #11773, #76151, #31516, #51688, #77391, #32766, #31099, #57174, #44539, #50449, #45380, #6675, #18491, #77816, #13419, #24781, #70230, #39076, #64757, #5438, #57594, #56766, #25607, #37833, #7096, #50862, #44134, #63511, #76972, #44954, #5841, #82872, #25196, #58433, #26456, #82465, #38243, #20147, #63920, #69418, #37426, #6255, #70650, #31932, #19302, #13005, #32347, #38661, #58008, #26028, #33194, #78657, #45796, #66430, #13842, #9185, #71494, #79903, #41163, #40338, #8765, #1219, #15505, #66018, #66853, #2038, #59682, #34857, #71916, #52529, #39500, #65188, #7524, #79077, #34440, #21799, #26868, #8354, #60519, #46220, #20978, #21393, #78236, #60107, #2868, #46638, #20569, #58862, #27283, #28118, #65614, #14266, #40746, #28531, #2460, #47049, #27703, #59269, #39925, #34022, #1626, #72741, #54188, #53367, #53773, #7945, #33606, #15088, #52943, #79485, #47463, #72333, #14681, #73155, #11794, #3821, #50067, #48833, #49245, #63121, #55141, #81259, #82083, #56384, #17696, #24397, #24804, #75348, #43324, #10555, #23990, #5052, #80852, #75762, #36614, #37032, #69024, #23164, #16880, #36213, #62714, #74534, #49658, #30722, #43737, #18104, #42518, #61882, #11375, #69442, #37447, #16463, #5459, #74117, #68221 ),
 ( #55966, #31121, #4223, #42108, #29887, #55550, #56788, #82488, #67805, #35807, #23574, #74948, #17294, #10142, #61473, #42921, #29482, #68616, #10956, #62292, #4629, #30300, #81679, #38684, #69847, #64362, #18912, #58458, #31956, #25217, #5863, #6699, #26053, #50883, #70253, #76583, #39521, #20167, #37856, #12608, #7546, #25630, #77838, #13862, #44562, #51712, #38266, #12198, #82897, #13442, #83308, #45403, #32368, #63532, #51293, #50471, #71099, #18512, #65209, #76175, #1241, #63943, #58032, #395, #58882, #6280, #76996, #57617, #77413, #33219, #818, #44155, #31539, #57195, #19327, #44979, #52131, #70675, #13031, #19749, #39098, #64780, #7118, #32789, #26480, #45817, #71516, #2481, #20589, #79508, #66877, #47898, #66039, #79928, #73606, #67284, #28556, #21824, #8788, #21000, #71937, #14286, #34042, #40359, #35288, #15948, #60950, #60130, #79098, #7966, #21417, #41594, #14704, #47487, #72356, #34461, #9617, #15529, #28140, #26890, #39950, #2892, #1649, #2060, #52549, #33629, #59705, #34880, #9207, #53796, #60541, #78258, #73179, #41187, #46662, #54212, #22243, #59292, #46241, #72762, #65636, #27306, #52965, #78679, #8377, #27724, #53391, #47071, #15113, #40767, #66452, #35697, #48729, #81571, #68923, #81981, #28965, #11272, #3300, #55040, #16358, #29787, #36110, #61782, #4949, #24295, #42822, #68515, #49556, #10856, #3716, #4122, #56284, #17189, #55861, #23473, #43637, #54629, #49965, #75663, #69340, #16773, #74011, #36516, #67697, #36931, #18003, #11691, #37348, #62192, #4529, #74426, #55448, #42003, #80342, #42411, #23890, #68108, #22655, #30199, #48314, #62609, #75250, #10456, #10033, #81157, #17594, #49140, #61364, #30619, #29380, #80747, #43226, #23061, #74845, #5359, #69748, #25112, #45299, #70995, #26369, #24705, #50784, #38164, #44056, #13338, #290, #12094, #45716, #38992, #18413, #12503, #64675, #32682, #56688, #51191, #82387, #76889, #31432, #7014, #44459, #37752, #63427, #19219, #38581, #5763, #82790, #57095, #52027, #58349, #50373, #76485, #20064, #63838, #710, #77733, #18812, #64260, #70150, #76071, #6176, #25946, #31851, #57926, #44869, #57513, #83204, #63021, #51604, #31020, #71413, #25526, #13760, #70568, #12922, #77309, #6594, #32266, #19639, #9112, #78996, #53285, #34784, #65530, #33109, #66778, #46555, #41089, #72663, #60027, #15429, #20485, #59605, #2795, #39841, #72253, #15012, #78154, #53697, #60443, #14602, #14183, #39417, #20902, #21725, #59190, #46139, #34361, #28454, #79406, #40668, #21316, #52866, #7863, #33941, #78576, #66353, #73079, #46969, #40256, #58777, #65939, #47388, #8275, #22146, #54114, #33527, #79829, #8691, #2382, #1549, #65101, #71834, #27203, #47804, #73507, #7438, #1137, #1960, #27622, #28039, #26787, #52444, #22563, #81890, #49465, #54531, #48635, #75159, #68833, #9520, #4031, #35192, #29696, #67601, #23793, #80657, #73920, #80247, #55358, #74746, #16261, #35604, #41907, #4850, #11179, #3207, #61266, #56188, #74330, #43136, #62512, #9932, #17095, #3620, #60853, #48224, #62099, #16677, #10766, #81064, #28869, #42316, #15855, #36426, #67189, #30525, #41504, #49872, #36839, #10359, #4441, #29287, #24201, #36019, #54950, #23380, #49048, #22969, #68015, #61691, #42730, #68426, #17504, #30107, #55769, #81476, #56595, #12410, #38900, #75979, #25018, #25431, #30928, #6502, #45199, #50691, #50281, #75572, #57003, #57828, #12001, #82295, #70471, #70901, #32172, #51097, #57419, #5670, #18319, #70056, #31337, #76794, #83112, #6083, #37655, #76389, #62931, #6917, #82699, #12828, #18722, #17912, #19125, #26272, #38485, #44774, #69657, #37255, #5264, #44364, #38068, #616, #64579, #43548, #64169, #63744, #24614, #31757, #32588, #63333, #196, #25848, #51508, #58251, #77212, #19541, #13251, #43961, #69248, #11595, #28259, #42127, #34166, #60253 ) ),
 .UNSPECIFIED., .F., .F., .F. ) 
 B_SPLINE_SURFACE_WITH_KNOTS ( ( 2, 2 ),
 ( 3, 2, 2, 2, 2, 2, 2, 2, 2, 2, 2, 2, 2, 2, 2, 2, 2, 2, 2, 2, 2, 2, 2, 2, 2, 2, 2, 2, 2, 2, 2, 2, 2, 2, 2, 2, 2, 2, 2, 2, 2, 2, 2, 2, 2, 2, 2, 2, 2, 2, 2, 2, 2, 2, 2, 2, 2, 2, 2, 2, 2, 2, 2, 2, 2, 2, 2, 2, 2, 2, 2, 2, 2, 2, 2, 2, 2, 2, 2, 2, 2, 2, 2, 2, 2, 2, 2, 2, 2, 2, 2, 2, 2, 2, 2, 2, 2, 2, 2, 2, 2, 2, 2, 2, 2, 2, 2, 2, 2, 2, 2, 2, 2, 2, 2, 2, 2, 2, 2, 2, 2, 2, 2, 2, 2, 2, 2, 2, 2, 2, 2, 2, 2, 2, 2, 2, 2, 2, 2, 2, 2, 2, 2, 2, 2, 2, 2, 2, 2, 2, 2, 2, 2, 2, 2, 2, 2, 2, 2, 2, 2, 2, 2, 2, 2, 2, 2, 2, 2, 2, 2, 2, 2, 2, 2, 2, 2, 2, 2, 2, 2, 2, 2, 2, 2, 2, 2, 2, 2, 2, 2, 2, 2, 2, 2, 2, 2, 2, 2, 2, 2, 2, 2, 2, 2, 2, 2, 2, 2, 2, 2, 2, 2, 2, 2, 2, 2, 2, 2, 2, 2, 2, 2, 2, 2, 2, 2, 2, 2, 2, 2, 2, 2, 2, 2, 2, 2, 3 ),
 ( 0.000000000000000000, 1.000000000000000000 ),
 ( 0.000000000000000000, 0.004166666666666666609, 0.008333333333333333218, 0.01250000000000000069, 0.01666666666666666644, 0.02083333333333333218, 0.02500000000000000139, 0.02916666666666666713, 0.03333333333333333287, 0.03749999999999999861, 0.04166666666666666435, 0.04583333333333333010, 0.05000000000000000278, 0.05416666666666666852, 0.05833333333333333426, 0.06250000000000000000, 0.06666666666666666574, 0.07083333333333333148, 0.07499999999999999722, 0.07916666666666666297, 0.08333333333333332871, 0.08749999999999999445, 0.09166666666666666019, 0.09583333333333333981, 0.1000000000000000056, 0.1041666666666666713, 0.1083333333333333370, 0.1125000000000000028, 0.1166666666666666685, 0.1208333333333333343, 0.1250000000000000000, 0.1291666666666666796, 0.1333333333333333315, 0.1375000000000000111, 0.1416666666666666630, 0.1458333333333333426, 0.1499999999999999944, 0.1541666666666666741, 0.1583333333333333259, 0.1625000000000000056, 0.1666666666666666574, 0.1708333333333333370, 0.1749999999999999889, 0.1791666666666666685, 0.1833333333333333204, 0.1875000000000000000, 0.1916666666666666796, 0.1958333333333333315, 0.2000000000000000111, 0.2041666666666666630, 0.2083333333333333426, 0.2124999999999999944, 0.2166666666666666741, 0.2208333333333333259, 0.2250000000000000056, 0.2291666666666666574, 0.2333333333333333370, 0.2374999999999999889, 0.2416666666666666685, 0.2458333333333333204, 0.2500000000000000000, 0.2541666666666666519, 0.2583333333333333592, 0.2625000000000000111, 0.2666666666666666630, 0.2708333333333333148, 0.2750000000000000222, 0.2791666666666666741, 0.2833333333333333259, 0.2874999999999999778, 0.2916666666666666852, 0.2958333333333333370, 0.2999999999999999889, 0.3041666666666666408, 0.3083333333333333481, 0.3125000000000000000, 0.3166666666666666519, 0.3208333333333333592, 0.3250000000000000111, 0.3291666666666666630, 0.3333333333333333148, 0.3375000000000000222, 0.3416666666666666741, 0.3458333333333333259, 0.3499999999999999778, 0.3541666666666666852, 0.3583333333333333370, 0.3624999999999999889, 0.3666666666666666408, 0.3708333333333333481, 0.3750000000000000000, 0.3791666666666666519, 0.3833333333333333592, 0.3875000000000000111, 0.3916666666666666630, 0.3958333333333333148, 0.4000000000000000222, 0.4041666666666666741, 0.4083333333333333259, 0.4124999999999999778, 0.4166666666666666852, 0.4208333333333333370, 0.4249999999999999889, 0.4291666666666666408, 0.4333333333333333481, 0.4375000000000000000, 0.4416666666666666519, 0.4458333333333333592, 0.4500000000000000111, 0.4541666666666666630, 0.4583333333333333148, 0.4625000000000000222, 0.4666666666666666741, 0.4708333333333333259, 0.4749999999999999778, 0.4791666666666666852, 0.4833333333333333370, 0.4874999999999999889, 0.4916666666666666408, 0.4958333333333333481, 0.5000000000000000000, 0.5041666666666666519, 0.5083333333333333037, 0.5124999999999999556, 0.5166666666666667185, 0.5208333333333333703, 0.5250000000000000222, 0.5291666666666666741, 0.5333333333333333259, 0.5374999999999999778, 0.5416666666666666297, 0.5458333333333332815, 0.5500000000000000444, 0.5541666666666666963, 0.5583333333333333481, 0.5625000000000000000, 0.5666666666666666519, 0.5708333333333333037, 0.5749999999999999556, 0.5791666666666667185, 0.5833333333333333703, 0.5875000000000000222, 0.5916666666666666741, 0.5958333333333333259, 0.5999999999999999778, 0.6041666666666666297, 0.6083333333333332815, 0.6125000000000000444, 0.6166666666666666963, 0.6208333333333333481, 0.6250000000000000000, 0.6291666666666666519, 0.6333333333333333037, 0.6374999999999999556, 0.6416666666666667185, 0.6458333333333333703, 0.6500000000000000222, 0.6541666666666666741, 0.6583333333333333259, 0.6624999999999999778, 0.6666666666666666297, 0.6708333333333332815, 0.6750000000000000444, 0.6791666666666666963, 0.6833333333333333481, 0.6875000000000000000, 0.6916666666666666519, 0.6958333333333333037, 0.6999999999999999556, 0.7041666666666667185, 0.7083333333333333703, 0.7125000000000000222, 0.7166666666666666741, 0.7208333333333333259, 0.7249999999999999778, 0.7291666666666666297, 0.7333333333333332815, 0.7375000000000000444, 0.7416666666666666963, 0.7458333333333333481, 0.7500000000000000000, 0.7541666666666666519, 0.7583333333333333037, 0.7624999999999999556, 0.7666666666666667185, 0.7708333333333333703, 0.7750000000000000222, 0.7791666666666666741, 0.7833333333333333259, 0.7874999999999999778, 0.7916666666666666297, 0.7958333333333332815, 0.8000000000000000444, 0.8041666666666666963, 0.8083333333333333481, 0.8125000000000000000, 0.8166666666666666519, 0.8208333333333333037, 0.8249999999999999556, 0.8291666666666667185, 0.8333333333333333703, 0.8375000000000000222, 0.8416666666666666741, 0.8458333333333333259, 0.8499999999999999778, 0.8541666666666666297, 0.8583333333333332815, 0.8625000000000000444, 0.8666666666666666963, 0.8708333333333333481, 0.8750000000000000000, 0.8791666666666666519, 0.8833333333333333037, 0.8874999999999999556, 0.8916666666666667185, 0.8958333333333333703, 0.9000000000000000222, 0.9041666666666666741, 0.9083333333333333259, 0.9124999999999999778, 0.9166666666666666297, 0.9208333333333332815, 0.9250000000000000444, 0.9291666666666666963, 0.9333333333333333481, 0.9375000000000000000, 0.9416666666666666519, 0.9458333333333333037, 0.9499999999999999556, 0.9541666666666667185, 0.9583333333333333703, 0.9625000000000000222, 0.9666666666666666741, 0.9708333333333333259, 0.9749999999999999778, 0.9791666666666666297, 0.9833333333333332815, 0.9875000000000000444 ),
 .UNSPECIFIED. ) 
 GEOMETRIC_REPRESENTATION_ITEM ( )  RATIONAL_B_SPLINE_SURFACE ( (
 ( 1.000000000000000000, 0.9659258262890683122, 1.000000000000000000, 0.9659258262890683122, 1.000000000000000000, 0.9659258262890683122, 1.000000000000000000, 0.9659258262890683122, 1.000000000000000000, 0.9659258262890683122, 1.000000000000000000, 0.9659258262890683122, 1.000000000000000000, 0.9659258262890683122, 1.000000000000000000, 0.9659258262890683122, 1.000000000000000000, 0.9659258262890683122, 1.000000000000000000, 0.9659258262890683122, 1.000000000000000000, 0.9659258262890683122, 1.000000000000000000, 0.9659258262890683122, 1.000000000000000000, 0.9659258262890683122, 1.000000000000000000, 0.9659258262890683122, 1.000000000000000000, 0.9659258262890683122, 1.000000000000000000, 0.9659258262890683122, 1.000000000000000000, 0.9659258262890683122, 1.000000000000000000, 0.9659258262890683122, 1.000000000000000000, 0.9659258262890683122, 1.000000000000000000, 0.9659258262890683122, 1.000000000000000000, 0.9659258262890683122, 1.000000000000000000, 0.9659258262890683122, 1.000000000000000000, 0.9659258262890683122, 1.000000000000000000, 0.9659258262890683122, 1.000000000000000000, 0.9659258262890683122, 1.000000000000000000, 0.9659258262890683122, 1.000000000000000000, 0.9659258262890683122, 1.000000000000000000, 0.9659258262890683122, 1.000000000000000000, 0.9659258262890683122, 1.000000000000000000, 0.9659258262890683122, 1.000000000000000000, 0.9659258262890683122, 1.000000000000000000, 0.9659258262890683122, 1.000000000000000000, 0.9659258262890683122, 1.000000000000000000, 0.9659258262890683122, 1.000000000000000000, 0.9659258262890683122, 1.000000000000000000, 0.9659258262890683122, 1.000000000000000000, 0.9659258262890683122, 1.000000000000000000, 0.9659258262890683122, 1.000000000000000000, 0.9659258262890683122, 1.000000000000000000, 0.9659258262890683122, 1.000000000000000000, 0.9659258262890683122, 1.000000000000000000, 0.9659258262890683122, 1.000000000000000000, 0.9659258262890683122, 1.000000000000000000, 0.9659258262890683122, 1.000000000000000000, 0.9659258262890683122, 1.000000000000000000, 0.9659258262890683122, 1.000000000000000000, 0.9659258262890683122, 1.000000000000000000, 0.9659258262890683122, 1.000000000000000000, 0.9659258262890683122, 1.000000000000000000, 0.9659258262890683122, 1.000000000000000000, 0.9659258262890683122, 1.000000000000000000, 0.9659258262890683122, 1.000000000000000000, 0.9659258262890683122, 1.000000000000000000, 0.9659258262890683122, 1.000000000000000000, 0.9659258262890683122, 1.000000000000000000, 0.9659258262890683122, 1.000000000000000000, 0.9659258262890683122, 1.000000000000000000, 0.9659258262890683122, 1.000000000000000000, 0.9659258262890683122, 1.000000000000000000, 0.9659258262890683122, 1.000000000000000000, 0.9659258262890683122, 1.000000000000000000, 0.9659258262890683122, 1.000000000000000000, 0.9659258262890683122, 1.000000000000000000, 0.9659258262890683122, 1.000000000000000000, 0.9659258262890683122, 1.000000000000000000, 0.9659258262890683122, 1.000000000000000000, 0.9659258262890683122, 1.000000000000000000, 0.9659258262890683122, 1.000000000000000000, 0.9659258262890683122, 1.000000000000000000, 0.9659258262890683122, 1.000000000000000000, 0.9659258262890683122, 1.000000000000000000, 0.9659258262890683122, 1.000000000000000000, 0.9659258262890683122, 1.000000000000000000, 0.9659258262890683122, 1.000000000000000000, 0.9659258262890683122, 1.000000000000000000, 0.9659258262890683122, 1.000000000000000000, 0.9659258262890683122, 1.000000000000000000, 0.9659258262890683122, 1.000000000000000000, 0.9659258262890683122, 1.000000000000000000, 0.9659258262890683122, 1.000000000000000000, 0.9659258262890683122, 1.000000000000000000, 0.9659258262890683122, 1.000000000000000000, 0.9659258262890683122, 1.000000000000000000, 0.9659258262890683122, 1.000000000000000000, 0.9659258262890683122, 1.000000000000000000, 0.9659258262890683122, 1.000000000000000000, 0.9659258262890683122, 1.000000000000000000, 0.9659258262890683122, 1.000000000000000000, 0.9659258262890683122, 1.000000000000000000, 0.9659258262890683122, 1.000000000000000000, 0.9659258262890683122, 1.000000000000000000, 0.9659258262890683122, 1.000000000000000000, 0.9659258262890683122, 1.000000000000000000, 0.9659258262890683122, 1.000000000000000000, 0.9659258262890683122, 1.000000000000000000, 0.9659258262890683122, 1.000000000000000000, 0.9659258262890683122, 1.000000000000000000, 0.9659258262890683122, 1.000000000000000000, 0.9659258262890683122, 1.000000000000000000, 0.9659258262890683122, 1.000000000000000000, 0.9659258262890683122, 1.000000000000000000, 0.9659258262890683122, 1.000000000000000000, 0.9659258262890683122, 1.000000000000000000, 0.9659258262890683122, 1.000000000000000000, 0.9659258262890683122, 1.000000000000000000, 0.9659258262890683122, 1.000000000000000000, 0.9659258262890683122, 1.000000000000000000, 0.9659258262890683122, 1.000000000000000000, 0.9659258262890683122, 1.000000000000000000, 0.9659258262890683122, 1.000000000000000000, 0.9659258262890683122, 1.000000000000000000, 0.9659258262890683122, 1.000000000000000000, 0.9659258262890683122, 1.000000000000000000, 0.9659258262890683122, 1.000000000000000000, 0.9659258262890683122, 1.000000000000000000, 0.9659258262890683122, 1.000000000000000000, 0.9659258262890683122, 1.000000000000000000, 0.9659258262890683122, 1.000000000000000000, 0.9659258262890683122, 1.000000000000000000, 0.9659258262890683122, 1.000000000000000000, 0.9659258262890683122, 1.000000000000000000, 0.9659258262890683122, 1.000000000000000000, 0.9659258262890683122, 1.000000000000000000, 0.9659258262890683122, 1.000000000000000000, 0.9659258262890683122, 1.000000000000000000, 0.9659258262890683122, 1.000000000000000000, 0.9659258262890683122, 1.000000000000000000, 0.9659258262890683122, 1.000000000000000000, 0.9659258262890683122, 1.000000000000000000, 0.9659258262890683122, 1.000000000000000000, 0.9659258262890683122, 1.000000000000000000, 0.9659258262890683122, 1.000000000000000000, 0.9659258262890683122, 1.000000000000000000, 0.9659258262890683122, 1.000000000000000000, 0.9659258262890683122, 1.000000000000000000, 0.9659258262890683122, 1.000000000000000000, 0.9659258262890683122, 1.000000000000000000, 0.9659258262890683122, 1.000000000000000000, 0.9659258262890683122, 1.000000000000000000, 0.9659258262890683122, 1.000000000000000000, 0.9659258262890683122, 1.000000000000000000, 0.9659258262890683122, 1.000000000000000000, 0.9659258262890683122, 1.000000000000000000, 0.9659258262890683122, 1.000000000000000000, 0.9659258262890683122, 1.000000000000000000, 0.9659258262890683122, 1.000000000000000000, 0.9659258262890683122, 1.000000000000000000, 0.9659258262890683122, 1.000000000000000000, 0.9659258262890683122, 1.000000000000000000, 0.9659258262890683122, 1.000000000000000000, 0.9659258262890683122, 1.000000000000000000, 0.9659258262890683122, 1.000000000000000000, 0.9659258262890683122, 1.000000000000000000, 0.9659258262890683122, 1.000000000000000000, 0.9659258262890683122, 1.000000000000000000, 0.9659258262890683122, 1.000000000000000000, 0.9659258262890683122, 1.000000000000000000, 0.9659258262890683122, 1.000000000000000000, 0.9659258262890683122, 1.000000000000000000, 0.9659258262890683122, 1.000000000000000000, 0.9659258262890683122, 1.000000000000000000, 0.9659258262890683122, 1.000000000000000000, 0.9659258262890683122, 1.000000000000000000, 0.9659258262890683122, 1.000000000000000000, 0.9659258262890683122, 1.000000000000000000, 0.9659258262890683122, 1.000000000000000000, 0.9659258262890683122, 1.000000000000000000, 0.9659258262890683122, 1.000000000000000000, 0.9659258262890683122, 1.000000000000000000, 0.9659258262890683122, 1.000000000000000000, 0.9659258262890683122, 1.000000000000000000, 0.9659258262890683122, 1.000000000000000000, 0.9659258262890683122, 1.000000000000000000, 0.9659258262890683122, 1.000000000000000000, 0.9659258262890683122, 1.000000000000000000, 0.9659258262890683122, 1.000000000000000000, 0.9659258262890683122, 1.000000000000000000, 0.9659258262890683122, 1.000000000000000000, 0.9659258262890683122, 1.000000000000000000, 0.9659258262890683122, 1.000000000000000000, 0.9659258262890683122, 1.000000000000000000, 0.9659258262890683122, 1.000000000000000000, 0.9659258262890683122, 1.000000000000000000, 0.9659258262890683122, 1.000000000000000000, 0.9659258262890683122, 1.000000000000000000, 0.9659258262890683122, 1.000000000000000000, 0.9659258262890683122, 1.000000000000000000, 0.9659258262890683122, 1.000000000000000000, 0.9659258262890683122, 1.000000000000000000, 0.9659258262890683122, 1.000000000000000000, 0.9659258262890683122, 1.000000000000000000, 0.9659258262890683122, 1.000000000000000000, 0.9659258262890683122, 1.000000000000000000, 0.9659258262890683122, 1.000000000000000000, 0.9659258262890683122, 1.000000000000000000, 0.9659258262890683122, 1.000000000000000000, 0.9659258262890683122, 1.000000000000000000, 0.9659258262890683122, 1.000000000000000000, 0.9659258262890683122, 1.000000000000000000, 0.9659258262890683122, 1.000000000000000000, 0.9659258262890683122, 1.000000000000000000, 0.9659258262890683122, 1.000000000000000000, 0.9659258262890683122, 1.000000000000000000, 0.9659258262890683122, 1.000000000000000000, 0.9659258262890683122, 1.000000000000000000, 0.9659258262890683122, 1.000000000000000000, 0.9659258262890683122, 1.000000000000000000, 0.9659258262890683122, 1.000000000000000000, 0.9659258262890683122, 1.000000000000000000, 0.9659258262890683122, 1.000000000000000000, 0.9659258262890683122, 1.000000000000000000, 0.9659258262890683122, 1.000000000000000000, 0.9659258262890683122, 1.000000000000000000, 0.9659258262890683122, 1.000000000000000000, 0.9659258262890683122, 1.000000000000000000, 0.9659258262890683122, 1.000000000000000000, 0.9659258262890683122, 1.000000000000000000, 0.9659258262890683122, 1.000000000000000000, 0.9659258262890683122, 1.000000000000000000, 0.9659258262890683122, 1.000000000000000000, 0.9659258262890683122, 1.000000000000000000, 0.9659258262890683122, 1.000000000000000000, 0.9659258262890683122, 1.000000000000000000, 0.9659258262890683122, 1.000000000000000000, 0.9659258262890683122, 1.000000000000000000, 0.9659258262890683122, 1.000000000000000000, 0.9659258262890683122, 1.000000000000000000, 0.9659258262890683122, 1.000000000000000000, 0.9659258262890683122, 1.000000000000000000, 0.9659258262890683122, 1.000000000000000000, 0.9659258262890683122, 1.000000000000000000, 0.9659258262890683122, 1.000000000000000000, 0.9659258262890683122, 1.000000000000000000, 0.9659258262890683122, 1.000000000000000000, 0.9659258262890683122, 1.000000000000000000, 0.9659258262890683122, 1.000000000000000000, 0.9659258262890683122, 1.000000000000000000),
 ( 1.000000000000000000, 0.9659258262890683122, 1.000000000000000000, 0.9659258262890683122, 1.000000000000000000, 0.9659258262890683122, 1.000000000000000000, 0.9659258262890683122, 1.000000000000000000, 0.9659258262890683122, 1.000000000000000000, 0.9659258262890683122, 1.000000000000000000, 0.9659258262890683122, 1.000000000000000000, 0.9659258262890683122, 1.000000000000000000, 0.9659258262890683122, 1.000000000000000000, 0.9659258262890683122, 1.000000000000000000, 0.9659258262890683122, 1.000000000000000000, 0.9659258262890683122, 1.000000000000000000, 0.9659258262890683122, 1.000000000000000000, 0.9659258262890683122, 1.000000000000000000, 0.9659258262890683122, 1.000000000000000000, 0.9659258262890683122, 1.000000000000000000, 0.9659258262890683122, 1.000000000000000000, 0.9659258262890683122, 1.000000000000000000, 0.9659258262890683122, 1.000000000000000000, 0.9659258262890683122, 1.000000000000000000, 0.9659258262890683122, 1.000000000000000000, 0.9659258262890683122, 1.000000000000000000, 0.9659258262890683122, 1.000000000000000000, 0.9659258262890683122, 1.000000000000000000, 0.9659258262890683122, 1.000000000000000000, 0.9659258262890683122, 1.000000000000000000, 0.9659258262890683122, 1.000000000000000000, 0.9659258262890683122, 1.000000000000000000, 0.9659258262890683122, 1.000000000000000000, 0.9659258262890683122, 1.000000000000000000, 0.9659258262890683122, 1.000000000000000000, 0.9659258262890683122, 1.000000000000000000, 0.9659258262890683122, 1.000000000000000000, 0.9659258262890683122, 1.000000000000000000, 0.9659258262890683122, 1.000000000000000000, 0.9659258262890683122, 1.000000000000000000, 0.9659258262890683122, 1.000000000000000000, 0.9659258262890683122, 1.000000000000000000, 0.9659258262890683122, 1.000000000000000000, 0.9659258262890683122, 1.000000000000000000, 0.9659258262890683122, 1.000000000000000000, 0.9659258262890683122, 1.000000000000000000, 0.9659258262890683122, 1.000000000000000000, 0.9659258262890683122, 1.000000000000000000, 0.9659258262890683122, 1.000000000000000000, 0.9659258262890683122, 1.000000000000000000, 0.9659258262890683122, 1.000000000000000000, 0.9659258262890683122, 1.000000000000000000, 0.9659258262890683122, 1.000000000000000000, 0.9659258262890683122, 1.000000000000000000, 0.9659258262890683122, 1.000000000000000000, 0.9659258262890683122, 1.000000000000000000, 0.9659258262890683122, 1.000000000000000000, 0.9659258262890683122, 1.000000000000000000, 0.9659258262890683122, 1.000000000000000000, 0.9659258262890683122, 1.000000000000000000, 0.9659258262890683122, 1.000000000000000000, 0.9659258262890683122, 1.000000000000000000, 0.9659258262890683122, 1.000000000000000000, 0.9659258262890683122, 1.000000000000000000, 0.9659258262890683122, 1.000000000000000000, 0.9659258262890683122, 1.000000000000000000, 0.9659258262890683122, 1.000000000000000000, 0.9659258262890683122, 1.000000000000000000, 0.9659258262890683122, 1.000000000000000000, 0.9659258262890683122, 1.000000000000000000, 0.9659258262890683122, 1.000000000000000000, 0.9659258262890683122, 1.000000000000000000, 0.9659258262890683122, 1.000000000000000000, 0.9659258262890683122, 1.000000000000000000, 0.9659258262890683122, 1.000000000000000000, 0.9659258262890683122, 1.000000000000000000, 0.9659258262890683122, 1.000000000000000000, 0.9659258262890683122, 1.000000000000000000, 0.9659258262890683122, 1.000000000000000000, 0.9659258262890683122, 1.000000000000000000, 0.9659258262890683122, 1.000000000000000000, 0.9659258262890683122, 1.000000000000000000, 0.9659258262890683122, 1.000000000000000000, 0.9659258262890683122, 1.000000000000000000, 0.9659258262890683122, 1.000000000000000000, 0.9659258262890683122, 1.000000000000000000, 0.9659258262890683122, 1.000000000000000000, 0.9659258262890683122, 1.000000000000000000, 0.9659258262890683122, 1.000000000000000000, 0.9659258262890683122, 1.000000000000000000, 0.9659258262890683122, 1.000000000000000000, 0.9659258262890683122, 1.000000000000000000, 0.9659258262890683122, 1.000000000000000000, 0.9659258262890683122, 1.000000000000000000, 0.9659258262890683122, 1.000000000000000000, 0.9659258262890683122, 1.000000000000000000, 0.9659258262890683122, 1.000000000000000000, 0.9659258262890683122, 1.000000000000000000, 0.9659258262890683122, 1.000000000000000000, 0.9659258262890683122, 1.000000000000000000, 0.9659258262890683122, 1.000000000000000000, 0.9659258262890683122, 1.000000000000000000, 0.9659258262890683122, 1.000000000000000000, 0.9659258262890683122, 1.000000000000000000, 0.9659258262890683122, 1.000000000000000000, 0.9659258262890683122, 1.000000000000000000, 0.9659258262890683122, 1.000000000000000000, 0.9659258262890683122, 1.000000000000000000, 0.9659258262890683122, 1.000000000000000000, 0.9659258262890683122, 1.000000000000000000, 0.9659258262890683122, 1.000000000000000000, 0.9659258262890683122, 1.000000000000000000, 0.9659258262890683122, 1.000000000000000000, 0.9659258262890683122, 1.000000000000000000, 0.9659258262890683122, 1.000000000000000000, 0.9659258262890683122, 1.000000000000000000, 0.9659258262890683122, 1.000000000000000000, 0.9659258262890683122, 1.000000000000000000, 0.9659258262890683122, 1.000000000000000000, 0.9659258262890683122, 1.000000000000000000, 0.9659258262890683122, 1.000000000000000000, 0.9659258262890683122, 1.000000000000000000, 0.9659258262890683122, 1.000000000000000000, 0.9659258262890683122, 1.000000000000000000, 0.9659258262890683122, 1.000000000000000000, 0.9659258262890683122, 1.000000000000000000, 0.9659258262890683122, 1.000000000000000000, 0.9659258262890683122, 1.000000000000000000, 0.9659258262890683122, 1.000000000000000000, 0.9659258262890683122, 1.000000000000000000, 0.9659258262890683122, 1.000000000000000000, 0.9659258262890683122, 1.000000000000000000, 0.9659258262890683122, 1.000000000000000000, 0.9659258262890683122, 1.000000000000000000, 0.9659258262890683122, 1.000000000000000000, 0.9659258262890683122, 1.000000000000000000, 0.9659258262890683122, 1.000000000000000000, 0.9659258262890683122, 1.000000000000000000, 0.9659258262890683122, 1.000000000000000000, 0.9659258262890683122, 1.000000000000000000, 0.9659258262890683122, 1.000000000000000000, 0.9659258262890683122, 1.000000000000000000, 0.9659258262890683122, 1.000000000000000000, 0.9659258262890683122, 1.000000000000000000, 0.9659258262890683122, 1.000000000000000000, 0.9659258262890683122, 1.000000000000000000, 0.9659258262890683122, 1.000000000000000000, 0.9659258262890683122, 1.000000000000000000, 0.9659258262890683122, 1.000000000000000000, 0.9659258262890683122, 1.000000000000000000, 0.9659258262890683122, 1.000000000000000000, 0.9659258262890683122, 1.000000000000000000, 0.9659258262890683122, 1.000000000000000000, 0.9659258262890683122, 1.000000000000000000, 0.9659258262890683122, 1.000000000000000000, 0.9659258262890683122, 1.000000000000000000, 0.9659258262890683122, 1.000000000000000000, 0.9659258262890683122, 1.000000000000000000, 0.9659258262890683122, 1.000000000000000000, 0.9659258262890683122, 1.000000000000000000, 0.9659258262890683122, 1.000000000000000000, 0.9659258262890683122, 1.000000000000000000, 0.9659258262890683122, 1.000000000000000000, 0.9659258262890683122, 1.000000000000000000, 0.9659258262890683122, 1.000000000000000000, 0.9659258262890683122, 1.000000000000000000, 0.9659258262890683122, 1.000000000000000000, 0.9659258262890683122, 1.000000000000000000, 0.9659258262890683122, 1.000000000000000000, 0.9659258262890683122, 1.000000000000000000, 0.9659258262890683122, 1.000000000000000000, 0.9659258262890683122, 1.000000000000000000, 0.9659258262890683122, 1.000000000000000000, 0.9659258262890683122, 1.000000000000000000, 0.9659258262890683122, 1.000000000000000000, 0.9659258262890683122, 1.000000000000000000, 0.9659258262890683122, 1.000000000000000000, 0.9659258262890683122, 1.000000000000000000, 0.9659258262890683122, 1.000000000000000000, 0.9659258262890683122, 1.000000000000000000, 0.9659258262890683122, 1.000000000000000000, 0.9659258262890683122, 1.000000000000000000, 0.9659258262890683122, 1.000000000000000000, 0.9659258262890683122, 1.000000000000000000, 0.9659258262890683122, 1.000000000000000000, 0.9659258262890683122, 1.000000000000000000, 0.9659258262890683122, 1.000000000000000000, 0.9659258262890683122, 1.000000000000000000, 0.9659258262890683122, 1.000000000000000000, 0.9659258262890683122, 1.000000000000000000, 0.9659258262890683122, 1.000000000000000000, 0.9659258262890683122, 1.000000000000000000, 0.9659258262890683122, 1.000000000000000000, 0.9659258262890683122, 1.000000000000000000, 0.9659258262890683122, 1.000000000000000000, 0.9659258262890683122, 1.000000000000000000, 0.9659258262890683122, 1.000000000000000000, 0.9659258262890683122, 1.000000000000000000, 0.9659258262890683122, 1.000000000000000000, 0.9659258262890683122, 1.000000000000000000, 0.9659258262890683122, 1.000000000000000000, 0.9659258262890683122, 1.000000000000000000, 0.9659258262890683122, 1.000000000000000000, 0.9659258262890683122, 1.000000000000000000, 0.9659258262890683122, 1.000000000000000000, 0.9659258262890683122, 1.000000000000000000, 0.9659258262890683122, 1.000000000000000000, 0.9659258262890683122, 1.000000000000000000, 0.9659258262890683122, 1.000000000000000000, 0.9659258262890683122, 1.000000000000000000, 0.9659258262890683122, 1.000000000000000000, 0.9659258262890683122, 1.000000000000000000, 0.9659258262890683122, 1.000000000000000000, 0.9659258262890683122, 1.000000000000000000, 0.9659258262890683122, 1.000000000000000000, 0.9659258262890683122, 1.000000000000000000, 0.9659258262890683122, 1.000000000000000000, 0.9659258262890683122, 1.000000000000000000, 0.9659258262890683122, 1.000000000000000000, 0.9659258262890683122, 1.000000000000000000, 0.9659258262890683122, 1.000000000000000000, 0.9659258262890683122, 1.000000000000000000, 0.9659258262890683122, 1.000000000000000000, 0.9659258262890683122, 1.000000000000000000, 0.9659258262890683122, 1.000000000000000000, 0.9659258262890683122, 1.000000000000000000, 0.9659258262890683122, 1.000000000000000000, 0.9659258262890683122, 1.000000000000000000, 0.9659258262890683122, 1.000000000000000000, 0.9659258262890683122, 1.000000000000000000, 0.9659258262890683122, 1.000000000000000000, 0.9659258262890683122, 1.000000000000000000, 0.9659258262890683122, 1.000000000000000000, 0.9659258262890683122, 1.000000000000000000, 0.9659258262890683122, 1.000000000000000000, 0.9659258262890683122, 1.000000000000000000, 0.9659258262890683122, 1.000000000000000000, 0.9659258262890683122, 1.000000000000000000, 0.9659258262890683122, 1.000000000000000000, 0.9659258262890683122, 1.000000000000000000, 0.9659258262890683122, 1.000000000000000000) ) ) 
 REPRESENTATION_ITEM ( '' )  SURFACE ( )  );
#17720=CARTESIAN_POINT ( 'NONE',  ( -0.2867679344610365999, 0.2867679344610364889, -1.521653543307086354 ) ) ;
#17725=CARTESIAN_POINT ( 'NONE',  ( 0.3458507752293908943, 0.3458507752293908943, -1.159448818897637734 ) ) ;
#17728=CARTESIAN_POINT ( 'NONE',  ( -0.2891555358219911054, 0.2891555358219909388, -0.8838582677165351953 ) ) ;
#17741=CARTESIAN_POINT ( 'NONE',  ( -0.2925321140481930149, -0.2925321140481933480, -1.553149606299212726 ) ) ;
#17743=CARTESIAN_POINT ( 'NONE',  ( -0.1049643490035307020, 0.3917322834645669549, -1.416010498687664043 ) ) ;
#17756=CARTESIAN_POINT ( 'NONE',  ( 0.1049643490035303689, 0.3917322834645670104, -1.180446194225722056 ) ) ;
#17770=CARTESIAN_POINT ( 'NONE',  ( -0.4724409448818898682, 5.785732909357575061E-17, -2.755905511811024056 ) ) ;
#17773=CARTESIAN_POINT ( 'NONE',  ( 0.2867679344610366554, 0.2867679344610366554, -2.177165354330708347 ) ) ;
#17776=CARTESIAN_POINT ( 'NONE',  ( 0.4724409448818897572, -0.1265901696524988906, -0.2690288713910760632 ) ) ;
#17777=CARTESIAN_POINT ( 'NONE',  ( 0.1058382717557500713, -0.3949938075777409408, -2.762467191601050587 ) ) ;
#17780=CARTESIAN_POINT ( 'NONE',  ( 0.2867679344610365999, 0.2867679344610365999, -1.232283464566929387 ) ) ;
#17782=CARTESIAN_POINT ( 'NONE',  ( 0.4724409448818897572, -0.1265901696524988906, -2.316272965879265122 ) ) ;
#17788=CARTESIAN_POINT ( 'NONE',  ( -0.1049643490035301746, -0.3917322834645670659, -0.7821329151892896236 ) ) ;
#17796=CARTESIAN_POINT ( 'NONE',  ( -0.3917322834645670104, -0.1049643490035307020, -1.932434013944568818 ) ) ;
#17803=CARTESIAN_POINT ( 'NONE',  ( -0.1049643490035302024, -0.3917322834645671215, -1.574146981627296604 ) ) ;
#17813=CARTESIAN_POINT ( 'NONE',  ( 0.2362204724409451007, -0.4091458600556402980, -0.9560367454068241511 ) ) ;
#17815=CARTESIAN_POINT ( 'NONE',  ( 0.3917322834645669549, 0.1049643490035304660, -2.793963254593175183 ) ) ;
#17822=CARTESIAN_POINT ( 'NONE',  ( 0.1958661417322836440, -0.3392501089628017219, -1.278871391076115582 ) ) ;
#17823=CARTESIAN_POINT ( 'NONE',  ( 0.2362204724409449064, 0.4091458600556404646, 0.09383202099737532331 ) ) ;
#17825=CARTESIAN_POINT ( 'NONE',  ( 0.1070741851644054776, -0.3996062992125984925, -2.839238845144356649 ) ) ;
#17834=CARTESIAN_POINT ( 'NONE',  ( -0.1998031496062991630, -0.3460692066303959202, -0.4573490813648293796 ) ) ;
#17836=CARTESIAN_POINT ( 'NONE',  ( -0.3917322834645670104, -7.196005306013484475E-17, -0.3464566929133857665 ) ) ;
#17843=CARTESIAN_POINT ( 'NONE',  ( 0.3917322834645668994, -0.1049643490035303134, -1.608904568732596685 ) ) ;
#17852=CARTESIAN_POINT ( 'NONE',  ( 0.3392501089628018884, -0.1958661417322833942, -0.8891269273303956666 ) ) ;
#17856=CARTESIAN_POINT ( 'NONE',  ( 0.1265901696524989462, 0.4724409448818897572, -2.117454068241469756 ) ) ;
#17876=CARTESIAN_POINT ( 'NONE',  ( 0.1998031496062994128, -0.3460692066303957537, -2.530839895013123453 ) ) ;
#17881=CARTESIAN_POINT ( 'NONE',  ( 0.2925321140481932369, 0.2925321140481932369, -2.027559055118109743 ) ) ;
#17882=CARTESIAN_POINT ( 'NONE',  ( 0.1058382717557500713, -0.3949938075777409408, -1.502624671916010790 ) ) ;
#17885=CARTESIAN_POINT ( 'NONE',  ( -0.1958661417322834220, -0.3392501089628018884, -0.5301837270341206443 ) ) ;
#17889=CARTESIAN_POINT ( 'NONE',  ( -0.1058382717557503072, 0.3949938075777408852, -2.603018372703412187 ) ) ;
#17894=CARTESIAN_POINT ( 'NONE',  ( -0.1998031496062994683, 0.3460692066303958092, -2.060367454068241511 ) ) ;
#17902=CARTESIAN_POINT ( 'NONE',  ( -0.1958661417322834220, -0.3392501089628018884, -0.1502624671916011345 ) ) ;
#17910=CARTESIAN_POINT ( 'NONE',  ( -9.594673741351313045E-17, 0.3917322834645670104, -0.3996062992125985480 ) ) ;
#17911=CARTESIAN_POINT ( 'NONE',  ( -9.594673741351313045E-17, 0.3917322834645670104, -1.409448818897637734 ) ) ;
#17912=CARTESIAN_POINT ( 'NONE',  ( -0.1958661417322834220, -0.3392501089628018884, -2.734908136482939511 ) ) ;
#17915=CARTESIAN_POINT ( 'NONE',  ( -0.1974969037888706647, 0.3420746716998658843, -2.847769028871391495 ) ) ;
#17916=ORIENTED_EDGE ( 'NONE', *, *, #8023, .T. ) ;
#17919=CARTESIAN_POINT ( 'NONE',  ( 0.3996062992125986590, -0.1070741851644053111, -1.371391076115485053 ) ) ;
#17923=CARTESIAN_POINT ( 'NONE',  ( 0.2867679344610365999, -0.2867679344610365444, -0.4980314960629922405 ) ) ;
#17924=VECTOR ( 'NONE', #25188, 39.37007874015748143 ) ;
#17933=CARTESIAN_POINT ( 'NONE',  ( 0.4724409448818898682, 2.892866454678787531E-17, -1.850393700787401619 ) ) ;
#17943=CARTESIAN_POINT ( 'NONE',  ( 0.3917322834645669549, 2.398668435337827645E-17, -0.3556237288375834749 ) ) ;
#17945=CARTESIAN_POINT ( 'NONE',  ( 0.3392501089628018329, 0.1958661417322835607, -0.6883202099737534274 ) ) ;
#17950=CARTESIAN_POINT ( 'NONE',  ( -0.1049643490035302024, -0.3917322834645671215, -2.583989501312335513 ) ) ;
#17953=CARTESIAN_POINT ( 'NONE',  ( -0.3458507752293906723, -0.3458507752293910609, -0.9232283464566929387 ) ) ;
#17964=VERTEX_POINT ( 'NONE', #23735 ) ;
#17965=CARTESIAN_POINT ( 'NONE',  ( 0.3996062992125984925, 0.1070741851644054637, -2.091207349081364519 ) ) ;
#17973=CARTESIAN_POINT ( 'NONE',  ( -9.787531504996566615E-17, 0.3996062992125985480, -0.8641732283464567121 ) ) ;
#17974=CARTESIAN_POINT ( 'NONE',  ( 0.3996062992125986035, 2.446882876249141962E-17, -1.062992125984252079 ) ) ;
#17976=CARTESIAN_POINT ( 'NONE',  ( -0.3949938075777409963, -7.255918531996591613E-17, -0.1968503937007874682 ) ) ;
#17982=CARTESIAN_POINT ( 'NONE',  ( 0.1974969037888706092, -0.3420746716998660508, -1.428477690288714186 ) ) ;
#17988=CARTESIAN_POINT ( 'NONE',  ( -0.4091458600556405756, 0.2362204724409446288, -1.286089238845144367 ) ) ;
#17989=CARTESIAN_POINT ( 'NONE',  ( 4.893765752498283924E-17, -0.3996062992125986035, -2.755905511811023612 ) ) ;
#17992=CARTESIAN_POINT ( 'NONE',  ( -0.1049643490035307158, 0.3917322834645670104, -0.9481820454406320042 ) ) ;
#18003=CARTESIAN_POINT ( 'NONE',  ( 0.3917322834645670104, 2.398668435337828261E-17, -1.055118110236220375 ) ) ;
#18006=CARTESIAN_POINT ( 'NONE',  ( -0.1974969037888706647, 0.3420746716998658843, -1.587926509186351920 ) ) ;
#18011=CARTESIAN_POINT ( 'NONE',  ( -0.3460692066303960868, 0.1998031496062990242, -0.1837270341207349056 ) ) ;
#18018=CARTESIAN_POINT ( 'NONE',  ( -0.1958661417322834220, -0.3392501089628018884, -0.1502624671916011345 ) ) ;
#18024=ORIENTED_EDGE ( 'NONE', *, *, #58932, .F. ) ;
#18025=CARTESIAN_POINT ( 'NONE',  ( -0.3996062992125987146, 0.1070741851644051862, -2.237532808398950301 ) ) ;
#18027=VERTEX_POINT ( 'NONE', #74273 ) ;
#18028=CARTESIAN_POINT ( 'NONE',  ( 0.2925321140481932369, 0.2925321140481932369, -1.789370078740157410 ) ) ;
#18032=CARTESIAN_POINT ( 'NONE',  ( -0.2362204724409447953, -0.4091458600556404646, -0.3805774278215223183 ) ) ;
#18034=CARTESIAN_POINT ( 'NONE',  ( 0.3917322834645670104, 2.398668435337828261E-17, 0.04724409448818902429 ) ) ;
#18040=CARTESIAN_POINT ( 'NONE',  ( -0.4724409448818899238, 0.1265901696524986686, -2.471784776902887337 ) ) ;
#18043=CARTESIAN_POINT ( 'NONE',  ( -9.674558042662122972E-17, 0.3949938075777409963, -2.281496062992126372 ) ) ;
#18054=CARTESIAN_POINT ( 'NONE',  ( -0.1265901696524993347, 0.4724409448818896462, -1.028215223097112663 ) ) ;
#18064=CARTESIAN_POINT ( 'NONE',  ( 4.893765752498283308E-17, -0.3996062992125985480, -0.6279527559055118058 ) ) ;
#18065=CARTESIAN_POINT ( 'NONE',  ( 4.797336870675656522E-17, -0.3917322834645670104, -2.053149606299212948 ) ) ;
#18074=CARTESIAN_POINT ( 'NONE',  ( -0.4091458600556405756, 0.2362204724409446288, -2.230971128608923770 ) ) ;
#18081=CARTESIAN_POINT ( 'NONE',  ( 0.3917322834645669549, 0.1049643490035304660, -1.626640419947506411 ) ) ;
#18085=CARTESIAN_POINT ( 'NONE',  ( -0.1265901696524993347, 0.4724409448818896462, -0.4790026246719158998 ) ) ;
#18086=CARTESIAN_POINT ( 'NONE',  ( 0.3996062992125985480, 2.446882876249141654E-17, -2.557086614173228689 ) ) ;
#18088=CARTESIAN_POINT ( 'NONE',  ( 0.3996062992125986035, 0.1070741851644054776, -1.069553805774278166 ) ) ;
#18091=CARTESIAN_POINT ( 'NONE',  ( -0.2867679344610365999, 0.2867679344610364889, -2.531496062992125484 ) ) ;
#18104=CARTESIAN_POINT ( 'NONE',  ( -0.2867679344610364334, -0.2867679344610367109, -2.820866141732283339 ) ) ;
#18107=CARTESIAN_POINT ( 'NONE',  ( 0.3949938075777409963, 2.418639510665530435E-17, -0.2755905511811024278 ) ) ;
#18114=CARTESIAN_POINT ( 'NONE',  ( 4.797336870675656522E-17, -0.3917322834645670659, -1.492801468012810329 ) ) ;
#18116=CARTESIAN_POINT ( 'NONE',  ( -0.3917322834645670104, -7.196005306013484475E-17, -2.643700787401574548 ) ) ;
#18122=CARTESIAN_POINT ( 'NONE',  ( -0.1070741851644051862, -0.3996062992125987146, -0.7020997375328084100 ) ) ;
#18124=CARTESIAN_POINT ( 'NONE',  ( -0.3996062992125985480, -7.340648628747423112E-17, -0.4311023622047244208 ) ) ;
#18126=CARTESIAN_POINT ( 'NONE',  ( 0.1998031496062994405, -0.3460692066303958092, -2.296587926509186417 ) ) ;
#18127=CARTESIAN_POINT ( 'NONE',  ( -0.3917322834645670104, -7.196005306013484475E-17, -1.541338582677165503 ) ) ;
#18131=CARTESIAN_POINT ( 'NONE',  ( -0.3458507752293909498, 0.3458507752293907833, -1.041338582677165281 ) ) ;
#18134=CARTESIAN_POINT ( 'NONE',  ( 4.837279021331061486E-17, -0.3949938075777409963, -1.100393700787401619 ) ) ;
#18146=CARTESIAN_POINT ( 'NONE',  ( -9.787531504996566615E-17, 0.3996062992125985480, -1.651574803149606474 ) ) ;
#18163=CARTESIAN_POINT ( 'NONE',  ( -0.1958661417322836718, 0.3392501089628017219, -1.042650918635170676 ) ) ;
#18182=CARTESIAN_POINT ( 'NONE',  ( -0.1958661417322836718, 0.3392501089628017219, -2.052493438320210029 ) ) ;
#18185=CARTESIAN_POINT ( 'NONE',  ( 0.4091458600556403535, 0.2362204724409449896, -0.2887139107611548794 ) ) ;
#18186=CARTESIAN_POINT ( 'NONE',  ( 0.3420746716998660508, -0.1974969037888703871, -2.782152230971128848 ) ) ;
#18189=CARTESIAN_POINT ( 'NONE',  ( 0.2867679344610365999, -0.2867679344610365444, -1.507874015748031260 ) ) ;
#18191=CARTESIAN_POINT ( 'NONE',  ( -0.2362204724409447953, -0.4091458600556404646, -2.270341207349081181 ) ) ;
#18198=CARTESIAN_POINT ( 'NONE',  ( 0.1958661417322834497, 0.3392501089628018329, -0.8543113928795783574 ) ) ;
#18202=CARTESIAN_POINT ( 'NONE',  ( -0.09156050430092219083, -0.3808816823641230087, -1.492482962822815952E-17 ) ) ;
#18205=CARTESIAN_POINT ( 'NONE',  ( 0.2867679344610366554, 0.2867679344610366554, -2.181777845965566343 ) ) ;
#18213=CARTESIAN_POINT ( 'NONE',  ( 4.797336870675656522E-17, -0.3917322834645670104, -1.580708661417322913 ) ) ;
#18222=CARTESIAN_POINT ( 'NONE',  ( -0.3917322834645670104, -7.196005306013484475E-17, -2.866141732283464361 ) ) ;
#18228=CYLINDRICAL_SURFACE ( 'NONE', #12908, 0.2952755905511810774 ) ;
#18229=CARTESIAN_POINT ( 'NONE',  ( -0.2867679344610364334, -0.2867679344610367109, -1.246062992125984481 ) ) ;
#18230=CARTESIAN_POINT ( 'NONE',  ( -0.1265901696524993347, 0.4724409448818895907, 0.07414698162729659037 ) ) ;
#18232=CARTESIAN_POINT ( 'NONE',  ( 0.1974969037888704704, 0.3420746716998660508, 0.09383202099737533719 ) ) ;
#18241=CARTESIAN_POINT ( 'NONE',  ( 0.2925321140481932369, -0.2925321140481931814, -0.6476377952755905110 ) ) ;
#18243=CARTESIAN_POINT ( 'NONE',  ( 0.2867679344610365999, -0.2867679344610365444, -0.4055118110236220486 ) ) ;
#18258=CARTESIAN_POINT ( 'NONE',  ( -0.1049643490035302301, -0.3917322834645671770, -1.013798843340894207 ) ) ;
#18262=CARTESIAN_POINT ( 'NONE',  ( 0.2362204724409451007, -0.4091458600556402980, -2.373359580052493367 ) ) ;
#18268=FACE_OUTER_BOUND ( 'NONE', #83116, .T. ) ;
#18283=CARTESIAN_POINT ( 'NONE',  ( 0.3460692066303959202, 0.1998031496062993295, -0.1312335958005249603 ) ) ;
#18284=CARTESIAN_POINT ( 'NONE',  ( 0.2925321140481932369, -0.2925321140481931814, -2.694881889763780070 ) ) ;
#18289=CARTESIAN_POINT ( 'NONE',  ( -0.1998031496062991907, -0.3460692066303959757, -2.270341207349081181 ) ) ;
#18290=CARTESIAN_POINT ( 'NONE',  ( 0.3949938075777411073, -0.1058382717557499464, -1.528871391076115804 ) ) ;
#18291=CARTESIAN_POINT ( 'NONE',  ( -0.3996062992125986035, -7.340648628747425578E-17, -2.716535433070865757 ) ) ;
#18293=CARTESIAN_POINT ( 'NONE',  ( -0.2867679344610364334, -0.2867679344610367109, -0.6811023622047243098 ) ) ;
#18296=CARTESIAN_POINT ( 'NONE',  ( -0.3949938075777409963, -7.255918531996591613E-17, -2.478346456692914312 ) ) ;
#18301=CARTESIAN_POINT ( 'NONE',  ( -0.4724409448818899238, 0.1265901696524986686, -2.709973753280840114 ) ) ;
#18302=CARTESIAN_POINT ( 'NONE',  ( 0.1998031496062994405, -0.3460692066303958092, -2.139107611548556331 ) ) ;
#18303=FACE_OUTER_BOUND ( 'NONE', #80659, .T. ) ;
#18304=AXIS2_PLACEMENT_3D ( 'NONE', #24348, #50017, #31905 ) ;
#18311=CARTESIAN_POINT ( 'NONE',  ( -0.2867679344610364334, -0.2867679344610367109, -0.3011811023622048000 ) ) ;
#18317=CARTESIAN_POINT ( 'NONE',  ( 0.3392501089628018884, -0.1958661417322834220, -0.6620734908136483021 ) ) ;
#18318=CARTESIAN_POINT ( 'NONE',  ( 0.2867679344610365999, 0.2867679344610365999, -1.547244094488189115 ) ) ;
#18319=CARTESIAN_POINT ( 'NONE',  ( 0.2867679344610365999, 0.2867679344610365999, -2.649606299212598604 ) ) ;
#18323=CARTESIAN_POINT ( 'NONE',  ( -0.2891555358219911054, 0.2891555358219909388, -2.539370078740157854 ) ) ;
#18328=CARTESIAN_POINT ( 'NONE',  ( -0.1998031496062991907, -0.3460692066303959757, -1.482939632545931863 ) ) ;
#18330=CARTESIAN_POINT ( 'NONE',  ( 5.785732909357575061E-17, -0.4724409448818898682, -0.7854330708661416693 ) ) ;
#18333=CARTESIAN_POINT ( 'NONE',  ( 4.797336870675656522E-17, -0.3917322834645670104, -0.3208661417322835607 ) ) ;
#18343=CARTESIAN_POINT ( 'NONE',  ( 0.1265901696524990294, -0.4724409448818896462, -2.132545931758530244 ) ) ;
#18353=CARTESIAN_POINT ( 'NONE',  ( -0.3917322834645669549, -7.196005306013483243E-17, -0.2768835713572685431 ) ) ;
#18355=CARTESIAN_POINT ( 'NONE',  ( 4.797336870675656522E-17, -0.3917322834645670104, -0.7933070866141732624 ) ) ;
#18360=CARTESIAN_POINT ( 'NONE',  ( -0.3917322834645669549, -0.1049643490035306603, -2.872703412073490448 ) ) ;
#18365=CARTESIAN_POINT ( 'NONE',  ( 0.4724409448818898682, 2.892866454678787531E-17, -0.9822834645669291653 ) ) ;
#18378=ORIENTED_EDGE ( 'NONE', *, *, #27425, .F. ) ;
#18379=CARTESIAN_POINT ( 'NONE',  ( 0.3460692066303958092, 0.1998031496062993018, -1.782808398950131101 ) ) ;
#18387=CARTESIAN_POINT ( 'NONE',  ( 0.1070741851644053527, 0.3996062992125985480, -0.5426509186351704539 ) ) ;
#18388=CARTESIAN_POINT ( 'NONE',  ( 0.1070741851644053527, 0.3996062992125986590, -1.095800524934382958 ) ) ;
#18389=CARTESIAN_POINT ( 'NONE',  ( -0.1974969037888706647, 0.3420746716998658843, -0.3280839895013124563 ) ) ;
#18395=CARTESIAN_POINT ( 'NONE',  ( 0.1058382717557499880, 0.3949938075777409408, -1.487532808398950523 ) ) ;
#18400=CARTESIAN_POINT ( 'NONE',  ( -0.2362204724409447953, -0.4091458600556404646, -1.640419947506561726 ) ) ;
#18413=CARTESIAN_POINT ( 'NONE',  ( 0.1958661417322836440, -0.3392501089628017219, -1.343832020997375531 ) ) ;
#18415=VERTEX_POINT ( 'NONE', #11946 ) ;
#18416=CARTESIAN_POINT ( 'NONE',  ( -0.3949938075777411628, 0.1058382717557497937, -1.607611548556430847 ) ) ;
#18423=CARTESIAN_POINT ( 'NONE',  ( 0.1070741851644053527, 0.3996062992125986590, -0.1509186351706036655 ) ) ;
#18436=CARTESIAN_POINT ( 'NONE',  ( -0.3460692066303958092, -0.1998031496062994683, -2.099737532808398921 ) ) ;
#18439=CARTESIAN_POINT ( 'NONE',  ( 0.3460692066303959202, -0.1998031496062991630, -1.441601049868766582 ) ) ;
#18443=CARTESIAN_POINT ( 'NONE',  ( -0.4724409448818898682, -8.678599364036362592E-17, -0.8267716535433070613 ) ) ;
#18445=CARTESIAN_POINT ( 'NONE',  ( -0.3917322834645669549, -0.1049643490035306603, -2.807742782152229832 ) ) ;
#18451=CARTESIAN_POINT ( 'NONE',  ( -1.157146581871515012E-16, 0.4724409448818898682, -2.596456692913385655 ) ) ;
#18453=CARTESIAN_POINT ( 'NONE',  ( -0.3420746716998660508, -0.1974969037888706924, -2.176509186351706759 ) ) ;
#18458=CARTESIAN_POINT ( 'NONE',  ( 0.1265901696524990572, -0.4724409448818897017, -2.209317585301837195 ) ) ;
#18466=FACE_OUTER_BOUND ( 'NONE', #10958, .T. ) ;
#18474=CARTESIAN_POINT ( 'NONE',  ( -0.3996062992125986590, 0.1070741851644051723, -0.8969816272965877024 ) ) ;
#18476=CARTESIAN_POINT ( 'NONE',  ( -0.1049643490035302024, -0.3917322834645671215, -2.361548556430446144 ) ) ;
#18491=CARTESIAN_POINT ( 'NONE',  ( 0.3392501089628018329, 0.1958661417322835607, -1.948162729658792891 ) ) ;
#18492=CARTESIAN_POINT ( 'NONE',  ( -0.3527845929029426175, 0.1716039559346188292, -1.220472440944881720 ) ) ;
#18498=CARTESIAN_POINT ( 'NONE',  ( -0.1998031496062991907, -0.3460692066303959757, -0.8530183727034120755 ) ) ;
#18500=CARTESIAN_POINT ( 'NONE',  ( 0.2867679344610365999, -0.2867679344610365444, -2.767716535433069946 ) ) ;
#18512=CARTESIAN_POINT ( 'NONE',  ( -0.2867679344610364334, -0.2867679344610367109, -0.2086614173228345248 ) ) ;
#18515=CARTESIAN_POINT ( 'NONE',  ( -0.2891555358219911054, 0.2891555358219909388, -0.1771653543307087630 ) ) ;
#18522=CARTESIAN_POINT ( 'NONE',  ( 0.2867679344610366554, -0.2867679344610365999, -1.827447137304149205 ) ) ;
#18524=CARTESIAN_POINT ( 'NONE',  ( 0.1049643490035304938, -0.3917322834645669549, -2.689632545931758489 ) ) ;
#18529=CARTESIAN_POINT ( 'NONE',  ( 0.1070741851644054915, -0.3996062992125986035, -0.7152230971128609172 ) ) ;
#18531=CARTESIAN_POINT ( 'NONE',  ( -0.3996062992125984925, -0.1070741851644056858, -0.2801837270341207553 ) ) ;
#18532=CARTESIAN_POINT ( 'NONE',  ( 0.2925321140481932369, -0.2925321140481931814, -0.1751968503937008370 ) ) ;
#18534=CARTESIAN_POINT ( 'NONE',  ( 4.893765752498283924E-17, -0.3996062992125986035, -2.755905511811023612 ) ) ;
#18535=CARTESIAN_POINT ( 'NONE',  ( 0.2867679344610365999, -0.2867679344610365444, -1.757874015748031260 ) ) ;
#18540=CARTESIAN_POINT ( 'NONE',  ( -0.4724409448818899238, 0.1265901696524986686, -1.684383202099737353 ) ) ;
#18543=CARTESIAN_POINT ( 'NONE',  ( 0.1058382717557499880, 0.3949938075777409408, -1.015091863517060489 ) ) ;
#18552=CARTESIAN_POINT ( 'NONE',  ( 0.1070741851644054776, -0.3996062992125984925, -1.579396325459317740 ) ) ;
#18568=CARTESIAN_POINT ( 'NONE',  ( -0.1958661417322836718, 0.3392501089628017219, -1.200131233595800540 ) ) ;
#18571=DIRECTION ( 'NONE',  ( 1.000000000000000000, 0.000000000000000000, -0.000000000000000000 ) ) ;
#18583=CARTESIAN_POINT ( 'NONE',  ( 0.4724409448818898682, 2.892866454678787531E-17, -0.5905511811023621549 ) ) ;
#18591=CARTESIAN_POINT ( 'NONE',  ( -0.2362204724409447953, -0.4091458600556404646, -0.2230971128608923715 ) ) ;
#18592=CARTESIAN_POINT ( 'NONE',  ( -0.3949938075777409963, -7.255918531996591613E-17, -2.716535433070866201 ) ) ;
#18595=CARTESIAN_POINT ( 'NONE',  ( 0.3917322834645669549, 0.1049643490035304660, -1.376640419947506189 ) ) ;
#18597=CARTESIAN_POINT ( 'NONE',  ( 0.4724409448818898682, 2.892866454678787531E-17, -2.795275590551181022 ) ) ;
#18604=CARTESIAN_POINT ( 'NONE',  ( -0.3917322834645669549, -7.196005306013483243E-17, -0.5918442012785283257 ) ) ;
#18610=ORIENTED_EDGE ( 'NONE', *, *, #71325, .T. ) ;
#18611=CARTESIAN_POINT ( 'NONE',  ( -0.3917322834645671770, 0.1049643490035302024, -2.234271284285776371 ) ) ;
#18618=CARTESIAN_POINT ( 'NONE',  ( -9.594673741351313045E-17, 0.3917322834645670104, -1.501968503937008093 ) ) ;
#18627=CARTESIAN_POINT ( 'NONE',  ( -0.2867679344610365999, 0.2867679344610364889, -2.846456692913385655 ) ) ;
#18629=ORIENTED_EDGE ( 'NONE', *, *, #55872, .F. ) ;
#18634=CARTESIAN_POINT ( 'NONE',  ( 0.2867679344610365999, -0.2867679344610365444, -1.127952755905512028 ) ) ;
#18635=CARTESIAN_POINT ( 'NONE',  ( -0.3458507752293906723, -0.3458507752293910609, 0.02165354330708659653 ) ) ;
#18638=CARTESIAN_POINT ( 'NONE',  ( 0.1070741851644054776, -0.3996062992125984925, -2.681758530183727895 ) ) ;
#18647=CARTESIAN_POINT ( 'NONE',  ( 0.3996062992125985480, 2.446882876249141654E-17, -0.6673228346456693272 ) ) ;
#18649=CARTESIAN_POINT ( 'NONE',  ( 0.3917322834645670104, 2.398668435337828261E-17, -0.4251968503937007537 ) ) ;
#18663=CARTESIAN_POINT ( 'NONE',  ( 0.1049643490035303967, 0.3917322834645670659, -0.7775783708999494115 ) ) ;
#18667=CARTESIAN_POINT ( 'NONE',  ( 0.4724409448818898682, 2.892866454678787531E-17, -2.557086614173228689 ) ) ;
#18688=CARTESIAN_POINT ( 'NONE',  ( -0.2925321140481930704, -0.2925321140481933480, -0.2165354330708661734 ) ) ;
#18689=CARTESIAN_POINT ( 'NONE',  ( -0.1998031496062991630, -0.3460692066303959202, -2.819553805774277944 ) ) ;
#18695=CARTESIAN_POINT ( 'NONE',  ( 0.1998031496062992740, 0.3460692066303959757, -2.034120734908136718 ) ) ;
#18696=CARTESIAN_POINT ( 'NONE',  ( 0.3949938075777409408, 0.1058382717557500574, -1.541994750656168200 ) ) ;
#18697=CARTESIAN_POINT ( 'NONE',  ( 0.3996062992125986035, 2.446882876249141962E-17, -2.952755905511811108 ) ) ;
#18699=CARTESIAN_POINT ( 'NONE',  ( -0.1049643490035301885, -0.3917322834645671215, -0.6942257217847767059 ) ) ;
#18702=CARTESIAN_POINT ( 'NONE',  ( 0.1974969037888704704, 0.3420746716998660508, -2.425853018372703396 ) ) ;
#18707=CARTESIAN_POINT ( 'NONE',  ( 0.1070741851644053527, 0.3996062992125986590, -2.040682414698162361 ) ) ;
#18714=CARTESIAN_POINT ( 'NONE',  ( 0.2867679344610365999, -0.2867679344610365444, -0.3405511811023621549 ) ) ;
#18720=CARTESIAN_POINT ( 'NONE',  ( 0.3917322834645669549, 0.1049643490035304660, -0.3667979002624672802 ) ) ;
#18721=CARTESIAN_POINT ( 'NONE',  ( 0.3917322834645670104, -0.1049643490035303411, -1.520997375328083656 ) ) ;
#18722=CARTESIAN_POINT ( 'NONE',  ( -0.2867679344610364334, -0.2867679344610367109, -2.728346456692912536 ) ) ;
#18724=CARTESIAN_POINT ( 'NONE',  ( -0.1070741851644051862, -0.3996062992125987146, -0.07217847769028871985 ) ) ;
#18728=CARTESIAN_POINT ( 'NONE',  ( 4.893765752498283924E-17, -0.3996062992125986035, -1.496062992125984259 ) ) ;
#18733=CARTESIAN_POINT ( 'NONE',  ( 0.3917322834645670104, 2.398668435337828261E-17, -0.5177165354330709457 ) ) ;
#18741=CARTESIAN_POINT ( 'NONE',  ( 0.2362204724409449064, 0.4091458600556404646, -2.191601049868766360 ) ) ;
#18751=CARTESIAN_POINT ( 'NONE',  ( 0.2867679344610365999, -0.2867679344610365999, -0.4934190044281346332 ) ) ;
#18753=CARTESIAN_POINT ( 'NONE',  ( -0.1049643490035307020, 0.3917322834645669549, -0.7211286089238846397 ) ) ;
#18758=CARTESIAN_POINT ( 'NONE',  ( -9.594673741351313045E-17, 0.3917322834645670659, 0.1607418390738039049 ) ) ;
#18760=EDGE_CURVE ( 'NONE', #79206, #58800, #19931, .T. ) ;
#18762=CARTESIAN_POINT ( 'NONE',  ( 0.4091458600556403535, 0.2362204724409449896, -1.310367454068241511 ) ) ;
#18769=DIRECTION ( 'NONE',  ( 1.000000000000000000, 0.000000000000000000, 0.000000000000000000 ) ) ;
#18774=CARTESIAN_POINT ( 'NONE',  ( -0.2925321140481930149, -0.2925321140481933480, -2.340551181102362488 ) ) ;
#18778=CARTESIAN_POINT ( 'NONE',  ( 0.3460692066303958092, 0.1998031496062993018, -1.310367454068241733 ) ) ;
#18784=CARTESIAN_POINT ( 'NONE',  ( -0.2925321140481932369, 0.2925321140481930704, -0.7263779527559055538 ) ) ;
#18785=CARTESIAN_POINT ( 'NONE',  ( -0.3996062992125986035, -7.340648628747425578E-17, -1.141732283464566899 ) ) ;
#18786=CARTESIAN_POINT ( 'NONE',  ( -0.3420746716998659953, -0.1974969037888706647, -0.2099737532808399476 ) ) ;
#18792=CARTESIAN_POINT ( 'NONE',  ( 0.2891555358219910499, 0.2891555358219910499, -1.316929133858267598 ) ) ;
#18798=CARTESIAN_POINT ( 'NONE',  ( 0.3458507752293908943, 0.3458507752293908943, -1.712598425196850460 ) ) ;
#18799=CARTESIAN_POINT ( 'NONE',  ( -0.3996062992125986035, -7.340648628747425578E-17, -2.716535433070865757 ) ) ;
#18806=CARTESIAN_POINT ( 'NONE',  ( -0.2867679344610364334, -0.2867679344610368219, -1.871371760333646606 ) ) ;
#18812=CARTESIAN_POINT ( 'NONE',  ( 0.3392501089628018884, -0.1958661417322834220, -1.514435695538058013 ) ) ;
#18815=CARTESIAN_POINT ( 'NONE',  ( -0.2891555358219911054, 0.2891555358219909388, -1.751968503937008093 ) ) ;
#18820=CARTESIAN_POINT ( 'NONE',  ( 0.3460692066303959757, -0.1998031496062991907, -0.2624671916010498651 ) ) ;
#18828=CARTESIAN_POINT ( 'NONE',  ( 0.1958661417322836440, -0.3392501089628017219, 0.1384514435695537171 ) ) ;
#18836=CARTESIAN_POINT ( 'NONE',  ( 0.3460692066303958092, 0.1998031496062993018, -1.467847769028871596 ) ) ;
#18841=CARTESIAN_POINT ( 'NONE',  ( -0.4091458600556402980, -0.2362204724409451284, -0.9973753280839895430 ) ) ;
#18843=CARTESIAN_POINT ( 'NONE',  ( 0.1958661417322836440, -0.3392501089628017219, 0.07349081364829400387 ) ) ;
#18845=CARTESIAN_POINT ( 'NONE',  ( -0.3917322834645670104, -7.196005306013484475E-17, -2.171259842519685179 ) ) ;
#18849=CARTESIAN_POINT ( 'NONE',  ( 0.2362204724409449064, 0.4091458600556404646, -2.740813648293963567 ) ) ;
#18852=CARTESIAN_POINT ( 'NONE',  ( -0.3949938075777408852, -0.1058382717557502933, -2.327427821522309870 ) ) ;
#18861=CARTESIAN_POINT ( 'NONE',  ( -0.4724409448818898682, -8.678599364036362592E-17, 0.1988188976377952832 ) ) ;
#18873=CARTESIAN_POINT ( 'NONE',  ( 0.3996062992125986035, -0.1070741851644052972, -0.9757217847769029673 ) ) ;
#18874=CARTESIAN_POINT ( 'NONE',  ( 0.3392501089628018884, -0.1958661417322834220, -2.236876640419947826 ) ) ;
#18883=CARTESIAN_POINT ( 'NONE',  ( -0.2362204724409447953, -0.4091458600556404646, -0.6955380577427822120 ) ) ;
#18884=CARTESIAN_POINT ( 'NONE',  ( 0.1049643490035304799, -0.3917322834645670104, -2.129284407645356314 ) ) ;
#18890=CARTESIAN_POINT ( 'NONE',  ( 0.1958661417322834775, 0.3392501089628018884, -1.803805774278215202 ) ) ;
#18897=CARTESIAN_POINT ( 'NONE',  ( 0.3996062992125986035, 2.446882876249141962E-17, -1.535433070866141669 ) ) ;
#18899=CARTESIAN_POINT ( 'NONE',  ( 4.797336870675656522E-17, -0.3917322834645670104, -2.905511811023621771 ) ) ;
#18912=CARTESIAN_POINT ( 'NONE',  ( -0.1958661417322836718, 0.3392501089628017219, -0.005249343832020950465 ) ) ;
#18915=CARTESIAN_POINT ( 'NONE',  ( -0.3949938075777411628, 0.1058382717557497937, -0.03280839895013128865 ) ) ;
#18918=CARTESIAN_POINT ( 'NONE',  ( -0.3458507752293909498, 0.3458507752293908388, -0.1771653543307086520 ) ) ;
#18923=CARTESIAN_POINT ( 'NONE',  ( 0.3917322834645670104, 0.1049643490035304660, -1.538733226542994048 ) ) ;
#18925=CARTESIAN_POINT ( 'NONE',  ( -0.1958661417322836718, 0.3392501089628017219, -2.774934383202099841 ) ) ;
#18930=CARTESIAN_POINT ( 'NONE',  ( 4.893765752498283924E-17, -0.3996062992125986035, -0.8661417322834645827 ) ) ;
#18932=CARTESIAN_POINT ( 'NONE',  ( 0.2925321140481932369, 0.2925321140481932369, -0.5295275590551181688 ) ) ;
#18933=CARTESIAN_POINT ( 'NONE',  ( 0.3996062992125984925, 0.1070741851644054637, -0.2014435695538057958 ) ) ;
#18935=CARTESIAN_POINT ( 'NONE',  ( -0.3996062992125986035, -0.1070741851644056997, -2.565616797900262647 ) ) ;
#18936=CARTESIAN_POINT ( 'NONE',  ( -0.3392501089628017219, -0.1958661417322836718, -1.869422572178477848 ) ) ;
#18941=CARTESIAN_POINT ( 'NONE',  ( 0.3458507752293908943, 0.3458507752293908943, -1.474409448818897683 ) ) ;
#18944=CARTESIAN_POINT ( 'NONE',  ( 0.3420746716998660508, -0.1974969037888704149, -0.9691601049868767692 ) ) ;
#18954=CARTESIAN_POINT ( 'NONE',  ( 0.3996062992125986035, -0.1070741851644052972, -2.078083989501312345 ) ) ;
#18968=CARTESIAN_POINT ( 'NONE',  ( 4.797336870675656522E-17, -0.3917322834645670104, -0.9507874015748032370 ) ) ;
#18985=CARTESIAN_POINT ( 'NONE',  ( -0.1265901696524986964, -0.4724409448818899238, -0.5446194225721784354 ) ) ;
#18992=CARTESIAN_POINT ( 'NONE',  ( -0.2362204724409451284, 0.4091458600556402425, -0.3280839895013123453 ) ) ;
#18993=CARTESIAN_POINT ( 'NONE',  ( 0.3996062992125986035, 2.446882876249141962E-17, -0.1181102362204724671 ) ) ;
#18996=CARTESIAN_POINT ( 'NONE',  ( -0.3392501089628017219, -0.1958661417322836718, -1.304461942257217899 ) ) ;
#18998=CARTESIAN_POINT ( 'NONE',  ( 0.2362204724409451007, -0.4091458600556402980, -2.769028871391076230 ) ) ;
#19005=CARTESIAN_POINT ( 'NONE',  ( -0.3392501089628018329, -0.1958661417322836440, -0.7624478758192109185 ) ) ;
#19013=CARTESIAN_POINT ( 'NONE',  ( 0.3917322834645670104, 0.1049643490035304660, -1.853693856464253997 ) ) ;
#19021=CARTESIAN_POINT ( 'NONE',  ( -0.3917322834645670104, -7.196005306013484475E-17, -1.383858267716535417 ) ) ;
#19030=CARTESIAN_POINT ( 'NONE',  ( 0.3917322834645670104, -0.1049643490035303411, -2.938320209973753538 ) ) ;
#19036=DIRECTION ( 'NONE',  ( 1.000000000000000000, 0.000000000000000000, 0.000000000000000000 ) ) ;
#19037=CARTESIAN_POINT ( 'NONE',  ( -9.594673741351313045E-17, 0.3917322834645670104, -1.187007874015748143 ) ) ;
#19038=CARTESIAN_POINT ( 'NONE',  ( -0.4724409448818898682, -8.678599364036362592E-17, -0.1161417322834645827 ) ) ;
#19041=CARTESIAN_POINT ( 'NONE',  ( -0.3949938075777408852, -0.1058382717557502933, 0.1922572178477690297 ) ) ;
#19046=CARTESIAN_POINT ( 'NONE',  ( 0.3949938075777409963, 2.418639510665530743E-17, -0.1948818897637795700 ) ) ;
#19053=CARTESIAN_POINT ( 'NONE',  ( 0.3996062992125984925, 0.1070741851644054637, -0.9888451443569553634 ) ) ;
#19055=CARTESIAN_POINT ( 'NONE',  ( -0.3392501089628017219, -0.1958661417322836718, -0.04461942257217842850 ) ) ;
#19068=CARTESIAN_POINT ( 'NONE',  ( -0.1049643490035302301, -0.3917322834645671770, -0.8563185283802644543 ) ) ;
#19072=CARTESIAN_POINT ( 'NONE',  ( -0.3458507752293909498, 0.3458507752293907833, -2.616141732283464805 ) ) ;
#19090=CARTESIAN_POINT ( 'NONE',  ( -0.3996062992125986590, 0.1070741851644051862, -0.3477690288713910505 ) ) ;
#19091=CARTESIAN_POINT ( 'NONE',  ( 0.1070741851644054776, -0.3996062992125984925, -2.681758530183727895 ) ) ;
#19096=CARTESIAN_POINT ( 'NONE',  ( 4.893765752498283924E-17, -0.3996062992125986035, -2.125984251968504157 ) ) ;
#19097=CARTESIAN_POINT ( 'NONE',  ( -0.1058382717557503211, 0.3949938075777409408, -1.581364829396325389 ) ) ;
#19098=CARTESIAN_POINT ( 'NONE',  ( -0.3996062992125986035, -0.1070741851644056997, -2.723097112860892288 ) ) ;
#19100=CARTESIAN_POINT ( 'NONE',  ( -0.2867679344610366554, 0.2867679344610365444, -1.114173228346456490 ) ) ;
#19104=CARTESIAN_POINT ( 'NONE',  ( -0.3420746716998660508, -0.1974969037888706924, -2.648950131233596128 ) ) ;
#19108=CARTESIAN_POINT ( 'NONE',  ( 0.4724409448818898682, 2.892866454678787531E-17, -2.952755905511811108 ) ) ;
#19109=CARTESIAN_POINT ( 'NONE',  ( -0.2925321140481932924, 0.2925321140481931814, -2.066929133858267154 ) ) ;
#19115=CARTESIAN_POINT ( 'NONE',  ( -0.2867679344610364334, -0.2867679344610367109, 0.01377952755905502598 ) ) ;
#19123=CARTESIAN_POINT ( 'NONE',  ( 4.797336870675656522E-17, -0.3917322834645670104, -0.6358267716535433989 ) ) ;
#19124=CARTESIAN_POINT ( 'NONE',  ( -0.1049643490035302024, -0.3917322834645671215, -1.639107611548556109 ) ) ;
#19125=CARTESIAN_POINT ( 'NONE',  ( -0.1049643490035302024, -0.3917322834645671215, -2.741469816272964710 ) ) ;
#19127=CARTESIAN_POINT ( 'NONE',  ( -0.2925321140481932924, 0.2925321140481931814, -0.01968503937007875723 ) ) ;
#19131=CARTESIAN_POINT ( 'NONE',  ( -0.2925321140481930704, -0.2925321140481933480, -1.318897637795275690 ) ) ;
#19133=CARTESIAN_POINT ( 'NONE',  ( 0.4724409448818897017, 0.1265901696524990294, -2.406167979002624246 ) ) ;
#19136=CARTESIAN_POINT ( 'NONE',  ( 0.1958661417322836440, -0.3392501089628017219, -0.6489501312335959060 ) ) ;
#19142=ORIENTED_EDGE ( 'NONE', *, *, #29607, .T. ) ;
#19145=CARTESIAN_POINT ( 'NONE',  ( -0.4091458600556402980, -0.2362204724409451284, -2.099737532808398921 ) ) ;
#19155=CARTESIAN_POINT ( 'NONE',  ( -9.594673741351310580E-17, 0.3917322834645669549, -0.7099544374990010009 ) ) ;
#19158=CARTESIAN_POINT ( 'NONE',  ( 0.1958661417322836440, -0.3392501089628017219, -0.6489501312335959060 ) ) ;
#19163=CARTESIAN_POINT ( 'NONE',  ( -9.594673741351313045E-17, 0.3917322834645670104, -2.669291338582676865 ) ) ;
#19165=EDGE_CURVE ( 'NONE', #56613, #48835, #80168, .T. ) ;
#19166=EDGE_CURVE ( 'NONE', #25602, #24503, #61112, .T. ) ;
#19168=CARTESIAN_POINT ( 'NONE',  ( 0.4091458600556403535, 0.2362204724409449896, -1.152887139107611425 ) ) ;
#19175=CYLINDRICAL_SURFACE ( 'NONE', #39389, 0.4724409448818898682 ) ;
#19180=CARTESIAN_POINT ( 'NONE',  ( 0.3996062992125986035, -0.1070741851644052972, -2.393044619422572072 ) ) ;
#19184=CARTESIAN_POINT ( 'NONE',  ( -0.2925321140481930149, -0.2925321140481933480, -1.553149606299212726 ) ) ;
#19190=CARTESIAN_POINT ( 'NONE',  ( 0.3460692066303958092, 0.1998031496062993018, -0.6804461942257218343 ) ) ;
#19191=CARTESIAN_POINT ( 'NONE',  ( 0.3460692066303959757, -0.1998031496062991907, -0.7349081364829396223 ) ) ;
#19192=CARTESIAN_POINT ( 'NONE',  ( 0.1058382717557499880, 0.3949938075777411073, -0.3083989501312336956 ) ) ;
#19198=CARTESIAN_POINT ( 'NONE',  ( -0.3458507752293906723, -0.3458507752293910609, -2.340551181102362488 ) ) ;
#19199=CARTESIAN_POINT ( 'NONE',  ( 0.3949938075777409963, 2.418639510665530743E-17, -1.454724409448818756 ) ) ;
#19204=CARTESIAN_POINT ( 'NONE',  ( -1.157146581871515012E-16, 0.4724409448818898682, -1.574803149606299302 ) ) ;
#19213=CARTESIAN_POINT ( 'NONE',  ( -0.1958661417322836440, 0.3392501089628016664, -2.140400631724722835 ) ) ;
#19219=CARTESIAN_POINT ( 'NONE',  ( -0.2867679344610365999, 0.2867679344610364889, -1.429133858267716661 ) ) ;
#19222=CARTESIAN_POINT ( 'NONE',  ( -0.1974969037888706647, 0.3420746716998658843, -1.745406824146981339 ) ) ;
#19227=CARTESIAN_POINT ( 'NONE',  ( 0.3996062992125986035, 2.446882876249141962E-17, -0.2755905511811023723 ) ) ;
#19234=CARTESIAN_POINT ( 'NONE',  ( -0.3392501089628017219, -0.1958661417322836718, -0.4520997375328084655 ) ) ;
#19241=CARTESIAN_POINT ( 'NONE',  ( -0.3996062992125986590, 0.1070741851644051723, -1.841863517060367439 ) ) ;
#19246=CARTESIAN_POINT ( 'NONE',  ( 0.4724409448818896462, 0.1265901696524990294, -0.9120734908136483021 ) ) ;
#19248=CARTESIAN_POINT ( 'NONE',  ( -0.1049643490035307020, 0.3917322834645669549, 0.001312335958005295946 ) ) ;
#19249=CARTESIAN_POINT ( 'NONE',  ( -0.3917322834645671215, 0.1049643490035301469, -2.164698162729658648 ) ) ;
#19253=CARTESIAN_POINT ( 'NONE',  ( -0.1265901696524993347, 0.4724409448818895907, -2.760498687664041384 ) ) ;
#19257=CARTESIAN_POINT ( 'NONE',  ( 0.3949938075777409408, -0.1058382717557499186, -2.708005249343832244 ) ) ;
#19265=CARTESIAN_POINT ( 'NONE',  ( -0.3392501089628017219, -0.1958661417322836718, -1.304461942257217899 ) ) ;
#19268=CARTESIAN_POINT ( 'NONE',  ( -0.3458507752293906723, -0.3458507752293910609, -0.1358267716535432879 ) ) ;
#19282=CARTESIAN_POINT ( 'NONE',  ( -0.3460692066303960313, 0.1998031496062989965, -1.047900262467191590 ) ) ;
#19283=CARTESIAN_POINT ( 'NONE',  ( 0.1049643490035304938, -0.3917322834645669549, -2.532152230971127960 ) ) ;
#19295=CARTESIAN_POINT ( 'NONE',  ( -0.1049643490035307158, 0.3917322834645670104, -2.050544250165041493 ) ) ;
#19302=CARTESIAN_POINT ( 'NONE',  ( -0.3392501089628019995, 0.1958661417322832277, -2.158136482939632561 ) ) ;
#19307=CARTESIAN_POINT ( 'NONE',  ( -0.1998031496062994405, 0.3460692066303957537, -2.609580052493438274 ) ) ;
#19309=CARTESIAN_POINT ( 'NONE',  ( -0.3996062992125986035, -0.1070741851644056997, -1.305774278215223072 ) ) ;
#19311=CARTESIAN_POINT ( 'NONE',  ( -9.594673741351313045E-17, 0.3917322834645670659, 0.003261524113173961108 ) ) ;
#19327=CARTESIAN_POINT ( 'NONE',  ( -0.1958661417322836718, 0.3392501089628017219, -0.3202099737532808077 ) ) ;
#19330=CARTESIAN_POINT ( 'NONE',  ( -0.1974969037888706647, 0.3420746716998658843, -0.6430446194225721834 ) ) ;
#19333=CARTESIAN_POINT ( 'NONE',  ( -0.4091458600556405756, 0.2362204724409446288, -0.1837270341207349056 ) ) ;
#19339=CARTESIAN_POINT ( 'NONE',  ( -0.2867679344610365444, -0.2867679344610367664, -1.788077058563991795 ) ) ;
#19345=CARTESIAN_POINT ( 'NONE',  ( -0.3460692066303958092, -0.1998031496062994683, -1.154855643044619518 ) ) ;
#19347=CARTESIAN_POINT ( 'NONE',  ( 4.893765752498283308E-17, -0.3996062992125985480, -0.7854330708661416693 ) ) ;
#19348=CARTESIAN_POINT ( 'NONE',  ( -0.1998031496062994405, 0.3460692066303957537, -0.2473753280839895152 ) ) ;
#19350=CARTESIAN_POINT ( 'NONE',  ( -9.787531504996567848E-17, 0.3996062992125986035, -2.519685039370078705 ) ) ;
#19352=CARTESIAN_POINT ( 'NONE',  ( -0.3392501089628019995, 0.1958661417322832277, -1.685695538057742970 ) ) ;
#19358=CARTESIAN_POINT ( 'NONE',  ( 0.3458507752293908943, 0.3458507752293908943, -1.631889763779527325 ) ) ;
#19361=CARTESIAN_POINT ( 'NONE',  ( 0.3949938075777409408, -0.1058382717557499186, -0.8182414698162731037 ) ) ;
#19367=LINE ( 'NONE', #76620, #60112 ) ;
#19370=CARTESIAN_POINT ( 'NONE',  ( 0.3460692066303958092, 0.1998031496062993018, -2.097769028871391050 ) ) ;
#19372=CARTESIAN_POINT ( 'NONE',  ( 0.1049643490035304522, -0.3917322834645668994, -1.740138164533121756 ) ) ;
#19384=CARTESIAN_POINT ( 'NONE',  ( -0.1070741851644051862, -0.3996062992125986590, 0.008530183727034111943 ) ) ;
#19386=CARTESIAN_POINT ( 'NONE',  ( -0.1049643490035302024, -0.3917322834645671215, -0.9442257217847768169 ) ) ;
#19390=PLANE ( 'NONE',  #73652 ) ;
#19407=CARTESIAN_POINT ( 'NONE',  ( 0.3917322834645669549, 0.1049643490035304660, -2.636482939632545541 ) ) ;
#19410=CARTESIAN_POINT ( 'NONE',  ( 0.4091458600556403535, 0.2362204724409449896, -0.6036745406824146620 ) ) ;
#19411=CARTESIAN_POINT ( 'NONE',  ( -0.2925321140481932924, 0.2925321140481931814, 0.1377952755905511584 ) ) ;
#19414=CARTESIAN_POINT ( 'NONE',  ( 0.1958661417322836440, -0.3392501089628017219, -1.973753280839895208 ) ) ;
#19424=CARTESIAN_POINT ( 'NONE',  ( -0.3917322834645668994, -0.1049643490035306742, -1.070846825950444448 ) ) ;
#19431=CARTESIAN_POINT ( 'NONE',  ( 0.3392501089628018329, 0.1958661417322835607, -2.332696481136169453 ) ) ;
#19439=CARTESIAN_POINT ( 'NONE',  ( 0.2867679344610365999, -0.2867679344610365444, -1.442913385826771755 ) ) ;
#19449=ORIENTED_EDGE ( 'NONE', *, *, #14771, .F. ) ;
#19455=CARTESIAN_POINT ( 'NONE',  ( 0.1958661417322834775, 0.3392501089628018884, -1.016404199475065662 ) ) ;
#19456=CARTESIAN_POINT ( 'NONE',  ( 0.3458507752293908943, -0.3458507752293908943, -0.3326771653543306728 ) ) ;
#19460=CARTESIAN_POINT ( 'NONE',  ( -0.3460692066303957537, -0.1998031496062994405, -2.648950131233595684 ) ) ;
#19465=CARTESIAN_POINT ( 'NONE',  ( 0.1974969037888704704, 0.3420746716998660508, 0.09383202099737533719 ) ) ;
#19472=CARTESIAN_POINT ( 'NONE',  ( -0.1070741851644056997, 0.3996062992125984925, -0.7132545931758530466 ) ) ;
#19474=CARTESIAN_POINT ( 'NONE',  ( -0.2867679344610365999, 0.2867679344610364889, -0.6417322834645668994 ) ) ;
#19476=CARTESIAN_POINT ( 'NONE',  ( 0.000000000000000000, 0.000000000000000000, -2.755905511811024056 ) ) ;
#19490=CARTESIAN_POINT ( 'NONE',  ( -0.4724409448818899238, 0.1265901696524986686, -2.314304461942256808 ) ) ;
#19506=CARTESIAN_POINT ( 'NONE',  ( -0.1070741851644057135, 0.3996062992125985480, -0.3215223097112860917 ) ) ;
#19507=CARTESIAN_POINT ( 'NONE',  ( 0.2952755905511810774, 0.000000000000000000, -1.220472440944881942 ) ) ;
#19512=CARTESIAN_POINT ( 'NONE',  ( 0.3996062992125986590, -0.1070741851644053111, -2.158792650918635037 ) ) ;
#19514=CARTESIAN_POINT ( 'NONE',  ( -9.674558042662121740E-17, 0.3949938075777409963, -2.047244094488188892 ) ) ;
#19515=CARTESIAN_POINT ( 'NONE',  ( -0.1958661417322836718, 0.3392501089628017219, -0.4776902887139107268 ) ) ;
#19517=CARTESIAN_POINT ( 'NONE',  ( 0.3392501089628018884, -0.1958661417322834220, -1.041994750656167756 ) ) ;
#19520=CARTESIAN_POINT ( 'NONE',  ( 0.3949938075777409963, 2.418639510665530743E-17, -2.714566929133857887 ) ) ;
#19524=CARTESIAN_POINT ( 'NONE',  ( 5.785732909357575061E-17, -0.4724409448818898682, -2.913385826771653697 ) ) ;
#19525=CARTESIAN_POINT ( 'NONE',  ( -0.1998031496062994683, 0.3460692066303958092, -2.532808398950130879 ) ) ;
#19526=CARTESIAN_POINT ( 'NONE',  ( -0.1049643490035307158, 0.3917322834645670104, -0.7907017304800020296 ) ) ;
#19531=CARTESIAN_POINT ( 'NONE',  ( -0.3917322834645669549, -0.1049643490035306603, 0.02690288713910752097 ) ) ;
#19539=CARTESIAN_POINT ( 'NONE',  ( 0.2867679344610365999, 0.2867679344610365999, -0.6948818897637795144 ) ) ;
#19540=CARTESIAN_POINT ( 'NONE',  ( -0.2867679344610365999, 0.2867679344610364889, -2.059055118110236116 ) ) ;
#19541=CARTESIAN_POINT ( 'NONE',  ( -0.1958661417322834220, -0.3392501089628018884, -2.892388451443569153 ) ) ;
#19543=CARTESIAN_POINT ( 'NONE',  ( 0.3460692066303959757, -0.1998031496062991907, 0.05249343832020995915 ) ) ;
#19547=CARTESIAN_POINT ( 'NONE',  ( 0.1998031496062992740, 0.3460692066303959757, -1.404199475065616820 ) ) ;
#19549=CARTESIAN_POINT ( 'NONE',  ( 0.4724409448818898682, 2.892866454678787531E-17, -0.2755905511811023723 ) ) ;
#19552=CARTESIAN_POINT ( 'NONE',  ( -0.1958661417322836718, 0.3392501089628017219, -1.042650918635170676 ) ) ;
#19561=CARTESIAN_POINT ( 'NONE',  ( 5.785732909357575061E-17, -0.4724409448818898682, -2.125984251968504157 ) ) ;
#19562=CARTESIAN_POINT ( 'NONE',  ( -1.157146581871515012E-16, 0.4724409448818898682, -2.677165354330708347 ) ) ;
#19568=EDGE_LOOP ( 'NONE', ( #43040, #31007, #55469, #65926, #12910, #911, #19142, #49775, #52868, #26137, #56373, #37975, #49891, #28631, #35273, #59296, #55935, #68851, #12924 ) ) ;
#19570=CARTESIAN_POINT ( 'NONE',  ( -0.4724409448818880364, -0.1265901696525023323, -2.642388451443570485 ) ) ;
#19573=CARTESIAN_POINT ( 'NONE',  ( 0.3917322834645668994, -0.1049643490035303134, -0.8215029939294470340 ) ) ;
#19576=CARTESIAN_POINT ( 'NONE',  ( 0.3917322834645670104, -0.1049643490035303273, -1.141076115485564202 ) ) ;
#19581=CARTESIAN_POINT ( 'NONE',  ( -0.3917322834645670104, -7.196005306013484475E-17, -2.551181102362204633 ) ) ;
#19585=CARTESIAN_POINT ( 'NONE',  ( 0.3458507752293908943, -0.3458507752293908943, -1.277559055118109965 ) ) ;
#19597=CARTESIAN_POINT ( 'NONE',  ( 0.3460692066303958092, 0.1998031496062993018, -2.255249343832020692 ) ) ;
#19601=CARTESIAN_POINT ( 'NONE',  ( -0.2925321140481930149, -0.2925321140481933480, -1.395669291338582640 ) ) ;
#19608=CARTESIAN_POINT ( 'NONE',  ( 0.1998031496062994128, -0.3460692066303957537, -0.7985564304461942875 ) ) ;
#19609=CARTESIAN_POINT ( 'NONE',  ( 0.3996062992125986590, -0.1070741851644053111, -0.7414698162729659314 ) ) ;
#19610=CARTESIAN_POINT ( 'NONE',  ( -0.3949938075777409408, -0.1058382717557502933, -0.8333333333333334814 ) ) ;
#19617=CARTESIAN_POINT ( 'NONE',  ( -0.1058382717557497660, -0.3949938075777411073, -1.251312335958005173 ) ) ;
#19622=CARTESIAN_POINT ( 'NONE',  ( 0.1265901696524989462, 0.4724409448818897572, -1.568241469816272993 ) ) ;
#19623=CARTESIAN_POINT ( 'NONE',  ( 0.3460692066303959757, -0.1998031496062991907, -2.624671916010498762 ) ) ;
#19631=CARTESIAN_POINT ( 'NONE',  ( 0.1958661417322834497, 0.3392501089628018329, -1.956673597603987957 ) ) ;
#19632=CARTESIAN_POINT ( 'NONE',  ( 0.2925321140481932369, -0.2925321140481931814, -2.852362204724409711 ) ) ;
#19639=CARTESIAN_POINT ( 'NONE',  ( 0.1958661417322836440, -0.3392501089628017219, -1.658792650918635259 ) ) ;
#19642=CARTESIAN_POINT ( 'NONE',  ( 0.3949938075777409963, 2.418639510665530435E-17, -2.007874015748031482 ) ) ;
#19647=CARTESIAN_POINT ( 'NONE',  ( 0.3460692066303959202, 0.1998031496062993295, -0.2887139107611548794 ) ) ;
#19650=CARTESIAN_POINT ( 'NONE',  ( -9.594673741351313045E-17, 0.3917322834645670104, 0.2303149606299211838 ) ) ;
#19653=CARTESIAN_POINT ( 'NONE',  ( 0.2867679344610365999, 0.2867679344610365999, -0.2224409448818898127 ) ) ;
#19660=CARTESIAN_POINT ( 'NONE',  ( 0.3460692066303959202, -0.1998031496062991630, -2.071522309711285814 ) ) ;
#19665=CARTESIAN_POINT ( 'NONE',  ( 0.4724409448818898682, 2.892866454678787531E-17, -0.7480314960629921295 ) ) ;
#19667=CARTESIAN_POINT ( 'NONE',  ( -0.3917322834645670104, -7.196005306013484475E-17, -0.3464566929133857665 ) ) ;
#19669=CARTESIAN_POINT ( 'NONE',  ( 0.1958661417322834775, 0.3392501089628018884, -1.961286089238845287 ) ) ;
#19675=CARTESIAN_POINT ( 'NONE',  ( 0.4724409448818898682, 2.892866454678787531E-17, -2.557086614173228689 ) ) ;
#19679=CARTESIAN_POINT ( 'NONE',  ( -0.3949938075777408852, -0.1058382717557502933, -2.484908136482939955 ) ) ;
#19688=CARTESIAN_POINT ( 'NONE',  ( 0.1049643490035304938, -0.3917322834645669549, -1.337270341207349000 ) ) ;
#19692=CARTESIAN_POINT ( 'NONE',  ( -0.3458507752293909498, 0.3458507752293907833, -0.09645669291338582196 ) ) ;
#19696=CARTESIAN_POINT ( 'NONE',  ( 0.4724409448818898682, 2.892866454678787531E-17, -0.6673228346456693272 ) ) ;
#19704=CARTESIAN_POINT ( 'NONE',  ( -0.1070741851644051862, -0.3996062992125986590, -0.9363517060367454459 ) ) ;
#19705=CARTESIAN_POINT ( 'NONE',  ( -0.3917322834645669549, -0.1049643490035306603, -2.650262467191601079 ) ) ;
#19714=CARTESIAN_POINT ( 'NONE',  ( -0.3996062992125986035, -0.1070741851644056997, 0.1115485564304461580 ) ) ;
#19715=CARTESIAN_POINT ( 'NONE',  ( 0.2867679344610366554, 0.2867679344610366554, -2.024297531004936701 ) ) ;
#19722=CARTESIAN_POINT ( 'NONE',  ( 0.3917322834645670104, 2.398668435337828261E-17, -1.777559055118110409 ) ) ;
#19732=CARTESIAN_POINT ( 'NONE',  ( -0.1070741851644051862, -0.3996062992125987146, -1.174540682414698001 ) ) ;
#19734=CARTESIAN_POINT ( 'NONE',  ( 0.2867679344610365999, -0.2867679344610365444, -2.925196850393700920 ) ) ;
#19749=CARTESIAN_POINT ( 'NONE',  ( -0.3917322834645669549, -0.1049643490035306603, -0.3530183727034120755 ) ) ;
#19752=CARTESIAN_POINT ( 'NONE',  ( 0.1974969037888706369, -0.3420746716998659953, -0.7217847769028871152 ) ) ;
#19760=CARTESIAN_POINT ( 'NONE',  ( -0.1958661417322833942, -0.3392501089628018884, -1.479678108432757933 ) ) ;
#19766=CARTESIAN_POINT ( 'NONE',  ( -0.2925321140481932924, 0.2925321140481931814, -1.122047244094488194 ) ) ;
#19768=CARTESIAN_POINT ( 'NONE',  ( 0.1998031496062994128, -0.3460692066303957537, -0.7985564304461942875 ) ) ;
#19769=CARTESIAN_POINT ( 'NONE',  ( 0.3996062992125984925, 0.1070741851644054637, -0.04396325459317587669 ) ) ;
#19771=CARTESIAN_POINT ( 'NONE',  ( 0.1070741851644054915, -0.3996062992125986035, -2.762467191601049255 ) ) ;
#19772=CARTESIAN_POINT ( 'NONE',  ( 0.3917322834645670104, -0.1049643490035303411, -1.928477690288713742 ) ) ;
#19778=CARTESIAN_POINT ( 'NONE',  ( 0.2362204724409449064, 0.4091458600556404646, -1.323490813648294129 ) ) ;
#19780=( BOUNDED_CURVE ( )  B_SPLINE_CURVE ( 2, ( #42983, #68678, #3053, #16526, #61537, #35039, #28719, #54382, #36676, #48069, #74597, #16940, #80505 ),
 .UNSPECIFIED., .F., .F. ) 
 B_SPLINE_CURVE_WITH_KNOTS ( ( 3, 2, 2, 2, 2, 2, 3 ),
 ( 0.1625000000000000056, 0.1666666666666666574, 0.1708333333333333370, 0.1749999999999999889, 0.1791666666666666685, 0.1833333333333333204, 0.1875000000000000000 ),
 .UNSPECIFIED. ) 
 CURVE ( )  GEOMETRIC_REPRESENTATION_ITEM ( )  RATIONAL_B_SPLINE_CURVE ( ( 1.000000000000000000, 0.9659258262890683122, 1.000000000000000000, 0.9659258262890683122, 1.000000000000000000, 0.9659258262890683122, 1.000000000000000000, 0.9659258262890683122, 1.000000000000000000, 0.9659258262890683122, 1.000000000000000000, 0.9659258262890683122, 1.000000000000000000 ) ) 
 REPRESENTATION_ITEM ( '' )  );
#19782=CARTESIAN_POINT ( 'NONE',  ( -0.2891555358219909388, -0.2891555358219912164, -1.395669291338582418 ) ) ;
#19789=DIRECTION ( 'NONE',  ( 0.000000000000000000, 0.000000000000000000, 1.000000000000000000 ) ) ;
#19793=AXIS2_PLACEMENT_3D ( 'NONE', #68704, #69529, #5546 ) ;
#19794=CARTESIAN_POINT ( 'NONE',  ( -0.2925321140481932369, 0.2925321140481931259, -2.301181102362204633 ) ) ;
#19798=CARTESIAN_POINT ( 'NONE',  ( -0.2867679344610366554, 0.2867679344610365444, -2.146962311514748478 ) ) ;
#19806=CARTESIAN_POINT ( 'NONE',  ( -0.2362204724409451284, 0.4091458600556402425, -2.375328083989501238 ) ) ;
#19810=CARTESIAN_POINT ( 'NONE',  ( -0.3996062992125986590, 0.1070741851644051723, 0.04790026246719158304 ) ) ;
#19812=CARTESIAN_POINT ( 'NONE',  ( -0.1958661417322834220, -0.3392501089628018884, -1.410104986876640654 ) ) ;
#19833=CARTESIAN_POINT ( 'NONE',  ( -0.1049643490035301885, -0.3917322834645671215, -2.269028871391076230 ) ) ;
#19836=CARTESIAN_POINT ( 'NONE',  ( 0.4091458600556403535, 0.2362204724409449896, -0.9186351706036745002 ) ) ;
#19837=CARTESIAN_POINT ( 'NONE',  ( -9.787531504996567848E-17, 0.3996062992125986035, -1.920830620545185230E-17 ) ) ;
#19840=CARTESIAN_POINT ( 'NONE',  ( -0.3917322834645670104, -7.196005306013484475E-17, -1.763779527559055094 ) ) ;
#19844=CARTESIAN_POINT ( 'NONE',  ( -0.3458507752293906723, -0.3458507752293910609, -2.893700787401574992 ) ) ;
#19851=CARTESIAN_POINT ( 'NONE',  ( 0.2867679344610365999, -0.2867679344610365999, -1.280820579231284340 ) ) ;
#19857=ORIENTED_EDGE ( 'NONE', *, *, #21817, .T. ) ;
#19858=CARTESIAN_POINT ( 'NONE',  ( 0.1049643490035304799, -0.3917322834645670104, -2.286764722605985956 ) ) ;
#19867=CARTESIAN_POINT ( 'NONE',  ( 0.3917322834645670104, 2.398668435337828261E-17, -1.620078740157480324 ) ) ;
#19882=CARTESIAN_POINT ( 'NONE',  ( -0.2362204724409447953, -0.4091458600556404646, -0.3805774278215223183 ) ) ;
#19883=CARTESIAN_POINT ( 'NONE',  ( -0.4091458600556405756, 0.2362204724409446288, -0.2604986876640419946 ) ) ;
#19887=CARTESIAN_POINT ( 'NONE',  ( 0.2891555358219910499, -0.2891555358219909944, -0.3326771653543307283 ) ) ;
#19892=ADVANCED_FACE ( 'NONE', ( #64418 ), #48907, .T. ) ;
#19893=CARTESIAN_POINT ( 'NONE',  ( -0.1974969037888706924, 0.3420746716998658843, -0.08989501312335958227 ) ) ;
#19900=CARTESIAN_POINT ( 'NONE',  ( -0.2925321140481932369, 0.2925321140481931259, -0.8838582677165351953 ) ) ;
#19902=CARTESIAN_POINT ( 'NONE',  ( 0.3917322834645670104, -0.1049643490035303411, -0.7335958005249343383 ) ) ;
#19915=CARTESIAN_POINT ( 'NONE',  ( -0.3948371832379763968, -0.006307039255732561391, -1.220472440944884163 ) ) ;
#19918=CARTESIAN_POINT ( 'NONE',  ( 5.785732909357575061E-17, -0.4724409448818898682, -2.517716535433071279 ) ) ;
#19931=B_SPLINE_CURVE_WITH_KNOTS ( 'NONE', 3,
 ( #14860, #33791, #52711, #59043, #7282, #19915, #1397, #26641, #20751, #46401, #72094, #64942, #78001, #64523, #8540, #20329, #14453, #45981 ),
 .UNSPECIFIED., .F., .F.,
 ( 4, 2, 2, 2, 2, 2, 2, 2, 4 ),
 ( 7.070062332036847214E-17, 0.001588476978679775799, 0.002382715468019628354, 0.002779834712689554631, 0.002978394335024517336, 0.003077674146191998906, 0.003127314051775739474, 0.003152134004567610191, 0.003176953957359480041 ),
 .UNSPECIFIED. ) ;
#19935=CARTESIAN_POINT ( 'NONE',  ( 0.3460692066303959202, 0.1998031496062993295, -0.4461942257217847430 ) ) ;
#19940=CARTESIAN_POINT ( 'NONE',  ( -9.787531504996567848E-17, 0.3996062992125986035, -2.519685039370078705 ) ) ;
#19941=CARTESIAN_POINT ( 'NONE',  ( -0.1974969037888703871, -0.3420746716998661063, -1.955380577427821454 ) ) ;
#19942=CARTESIAN_POINT ( 'NONE',  ( -0.3917322834645671215, 0.1049643490035301469, -0.6548556430446192955 ) ) ;
#19944=CARTESIAN_POINT ( 'NONE',  ( 4.797336870675656522E-17, -0.3917322834645670104, -0.8582677165354329896 ) ) ;
#19946=CARTESIAN_POINT ( 'NONE',  ( 0.3917322834645669549, 0.1049643490035304660, -1.061679790026246462 ) ) ;
#19948=CARTESIAN_POINT ( 'NONE',  ( -0.1049643490035306742, 0.3917322834645668994, 0.07088545751412257678 ) ) ;
#19953=CARTESIAN_POINT ( 'NONE',  ( -0.1265901696524993347, 0.4724409448818896462, -0.08333333333333334259 ) ) ;
#19954=CARTESIAN_POINT ( 'NONE',  ( -9.787531504996567848E-17, 0.3996062992125986035, -2.677165354330708347 ) ) ;
#19955=CARTESIAN_POINT ( 'NONE',  ( 0.3917322834645670659, 2.398668435337828261E-17, -1.374691231792337653 ) ) ;
#19960=CARTESIAN_POINT ( 'NONE',  ( -0.1049643490035307020, 0.3917322834645669549, -0.7211286089238846397 ) ) ;
#19968=CARTESIAN_POINT ( 'NONE',  ( -0.006303098002812318121, -0.3922539627124579931, -1.929133858267716883 ) ) ;
#19969=CARTESIAN_POINT ( 'NONE',  ( 0.1958661417322834775, 0.3392501089628018884, -1.868766404199474929 ) ) ;
#19972=CARTESIAN_POINT ( 'NONE',  ( 0.3420746716998660508, -0.1974969037888703871, -2.939632545931758489 ) ) ;
#19979=CARTESIAN_POINT ( 'NONE',  ( -0.2867679344610365999, 0.2867679344610364889, -0.7342519685039372579 ) ) ;
#19994=CARTESIAN_POINT ( 'NONE',  ( -0.3458507752293906723, -0.3458507752293910609, -2.498031496062992574 ) ) ;
#19995=CARTESIAN_POINT ( 'NONE',  ( 0.4724409448818898682, 2.892866454678787531E-17, -2.480314960629921295 ) ) ;
#19998=CARTESIAN_POINT ( 'NONE',  ( -0.3392501089628018329, -0.1958661417322836440, -0.7624478758192109185 ) ) ;
#20007=CARTESIAN_POINT ( 'NONE',  ( -0.3917322834645670104, -0.1049643490035307020, 0.1148100805436201299 ) ) ;
#20010=CARTESIAN_POINT ( 'NONE',  ( -0.4091458600556402980, -0.2362204724409451284, -1.074146981627296604 ) ) ;
#20024=CARTESIAN_POINT ( 'NONE',  ( 0.1998031496062992463, 0.3460692066303959202, -2.583333333333333481 ) ) ;
#20028=CARTESIAN_POINT ( 'NONE',  ( 0.3996062992125986035, -0.1070741851644052972, -1.920603674540682260 ) ) ;
#20034=CARTESIAN_POINT ( 'NONE',  ( 0.3460692066303958092, 0.1998031496062993018, -0.9954068241469815614 ) ) ;
#20035=CARTESIAN_POINT ( 'NONE',  ( 0.3996062992125986590, -0.1070741851644053111, -1.213910761154855189 ) ) ;
#20036=CARTESIAN_POINT ( 'NONE',  ( 0.1974969037888704704, 0.3420746716998660508, -0.6167979002624671692 ) ) ;
#20042=CARTESIAN_POINT ( 'NONE',  ( -0.1974969037888706924, 0.3420746716998658843, -1.664698162729658870 ) ) ;
#20047=CARTESIAN_POINT ( 'NONE',  ( -0.4091458600556405756, 0.2362204724409446288, -1.758530183727034180 ) ) ;
#20048=CARTESIAN_POINT ( 'NONE',  ( 0.3165741174738966324, 0.2316922116739144610, -2.755905511811024944 ) ) ;
#20055=CARTESIAN_POINT ( 'NONE',  ( 0.2867679344610365999, 0.2867679344610365999, -1.792631602853332007 ) ) ;
#20061=CARTESIAN_POINT ( 'NONE',  ( -0.1049643490035307020, 0.3917322834645669549, 0.06627296587926499727 ) ) ;
#20064=CARTESIAN_POINT ( 'NONE',  ( 4.797336870675656522E-17, -0.3917322834645670104, -1.488188976377952777 ) ) ;
#20066=ORIENTED_EDGE ( 'NONE', *, *, #16700, .T. ) ;
#20067=CARTESIAN_POINT ( 'NONE',  ( -0.3949938075777411628, 0.1058382717557497937, -1.922572178477690130 ) ) ;
#20072=CARTESIAN_POINT ( 'NONE',  ( 0.1998031496062992740, 0.3460692066303959757, -0.6167979002624671692 ) ) ;
#20082=CARTESIAN_POINT ( 'NONE',  ( -0.3392501089628019995, 0.1958661417322832277, -0.2683727034120735877 ) ) ;
#20089=CARTESIAN_POINT ( 'NONE',  ( 0.2925321140481932369, -0.2925321140481931814, -1.907480314960629197 ) ) ;
#20093=CARTESIAN_POINT ( 'NONE',  ( 0.4091458600556403535, 0.2362204724409449896, -0.7611548556430446366 ) ) ;
#20095=CARTESIAN_POINT ( 'NONE',  ( 0.3917322834645670104, 2.398668435337828261E-17, -0.4251968503937007537 ) ) ;
#20096=LINE ( 'NONE', #38611, #11637 ) ;
#20100=CARTESIAN_POINT ( 'NONE',  ( -0.3996062992125986590, 0.1070741851644051723, 0.2053805774278214813 ) ) ;
#20105=CARTESIAN_POINT ( 'NONE',  ( 4.837279021331061486E-17, -0.3949938075777409963, -2.832677165354331006 ) ) ;
#20108=CARTESIAN_POINT ( 'NONE',  ( 0.2867679344610366554, -0.2867679344610365444, -0.02559055118110245552 ) ) ;
#20114=CARTESIAN_POINT ( 'NONE',  ( -0.3917322834645669549, -0.1049643490035306603, -1.612860892388451539 ) ) ;
#20117=CARTESIAN_POINT ( 'NONE',  ( -0.4724409448818895907, -0.1265901696524993070, 0.03477690288713909672 ) ) ;
#20119=CARTESIAN_POINT ( 'NONE',  ( -0.4724409448818898682, -8.678599364036362592E-17, -1.061023622047243986 ) ) ;
#20121=CARTESIAN_POINT ( 'NONE',  ( -0.2362204724409451284, 0.4091458600556402425, -0.7198162729658792447 ) ) ;
#20130=CARTESIAN_POINT ( 'NONE',  ( 0.3996062992125985480, 2.446882876249141654E-17, -1.139763779527559029 ) ) ;
#20131=CARTESIAN_POINT ( 'NONE',  ( 0.1958661417322834775, 0.3392501089628018884, -2.748687664041994605 ) ) ;
#20140=CARTESIAN_POINT ( 'NONE',  ( -0.3917322834645670104, -0.1049643490035307020, -2.562355273787088716 ) ) ;
#20143=CARTESIAN_POINT ( 'NONE',  ( 0.01150853369506186011, -0.3951562584566668535, -5.613290098372280880E-13 ) ) ;
#20147=CARTESIAN_POINT ( 'NONE',  ( 0.2867679344610365999, 0.2867679344610365999, -2.112204724409449064 ) ) ;
#20152=CARTESIAN_POINT ( 'NONE',  ( 0.3996062992125985480, -0.1070741851644052972, -2.708005249343832244 ) ) ;
#20154=CARTESIAN_POINT ( 'NONE',  ( -0.1998031496062994683, 0.3460692066303958092, -1.272965879265091749 ) ) ;
#20156=CARTESIAN_POINT ( 'NONE',  ( 0.3392501089628018884, -0.1958661417322834220, -2.931758530183726563 ) ) ;
#20167=CARTESIAN_POINT ( 'NONE',  ( 0.1049643490035304938, -0.3917322834645669549, -0.07742782152230966164 ) ) ;
#20170=CARTESIAN_POINT ( 'NONE',  ( 0.3949938075777409408, 0.1058382717557500574, -0.4396325459317587114 ) ) ;
#20184=CARTESIAN_POINT ( 'NONE',  ( -0.3460692066303960868, 0.1998031496062990242, -1.443569553805774230 ) ) ;
#20186=CARTESIAN_POINT ( 'NONE',  ( -0.1998031496062994405, 0.3460692066303957537, -0.5623359580052492701 ) ) ;
#20187=CARTESIAN_POINT ( 'NONE',  ( -0.3996062992125984925, -0.1070741851644056858, -0.1227034120734908501 ) ) ;
#20189=CARTESIAN_POINT ( 'NONE',  ( 4.893765752498283924E-17, -0.3996062992125986035, -2.598425196850393970 ) ) ;
#20190=CARTESIAN_POINT ( 'NONE',  ( 0.3392501089628018884, -0.1958661417322834220, -2.079396325459317740 ) ) ;
#20196=CARTESIAN_POINT ( 'NONE',  ( 0.4724409448818898682, 2.892866454678787531E-17, -1.454724409448818756 ) ) ;
#20199=CARTESIAN_POINT ( 'NONE',  ( -0.1058382717557497660, -0.3949938075777411073, -1.251312335958005173 ) ) ;
#20205=EDGE_CURVE ( 'NONE', #49832, #34363, #9111, .T. ) ;
#20211=CARTESIAN_POINT ( 'NONE',  ( -9.787531504996566615E-17, 0.3996062992125985480, -2.281496062992125928 ) ) ;
#20214=CARTESIAN_POINT ( 'NONE',  ( -9.594673741351310580E-17, 0.3917322834645669549, -2.127277272144670217 ) ) ;
#20227=CARTESIAN_POINT ( 'NONE',  ( 0.3996062992125984925, 0.1070741851644054637, -0.04396325459317586282 ) ) ;
#20229=CARTESIAN_POINT ( 'NONE',  ( -0.1049643490035302024, -0.3917322834645671215, -1.259186351706037099 ) ) ;
#20250=CARTESIAN_POINT ( 'NONE',  ( -0.1049643490035307020, 0.3917322834645669549, -2.675853018372703396 ) ) ;
#20253=CARTESIAN_POINT ( 'NONE',  ( 0.4724409448818898682, 2.892866454678787531E-17, -0.7480314960629921295 ) ) ;
#20254=CARTESIAN_POINT ( 'NONE',  ( -0.3460692066303958092, -0.1998031496062994683, 0.1049868766404199322 ) ) ;
#20257=CARTESIAN_POINT ( 'NONE',  ( -0.1958661417322836718, 0.3392501089628017219, -1.737532808398950079 ) ) ;
#20261=CARTESIAN_POINT ( 'NONE',  ( 0.07128922432405689069, 0.3857547143408421864, -2.755905511811022279 ) ) ;
#20267=CARTESIAN_POINT ( 'NONE',  ( 0.1049643490035303689, 0.3917322834645668994, -1.018353387630234419 ) ) ;
#20273=CARTESIAN_POINT ( 'NONE',  ( 0.3392501089628018884, -0.1958661417322833942, -2.621410391897324832 ) ) ;
#20282=CARTESIAN_POINT ( 'NONE',  ( 0.3392501089628018329, 0.1958661417322835607, -1.790682414698162805 ) ) ;
#20299=CARTESIAN_POINT ( 'NONE',  ( 0.3458507752293908943, 0.3458507752293908943, -0.3720472440944882497 ) ) ;
#20302=CARTESIAN_POINT ( 'NONE',  ( 0.3949938075777409408, -0.1058382717557499186, -0.03083989501312336609 ) ) ;
#20307=CARTESIAN_POINT ( 'NONE',  ( 0.3949938075777409408, -0.1058382717557499186, -0.03083989501312336609 ) ) ;
#20314=CARTESIAN_POINT ( 'NONE',  ( 0.1070741851644053388, 0.3996062992125986035, -0.7001312335958002064 ) ) ;
#20316=CARTESIAN_POINT ( 'NONE',  ( -0.3917322834645669549, -0.1049643490035306603, -0.8254593175853015552 ) ) ;
#20329=CARTESIAN_POINT ( 'NONE',  ( -0.3977953519386773773, -0.03143970413924696006, -1.220472440944937897 ) ) ;
#20331=CARTESIAN_POINT ( 'NONE',  ( 0.2925321140481932369, -0.2925321140481931814, 0.1397637795275590289 ) ) ;
#20348=CARTESIAN_POINT ( 'NONE',  ( 0.3460692066303959757, -0.1998031496062991907, -0.5774278215223097588 ) ) ;
#20349=CARTESIAN_POINT ( 'NONE',  ( -0.4724409448818917001, 0.1265901696524956710, -1.211942257217847985 ) ) ;
#20354=CARTESIAN_POINT ( 'NONE',  ( 0.3996062992125986035, 0.1070741851644054776, -2.486876640419947382 ) ) ;
#20355=CARTESIAN_POINT ( 'NONE',  ( -0.1058382717557497937, -0.3949938075777411628, -1.961942257217847763 ) ) ;
#20356=CARTESIAN_POINT ( 'NONE',  ( -0.1958661417322834220, -0.3392501089628018884, -0.6876640419947506189 ) ) ;
#20358=CARTESIAN_POINT ( 'NONE',  ( -0.3917322834645670104, -7.196005306013484475E-17, -1.133858267716535195 ) ) ;
#20361=CARTESIAN_POINT ( 'NONE',  ( 0.2867679344610365999, -0.2867679344610365444, -1.192913385826771755 ) ) ;
#20363=CARTESIAN_POINT ( 'NONE',  ( -9.594673741351310580E-17, 0.3917322834645669549, 0.2349274522647787078 ) ) ;
#20369=CARTESIAN_POINT ( 'NONE',  ( -0.1070741851644051862, -0.3996062992125987146, -2.591863517060367439 ) ) ;
#20370=CARTESIAN_POINT ( 'NONE',  ( 0.3917322834645670659, -0.1049643490035303273, -1.368129552002311788 ) ) ;
#20376=CARTESIAN_POINT ( 'NONE',  ( 0.3917322834645670104, -0.1049643490035303411, -0.6686351706036747222 ) ) ;
#20386=CARTESIAN_POINT ( 'NONE',  ( -0.3392501089628019995, 0.1958661417322832277, -2.065616797900262647 ) ) ;
#20388=CARTESIAN_POINT ( 'NONE',  ( -9.787531504996567848E-17, 0.3996062992125986035, -0.1574803149606299746 ) ) ;
#20395=CARTESIAN_POINT ( 'NONE',  ( 0.3392501089628018329, 0.1958661417322835607, -0.8458005249343831800 ) ) ;
#20417=CARTESIAN_POINT ( 'NONE',  ( 0.1049643490035304522, -0.3917322834645668994, -0.7952562747693419087 ) ) ;
#20420=CARTESIAN_POINT ( 'NONE',  ( 0.4724409448818898682, 2.892866454678787531E-17, -0.7480314960629921295 ) ) ;
#20426=CARTESIAN_POINT ( 'NONE',  ( -0.3392501089628019995, 0.1958661417322831999, -0.1804655100075609198 ) ) ;
#20429=CARTESIAN_POINT ( 'NONE',  ( -0.3458507752293909498, 0.3458507752293907833, -1.041338582677165281 ) ) ;
#20446=CARTESIAN_POINT ( 'NONE',  ( -0.3996062992125984925, -0.1070741851644056858, -2.327427821522309426 ) ) ;
#20450=CARTESIAN_POINT ( 'NONE',  ( 0.1998031496062992463, 0.3460692066303959202, -1.953412073490813805 ) ) ;
#20456=CARTESIAN_POINT ( 'NONE',  ( -0.1070741851644057135, 0.3996062992125984925, -1.185695538057742748 ) ) ;
#20458=CARTESIAN_POINT ( 'NONE',  ( 0.3460692066303959757, -0.1998031496062991907, -1.207349081364829324 ) ) ;
#20459=CARTESIAN_POINT ( 'NONE',  ( -0.3420746716998661618, 0.1974969037888702206, -0.8136482939632546652 ) ) ;
#20465=CARTESIAN_POINT ( 'NONE',  ( -0.3949938075777409963, -7.255918531996591613E-17, -1.533464566929133577 ) ) ;
#20470=CARTESIAN_POINT ( 'NONE',  ( 0.4724409448818898682, 2.892866454678787531E-17, -1.850393700787401619 ) ) ;
#20477=CARTESIAN_POINT ( 'NONE',  ( -0.1958661417322834497, -0.3392501089628018884, -2.507854699966192147 ) ) ;
#20483=CARTESIAN_POINT ( 'NONE',  ( 0.1049643490035304522, -0.3917322834645668994, -2.685020054296901382 ) ) ;
#20485=CARTESIAN_POINT ( 'NONE',  ( -0.2867679344610365999, 0.2867679344610364889, -1.744094488188976610 ) ) ;
#20488=CARTESIAN_POINT ( 'NONE',  ( -0.3949938075777409963, -7.255918531996591613E-17, -1.929133858267716439 ) ) ;
#20493=CARTESIAN_POINT ( 'NONE',  ( 0.3996062992125986035, 0.1070741851644054776, -0.5971128608923884640 ) ) ;
#20501=CARTESIAN_POINT ( 'NONE',  ( -0.1049643490035307020, 0.3917322834645669549, -0.5636482939632546652 ) ) ;
#20513=CARTESIAN_POINT ( 'NONE',  ( -0.4091458600556402980, -0.2362204724409451284, -1.154855643044619518 ) ) ;
#20515=CARTESIAN_POINT ( 'NONE',  ( -0.3917322834645669549, -0.1049643490035306603, -0.1955380577427821009 ) ) ;
#20516=CARTESIAN_POINT ( 'NONE',  ( 0.1958661417322834775, 0.3392501089628018884, -2.591207349081364519 ) ) ;
#20520=CARTESIAN_POINT ( 'NONE',  ( 0.2925321140481932369, 0.2925321140481932369, -0.05708661417322837689 ) ) ;
#20525=CARTESIAN_POINT ( 'NONE',  ( -0.3949938075777411073, 0.1058382717557497660, -2.629265091863516979 ) ) ;
#20532=CARTESIAN_POINT ( 'NONE',  ( 0.1049643490035304938, -0.3917322834645669549, -1.967191601049868899 ) ) ;
#20536=CARTESIAN_POINT ( 'NONE',  ( -0.4091458600556402980, -0.2362204724409451284, 0.02821522309711285356 ) ) ;
#20550=CARTESIAN_POINT ( 'NONE',  ( 0.1070741851644054776, -0.3996062992125984925, -0.9494750656167976199 ) ) ;
#20552=CARTESIAN_POINT ( 'NONE',  ( -0.3392501089628019995, 0.1958661417322832277, -2.630577427821522374 ) ) ;
#20561=CARTESIAN_POINT ( 'NONE',  ( 0.2925321140481932369, 0.2925321140481932369, -0.1377952755905512139 ) ) ;
#20563=CARTESIAN_POINT ( 'NONE',  ( 0.3917322834645670659, -0.1049643490035303273, -2.627972071687351363 ) ) ;
#20569=CARTESIAN_POINT ( 'NONE',  ( 0.1958661417322834775, 0.3392501089628018884, -2.433727034120734878 ) ) ;
#20576=CARTESIAN_POINT ( 'NONE',  ( -0.1070741851644051862, -0.3996062992125987146, -1.489501312335957950 ) ) ;
#20578=CARTESIAN_POINT ( 'NONE',  ( 0.3917322834645670104, 0.1049643490035304660, 0.03606992306330520509 ) ) ;
#20589=CARTESIAN_POINT ( 'NONE',  ( 0.3392501089628018884, -0.1958661417322834220, -0.4120734908136482466 ) ) ;
#20592=CARTESIAN_POINT ( 'NONE',  ( -0.3420746716998661618, 0.1974969037888702206, -0.4986876640419948270 ) ) ;
#20608=CARTESIAN_POINT ( 'NONE',  ( -0.3996062992125987146, 0.1070741851644051862, -1.292650918635170454 ) ) ;
#20610=CARTESIAN_POINT ( 'NONE',  ( -0.2925321140481930149, -0.2925321140481933480, -0.7657480314960628531 ) ) ;
#20611=CARTESIAN_POINT ( 'NONE',  ( 0.1998031496062992463, 0.3460692066303959202, -0.5360892388451443669 ) ) ;
#20613=CARTESIAN_POINT ( 'NONE',  ( -0.4091458600556402980, -0.2362204724409451284, -0.2099737532808398921 ) ) ;
#20614=CARTESIAN_POINT ( 'NONE',  ( 0.3917322834645670104, 2.398668435337828261E-17, -2.250000000000000000 ) ) ;
#20620=CARTESIAN_POINT ( 'NONE',  ( 0.3458507752293908943, -0.3458507752293908943, -1.750000000000000222 ) ) ;
#20624=CARTESIAN_POINT ( 'NONE',  ( -0.3949938075777409963, -7.255918531996591613E-17, -1.533464566929133577 ) ) ;
#20634=CARTESIAN_POINT ( 'NONE',  ( 0.1998031496062994128, -0.3460692066303957537, -2.373359580052493367 ) ) ;
#20635=CARTESIAN_POINT ( 'NONE',  ( -0.1049643490035301746, -0.3917322834645670659, -2.199455749834958951 ) ) ;
#20647=CARTESIAN_POINT ( 'NONE',  ( -9.787531504996566615E-17, 0.3996062992125985480, 0.08070866141732283006 ) ) ;
#20650=CARTESIAN_POINT ( 'NONE',  ( 0.3392501089628018884, -0.1958661417322834220, -1.291994750656167978 ) ) ;
#20672=CARTESIAN_POINT ( 'NONE',  ( -0.2867679344610364334, -0.2867679344610367109, -2.570866141732283339 ) ) ;
#20675=CARTESIAN_POINT ( 'NONE',  ( -0.1070741851644051862, -0.3996062992125987146, -0.2296587926509186528 ) ) ;
#20679=CARTESIAN_POINT ( 'NONE',  ( 0.1049643490035304938, -0.3917322834645669549, -1.809711286089239035 ) ) ;
#20687=EDGE_CURVE ( 'NONE', #29367, #82700, #38092, .T. ) ;
#20690=CARTESIAN_POINT ( 'NONE',  ( 0.1049643490035304522, -0.3917322834645668994, -0.9527365897299718833 ) ) ;
#20695=ORIENTED_EDGE ( 'NONE', *, *, #65801, .T. ) ;
#20696=CARTESIAN_POINT ( 'NONE',  ( 4.797336870675656522E-17, -0.3917322834645670659, -2.437683357776589510 ) ) ;
#20705=CARTESIAN_POINT ( 'NONE',  ( -0.1049643490035307020, 0.3917322834645669549, -1.666010498687664043 ) ) ;
#20720=CARTESIAN_POINT ( 'NONE',  ( 0.4724409448818896462, 0.1265901696524990294, -0.3589238845144357426 ) ) ;
#20723=CARTESIAN_POINT ( 'NONE',  ( 0.1974969037888704704, 0.3420746716998660508, -0.2211286089238845842 ) ) ;
#20729=CARTESIAN_POINT ( 'NONE',  ( -0.3949938075777409963, -7.255918531996591613E-17, -0.1161417322834646104 ) ) ;
#20736=CARTESIAN_POINT ( 'NONE',  ( 0.1998031496062992463, 0.3460692066303959202, -0.8510498687664042050 ) ) ;
#20738=CARTESIAN_POINT ( 'NONE',  ( 0.3917322834645670104, 2.398668435337828261E-17, -0.5826771653543306728 ) ) ;
#20751=CARTESIAN_POINT ( 'NONE',  ( -0.3959418824714271423, -0.02190130575838673821, -1.220472440944882386 ) ) ;
#20753=CARTESIAN_POINT ( 'NONE',  ( -0.1265901696524993347, 0.4724409448818895907, -2.760498687664041384 ) ) ;
#20768=CARTESIAN_POINT ( 'NONE',  ( -0.3996062992125986590, 0.1070741851644051862, -0.8202099737532806412 ) ) ;
#20769=CARTESIAN_POINT ( 'NONE',  ( 0.1265901696524989184, 0.4724409448818898127, -1.172572178477690352 ) ) ;
#20773=CARTESIAN_POINT ( 'NONE',  ( -0.1070741851644056997, 0.3996062992125986035, -2.683727034120735322 ) ) ;
#20774=CARTESIAN_POINT ( 'NONE',  ( 0.1058382717557499880, 0.3949938075777411073, -1.883202099737532720 ) ) ;
#20775=CARTESIAN_POINT ( 'NONE',  ( 0.2867679344610365999, -0.2867679344610365444, -0.7204724409448818312 ) ) ;
#20776=CARTESIAN_POINT ( 'NONE',  ( 0.3392501089628018884, -0.1958661417322834220, -1.199475065616797842 ) ) ;
#20778=CARTESIAN_POINT ( 'NONE',  ( -0.3917322834645669549, -0.1049643490035306603, -1.297900262467191590 ) ) ;
#20780=CARTESIAN_POINT ( 'NONE',  ( 0.1958661417322834497, 0.3392501089628018329, 0.09057049688420130973 ) ) ;
#20786=CARTESIAN_POINT ( 'NONE',  ( 0.2925321140481932369, -0.2925321140481932369, -2.775590551181101429 ) ) ;
#20787=CARTESIAN_POINT ( 'NONE',  ( 4.797336870675656522E-17, -0.3917322834645670659, -1.020360523130920738 ) ) ;
#20793=CARTESIAN_POINT ( 'NONE',  ( -0.1049643490035307020, 0.3917322834645669549, -0.4061679790026246351 ) ) ;
#20802=CARTESIAN_POINT ( 'NONE',  ( -0.2867679344610364334, -0.2867679344610367109, -1.940944881889763884 ) ) ;
#20804=CARTESIAN_POINT ( 'NONE',  ( 4.893765752498283924E-17, -0.3996062992125986035, -0.5511811023622047445 ) ) ;
#20809=ADVANCED_FACE ( 'NONE', ( #50389 ), #17719, .T. ) ;
#20811=CARTESIAN_POINT ( 'NONE',  ( 5.785732909357575061E-17, -0.4724409448818898682, -1.181102362204724310 ) ) ;
#20812=CARTESIAN_POINT ( 'NONE',  ( -0.2867679344610364334, -0.2867679344610367109, -1.246062992125984481 ) ) ;
#20832=CARTESIAN_POINT ( 'NONE',  ( 0.3917322834645668994, -0.1049643490035303134, -0.6640226789688171705 ) ) ;
#20835=CARTESIAN_POINT ( 'NONE',  ( -0.3808816823641234528, 0.09156050430092053938, -1.220472440944881942 ) ) ;
#20842=CARTESIAN_POINT ( 'NONE',  ( 0.3392501089628018884, -0.1958661417322833942, -0.2592056674878758793 ) ) ;
#20845=CARTESIAN_POINT ( 'NONE',  ( 0.4724409448818896462, 0.1265901696524990294, -1.618766404199474929 ) ) ;
#20855=CARTESIAN_POINT ( 'NONE',  ( -1.157146581871515012E-16, 0.4724409448818898682, -2.124015748031495843 ) ) ;
#20863=CARTESIAN_POINT ( 'NONE',  ( 0.1998031496062994128, -0.3460692066303957537, -2.688320209973753538 ) ) ;
#20868=CARTESIAN_POINT ( 'NONE',  ( 0.1070741851644054776, -0.3996062992125984925, -1.736876640419947826 ) ) ;
#20874=CARTESIAN_POINT ( 'NONE',  ( 0.3460692066303959202, 0.1998031496062993295, -1.233595800524934338 ) ) ;
#20876=CARTESIAN_POINT ( 'NONE',  ( 0.2891555358219910499, -0.2891555358219909944, -0.7283464566929134243 ) ) ;
#20881=CARTESIAN_POINT ( 'NONE',  ( -0.1058382717557497660, -0.3949938075777411073, -1.566272965879265344 ) ) ;
#20887=CARTESIAN_POINT ( 'NONE',  ( -1.157146581871515012E-16, 0.4724409448818898682, -2.204724409448818978 ) ) ;
#20888=CARTESIAN_POINT ( 'NONE',  ( 0.2502216998114611402, -0.3021538998228294748, -2.755905511811026720 ) ) ;
#20894=CARTESIAN_POINT ( 'NONE',  ( 0.2867679344610365999, -0.2867679344610365999, -2.383182783955693829 ) ) ;
#20895=CARTESIAN_POINT ( 'NONE',  ( 0.3996062992125986035, -0.1070741851644052972, -2.865485564304462329 ) ) ;
#20900=CARTESIAN_POINT ( 'NONE',  ( -0.3917322834645670659, 0.1049643490035301607, -2.790006930937320995 ) ) ;
#20902=CARTESIAN_POINT ( 'NONE',  ( 0.2867679344610365999, -0.2867679344610365444, -1.822834645669291653 ) ) ;
#20905=CARTESIAN_POINT ( 'NONE',  ( 0.1974969037888706369, -0.3420746716998659953, -2.139107611548556331 ) ) ;
#20910=CARTESIAN_POINT ( 'NONE',  ( 0.3460692066303959202, 0.1998031496062993295, -0.4461942257217847430 ) ) ;
#20917=CARTESIAN_POINT ( 'NONE',  ( 0.1049643490035304938, -0.3917322834645669549, -0.3274278215223098143 ) ) ;
#20927=CARTESIAN_POINT ( 'NONE',  ( -0.3458507752293909498, 0.3458507752293907833, -1.279527559055118058 ) ) ;
#20929=CARTESIAN_POINT ( 'NONE',  ( 0.3392501089628018884, -0.1958661417322834220, -0.4120734908136482466 ) ) ;
#20930=CARTESIAN_POINT ( 'NONE',  ( -0.3392501089628017219, -0.1958661417322836718, -2.341863517060367439 ) ) ;
#20933=CARTESIAN_POINT ( 'NONE',  ( 0.2925321140481932369, 0.2925321140481932369, 0.1003937007874015491 ) ) ;
#20939=CARTESIAN_POINT ( 'NONE',  ( 0.3949938075777409408, -0.1058382717557499186, -2.865485564304462329 ) ) ;
#20947=CARTESIAN_POINT ( 'NONE',  ( 0.2867679344610365999, 0.2867679344610365999, -2.019685039370078261 ) ) ;
#20950=CARTESIAN_POINT ( 'NONE',  ( 0.3458507752293908943, -0.3458507752293908943, -0.1751968503937007537 ) ) ;
#20959=DIRECTION ( 'NONE',  ( 1.000000000000000000, 0.000000000000000000, 0.000000000000000000 ) ) ;
#20963=CARTESIAN_POINT ( 'NONE',  ( 0.3996062992125985480, 2.446882876249141654E-17, -1.612204724409448842 ) ) ;
#20964=CARTESIAN_POINT ( 'NONE',  ( -0.3917322834645670104, -7.196005306013484475E-17, -2.643700787401574548 ) ) ;
#20972=CARTESIAN_POINT ( 'NONE',  ( -0.1070741851644051862, -0.3996062992125987146, 0.08530183727034119923 ) ) ;
#20973=CARTESIAN_POINT ( 'NONE',  ( -0.3392501089628019995, 0.1958661417322831999, -2.542670234417010011 ) ) ;
#20978=CARTESIAN_POINT ( 'NONE',  ( 0.3392501089628018884, -0.1958661417322834220, -2.394356955380577467 ) ) ;
#20983=CARTESIAN_POINT ( 'NONE',  ( 0.1070741851644053666, 0.3996062992125986035, -2.040682414698162361 ) ) ;
#20985=CARTESIAN_POINT ( 'NONE',  ( 0.3460692066303959202, 0.1998031496062993295, -1.863517060367454015 ) ) ;
#20987=CARTESIAN_POINT ( 'NONE',  ( 0.1958661417322836718, -0.3392501089628017219, -0.4035626228684533467 ) ) ;
#20989=B_SPLINE_CURVE_WITH_KNOTS ( 'NONE', 1,
 ( #62620, #75674 ),
 .UNSPECIFIED., .F., .F.,
 ( 2, 2 ),
 ( 0.000000000000000000, 0.001849999999999997480 ),
 .UNSPECIFIED. ) ;
#21000=CARTESIAN_POINT ( 'NONE',  ( -0.2867679344610365999, 0.2867679344610364889, -0.4842519685039369248 ) ) ;
#21002=EDGE_LOOP ( 'NONE', ( #25873, #77401 ) ) ;
#21003=CARTESIAN_POINT ( 'NONE',  ( 0.1058382717557499880, 0.3949938075777411073, -0.6233595800524935893 ) ) ;
#21016=CARTESIAN_POINT ( 'NONE',  ( -0.4091458600556402980, -0.2362204724409451284, -2.729658792650918375 ) ) ;
#21020=CARTESIAN_POINT ( 'NONE',  ( 0.2925321140481932369, 0.2925321140481932369, -1.240157480314960647 ) ) ;
#21022=CARTESIAN_POINT ( 'NONE',  ( -0.3996062992125986590, 0.1070741851644051723, -0.7395013123359580609 ) ) ;
#21023=CARTESIAN_POINT ( 'NONE',  ( 0.3460692066303959202, -0.1998031496062991630, -0.6541994750656167090 ) ) ;
#21026=CARTESIAN_POINT ( 'NONE',  ( 0.4724409448818898682, 2.892866454678787531E-17, 0.03937007874015747977 ) ) ;
#21027=CARTESIAN_POINT ( 'NONE',  ( -0.2867679344610364334, -0.2867679344610367109, -2.033464566929133355 ) ) ;
#21033=CARTESIAN_POINT ( 'NONE',  ( 5.785732909357575061E-17, -0.4724409448818898682, -1.887795275590550936 ) ) ;
#21037=CARTESIAN_POINT ( 'NONE',  ( -0.1058382717557497660, -0.3949938075777411073, -1.566272965879265344 ) ) ;
#21043=CARTESIAN_POINT ( 'NONE',  ( 0.4724409448818898682, 2.892866454678787531E-17, -2.242125984251968518 ) ) ;
#21047=CARTESIAN_POINT ( 'NONE',  ( 4.893765752498283308E-17, -0.3996062992125985480, -2.517716535433071279 ) ) ;
#21049=CARTESIAN_POINT ( 'NONE',  ( -0.2867679344610364334, -0.2867679344610368219, -2.028852075294276691 ) ) ;
#21062=CARTESIAN_POINT ( 'NONE',  ( -0.2867679344610364334, -0.2867679344610367109, -1.246062992125984481 ) ) ;
#21073=CARTESIAN_POINT ( 'NONE',  ( 4.893765752498283308E-17, -0.3996062992125985480, -0.9429133858267716439 ) ) ;
#21085=CARTESIAN_POINT ( 'NONE',  ( -0.3392501089628017219, -0.1958661417322836718, -2.564304461942256808 ) ) ;
#21088=CARTESIAN_POINT ( 'NONE',  ( -0.2925321140481932924, 0.2925321140481931814, -0.6496062992125984925 ) ) ;
#21091=CARTESIAN_POINT ( 'NONE',  ( -0.1958661417322836718, 0.3392501089628017219, -2.367454068241469756 ) ) ;
#21103=CARTESIAN_POINT ( 'NONE',  ( -9.594673741351310580E-17, 0.3917322834645669549, -1.024915067420260728 ) ) ;
#21109=CARTESIAN_POINT ( 'NONE',  ( -0.3917322834645670659, -7.196005306013484475E-17, -2.398313279036432100 ) ) ;
#21118=CARTESIAN_POINT ( 'NONE',  ( 0.3917322834645669549, 0.1049643490035304660, -1.626640419947506411 ) ) ;
#21127=CARTESIAN_POINT ( 'NONE',  ( 0.1998031496062994405, -0.3460692066303958092, -1.666666666666666741 ) ) ;
#21136=CARTESIAN_POINT ( 'NONE',  ( -1.157146581871515012E-16, 0.4724409448818898682, -0.5492125984251968740 ) ) ;
#21139=CARTESIAN_POINT ( 'NONE',  ( 0.2891555358219910499, -0.2891555358219909944, -0.1751968503937007815 ) ) ;
#21144=CARTESIAN_POINT ( 'NONE',  ( -0.1974969037888704149, -0.3420746716998661063, -0.6148293963254595207 ) ) ;
#21151=CARTESIAN_POINT ( 'NONE',  ( -0.3460692066303960313, 0.1998031496062989965, -1.362860892388451539 ) ) ;
#21153=CARTESIAN_POINT ( 'NONE',  ( 0.1958661417322836440, -0.3392501089628017219, -0.7139107611548556331 ) ) ;
#21166=CARTESIAN_POINT ( 'NONE',  ( -0.2925321140481930149, -0.2925321140481933480, 0.1791338582677164948 ) ) ;
#21183=CARTESIAN_POINT ( 'NONE',  ( -0.3460692066303958092, -0.1998031496062994683, -0.9973753280839895430 ) ) ;
#21188=CARTESIAN_POINT ( 'NONE',  ( 0.3996062992125986035, 2.446882876249141962E-17, -2.480314960629921295 ) ) ;
#21189=CARTESIAN_POINT ( 'NONE',  ( 0.3949938075777409408, 0.1058382717557500574, -1.856955380577427928 ) ) ;
#21190=CARTESIAN_POINT ( 'NONE',  ( -0.1958661417322836718, 0.3392501089628017219, -0.6351706036745405903 ) ) ;
#21193=CARTESIAN_POINT ( 'NONE',  ( -0.1958661417322834220, -0.3392501089628018884, -1.002624671916010568 ) ) ;
#21195=CARTESIAN_POINT ( 'NONE',  ( -0.1049643490035306742, 0.3917322834645668994, -0.08659485744650738392 ) ) ;
#21201=CARTESIAN_POINT ( 'NONE',  ( 0.2925321140481932369, 0.2925321140481932369, -2.500000000000000444 ) ) ;
#21202=CARTESIAN_POINT ( 'NONE',  ( -0.1958661417322833942, -0.3392501089628018884, -1.164717478511497983 ) ) ;
#21207=CARTESIAN_POINT ( 'NONE',  ( 0.3917322834645670104, 2.398668435337828261E-17, -0.5177165354330709457 ) ) ;
#21215=CARTESIAN_POINT ( 'NONE',  ( -0.2065800152999316408, -0.3330030935792791524, -1.929133858267716217 ) ) ;
#21216=CARTESIAN_POINT ( 'NONE',  ( -0.3392501089628017219, -0.1958661417322836718, -1.934383202099737575 ) ) ;
#21217=VERTEX_POINT ( 'NONE', #15022 ) ;
#21218=CARTESIAN_POINT ( 'NONE',  ( -0.1998031496062994683, 0.3460692066303958092, -0.4855643044619422644 ) ) ;
#21223=CARTESIAN_POINT ( 'NONE',  ( 0.4724409448818898682, 2.892866454678787531E-17, -0.03740157480314962313 ) ) ;
#21224=CARTESIAN_POINT ( 'NONE',  ( 0.3973686378485507542, 0.03056273350766219865, -1.929133858267715773 ) ) ;
#21225=CARTESIAN_POINT ( 'NONE',  ( -0.3917322834645671215, 0.1049643490035301469, -1.062335958005249603 ) ) ;
#21227=CARTESIAN_POINT ( 'NONE',  ( -0.3974711515624869129, -0.004548682155782115578, -1.929133858267716439 ) ) ;
#21240=VERTEX_POINT ( 'NONE', #67198 ) ;
#21246=CARTESIAN_POINT ( 'NONE',  ( 0.1049643490035303689, 0.3917322834645668994, -1.175833702590864283 ) ) ;
#21249=CARTESIAN_POINT ( 'NONE',  ( -0.3392501089628019995, 0.1958661417322832277, -1.055774278215223294 ) ) ;
#21256=CARTESIAN_POINT ( 'NONE',  ( 4.797336870675656522E-17, -0.3917322834645670659, -0.2329589483277709483 ) ) ;
#21260=CARTESIAN_POINT ( 'NONE',  ( 0.3458507752293908943, -0.3458507752293908943, -1.592519685039370358 ) ) ;
#21275=CARTESIAN_POINT ( 'NONE',  ( -0.3460692066303957537, -0.1998031496062994405, -2.806430446194225770 ) ) ;
#21281=CARTESIAN_POINT ( 'NONE',  ( -0.1070741851644056997, 0.3996062992125984925, -1.658136482939632339 ) ) ;
#21287=CARTESIAN_POINT ( 'NONE',  ( -9.787531504996566615E-17, 0.3996062992125985480, -1.179133858267716661 ) ) ;
#21288=CARTESIAN_POINT ( 'NONE',  ( 0.3996062992125986590, -0.1070741851644053111, -1.371391076115485053 ) ) ;
#21289=CARTESIAN_POINT ( 'NONE',  ( -0.1974969037888706647, 0.3420746716998658843, -0.4855643044619423754 ) ) ;
#21291=CARTESIAN_POINT ( 'NONE',  ( 0.3917322834645670104, 2.398668435337828261E-17, -0.2677165354330708347 ) ) ;
#21295=CARTESIAN_POINT ( 'NONE',  ( -0.2891555358219911054, 0.2891555358219909388, -1.828740157480315487 ) ) ;
#21299=CARTESIAN_POINT ( 'NONE',  ( -1.157146581871515012E-16, 0.4724409448818898682, -2.047244094488188892 ) ) ;
#21300=CARTESIAN_POINT ( 'NONE',  ( 0.3738583250858177887, 0.1188761721681784872, -2.755905511811022279 ) ) ;
#21307=CARTESIAN_POINT ( 'NONE',  ( 0.3917322834645668994, 0.1049643490035304522, -2.251949188155168979 ) ) ;
#21314=CARTESIAN_POINT ( 'NONE',  ( -0.1049643490035301746, -0.3917322834645670659, -2.671896694716848764 ) ) ;
#21316=CARTESIAN_POINT ( 'NONE',  ( 0.1049643490035303689, 0.3917322834645670104, -1.875328083989501460 ) ) ;
#21319=CARTESIAN_POINT ( 'NONE',  ( 0.2891555358219910499, 0.2891555358219910499, -2.185039370078740273 ) ) ;
#21320=ORIENTED_EDGE ( 'NONE', *, *, #68913, .F. ) ;
#21324=CARTESIAN_POINT ( 'NONE',  ( 0.1070741851644053527, 0.3996062992125986590, -0.7808398950131233418 ) ) ;
#21330=CARTESIAN_POINT ( 'NONE',  ( -0.3392501089628017219, -0.1958661417322836718, 0.1778215223097112108 ) ) ;
#21332=CARTESIAN_POINT ( 'NONE',  ( 0.3917322834645670104, -0.1049643490035303411, -0.8261154855643043637 ) ) ;
#21337=CARTESIAN_POINT ( 'NONE',  ( -9.594673741351313045E-17, 0.3917322834645670104, 0.007874015748031541057 ) ) ;
#21342=CARTESIAN_POINT ( 'NONE',  ( 0.4091458600556403535, 0.2362204724409449896, -1.391076115485564424 ) ) ;
#21345=CARTESIAN_POINT ( 'NONE',  ( 0.2867679344610365999, -0.2867679344610365444, -0.4055118110236220486 ) ) ;
#21346=CARTESIAN_POINT ( 'NONE',  ( 0.1049643490035303689, 0.3917322834645670104, -2.597769028871390606 ) ) ;
#21349=CARTESIAN_POINT ( 'NONE',  ( -0.2925321140481930149, -0.2925321140481933480, -0.1358267716535433156 ) ) ;
#21354=CARTESIAN_POINT ( 'NONE',  ( -0.3392501089628019439, 0.1958661417322832554, 0.2086807331046737768 ) ) ;
#21356=CARTESIAN_POINT ( 'NONE',  ( -0.2867679344610364334, -0.2867679344610367109, -0.1437007874015748810 ) ) ;
#21361=CARTESIAN_POINT ( 'NONE',  ( 0.3917322834645670104, -0.1049643490035303411, -1.993438320209974135 ) ) ;
#21365=CARTESIAN_POINT ( 'NONE',  ( -0.4724409448818895907, -0.1265901696524993070, -0.2801837270341207553 ) ) ;
#21378=CARTESIAN_POINT ( 'NONE',  ( 0.3996062992125985480, 2.446882876249141654E-17, -1.454724409448818756 ) ) ;
#21385=CARTESIAN_POINT ( 'NONE',  ( 0.1216921365961834839, -0.3911666210184605585, -0.005627570198504562755 ) ) ;
#21387=CARTESIAN_POINT ( 'NONE',  ( -0.2925321140481930704, -0.2925321140481933480, -0.05905511811023621965 ) ) ;
#21388=CARTESIAN_POINT ( 'NONE',  ( -0.3917322834645671770, 0.1049643490035302024, -2.706712229167666184 ) ) ;
#21393=CARTESIAN_POINT ( 'NONE',  ( 0.3917322834645670104, -0.1049643490035303411, -2.400918635170603554 ) ) ;
#21401=EDGE_CURVE ( 'NONE', #13953, #66690, #51586, .T. ) ;
#21403=CARTESIAN_POINT ( 'NONE',  ( 0.1049643490035304799, -0.3917322834645670104, -0.3970009430784271487 ) ) ;
#21417=CARTESIAN_POINT ( 'NONE',  ( 0.1958661417322836440, -0.3392501089628017219, -0.5564304461942257696 ) ) ;
#21420=CARTESIAN_POINT ( 'NONE',  ( 0.3949938075777409963, 2.418639510665530435E-17, -1.220472440944881942 ) ) ;
#21431=CARTESIAN_POINT ( 'NONE',  ( -0.4091458600556402980, -0.2362204724409451284, -0.6017060367454067915 ) ) ;
#21436=CARTESIAN_POINT ( 'NONE',  ( 0.2925321140481932369, 0.2925321140481932369, -1.870078740157480546 ) ) ;
#21437=CARTESIAN_POINT ( 'NONE',  ( -0.2925321140481932369, 0.2925321140481931259, -1.041338582677165281 ) ) ;
#21438=CARTESIAN_POINT ( 'NONE',  ( 0.3996062992125984925, 0.1070741851644054637, -0.3589238845144357426 ) ) ;
#21440=CARTESIAN_POINT ( 'NONE',  ( -1.157146581871515012E-16, 0.4724409448818898682, 0.1574803149606299191 ) ) ;
#21441=CARTESIAN_POINT ( 'NONE',  ( -0.1049643490035307020, 0.3917322834645669549, -2.295931758530183497 ) ) ;
#21447=CARTESIAN_POINT ( 'NONE',  ( 0.3458507752293908943, -0.3458507752293908943, -2.064960629921259283 ) ) ;
#21450=CARTESIAN_POINT ( 'NONE',  ( -0.1058382717557503072, 0.3949938075777408852, -1.343175853018372834 ) ) ;
#21460=CARTESIAN_POINT ( 'NONE',  ( 0.1998031496062992463, 0.3460692066303959202, -2.425853018372703396 ) ) ;
#21461=CARTESIAN_POINT ( 'NONE',  ( 0.1958661417322836162, -0.3392501089628018329, -2.061660474244408014 ) ) ;
#21470=CARTESIAN_POINT ( 'NONE',  ( -0.4724409448818898682, -8.678599364036362592E-17, -0.8267716535433070613 ) ) ;
#21473=CARTESIAN_POINT ( 'NONE',  ( 0.1070741851644054776, -0.3996062992125984925, -0.4770341207349080848 ) ) ;
#21475=CARTESIAN_POINT ( 'NONE',  ( 4.797336870675656522E-17, -0.3917322834645670104, -1.265748031496062964 ) ) ;
#21484=CARTESIAN_POINT ( 'NONE',  ( 0.3996062992125985480, 2.446882876249141654E-17, -1.139763779527559029 ) ) ;
#21500=CARTESIAN_POINT ( 'NONE',  ( -9.787531504996567848E-17, 0.3996062992125986035, -0.3149606299212598381 ) ) ;
#21503=CARTESIAN_POINT ( 'NONE',  ( -0.1958661417322836718, 0.3392501089628017219, -2.209973753280840114 ) ) ;
#21504=ORIENTED_EDGE ( 'NONE', *, *, #4894, .F. ) ;
#21514=CARTESIAN_POINT ( 'NONE',  ( 0.1958661417322836162, -0.3392501089628018329, -1.746699844323147843 ) ) ;
#21519=ORIENTED_EDGE ( 'NONE', *, *, #52927, .F. ) ;
#21520=CARTESIAN_POINT ( 'NONE',  ( -0.2867679344610365444, -0.2867679344610367664, -2.890439263288400618 ) ) ;
#21529=CARTESIAN_POINT ( 'NONE',  ( -0.2867679344610364334, -0.2867679344610367109, -1.875984251968503935 ) ) ;
#21533=CARTESIAN_POINT ( 'NONE',  ( -0.1208384647389192101, 0.3726288332213502641, 1.112018681666451222E-17 ) ) ;
#21536=CARTESIAN_POINT ( 'NONE',  ( 0.3996062992125984925, 0.1070741851644054637, -0.04396325459317586282 ) ) ;
#21538=CARTESIAN_POINT ( 'NONE',  ( -0.1070741851644051862, -0.3996062992125987146, -1.961942257217847763 ) ) ;
#21543=CARTESIAN_POINT ( 'NONE',  ( -0.1265901696524993347, 0.4724409448818895907, -0.5557742782152230721 ) ) ;
#21546=CARTESIAN_POINT ( 'NONE',  ( 0.2891555358219910499, 0.2891555358219910499, -0.2145669291338582474 ) ) ;
#21551=CARTESIAN_POINT ( 'NONE',  ( -0.3420746716998662729, 0.1974969037888702206, -0.4179790026246719137 ) ) ;
#21558=CARTESIAN_POINT ( 'NONE',  ( -0.2925321140481930149, -0.2925321140481933480, -1.395669291338582640 ) ) ;
#21560=CARTESIAN_POINT ( 'NONE',  ( -0.2867679344610365999, 0.2867679344610364889, -1.271653543307086798 ) ) ;
#21573=CARTESIAN_POINT ( 'NONE',  ( 0.4724409448818896462, 0.1265901696524990294, -2.721128608923884418 ) ) ;
#21590=CARTESIAN_POINT ( 'NONE',  ( 4.893765752498283924E-17, -0.3996062992125986035, -0.7086614173228346081 ) ) ;
#21594=CARTESIAN_POINT ( 'NONE',  ( 0.3996062992125986590, -0.1070741851644053111, -2.631233595800525293 ) ) ;
#21595=CARTESIAN_POINT ( 'NONE',  ( -0.3949938075777409963, -7.255918531996591613E-17, -2.244094488188976388 ) ) ;
#21597=CARTESIAN_POINT ( 'NONE',  ( -0.3917322834645670104, -7.196005306013484475E-17, -1.133858267716535195 ) ) ;
#21603=CARTESIAN_POINT ( 'NONE',  ( 0.1958661417322836440, -0.3392501089628017219, -1.186351706036745446 ) ) ;
#21605=CARTESIAN_POINT ( 'NONE',  ( -0.3917322834645669549, -7.196005306013483243E-17, 0.1955573735246212974 ) ) ;
#21611=CARTESIAN_POINT ( 'NONE',  ( -0.2925321140481930704, -0.2925321140481933480, -2.893700787401574992 ) ) ;
#21612=CARTESIAN_POINT ( 'NONE',  ( -0.3917322834645670659, -7.196005306013484475E-17, -1.138470759351392969 ) ) ;
#21618=CARTESIAN_POINT ( 'NONE',  ( -0.1958661417322836718, 0.3392501089628017219, -0.5702099737532808632 ) ) ;
#21626=CARTESIAN_POINT ( 'NONE',  ( 0.2362204724409449064, 0.4091458600556404646, -0.5360892388451443669 ) ) ;
#21627=CARTESIAN_POINT ( 'NONE',  ( -0.2867679344610365999, 0.2867679344610364889, -2.216535433070866201 ) ) ;
#21630=CARTESIAN_POINT ( 'NONE',  ( -0.3460692066303960868, 0.1998031496062990242, -0.3412073490813647969 ) ) ;
#21637=CARTESIAN_POINT ( 'NONE',  ( 0.2867679344610365999, 0.2867679344610365999, -1.324803149606299302 ) ) ;
#21638=CARTESIAN_POINT ( 'NONE',  ( -9.787531504996566615E-17, 0.3996062992125985480, -1.966535433070865979 ) ) ;
#21639=CARTESIAN_POINT ( 'NONE',  ( -0.3964540044758075865, -0.009627693922155141845, -1.929133858265299484 ) ) ;
#21649=LINE ( 'NONE', #70925, #44909 ) ;
#21657=CARTESIAN_POINT ( 'NONE',  ( 4.797336870675655290E-17, -0.3917322834645669549, -1.261135539861205412 ) ) ;
#21667=CARTESIAN_POINT ( 'NONE',  ( 0.3917322834645670104, 0.1049643490035304660, 0.03606992306330520509 ) ) ;
#21669=CARTESIAN_POINT ( 'NONE',  ( 0.1265901696524990572, -0.4724409448818897017, -0.2427821522309711322 ) ) ;
#21670=CARTESIAN_POINT ( 'NONE',  ( 5.785732909357575061E-17, -0.4724409448818898682, -1.415354330708661346 ) ) ;
#21685=CARTESIAN_POINT ( 'NONE',  ( -9.787531504996566615E-17, 0.3996062992125985480, -2.753937007874015741 ) ) ;
#21690=CARTESIAN_POINT ( 'NONE',  ( 0.3460692066303959202, -0.1998031496062991630, -1.756561679790026309 ) ) ;
#21695=CARTESIAN_POINT ( 'NONE',  ( -0.2925321140481930149, -0.2925321140481933480, -0.9232283464566929387 ) ) ;
#21696=CARTESIAN_POINT ( 'NONE',  ( -0.2925321140481930704, -0.2925321140481933480, -1.318897637795275690 ) ) ;
#21697=CARTESIAN_POINT ( 'NONE',  ( 0.3949938075777411073, -0.1058382717557499464, -0.8989501312335956840 ) ) ;
#21698=CARTESIAN_POINT ( 'NONE',  ( 0.2925321140481932369, 0.2925321140481932369, -2.342519685039369914 ) ) ;
#21699=CARTESIAN_POINT ( 'NONE',  ( 0.2867679344610366554, 0.2867679344610366554, -0.2874015748031495399 ) ) ;
#21703=CARTESIAN_POINT ( 'NONE',  ( 0.3420746716998660508, 0.1974969037888705814, -1.625328083989501460 ) ) ;
#21707=CARTESIAN_POINT ( 'NONE',  ( 0.4724409448818897572, -0.1265901696524988906, -1.843832020997375309 ) ) ;
#21708=CARTESIAN_POINT ( 'NONE',  ( 0.2898214735618554472, 0.2643935821217320292, -2.755905511811024944 ) ) ;
#21715=CARTESIAN_POINT ( 'NONE',  ( -0.1049643490035306742, 0.3917322834645668994, -2.606279896816586117 ) ) ;
#21723=CARTESIAN_POINT ( 'NONE',  ( 0.1049643490035304522, -0.3917322834645668994, -2.842500369257531023 ) ) ;
#21725=CARTESIAN_POINT ( 'NONE',  ( 0.3392501089628018884, -0.1958661417322834220, -1.829396325459317518 ) ) ;
#21728=CARTESIAN_POINT ( 'NONE',  ( 0.1974969037888706369, -0.3420746716998659953, -2.454068241469816503 ) ) ;
#21733=CARTESIAN_POINT ( 'NONE',  ( -0.3460692066303958092, -0.1998031496062994683, -0.6824146981627295938 ) ) ;
#21738=CARTESIAN_POINT ( 'NONE',  ( -0.1049643490035302024, -0.3917322834645671215, 0.1581364829396324501 ) ) ;
#21744=CARTESIAN_POINT ( 'NONE',  ( 4.797336870675656522E-17, -0.3917322834645670104, 0.08661417322834649712 ) ) ;
#21749=CARTESIAN_POINT ( 'NONE',  ( -1.157146581871515012E-16, 0.4724409448818898682, -1.102362204724409489 ) ) ;
#21752=CARTESIAN_POINT ( 'NONE',  ( 0.1049643490035304938, -0.3917322834645669549, -0.5498687664041993495 ) ) ;
#21753=CARTESIAN_POINT ( 'NONE',  ( 0.2867679344610366554, -0.2867679344610365444, -2.230314960629921295 ) ) ;
#21756=CARTESIAN_POINT ( 'NONE',  ( 0.3460692066303959202, -0.1998031496062991630, -0.1817585301837270351 ) ) ;
#21761=CARTESIAN_POINT ( 'NONE',  ( -0.1049643490035301746, -0.3917322834645670659, 0.1627489745744900018 ) ) ;
#21763=CARTESIAN_POINT ( 'NONE',  ( 0.3392501089628018884, -0.1958661417322834220, -0.03215223097112869521 ) ) ;
#21769=CARTESIAN_POINT ( 'NONE',  ( 4.797336870675656522E-17, -0.3917322834645670104, -2.118110236220472675 ) ) ;
#21773=CARTESIAN_POINT ( 'NONE',  ( -0.1265901696524986964, -0.4724409448818899238, -0.3064304461942257141 ) ) ;
#21785=CARTESIAN_POINT ( 'NONE',  ( -0.3996062992125985480, -7.340648628747423112E-17, -1.690944881889763884 ) ) ;
#21793=CARTESIAN_POINT ( 'NONE',  ( -9.787531504996567848E-17, 0.3996062992125986035, -0.1574803149606299191 ) ) ;
#21794=CARTESIAN_POINT ( 'NONE',  ( -0.3392501089628017219, -0.1958661417322836995, -2.411436638616484718 ) ) ;
#21797=CARTESIAN_POINT ( 'NONE',  ( -0.4724409448818898682, -8.678599364036362592E-17, -2.086614173228346303 ) ) ;
#21799=CARTESIAN_POINT ( 'NONE',  ( -0.1049643490035302024, -0.3917322834645671215, -2.361548556430446144 ) ) ;
#21801=( BOUNDED_CURVE ( )  B_SPLINE_CURVE ( 2, ( #51573, #6146, #51160, #12063, #70535, #64645, #65068, #76040, #50343, #44026, #50755, #57066, #58317 ),
 .UNSPECIFIED., .F., .F. ) 
 B_SPLINE_CURVE_WITH_KNOTS ( ( 3, 2, 2, 2, 2, 2, 3 ),
 ( 0.06250000000000000000, 0.06666666666666666574, 0.07083333333333333148, 0.07500000000000001110, 0.07916666666666666297, 0.08333333333333334259, 0.08750000000000000833 ),
 .UNSPECIFIED. ) 
 CURVE ( )  GEOMETRIC_REPRESENTATION_ITEM ( )  RATIONAL_B_SPLINE_CURVE ( ( 1.000000000000000000, 0.9659258262890683122, 1.000000000000000000, 0.9659258262890683122, 1.000000000000000000, 0.9659258262890683122, 1.000000000000000000, 0.9659258262890683122, 1.000000000000000000, 0.9659258262890683122, 1.000000000000000000, 0.9659258262890682012, 1.000000000000000222 ) ) 
 REPRESENTATION_ITEM ( '' )  );
#21805=CARTESIAN_POINT ( 'NONE',  ( -0.4091458600556405756, 0.2362204724409446288, -0.8136482939632546652 ) ) ;
#21806=CARTESIAN_POINT ( 'NONE',  ( 0.1070741851644054915, -0.3996062992125985480, -1.975065616797900159 ) ) ;
#21809=CARTESIAN_POINT ( 'NONE',  ( -0.1958661417322836995, 0.3392501089628017219, -0.1673421504275084681 ) ) ;
#21817=EDGE_CURVE ( 'NONE', #23246, #24385, #60234, .T. ) ;
#21824=CARTESIAN_POINT ( 'NONE',  ( -0.1049643490035307020, 0.3917322834645669549, -0.4711286089238844177 ) ) ;
#21827=CARTESIAN_POINT ( 'NONE',  ( 4.837279021331060870E-17, -0.3949938075777409963, -1.181102362204724532 ) ) ;
#21828=VERTEX_POINT ( 'NONE', #77220 ) ;
#21837=CARTESIAN_POINT ( 'NONE',  ( 0.4091458600556404646, -0.2362204724409448231, -1.049868766404199460 ) ) ;
#21843=CARTESIAN_POINT ( 'NONE',  ( -0.2925321140481932924, 0.2925321140481931814, -1.594488188976378229 ) ) ;
#21846=CARTESIAN_POINT ( 'NONE',  ( 0.3996062992125986035, -0.1070741851644052972, -1.290682414698162583 ) ) ;
#21847=CARTESIAN_POINT ( 'NONE',  ( 0.1070741851644053388, 0.3996062992125986035, -0.5426509186351704539 ) ) ;
#21849=CARTESIAN_POINT ( 'NONE',  ( 0.4091458600556403535, 0.2362204724409449896, 0.02624671916010498651 ) ) ;
#21850=CARTESIAN_POINT ( 'NONE',  ( -0.1049643490035307020, 0.3917322834645669549, -2.453412073490813139 ) ) ;
#21856=CARTESIAN_POINT ( 'NONE',  ( -0.1265901696524993347, 0.4724409448818895907, -1.815616797900262425 ) ) ;
#21859=CARTESIAN_POINT ( 'NONE',  ( 0.3949938075777409408, -0.1058382717557499186, -1.763123359580052396 ) ) ;
#21869=CARTESIAN_POINT ( 'NONE',  ( -0.1070741851644056997, 0.3996062992125984925, -2.603018372703412631 ) ) ;
#21870=CARTESIAN_POINT ( 'NONE',  ( -0.1049643490035306742, 0.3917322834645668994, -2.448799581855955587 ) ) ;
#21881=CARTESIAN_POINT ( 'NONE',  ( -0.3458507752293906723, -0.3458507752293910609, -0.8464566929133857665 ) ) ;
#21885=CARTESIAN_POINT ( 'NONE',  ( -0.1998031496062991630, -0.3460692066303959202, -0.4573490813648293796 ) ) ;
#21887=CARTESIAN_POINT ( 'NONE',  ( -0.3392501089628019995, 0.1958661417322832277, -1.685695538057742970 ) ) ;
#21896=CARTESIAN_POINT ( 'NONE',  ( -0.3460692066303957537, -0.1998031496062994405, -0.9166666666666666297 ) ) ;
#21899=VERTEX_POINT ( 'NONE', #19549 ) ;
#21906=CARTESIAN_POINT ( 'NONE',  ( 0.1265901696524990572, -0.4724409448818897017, -2.132545931758530244 ) ) ;
#21913=CARTESIAN_POINT ( 'NONE',  ( -0.2925321140481932924, 0.2925321140481931814, -0.3346456692913385988 ) ) ;
#21917=CARTESIAN_POINT ( 'NONE',  ( 4.797336870675656522E-17, -0.3917322834645670104, -2.275590551181102317 ) ) ;
#21929=CARTESIAN_POINT ( 'NONE',  ( -0.3392501089628018329, -0.1958661417322836440, -1.549849450622360791 ) ) ;
#21932=EDGE_CURVE ( 'NONE', #32199, #23562, #55165, .T. ) ;
#21936=CARTESIAN_POINT ( 'NONE',  ( -0.2867679344610367109, 0.2867679344610365444, -2.851069184548242763 ) ) ;
#21946=CARTESIAN_POINT ( 'NONE',  ( 0.2867679344610365999, 0.2867679344610365999, -2.269685039370078705 ) ) ;
#21953=CARTESIAN_POINT ( 'NONE',  ( -0.3996062992125986590, 0.1070741851644051723, 0.2053805774278214813 ) ) ;
#21955=CARTESIAN_POINT ( 'NONE',  ( -0.3460692066303960868, 0.1998031496062990242, -1.758530183727034180 ) ) ;
#21960=CARTESIAN_POINT ( 'NONE',  ( -0.1265901696524993347, 0.4724409448818895907, -0.8707349081364830212 ) ) ;
#21963=CARTESIAN_POINT ( 'NONE',  ( 0.3420746716998660508, 0.1974969037888705814, -0.3654855643044619407 ) ) ;
#21968=CARTESIAN_POINT ( 'NONE',  ( 0.3420746716998660508, 0.1974969037888705814, -0.5229658792650918597 ) ) ;
#21972=CARTESIAN_POINT ( 'NONE',  ( -0.4091458600556402980, -0.2362204724409451284, -0.1292650918635170620 ) ) ;
#21975=CARTESIAN_POINT ( 'NONE',  ( 0.3460692066303958092, 0.1998031496062993018, -1.467847769028871596 ) ) ;
#21977=CARTESIAN_POINT ( 'NONE',  ( 0.1049643490035304938, -0.3917322834645669549, -1.022309711286088829 ) ) ;
#21979=CARTESIAN_POINT ( 'NONE',  ( -0.3910482532979368542, -0.02544847934398145398, -4.648478490738263808E-18 ) ) ;
#22008=CARTESIAN_POINT ( 'NONE',  ( -0.3996062992125986035, -7.340648628747425578E-17, -0.8267716535433070613 ) ) ;
#22012=CARTESIAN_POINT ( 'NONE',  ( -0.3460692066303958092, -0.1998031496062994683, -2.887139107611548461 ) ) ;
#22013=CARTESIAN_POINT ( 'NONE',  ( -0.1974969037888706647, 0.3420746716998658843, -2.375328083989501238 ) ) ;
#22016=CARTESIAN_POINT ( 'NONE',  ( -0.3917322834645670104, -7.196005306013484475E-17, -0.8188976377952754682 ) ) ;
#22022=CARTESIAN_POINT ( 'NONE',  ( 0.1958661417322836162, -0.3392501089628018329, -0.3293770096774785161 ) ) ;
#22029=CARTESIAN_POINT ( 'NONE',  ( 0.3392501089628018884, -0.1958661417322833942, -1.834008817094174848 ) ) ;
#22034=B_SPLINE_CURVE_WITH_KNOTS ( 'NONE', 3,
 ( #41159, #34853, #60515, #2864, #28527, #77812, #20143, #45792, #39496, #13838, #65184, #7520, #74401, #23448, #16745, #11249, #54184, #17568 ),
 .UNSPECIFIED., .F., .F.,
 ( 4, 2, 2, 2, 2, 2, 2, 2, 4 ),
 ( 0.000000000000000000, 0.001588476978679734600, 0.002382715468019601900, 0.002779834712689535550, 0.002978394335024502158, 0.003077674146191985462, 0.003127314051775727331, 0.003152134004567599349, 0.003176953957359471368 ),
 .UNSPECIFIED. ) ;
#22036=CARTESIAN_POINT ( 'NONE',  ( -9.594673741351313045E-17, 0.3917322834645670104, -0.8720472440944883052 ) ) ;
#22045=CARTESIAN_POINT ( 'NONE',  ( 0.3917322834645670104, -0.1049643490035303411, -2.308398950131233640 ) ) ;
#22052=CARTESIAN_POINT ( 'NONE',  ( 0.1958661417322836440, -0.3392501089628017219, -1.121391076115485719 ) ) ;
#22054=CARTESIAN_POINT ( 'NONE',  ( -0.3460692066303960313, 0.1998031496062989965, -1.835301837270341352 ) ) ;
#22064=CARTESIAN_POINT ( 'NONE',  ( -0.1070741851644057135, 0.3996062992125984925, -2.130577427821522374 ) ) ;
#22074=CARTESIAN_POINT ( 'NONE',  ( -0.2867679344610364334, -0.2867679344610368219, -1.241450500491126707 ) ) ;
#22083=CARTESIAN_POINT ( 'NONE',  ( 0.1049643490035303967, 0.3917322834645670659, -0.3051374260180596543 ) ) ;
#22086=CARTESIAN_POINT ( 'NONE',  ( -0.4091458600556402980, -0.2362204724409451284, -1.704068241469816058 ) ) ;
#22098=AXIS2_PLACEMENT_3D ( 'NONE', #9136, #2406, #28064 ) ;
#22104=CARTESIAN_POINT ( 'NONE',  ( 4.893765752498283308E-17, -0.3996062992125985480, -2.832677165354331006 ) ) ;
#22109=CARTESIAN_POINT ( 'NONE',  ( -0.1998031496062994405, 0.3460692066303957537, -2.294619422572178546 ) ) ;
#22114=DIRECTION ( 'NONE',  ( -0.000000000000000000, -0.000000000000000000, 1.000000000000000000 ) ) ;
#22115=CARTESIAN_POINT ( 'NONE',  ( -0.3460692066303958092, -0.1998031496062994683, -1.942257217847769057 ) ) ;
#22116=CARTESIAN_POINT ( 'NONE',  ( 0.1974969037888706369, -0.3420746716998659953, -1.194225721784776928 ) ) ;
#22117=CARTESIAN_POINT ( 'NONE',  ( -9.787531504996567848E-17, 0.3996062992125986035, -2.362204724409448620 ) ) ;
#22118=CARTESIAN_POINT ( 'NONE',  ( 0.1265901696524989184, 0.4724409448818898127, -0.6233595800524933672 ) ) ;
#22119=CARTESIAN_POINT ( 'NONE',  ( 0.3917322834645670104, 2.398668435337828261E-17, -0.1102362204724409017 ) ) ;
#22123=CARTESIAN_POINT ( 'NONE',  ( -0.2891555358219911054, 0.2891555358219909388, -1.986220472440945128 ) ) ;
#22128=CARTESIAN_POINT ( 'NONE',  ( -0.3458507752293909498, 0.3458507752293907833, -2.066929133858267154 ) ) ;
#22136=CARTESIAN_POINT ( 'NONE',  ( -0.3392501089628019439, 0.1958661417322832554, -2.311004306265404651 ) ) ;
#22144=CARTESIAN_POINT ( 'NONE',  ( 0.1958661417322836440, -0.3392501089628017219, -0.3339895013123360679 ) ) ;
#22146=CARTESIAN_POINT ( 'NONE',  ( 4.797336870675656522E-17, -0.3917322834645670104, -1.960629921259842368 ) ) ;
#22149=CARTESIAN_POINT ( 'NONE',  ( -0.2891555358219908833, -0.2891555358219912164, -2.421259842519685623 ) ) ;
#22153=CARTESIAN_POINT ( 'NONE',  ( -0.1070741851644056997, 0.3996062992125986035, -0.9514435695538056015 ) ) ;
#22158=CARTESIAN_POINT ( 'NONE',  ( -0.3392501089628019995, 0.1958661417322832277, 0.04658792650918625738 ) ) ;
#22165=CARTESIAN_POINT ( 'NONE',  ( -0.3392501089628019995, 0.1958661417322832277, 0.1391076115485564701 ) ) ;
#22169=CARTESIAN_POINT ( 'NONE',  ( 0.1265901696524990294, -0.4724409448818896462, -1.187664041994750619 ) ) ;
#22172=CARTESIAN_POINT ( 'NONE',  ( -0.1958661417322836718, 0.3392501089628017219, -0.7926509186351704539 ) ) ;
#22173=CARTESIAN_POINT ( 'NONE',  ( -0.1049643490035307020, 0.3917322834645669549, -2.295931758530183497 ) ) ;
#22176=CARTESIAN_POINT ( 'NONE',  ( -0.2925321140481932369, 0.2925321140481931259, -0.2539370078740156855 ) ) ;
#22182=CARTESIAN_POINT ( 'NONE',  ( -9.594673741351310580E-17, 0.3917322834645669549, 0.2349274522647787078 ) ) ;
#22184=CARTESIAN_POINT ( 'NONE',  ( -0.3392501089628017219, -0.1958661417322836718, -0.4520997375328084655 ) ) ;
#22189=CARTESIAN_POINT ( 'NONE',  ( -0.3392501089628017219, -0.1958661417322836718, -1.776902887139107490 ) ) ;
#22193=CARTESIAN_POINT ( 'NONE',  ( -0.4091458600556402980, -0.2362204724409451284, -0.4442257217847768724 ) ) ;
#22204=CARTESIAN_POINT ( 'NONE',  ( 4.893765752498283308E-17, -0.3996062992125985480, -1.730314960629921517 ) ) ;
#22212=CARTESIAN_POINT ( 'NONE',  ( -0.1998031496062994405, 0.3460692066303957537, -0.4048556430446194621 ) ) ;
#22213=CARTESIAN_POINT ( 'NONE',  ( 0.2925321140481932369, 0.2925321140481932369, 0.01968503937007873641 ) ) ;
#22214=CARTESIAN_POINT ( 'NONE',  ( 4.797336870675656522E-17, -0.3917322834645670659, -2.752643987697849237 ) ) ;
#22220=CARTESIAN_POINT ( 'NONE',  ( 0.1058382717557500852, -0.3949938075777408852, -0.9494750656167980640 ) ) ;
#22225=CARTESIAN_POINT ( 'NONE',  ( -0.2362204724409451284, 0.4091458600556402425, -0.6430446194225721834 ) ) ;
#22230=CARTESIAN_POINT ( 'NONE',  ( 0.3917322834645670659, 2.398668435337828261E-17, -0.4298093420285583055 ) ) ;
#22243=CARTESIAN_POINT ( 'NONE',  ( 0.3392501089628018884, -0.1958661417322834220, -0.7270341207349080292 ) ) ;
#22246=CARTESIAN_POINT ( 'NONE',  ( 0.3949938075777411073, -0.1058382717557499464, -1.056430446194225770 ) ) ;
#22256=CARTESIAN_POINT ( 'NONE',  ( -0.4091458600556405756, 0.2362204724409446288, -0.4179790026246719137 ) ) ;
#22262=CARTESIAN_POINT ( 'NONE',  ( 0.1070741851644054915, -0.3996062992125986035, -1.817585301837270517 ) ) ;
#22265=CARTESIAN_POINT ( 'NONE',  ( -0.1070741851644056997, 0.3996062992125984925, -1.343175853018372834 ) ) ;
#22266=CARTESIAN_POINT ( 'NONE',  ( 0.3996062992125985480, 2.446882876249141654E-17, -0.6673228346456693272 ) ) ;
#22269=CARTESIAN_POINT ( 'NONE',  ( -0.4724409448818899238, 0.1265901696524986686, -0.1902887139107611314 ) ) ;
#22270=CARTESIAN_POINT ( 'NONE',  ( 0.1049643490035303689, 0.3917322834645670104, -2.597769028871390606 ) ) ;
#22276=CARTESIAN_POINT ( 'NONE',  ( -0.4724409448818898682, -8.678599364036362592E-17, -1.848425196850393526 ) ) ;
#22279=CARTESIAN_POINT ( 'NONE',  ( 4.837279021331061486E-17, -0.3949938075777409963, -1.887795275590550936 ) ) ;
#22285=CARTESIAN_POINT ( 'NONE',  ( -0.3458507752293909498, 0.3458507752293908388, -2.301181102362204633 ) ) ;
#22288=CARTESIAN_POINT ( 'NONE',  ( -9.787531504996566615E-17, 0.3996062992125985480, -2.438976377952756014 ) ) ;
#22289=CARTESIAN_POINT ( 'NONE',  ( -0.1049643490035301746, -0.3917322834645670659, -2.356936064795589036 ) ) ;
#22303=CARTESIAN_POINT ( 'NONE',  ( -0.1070741851644051862, -0.3996062992125986590, -0.3064304461942257141 ) ) ;
#22306=CARTESIAN_POINT ( 'NONE',  ( -0.2867679344610364334, -0.2867679344610367109, -2.033464566929133355 ) ) ;
#22315=CARTESIAN_POINT ( 'NONE',  ( -0.3996062992125985480, -7.340648628747423112E-17, -1.061023622047243986 ) ) ;
#22323=CARTESIAN_POINT ( 'NONE',  ( -0.4724409448818898682, -8.678599364036362592E-17, -2.163385826771653697 ) ) ;
#22327=CARTESIAN_POINT ( 'NONE',  ( -0.2867679344610364334, -0.2867679344610367109, -2.728346456692912536 ) ) ;
#22332=CARTESIAN_POINT ( 'NONE',  ( -0.1998031496062991907, -0.3460692066303959757, -0.5380577427821522374 ) ) ;
#22335=CARTESIAN_POINT ( 'NONE',  ( 0.3917322834645670104, -0.1049643490035303411, -2.308398950131233640 ) ) ;
#22343=CARTESIAN_POINT ( 'NONE',  ( 0.4724409448818881474, -0.1265901696525019160, -2.078083989501312345 ) ) ;
#22346=CARTESIAN_POINT ( 'NONE',  ( 0.1958661417322834497, 0.3392501089628018329, -1.641712967682728008 ) ) ;
#22352=CARTESIAN_POINT ( 'NONE',  ( -0.3392501089628017219, -0.1958661417322836995, -2.726397268537744445 ) ) ;
#22361=CARTESIAN_POINT ( 'NONE',  ( 0.3392501089628018884, -0.1958661417322833942, -1.361567872212285257 ) ) ;
#22363=CARTESIAN_POINT ( 'NONE',  ( 0.3392501089628018884, -0.1958661417322834220, -2.079396325459317740 ) ) ;
#22370=CARTESIAN_POINT ( 'NONE',  ( -0.3996062992125984925, -0.1070741851644056858, 0.1922572178477690297 ) ) ;
#22372=CARTESIAN_POINT ( 'NONE',  ( -0.2925321140481930704, -0.2925321140481933480, -1.948818897637795144 ) ) ;
#22377=CARTESIAN_POINT ( 'NONE',  ( 0.2362204724409449064, 0.4091458600556404646, -0.5360892388451443669 ) ) ;
#22381=CARTESIAN_POINT ( 'NONE',  ( 4.837279021331061486E-17, -0.3949938075777409963, -0.6279527559055118058 ) ) ;
#22386=CARTESIAN_POINT ( 'NONE',  ( -0.1974969037888706924, 0.3420746716998658843, -0.5623359580052492701 ) ) ;
#22394=CARTESIAN_POINT ( 'NONE',  ( -9.787531504996566615E-17, 0.3996062992125985480, -1.179133858267716661 ) ) ;
#22397=CARTESIAN_POINT ( 'NONE',  ( 0.2867679344610365999, 0.2867679344610365999, -1.074803149606299080 ) ) ;
#22399=CARTESIAN_POINT ( 'NONE',  ( -0.4724409448818898682, 5.785732909357575061E-17, -2.755905511811024056 ) ) ;
#22400=CARTESIAN_POINT ( 'NONE',  ( -0.2955417804206763588, 0.2579773093944630613, -1.506228638669166960E-17 ) ) ;
#22425=CARTESIAN_POINT ( 'NONE',  ( -0.3460692066303960868, 0.1998031496062990242, -0.6561679790026246906 ) ) ;
#22429=CARTESIAN_POINT ( 'NONE',  ( -0.4091458600556405756, 0.2362204724409446288, -0.02624671916010498651 ) ) ;
#22430=CARTESIAN_POINT ( 'NONE',  ( 0.3949938075777411073, -0.1058382717557499464, -2.158792650918635481 ) ) ;
#22433=CARTESIAN_POINT ( 'NONE',  ( -0.2867679344610364334, -0.2867679344610367109, -0.8385826771653541734 ) ) ;
#22441=CARTESIAN_POINT ( 'NONE',  ( -0.3917322834645669549, -7.196005306013483243E-17, -0.1194032563966385962 ) ) ;
#22446=VECTOR ( 'NONE', #56333, 39.37007874015748143 ) ;
#22447=CARTESIAN_POINT ( 'NONE',  ( -0.4724409448818898682, -8.678599364036362592E-17, -0.5118110236220472231 ) ) ;
#22448=CARTESIAN_POINT ( 'NONE',  ( 0.1958661417322834775, 0.3392501089628018884, -1.715898580873702617 ) ) ;
#22456=CARTESIAN_POINT ( 'NONE',  ( -0.1958661417322836718, 0.3392501089628017219, -1.042650918635170676 ) ) ;
#22465=CARTESIAN_POINT ( 'NONE',  ( -0.1049643490035307020, 0.3917322834645669549, -2.518372703412073754 ) ) ;
#22471=CARTESIAN_POINT ( 'NONE',  ( 0.4724409448818898682, 2.892866454678787531E-17, -2.399606299212598604 ) ) ;
#22472=CARTESIAN_POINT ( 'NONE',  ( 0.1438724767639566193, -0.4624630002188719891, -0.005627570198504299945 ) ) ;
#22473=CARTESIAN_POINT ( 'NONE',  ( -9.594673741351313045E-17, 0.3917322834645670104, -1.344488188976378007 ) ) ;
#22474=CARTESIAN_POINT ( 'NONE',  ( 0.3996062992125984925, 0.1070741851644054637, -2.406167979002624246 ) ) ;
#22482=CARTESIAN_POINT ( 'NONE',  ( -0.3460692066303957537, -0.1998031496062994405, -2.019028871391076230 ) ) ;
#22484=CARTESIAN_POINT ( 'NONE',  ( 0.2867679344610365999, -0.2867679344610365444, 0.06692913385826775030 ) ) ;
#22492=CARTESIAN_POINT ( 'NONE',  ( -0.3917322834645669549, -7.196005306013483243E-17, -1.379245776081677866 ) ) ;
#22495=CARTESIAN_POINT ( 'NONE',  ( -0.4724409448818898682, -8.678599364036362592E-17, -2.635826771653543066 ) ) ;
#22501=CARTESIAN_POINT ( 'NONE',  ( -0.3917322834645670659, -7.196005306013484475E-17, -0.3510691845482433182 ) ) ;
#22505=AXIS2_PLACEMENT_3D ( 'NONE', #79608, #40045, #4623 ) ;
#22506=CARTESIAN_POINT ( 'NONE',  ( -0.3458507752293906723, -0.3458507752293910609, -1.553149606299212726 ) ) ;
#22525=CARTESIAN_POINT ( 'NONE',  ( -0.3996062992125984925, -0.1070741851644056858, -2.327427821522309870 ) ) ;
#22531=CARTESIAN_POINT ( 'NONE',  ( 0.3460692066303959202, 0.1998031496062993295, -1.706036745406824151 ) ) ;
#22532=CARTESIAN_POINT ( 'NONE',  ( -0.1974969037888706647, 0.3420746716998658843, -1.272965879265091749 ) ) ;
#22533=CARTESIAN_POINT ( 'NONE',  ( 4.893765752498283924E-17, -0.3996062992125986035, -2.440944881889763884 ) ) ;
#22535=CARTESIAN_POINT ( 'NONE',  ( -0.1958661417322834220, -0.3392501089628018884, -0.2152230971128608339 ) ) ;
#22539=CARTESIAN_POINT ( 'NONE',  ( 0.3420746716998660508, 0.1974969037888705814, -2.255249343832021136 ) ) ;
#22543=CARTESIAN_POINT ( 'NONE',  ( -0.4724409448818898682, -8.678599364036362592E-17, -2.401574803149606474 ) ) ;
#22544=CARTESIAN_POINT ( 'NONE',  ( 0.3996062992125986590, -0.1070741851644053111, -1.686351706036745446 ) ) ;
#22553=CARTESIAN_POINT ( 'NONE',  ( 0.3392501089628018329, -0.1958661417322834497, -2.862185408627609728 ) ) ;
#22560=CARTESIAN_POINT ( 'NONE',  ( 0.2867679344610365999, 0.2867679344610365999, -0.06496062992125994917 ) ) ;
#22563=CARTESIAN_POINT ( 'NONE',  ( -0.3917322834645669549, -0.1049643490035306603, -2.085301837270341352 ) ) ;
#22566=CARTESIAN_POINT ( 'NONE',  ( 0.3949938075777409408, 0.1058382717557500574, -2.329396325459317740 ) ) ;
#22571=CARTESIAN_POINT ( 'NONE',  ( 0.3996062992125986590, -0.1070741851644053111, -1.056430446194225992 ) ) ;
#22574=LINE ( 'NONE', #34794, #71925 ) ;
#22575=CARTESIAN_POINT ( 'NONE',  ( 0.1958661417322836440, -0.3392501089628017219, 0.1384514435695537171 ) ) ;
#22581=CARTESIAN_POINT ( 'NONE',  ( -0.2867679344610364334, -0.2867679344610367109, 0.1062992125984252439 ) ) ;
#22585=CARTESIAN_POINT ( 'NONE',  ( 0.2362204724409449064, 0.4091458600556404646, -1.719160104986876769 ) ) ;
#22587=CARTESIAN_POINT ( 'NONE',  ( -0.1958661417322836718, 0.3392501089628017219, -0.6351706036745405903 ) ) ;
#22588=CARTESIAN_POINT ( 'NONE',  ( 0.3917322834645669549, 0.1049643490035304660, -2.729002624671915900 ) ) ;
#22595=CARTESIAN_POINT ( 'NONE',  ( 0.3917322834645669549, 2.398668435337827645E-17, 0.1168172160443062824 ) ) ;
#22597=CARTESIAN_POINT ( 'NONE',  ( 0.1049643490035303689, 0.3917322834645670104, -0.5505249343832021580 ) ) ;
#22601=UNCERTAINTY_MEASURE_WITH_UNIT (LENGTH_MEASURE( 1.000000000000000082E-05 ), #12933, 'distance_accuracy_value', 'NONE');
#22603=CARTESIAN_POINT ( 'NONE',  ( -0.3917322834645670104, -7.196005306013484475E-17, -2.236220472440944906 ) ) ;
#22606=CARTESIAN_POINT ( 'NONE',  ( -0.4091458600556405756, 0.2362204724409446288, -0.2604986876640419946 ) ) ;
#22614=CARTESIAN_POINT ( 'NONE',  ( -0.3458507752293909498, 0.3458507752293908388, -1.986220472440944684 ) ) ;
#22616=CARTESIAN_POINT ( 'NONE',  ( -0.1070741851644056997, 0.3996062992125984925, -1.500656167979002031 ) ) ;
#22626=CARTESIAN_POINT ( 'NONE',  ( 0.3996062992125985480, -0.1070741851644052972, -0.3458005249343831244 ) ) ;
#22627=CARTESIAN_POINT ( 'NONE',  ( -9.787531504996567848E-17, 0.3996062992125986035, -0.6299212598425196763 ) ) ;
#22628=CARTESIAN_POINT ( 'NONE',  ( 4.797336870675656522E-17, -0.3917322834645670659, -2.910124302658479767 ) ) ;
#22633=CARTESIAN_POINT ( 'NONE',  ( 0.3420746716998660508, -0.1974969037888704149, -0.9691601049868767692 ) ) ;
#22639=CARTESIAN_POINT ( 'NONE',  ( 0.1265901696524990294, -0.4724409448818896462, -1.030183727034120533 ) ) ;
#22640=CARTESIAN_POINT ( 'NONE',  ( 0.3996062992125986035, 2.446882876249141962E-17, -2.322834645669291209 ) ) ;
#22643=CARTESIAN_POINT ( 'NONE',  ( -0.1049643490035302301, -0.3917322834645671770, -0.2263972685377446670 ) ) ;
#22655=CARTESIAN_POINT ( 'NONE',  ( -0.3917322834645670104, -7.196005306013484475E-17, -1.133858267716535195 ) ) ;
#22658=CARTESIAN_POINT ( 'NONE',  ( -0.3420746716998659953, -0.1974969037888706647, -0.8398950131233596794 ) ) ;
#22669=CARTESIAN_POINT ( 'NONE',  ( 0.4724409448818905899, -0.1265901696524973641, -0.6607611548556431291 ) ) ;
#22674=CARTESIAN_POINT ( 'NONE',  ( 0.3460692066303959757, -0.1998031496062991907, -1.679790026246719137 ) ) ;
#22677=CARTESIAN_POINT ( 'NONE',  ( 0.3996062992125985480, 2.446882876249141654E-17, -1.139763779527559029 ) ) ;
#22681=CARTESIAN_POINT ( 'NONE',  ( 0.2362204724409449064, 0.4091458600556404646, -0.6167979002624671692 ) ) ;
#22682=CARTESIAN_POINT ( 'NONE',  ( 0.2867679344610365999, -0.2867679344610365444, -2.545275590551181022 ) ) ;
#22688=CARTESIAN_POINT ( 'NONE',  ( -0.2362204724409447953, -0.4091458600556404646, -2.189632545931758489 ) ) ;
#22691=CARTESIAN_POINT ( 'NONE',  ( -0.1058382717557497660, -0.3949938075777411073, -1.881233595800524849 ) ) ;
#22701=CARTESIAN_POINT ( 'NONE',  ( -0.1049643490035301746, -0.3917322834645670659, -2.514416379756218678 ) ) ;
#22712=CARTESIAN_POINT ( 'NONE',  ( 0.1265901696524990572, -0.4724409448818897017, -0.8727034120734907807 ) ) ;
#22715=CARTESIAN_POINT ( 'NONE',  ( 0.3996062992125986035, -0.1070741851644052972, -0.1883202099737532054 ) ) ;
#22717=CARTESIAN_POINT ( 'NONE',  ( 4.797336870675656522E-17, -0.3917322834645670104, -1.738188976377952777 ) ) ;
#22726=CARTESIAN_POINT ( 'NONE',  ( 0.3996062992125986035, -0.1070741851644052972, -0.8182414698162727706 ) ) ;
#22728=CARTESIAN_POINT ( 'NONE',  ( 0.1265901696524989184, 0.4724409448818898127, -2.589895013123359568 ) ) ;
#22734=CARTESIAN_POINT ( 'NONE',  ( 0.1958661417322834775, 0.3392501089628018884, -1.646325459317585338 ) ) ;
#22738=CARTESIAN_POINT ( 'NONE',  ( -0.1998031496062994405, 0.3460692066303957537, -2.294619422572178546 ) ) ;
#22740=CARTESIAN_POINT ( 'NONE',  ( 0.3996062992125986035, 2.446882876249141962E-17, -0.5905511811023621549 ) ) ;
#22743=CARTESIAN_POINT ( 'NONE',  ( 0.2867679344610365999, 0.2867679344610365999, -2.177165354330708347 ) ) ;
#22753=CARTESIAN_POINT ( 'NONE',  ( -0.3917322834645669549, -7.196005306013483243E-17, -1.694206406002937593 ) ) ;
#22758=ORIENTED_EDGE ( 'NONE', *, *, #66685, .F. ) ;
#22759=CARTESIAN_POINT ( 'NONE',  ( -0.2867679344610367109, 0.2867679344610365444, -2.693588869587613566 ) ) ;
#22763=CARTESIAN_POINT ( 'NONE',  ( -0.1265901696524993347, 0.4724409448818896462, -0.1640419947506561726 ) ) ;
#22767=CARTESIAN_POINT ( 'NONE',  ( 0.3917322834645670659, 2.398668435337828261E-17, -1.374691231792337653 ) ) ;
#22769=CARTESIAN_POINT ( 'NONE',  ( 0.3392501089628018329, 0.1958661417322835607, -2.420603674540682260 ) ) ;
#22776=CARTESIAN_POINT ( 'NONE',  ( -0.3996062992125986590, 0.1070741851644051723, -0.1095800524934383152 ) ) ;
#22779=CARTESIAN_POINT ( 'NONE',  ( 0.1998031496062994405, -0.3460692066303958092, -1.824146981627296604 ) ) ;
#22785=CARTESIAN_POINT ( 'NONE',  ( -0.2362204724409451284, 0.4091458600556402425, -0.5623359580052492701 ) ) ;
#22788=CARTESIAN_POINT ( 'NONE',  ( 0.1974969037888704704, 0.3420746716998660508, -0.5360892388451443669 ) ) ;
#22793=CARTESIAN_POINT ( 'NONE',  ( -0.2891555358219909388, -0.2891555358219912164, -0.6082677165354331006 ) ) ;
#22803=CARTESIAN_POINT ( 'NONE',  ( -0.3996062992125985480, -7.340648628747423112E-17, -1.375984251968504157 ) ) ;
#22806=CARTESIAN_POINT ( 'NONE',  ( 0.1958661417322834775, 0.3392501089628018884, -1.081364829396325389 ) ) ;
#22808=CARTESIAN_POINT ( 'NONE',  ( -0.1208384647389192101, 0.3726288332213502641, 1.112018681666451222E-17 ) ) ;
#22830=CARTESIAN_POINT ( 'NONE',  ( 0.2017716535433070613, -0.2017716535433070890, -0.3937007874015748254 ) ) ;
#22836=CARTESIAN_POINT ( 'NONE',  ( -0.4724409448818895907, -0.1265901696524993070, 0.1115485564304461719 ) ) ;
#22837=CARTESIAN_POINT ( 'NONE',  ( -0.2891555358219911054, 0.2891555358219909388, -2.381889763779527769 ) ) ;
#22840=CARTESIAN_POINT ( 'NONE',  ( 0.3917322834645670104, -0.1049643490035303411, -1.048556430446194287 ) ) ;
#22842=CARTESIAN_POINT ( 'NONE',  ( 0.4091458600556403535, 0.2362204724409449896, -2.335958005249343827 ) ) ;
#22848=CARTESIAN_POINT ( 'NONE',  ( 0.1049643490035304522, -0.3917322834645668994, -0.1653350149268222880 ) ) ;
#22856=CARTESIAN_POINT ( 'NONE',  ( 0.1049643490035304799, -0.3917322834645670104, -1.656843462763466723 ) ) ;
#22862=CARTESIAN_POINT ( 'NONE',  ( -0.3392501089628017219, -0.1958661417322836718, -0.9245406824146982228 ) ) ;
#22870=CARTESIAN_POINT ( 'NONE',  ( -0.2362204724409447953, -0.4091458600556404646, -0.9297900262467192478 ) ) ;
#22871=CARTESIAN_POINT ( 'NONE',  ( 0.3917322834645670104, 2.398668435337828261E-17, -2.472440944881889813 ) ) ;
#22878=CARTESIAN_POINT ( 'NONE',  ( -0.1049643490035302024, -0.3917322834645671215, -0.9442257217847768169 ) ) ;
#22881=CARTESIAN_POINT ( 'NONE',  ( 4.797336870675656522E-17, -0.3917322834645670104, -1.580708661417322913 ) ) ;
#22882=CARTESIAN_POINT ( 'NONE',  ( -0.1070741851644056997, 0.3996062992125984925, -2.603018372703412631 ) ) ;
#22890=CARTESIAN_POINT ( 'NONE',  ( -9.594673741351313045E-17, 0.3917322834645670104, 0.1653543307086614844 ) ) ;
#22897=CARTESIAN_POINT ( 'NONE',  ( -0.3392501089628018329, -0.1958661417322836440, -1.077408505740470535 ) ) ;
#22906=CARTESIAN_POINT ( 'NONE',  ( 0.3917322834645670104, 0.1049643490035304660, -0.2788907068579546400 ) ) ;
#22910=CARTESIAN_POINT ( 'NONE',  ( -0.3458507752293906723, -0.3458507752293910609, -2.025590551181101873 ) ) ;
#22920=B_SPLINE_CURVE_WITH_KNOTS ( 'NONE', 3,
 ( #25441, #51107, #76804, #44784, #70481, #45210, #64590, #6926, #58259, #74242, #35513, #35934, #46879, #21224, #40580, #9019, #3531, #59934 ),
 .UNSPECIFIED., .F., .F.,
 ( 4, 2, 2, 2, 2, 2, 2, 2, 4 ),
 ( 1.401326170026117541E-16, 0.001588476978679904169, 0.002382715468019786214, 0.002779834712689726369, 0.002978394335024696880, 0.003077674146192181919, 0.003127314051775924655, 0.003152134004567797108, 0.003176953957359669126 ),
 .UNSPECIFIED. ) ;
#22932=CARTESIAN_POINT ( 'NONE',  ( -9.787531504996567848E-17, 0.3996062992125986035, -0.1574803149606299746 ) ) ;
#22933=CARTESIAN_POINT ( 'NONE',  ( 4.893765752498283308E-17, -0.3996062992125985480, -2.202755905511811108 ) ) ;
#22938=CARTESIAN_POINT ( 'NONE',  ( -0.3996062992125986035, -0.1070741851644056997, -1.778215223097112663 ) ) ;
#22939=CARTESIAN_POINT ( 'NONE',  ( 0.1974969037888704704, 0.3420746716998660508, -1.246719160104986734 ) ) ;
#22940=CARTESIAN_POINT ( 'NONE',  ( 0.3996062992125986590, -0.1070741851644053111, -2.316272965879265122 ) ) ;
#22942=CARTESIAN_POINT ( 'NONE',  ( -0.1958661417322834220, -0.3392501089628018884, -0.05774278215223092176 ) ) ;
#22946=CARTESIAN_POINT ( 'NONE',  ( -0.3420746716998662729, 0.1974969037888702206, -2.307742782152230721 ) ) ;
#22951=CARTESIAN_POINT ( 'NONE',  ( -0.2362204724409451284, 0.4091458600556402425, -2.375328083989501238 ) ) ;
#22952=CARTESIAN_POINT ( 'NONE',  ( 0.3996062992125986035, 2.446882876249141962E-17, -1.692913385826771533 ) ) ;
#22960=CARTESIAN_POINT ( 'NONE',  ( 0.3392501089628018884, -0.1958661417322834220, 0.1253280839895012100 ) ) ;
#22967=CARTESIAN_POINT ( 'NONE',  ( 0.1958661417322834775, 0.3392501089628018884, -0.2290026246719160941 ) ) ;
#22969=CARTESIAN_POINT ( 'NONE',  ( 0.1958661417322836440, -0.3392501089628017219, -2.446194225721784576 ) ) ;
#22972=CARTESIAN_POINT ( 'NONE',  ( -0.3949938075777409963, -7.255918531996591613E-17, -2.559055118110236560 ) ) ;
#22976=CARTESIAN_POINT ( 'NONE',  ( -0.3460692066303960868, 0.1998031496062990242, -0.9711286089238845287 ) ) ;
#22981=CARTESIAN_POINT ( 'NONE',  ( 0.3917322834645670104, -0.1049643490035303411, 0.1187664041994749703 ) ) ;
#22989=CARTESIAN_POINT ( 'NONE',  ( 0.2867679344610365999, -0.2867679344610365444, 0.06692913385826775030 ) ) ;
#22993=CARTESIAN_POINT ( 'NONE',  ( 0.2362204724409451007, -0.4091458600556402980, -1.666666666666666741 ) ) ;
#22995=CARTESIAN_POINT ( 'NONE',  ( 0.1958661417322836440, -0.3392501089628017219, -0.5564304461942257696 ) ) ;
#23003=CARTESIAN_POINT ( 'NONE',  ( -0.3392501089628018329, -0.1958661417322836440, -0.1325266159766911034 ) ) ;
#23005=CARTESIAN_POINT ( 'NONE',  ( 0.2867679344610366554, -0.2867679344610365444, -0.3405511811023621549 ) ) ;
#23010=CARTESIAN_POINT ( 'NONE',  ( 0.3392501089628018884, -0.1958661417322834220, -2.144356955380577467 ) ) ;
#23013=CARTESIAN_POINT ( 'NONE',  ( 0.2362204724409451007, -0.4091458600556402980, -0.6410761154855643129 ) ) ;
#23022=CARTESIAN_POINT ( 'NONE',  ( -0.1265901696524993347, 0.4724409448818896462, -0.3215223097112860917 ) ) ;
#23025=CARTESIAN_POINT ( 'NONE',  ( 0.1998031496062992463, 0.3460692066303959202, -2.110892388451443225 ) ) ;
#23033=CARTESIAN_POINT ( 'NONE',  ( 0.1998031496062992463, 0.3460692066303959202, -0.3786089238845143923 ) ) ;
#23034=CARTESIAN_POINT ( 'NONE',  ( -0.2925321140481932924, 0.2925321140481931814, -0.4921259842519684624 ) ) ;
#23035=CARTESIAN_POINT ( 'NONE',  ( -0.2891555358219908833, -0.2891555358219912164, 0.09842519685039366473 ) ) ;
#23041=CARTESIAN_POINT ( 'NONE',  ( -0.2891555358219909388, -0.2891555358219912164, -0.9232283464566930498 ) ) ;
#23046=CARTESIAN_POINT ( 'NONE',  ( -0.4091458600556405756, 0.2362204724409446288, -1.128608923884514503 ) ) ;
#23047=CARTESIAN_POINT ( 'NONE',  ( -0.1070741851644051862, -0.3996062992125986590, -2.119422572178477626 ) ) ;
#23050=CARTESIAN_POINT ( 'NONE',  ( -0.1958661417322836995, 0.3392501089628017219, -0.6397830953093982531 ) ) ;
#23061=CARTESIAN_POINT ( 'NONE',  ( 0.2867679344610365999, 0.2867679344610365999, -1.232283464566929387 ) ) ;
#23063=VERTEX_POINT ( 'NONE', #61174 ) ;
#23064=CARTESIAN_POINT ( 'NONE',  ( 0.1974969037888706369, -0.3420746716998659953, -1.036745406824147064 ) ) ;
#23068=FACE_OUTER_BOUND ( 'NONE', #19568, .T. ) ;
#23081=CARTESIAN_POINT ( 'NONE',  ( 4.893765752498283924E-17, -0.3996062992125986035, -1.811023622047244208 ) ) ;
#23084=CARTESIAN_POINT ( 'NONE',  ( 0.3460692066303959202, -0.1998031496062991630, -0.9691601049868766582 ) ) ;
#23088=CARTESIAN_POINT ( 'NONE',  ( 0.2362204724409449064, 0.4091458600556404646, -0.3018372703412073310 ) ) ;
#23090=CARTESIAN_POINT ( 'NONE',  ( -0.3917322834645669549, -0.1049643490035306603, -2.335301837270341352 ) ) ;
#23096=CARTESIAN_POINT ( 'NONE',  ( 0.2362204724409451007, -0.4091458600556402980, -2.373359580052493367 ) ) ;
#23098=CARTESIAN_POINT ( 'NONE',  ( 0.3420746716998660508, 0.1974969037888705814, -1.940288713910761187 ) ) ;
#23110=CARTESIAN_POINT ( 'NONE',  ( 0.3917322834645669549, 2.398668435337827645E-17, -2.560348138286403064 ) ) ;
#23114=CARTESIAN_POINT ( 'NONE',  ( -0.4091458600556405756, 0.2362204724409446288, -1.047900262467191590 ) ) ;
#23123=CARTESIAN_POINT ( 'NONE',  ( 0.2925321140481932369, 0.2925321140481932369, -0.3720472440944882497 ) ) ;
#23125=CARTESIAN_POINT ( 'NONE',  ( 0.3917322834645670104, -0.1049643490035303411, -1.928477690288713742 ) ) ;
#23134=CARTESIAN_POINT ( 'NONE',  ( 0.3460692066303959202, -0.1998031496062991630, -1.284120734908136496 ) ) ;
#23140=CARTESIAN_POINT ( 'NONE',  ( -0.3392501089628017219, -0.1958661417322836718, -1.711942257217847763 ) ) ;
#23141=CARTESIAN_POINT ( 'NONE',  ( 0.4091458600556404646, -0.2362204724409448231, -2.152230971128608950 ) ) ;
#23144=CARTESIAN_POINT ( 'NONE',  ( 0.1208384647389237204, -0.3726288332213487653, -2.755905511811024056 ) ) ;
#23145=CARTESIAN_POINT ( 'NONE',  ( -0.1070741851644051862, -0.3996062992125986035, -2.196194225721784576 ) ) ;
#23147=CARTESIAN_POINT ( 'NONE',  ( 0.3460692066303959202, 0.1998031496062993295, -0.9186351706036745002 ) ) ;
#23150=CARTESIAN_POINT ( 'NONE',  ( 0.1049643490035304938, -0.3917322834645669549, -2.439632545931758045 ) ) ;
#23160=CARTESIAN_POINT ( 'NONE',  ( 4.797336870675655290E-17, -0.3917322834645669549, -1.733576484743095669 ) ) ;
#23162=CARTESIAN_POINT ( 'NONE',  ( 0.3726288332213487653, 0.1208384647389236927, -1.220472440944882164 ) ) ;
#23164=CARTESIAN_POINT ( 'NONE',  ( -0.1049643490035307020, 0.3917322834645669549, -2.768372703412072866 ) ) ;
#23167=CARTESIAN_POINT ( 'NONE',  ( -0.1058382717557503211, 0.3949938075777409408, 0.1509186351706036378 ) ) ;
#23175=CARTESIAN_POINT ( 'NONE',  ( 0.3917322834645670659, 2.398668435337828261E-17, -1.217210916831708012 ) ) ;
#23177=CARTESIAN_POINT ( 'NONE',  ( 0.3917322834645670104, -0.1049643490035303411, -2.085958005249344271 ) ) ;
#23182=CARTESIAN_POINT ( 'NONE',  ( 0.3996062992125986035, 0.1070741851644054776, -0.5971128608923884640 ) ) ;
#23184=CARTESIAN_POINT ( 'NONE',  ( -0.1998031496062994405, 0.3460692066303957537, 0.2250656167979002698 ) ) ;
#23186=CARTESIAN_POINT ( 'NONE',  ( -0.1998031496062994683, 0.3460692066303958092, -2.217847769028871596 ) ) ;
#23191=CARTESIAN_POINT ( 'NONE',  ( -0.1265901696524986964, -0.4724409448818899238, -0.9363517060367454459 ) ) ;
#23195=CARTESIAN_POINT ( 'NONE',  ( -0.3949938075777409963, -7.255918531996591613E-17, -0.5885826771653542844 ) ) ;
#23208=CARTESIAN_POINT ( 'NONE',  ( -0.1998031496062994405, 0.3460692066303957537, -1.822178477690288956 ) ) ;
#23211=CARTESIAN_POINT ( 'NONE',  ( 0.3392501089628018329, 0.1958661417322835607, -1.225721784776902634 ) ) ;
#23213=CARTESIAN_POINT ( 'NONE',  ( -0.1614515132151654597, 0.3594585737333474973, 1.112018681666451376E-17 ) ) ;
#23234=CARTESIAN_POINT ( 'NONE',  ( 0.3917322834645670659, -0.1049643490035303273, -2.155531126805461550 ) ) ;
#23244=CARTESIAN_POINT ( 'NONE',  ( 5.785732909357575061E-17, -0.4724409448818898682, -0.07874015748031495954 ) ) ;
#23245=CARTESIAN_POINT ( 'NONE',  ( -0.3949938075777409408, -0.1058382717557502933, -2.408136482939633449 ) ) ;
#23246=VERTEX_POINT ( 'NONE', #22471 ) ;
#23249=CARTESIAN_POINT ( 'NONE',  ( 0.2867679344610365999, 0.2867679344610365999, -0.7598425196850391306 ) ) ;
#23251=CARTESIAN_POINT ( 'NONE',  ( -0.2362204724409451284, 0.4091458600556402425, -2.532808398950130879 ) ) ;
#23257=CARTESIAN_POINT ( 'NONE',  ( -0.3917322834645668994, -0.1049643490035306742, -0.4409255661079247157 ) ) ;
#23264=CARTESIAN_POINT ( 'NONE',  ( 0.3996062992125986035, 2.446882876249141962E-17, -2.952755905511811108 ) ) ;
#23265=CARTESIAN_POINT ( 'NONE',  ( 0.3392501089628018329, 0.1958661417322835607, -1.702775221293650443 ) ) ;
#23271=CARTESIAN_POINT ( 'NONE',  ( 0.3392501089628018884, -0.1958661417322834220, -1.134514435695538115 ) ) ;
#23281=CARTESIAN_POINT ( 'NONE',  ( 0.2867679344610365999, 0.2867679344610365999, -2.492125984251968518 ) ) ;
#23288=CARTESIAN_POINT ( 'NONE',  ( -0.1049643490035302024, -0.3917322834645671215, -0.7867454068241470644 ) ) ;
#23289=CARTESIAN_POINT ( 'NONE',  ( 0.3458507752293908943, -0.3458507752293908943, -0.01771653543307087630 ) ) ;
#23291=CARTESIAN_POINT ( 'NONE',  ( -0.2925321140481932369, 0.2925321140481931259, -2.301181102362204633 ) ) ;
#23294=VECTOR ( 'NONE', #79781, 39.37007874015748143 ) ;
#23301=CARTESIAN_POINT ( 'NONE',  ( -0.2925321140481930149, -0.2925321140481933480, -2.025590551181102317 ) ) ;
#23310=CARTESIAN_POINT ( 'NONE',  ( 0.2867679344610365999, 0.2867679344610365999, -1.635151287892701255 ) ) ;
#23320=CARTESIAN_POINT ( 'NONE',  ( -0.2867679344610365444, -0.2867679344610367664, -0.6857148538395820836 ) ) ;
#23323=CARTESIAN_POINT ( 'NONE',  ( 0.3458507752293908943, -0.3458507752293908943, -1.907480314960629197 ) ) ;
#23344=CARTESIAN_POINT ( 'NONE',  ( 0.2925321140481932369, -0.2925321140481931814, -2.379921259842520342 ) ) ;
#23349=CARTESIAN_POINT ( 'NONE',  ( -0.3996062992125986035, -7.340648628747425578E-17, -1.614173228346456712 ) ) ;
#23350=CARTESIAN_POINT ( 'NONE',  ( -0.3949938075777411628, 0.1058382717557497937, -0.9776902887139109488 ) ) ;
#23351=CARTESIAN_POINT ( 'NONE',  ( -9.787531504996567848E-17, 0.3996062992125986035, -2.519685039370078705 ) ) ;
#23354=CARTESIAN_POINT ( 'NONE',  ( 0.3917322834645670104, -0.1049643490035303273, -0.4186351706036745557 ) ) ;
#23358=CARTESIAN_POINT ( 'NONE',  ( -0.3420746716998662729, 0.1974969037888702206, -2.150262467191601523 ) ) ;
#23361=CARTESIAN_POINT ( 'NONE',  ( -0.2362204724409451284, 0.4091458600556402425, -2.532808398950130879 ) ) ;
#23362=CARTESIAN_POINT ( 'NONE',  ( -0.3996062992125986035, -7.340648628747425578E-17, -1.614173228346456712 ) ) ;
#23364=ADVANCED_FACE ( 'NONE', ( #42642 ), #68339, .T. ) ;
#23371=CARTESIAN_POINT ( 'NONE',  ( -0.2867679344610366554, 0.2867679344610365444, -2.776883571357268821 ) ) ;
#23378=CARTESIAN_POINT ( 'NONE',  ( -0.1958661417322834220, -0.3392501089628018884, 0.007217847769028785422 ) ) ;
#23380=CARTESIAN_POINT ( 'NONE',  ( 4.797336870675656522E-17, -0.3917322834645670104, -2.433070866141732402 ) ) ;
#23383=CARTESIAN_POINT ( 'NONE',  ( -0.3949938075777409408, -0.1058382717557502933, -2.565616797900262647 ) ) ;
#23387=CARTESIAN_POINT ( 'NONE',  ( -0.3460692066303960868, 0.1998031496062990242, -1.128608923884514503 ) ) ;
#23393=CARTESIAN_POINT ( 'NONE',  ( 0.1049643490035304938, -0.3917322834645669549, -0.4849081364829396779 ) ) ;
#23400=CARTESIAN_POINT ( 'NONE',  ( 4.797336870675656522E-17, -0.3917322834645670104, -0.2283464566929133410 ) ) ;
#23404=CARTESIAN_POINT ( 'NONE',  ( 5.785732909357575061E-17, -0.4724409448818898682, -1.653543307086614123 ) ) ;
#23410=DIRECTION ( 'NONE',  ( 0.000000000000000000, 0.000000000000000000, 1.000000000000000000 ) ) ;
#23413=CARTESIAN_POINT ( 'NONE',  ( 0.1049643490035304522, -0.3917322834645668994, -0.4802956448480821261 ) ) ;
#23415=CARTESIAN_POINT ( 'NONE',  ( -0.1958661417322834220, -0.3392501089628018884, -0.4652230971128609727 ) ) ;
#23421=CARTESIAN_POINT ( 'NONE',  ( -0.1049643490035307020, 0.3917322834645669549, -2.518372703412073754 ) ) ;
#23425=CARTESIAN_POINT ( 'NONE',  ( 0.3458507752293908943, 0.3458507752293908943, -0.6870078740157479213 ) ) ;
#23436=CARTESIAN_POINT ( 'NONE',  ( 0.3996062992125986035, -0.1070741851644052972, -2.078083989501312345 ) ) ;
#23445=CARTESIAN_POINT ( 'NONE',  ( -0.3460692066303957537, -0.1998031496062994405, -0.2867454068241469534 ) ) ;
#23446=CARTESIAN_POINT ( 'NONE',  ( 0.3996062992125986035, 0.1070741851644054776, -0.5971128608923884640 ) ) ;
#23447=CARTESIAN_POINT ( 'NONE',  ( -0.1058382717557503211, 0.3949938075777409408, 0.1509186351706036378 ) ) ;
#23448=CARTESIAN_POINT ( 'NONE',  ( 0.03056273350766125496, -0.3973686378485505322, -8.612909436664462853E-17 ) ) ;
#23452=CARTESIAN_POINT ( 'NONE',  ( 0.2891555358219910499, -0.2891555358219909944, -0.8051181102362204856 ) ) ;
#23457=CARTESIAN_POINT ( 'NONE',  ( -0.3458507752293909498, 0.3458507752293907833, -1.279527559055118058 ) ) ;
#23458=CARTESIAN_POINT ( 'NONE',  ( 0.1070741851644053666, 0.3996062992125986035, -2.355643044619422533 ) ) ;
#23461=CARTESIAN_POINT ( 'NONE',  ( -0.3917322834645671770, 0.1049643490035302024, -0.6594681346794770693 ) ) ;
#23473=CARTESIAN_POINT ( 'NONE',  ( -0.3917322834645669549, -0.1049643490035306603, -0.9829396325459317518 ) ) ;
#23476=CARTESIAN_POINT ( 'NONE',  ( -0.3420746716998659953, -0.1974969037888706647, -1.627296587926509330 ) ) ;
#23480=CARTESIAN_POINT ( 'NONE',  ( 0.1070741851644054915, -0.3996062992125986035, 0.07217847769028869209 ) ) ;
#23484=EDGE_CURVE ( 'NONE', #40183, #5969, #11816, .T. ) ;
#23489=CARTESIAN_POINT ( 'NONE',  ( -0.3917322834645669549, -0.1049643490035306603, -0.1305774278215224293 ) ) ;
#23494=CARTESIAN_POINT ( 'NONE',  ( -0.2925321140481930704, -0.2925321140481933480, -1.948818897637795144 ) ) ;
#23497=CARTESIAN_POINT ( 'NONE',  ( -0.2925321140481930149, -0.2925321140481933480, -1.553149606299212726 ) ) ;
#23501=CARTESIAN_POINT ( 'NONE',  ( 0.4091458600556404646, -0.2362204724409448231, -0.5774278215223097588 ) ) ;
#23503=CARTESIAN_POINT ( 'NONE',  ( -9.594673741351313045E-17, 0.3917322834645670104, -2.446850393700787496 ) ) ;
#23509=CARTESIAN_POINT ( 'NONE',  ( -0.1265901696524986964, -0.4724409448818899238, -2.511154855643044748 ) ) ;
#23511=CARTESIAN_POINT ( 'NONE',  ( -0.1974969037888706924, 0.3420746716998658843, -1.664698162729658870 ) ) ;
#23531=CARTESIAN_POINT ( 'NONE',  ( 0.3996062992125986035, 2.446882876249141962E-17, -0.7480314960629921295 ) ) ;
#23533=CARTESIAN_POINT ( 'NONE',  ( -0.1998031496062991630, -0.3460692066303959202, -0.7723097112860892732 ) ) ;
#23534=CARTESIAN_POINT ( 'NONE',  ( 0.3392501089628018329, 0.1958661417322835607, -1.948162729658792891 ) ) ;
#23544=CARTESIAN_POINT ( 'NONE',  ( 0.1998031496062992463, 0.3460692066303959202, -1.323490813648294129 ) ) ;
#23551=CARTESIAN_POINT ( 'NONE',  ( -0.3917322834645669549, -0.1049643490035306603, -1.705380577427821898 ) ) ;
#23556=CARTESIAN_POINT ( 'NONE',  ( -0.1070741851644051862, -0.3996062992125986035, -2.353674540682414662 ) ) ;
#23558=CARTESIAN_POINT ( 'NONE',  ( -0.3996062992125986035, -0.1070741851644056997, -0.8333333333333332593 ) ) ;
#23561=CARTESIAN_POINT ( 'NONE',  ( 0.3392501089628018884, -0.1958661417322834220, -2.459317585301837195 ) ) ;
#23562=VERTEX_POINT ( 'NONE', #70379 ) ;
#23571=CARTESIAN_POINT ( 'NONE',  ( 0.3917322834645668994, 0.1049643490035304522, -1.936988558233908808 ) ) ;
#23574=CARTESIAN_POINT ( 'NONE',  ( -0.1958661417322834220, -0.3392501089628018884, 0.09973753280839900426 ) ) ;
#23577=CARTESIAN_POINT ( 'NONE',  ( 0.3949938075777409963, 2.418639510665530435E-17, -0.1181102362204724948 ) ) ;
#23586=CARTESIAN_POINT ( 'NONE',  ( -0.3917322834645671770, 0.1049643490035302024, -1.289389394521996968 ) ) ;
#23588=CARTESIAN_POINT ( 'NONE',  ( -9.594673741351313045E-17, 0.3917322834645670104, -2.289370078740157410 ) ) ;
#23593=CARTESIAN_POINT ( 'NONE',  ( 0.3460692066303959757, -0.1998031496062991907, -0.4199475065616797842 ) ) ;
#23595=CARTESIAN_POINT ( 'NONE',  ( -0.3460692066303957537, -0.1998031496062994405, -0.2867454068241469534 ) ) ;
#23597=CARTESIAN_POINT ( 'NONE',  ( 0.1070741851644053527, 0.3996062992125986590, -2.355643044619422533 ) ) ;
#23598=( BOUNDED_CURVE ( )  B_SPLINE_CURVE ( 2, ( #44391, #19570, #43992, #64197, #45229, #32615, #63362, #44803, #5297, #51126, #82324, #31367, #6531 ),
 .UNSPECIFIED., .F., .F. ) 
 B_SPLINE_CURVE_WITH_KNOTS ( ( 3, 2, 2, 2, 2, 2, 3 ),
 ( 0.9125000000000000888, 0.9166666666666667407, 0.9208333333333333925, 0.9250000000000000444, 0.9291666666666666963, 0.9333333333333333481, 0.9375000000000000000 ),
 .UNSPECIFIED. ) 
 CURVE ( )  GEOMETRIC_REPRESENTATION_ITEM ( )  RATIONAL_B_SPLINE_CURVE ( ( 0.9999999999999991118, 0.9659258262890692004, 1.000000000000000000, 0.9659258262890683122, 1.000000000000000000, 0.9659258262890683122, 1.000000000000000000, 0.9659258262890683122, 1.000000000000000000, 0.9659258262890683122, 1.000000000000000000, 0.9659258262890683122, 1.000000000000000000 ) ) 
 REPRESENTATION_ITEM ( '' )  );
#23604=CARTESIAN_POINT ( 'NONE',  ( -0.3458507752293909498, 0.3458507752293907833, -0.8838582677165351953 ) ) ;
#23607=CARTESIAN_POINT ( 'NONE',  ( -0.3949938075777409963, -7.255918531996591613E-17, -0.7460629921259843700 ) ) ;
#23620=CARTESIAN_POINT ( 'NONE',  ( 0.3996062992125986035, -0.1070741851644052972, -1.605643044619422977 ) ) ;
#23622=CARTESIAN_POINT ( 'NONE',  ( 0.3392501089628018884, -0.1958661417322834220, -1.671916010498687655 ) ) ;
#23624=CARTESIAN_POINT ( 'NONE',  ( -0.3588842212258053777, -0.1584414948821128155, 7.390873527593507220E-17 ) ) ;
#23644=CARTESIAN_POINT ( 'NONE',  ( 0.1049643490035304799, -0.3917322834645670104, -1.971804092684726228 ) ) ;
#23652=CARTESIAN_POINT ( 'NONE',  ( 0.1958661417322834775, 0.3392501089628018884, -2.183727034120734878 ) ) ;
#23656=CARTESIAN_POINT ( 'NONE',  ( 0.4724409448818897572, -0.1265901696524988906, -0.1115485564304461719 ) ) ;
#23657=CARTESIAN_POINT ( 'NONE',  ( -0.1974969037888703871, -0.3420746716998661063, -2.585301837270341352 ) ) ;
#23660=CARTESIAN_POINT ( 'NONE',  ( -0.3392501089628019995, 0.1958661417322832277, -1.278215223097112885 ) ) ;
#23662=CARTESIAN_POINT ( 'NONE',  ( -0.2362204724409447953, -0.4091458600556404646, -2.427821522309711266 ) ) ;
#23667=CARTESIAN_POINT ( 'NONE',  ( -9.594673741351310580E-17, 0.3917322834645669549, -0.8674347524596309755 ) ) ;
#23675=CARTESIAN_POINT ( 'NONE',  ( -0.2867679344610367109, 0.2867679344610365444, -2.221147924705723753 ) ) ;
#23681=CARTESIAN_POINT ( 'NONE',  ( 0.3917322834645670104, 2.398668435337828261E-17, -0.9901574803149607584 ) ) ;
#23689=CARTESIAN_POINT ( 'NONE',  ( -0.4724409448818898682, -8.678599364036362592E-17, -1.061023622047243986 ) ) ;
#23691=CARTESIAN_POINT ( 'NONE',  ( 0.3917322834645669549, 0.1049643490035304660, -2.636482939632545985 ) ) ;
#23701=CARTESIAN_POINT ( 'NONE',  ( 0.2867679344610365999, -0.2867679344610365444, -0.9704724409448820532 ) ) ;
#23702=CARTESIAN_POINT ( 'NONE',  ( -0.1265901696524993347, 0.4724409448818895907, 0.2316272965879264956 ) ) ;
#23704=CARTESIAN_POINT ( 'NONE',  ( 0.1070741851644054776, -0.3996062992125984925, -2.366797900262467280 ) ) ;
#23714=CARTESIAN_POINT ( 'NONE',  ( -0.1070741851644056997, 0.3996062992125984925, -0.3982939632545932085 ) ) ;
#23716=CARTESIAN_POINT ( 'NONE',  ( 0.1049643490035303689, 0.3917322834645670104, -0.3005249343832020470 ) ) ;
#23724=CARTESIAN_POINT ( 'NONE',  ( 0.1049643490035304522, -0.3917322834645668994, -1.582657849572491449 ) ) ;
#23733=CARTESIAN_POINT ( 'NONE',  ( -0.1958661417322833942, -0.3392501089628018884, -0.5347962186689783071 ) ) ;
#23735=CARTESIAN_POINT ( 'NONE',  ( 0.2017716535433070613, 0.2017716535433070613, 0.000000000000000000 ) ) ;
#23737=CARTESIAN_POINT ( 'NONE',  ( -0.1265901696524986964, -0.4724409448818899238, -2.196194225721784576 ) ) ;
#23758=CARTESIAN_POINT ( 'NONE',  ( 4.893765752498283308E-17, -0.3996062992125985480, -2.045275590551181466 ) ) ;
#23765=CARTESIAN_POINT ( 'NONE',  ( -0.1998031496062991907, -0.3460692066303959757, -1.640419947506561726 ) ) ;
#23766=CARTESIAN_POINT ( 'NONE',  ( -0.2891555358219908833, -0.2891555358219912164, -1.318897637795275912 ) ) ;
#23767=CARTESIAN_POINT ( 'NONE',  ( 0.3460692066303959202, 0.1998031496062993295, -2.808398950131233640 ) ) ;
#23769=CARTESIAN_POINT ( 'NONE',  ( -0.3917322834645671215, 0.1049643490035301469, -0.6548556430446192955 ) ) ;
#23773=CARTESIAN_POINT ( 'NONE',  ( -0.1058382717557503072, 0.3949938075777408852, -1.973097112860892510 ) ) ;
#23777=CARTESIAN_POINT ( 'NONE',  ( 0.4724409448818896462, 0.1265901696524990294, -2.486876640419947382 ) ) ;
#23778=CARTESIAN_POINT ( 'NONE',  ( -0.1998031496062994683, 0.3460692066303958092, -1.587926509186351698 ) ) ;
#23785=CARTESIAN_POINT ( 'NONE',  ( 0.1958661417322834497, 0.3392501089628018329, -2.744075172407137497 ) ) ;
#23791=CARTESIAN_POINT ( 'NONE',  ( -9.594673741351313045E-17, 0.3917322834645670104, -0.2421259842519686289 ) ) ;
#23793=CARTESIAN_POINT ( 'NONE',  ( 0.3917322834645669549, 0.1049643490035304660, -2.164041994750655729 ) ) ;
#23795=ORIENTED_EDGE ( 'NONE', *, *, #2885, .T. ) ;
#23796=CARTESIAN_POINT ( 'NONE',  ( -0.1058382717557497937, -0.3949938075777411628, -2.591863517060367883 ) ) ;
#23800=CARTESIAN_POINT ( 'NONE',  ( -0.3460692066303958092, -0.1998031496062994683, -0.9973753280839895430 ) ) ;
#23805=CARTESIAN_POINT ( 'NONE',  ( 0.3917322834645670104, -0.1049643490035303411, -0.3536745406824148286 ) ) ;
#23811=CARTESIAN_POINT ( 'NONE',  ( -0.2867679344610365999, 0.2867679344610364889, -0.3267716535433070613 ) ) ;
#23812=ORIENTED_EDGE ( 'NONE', *, *, #15671, .T. ) ;
#23818=CARTESIAN_POINT ( 'NONE',  ( -0.3458507752293909498, 0.3458507752293907833, -1.751968503937007648 ) ) ;
#23819=CARTESIAN_POINT ( 'NONE',  ( -0.2017716535433071445, -0.2017716535433071723, 0.000000000000000000 ) ) ;
#23820=ADVANCED_FACE ( 'NONE', ( #57325 ), #11914, .T. ) ;
#23822=CARTESIAN_POINT ( 'NONE',  ( 0.4724409448818898682, 2.892866454678787531E-17, -0.9055118110236221041 ) ) ;
#23830=CARTESIAN_POINT ( 'NONE',  ( -9.594673741351310580E-17, 0.3917322834645669549, -0.2375134926171111049 ) ) ;
#23832=CARTESIAN_POINT ( 'NONE',  ( -0.3392501089628019995, 0.1958661417322832277, -0.2683727034120735877 ) ) ;
#23837=CARTESIAN_POINT ( 'NONE',  ( -0.3392501089628019995, 0.1958661417322832277, -2.223097112860892288 ) ) ;
#23839=ADVANCED_FACE ( 'NONE', ( #75887 ), #18228, .T. ) ;
#23841=CARTESIAN_POINT ( 'NONE',  ( -0.3458507752293906723, -0.3458507752293910609, -0.7657480314960628531 ) ) ;
#23851=VERTEX_POINT ( 'NONE', #57741 ) ;
#23852=CARTESIAN_POINT ( 'NONE',  ( 0.1070741851644053388, 0.3996062992125986035, -1.959973753280839892 ) ) ;
#23860=CARTESIAN_POINT ( 'NONE',  ( 0.3996062992125984925, 0.1070741851644054499, -0.04396325459317587669 ) ) ;
#23861=CARTESIAN_POINT ( 'NONE',  ( 0.1070741851644053527, 0.3996062992125986590, -0.6233595800524933672 ) ) ;
#23862=CARTESIAN_POINT ( 'NONE',  ( 0.1974969037888704704, 0.3420746716998660508, 0.01312335958005243601 ) ) ;
#23866=CARTESIAN_POINT ( 'NONE',  ( 0.4724409448818898682, 2.892866454678787531E-17, -2.399606299212598604 ) ) ;
#23867=CARTESIAN_POINT ( 'NONE',  ( -0.3949938075777408852, -0.1058382717557502933, -0.7526246719160105680 ) ) ;
#23872=CARTESIAN_POINT ( 'NONE',  ( 0.2362204724409451007, -0.4091458600556402980, -1.351706036745406792 ) ) ;
#23874=CARTESIAN_POINT ( 'NONE',  ( 0.3460692066303959202, 0.1998031496062993295, -2.178477690288713742 ) ) ;
#23878=CARTESIAN_POINT ( 'NONE',  ( 0.1958661417322834775, 0.3392501089628018884, -0.7710166911099232134 ) ) ;
#23890=CARTESIAN_POINT ( 'NONE',  ( -0.3392501089628019995, 0.1958661417322832277, -1.120734908136482799 ) ) ;
#23893=CARTESIAN_POINT ( 'NONE',  ( -0.2891555358219908833, -0.2891555358219912164, -1.633858267716535195 ) ) ;
#23905=CARTESIAN_POINT ( 'NONE',  ( 0.1049643490035304938, -0.3917322834645669549, -0.01246719160104995359 ) ) ;
#23911=CARTESIAN_POINT ( 'NONE',  ( 0.1998031496062994405, -0.3460692066303958092, -1.981627296587926690 ) ) ;
#23914=CARTESIAN_POINT ( 'NONE',  ( -0.2925321140481930149, -0.2925321140481933480, -1.395669291338582196 ) ) ;
#23918=CARTESIAN_POINT ( 'NONE',  ( 0.4724409448818898682, 2.892866454678787531E-17, -0.5905511811023621549 ) ) ;
#23920=CARTESIAN_POINT ( 'NONE',  ( -0.3917322834645671215, 0.1049643490035301469, 0.1325459317585302443 ) ) ;
#23926=CARTESIAN_POINT ( 'NONE',  ( 5.785732909357575061E-17, -0.4724409448818898682, -2.360236220472441193 ) ) ;
#23928=CARTESIAN_POINT ( 'NONE',  ( 0.2891555358219910499, -0.2891555358219909944, -2.379921259842519898 ) ) ;
#23938=DIRECTION ( 'NONE',  ( 1.000000000000000000, 0.000000000000000000, 0.000000000000000000 ) ) ;
#23947=CARTESIAN_POINT ( 'NONE',  ( 0.3996062992125986035, -0.1070741851644052972, -0.6607611548556431291 ) ) ;
#23948=CARTESIAN_POINT ( 'NONE',  ( 0.1958661417322836440, -0.3392501089628017219, -2.066272965879265122 ) ) ;
#23958=CARTESIAN_POINT ( 'NONE',  ( 0.3458507752293908943, 0.3458507752293908943, -2.185039370078739829 ) ) ;
#23966=CARTESIAN_POINT ( 'NONE',  ( 0.1958661417322834775, 0.3392501089628018884, -1.488845144356955252 ) ) ;
#23967=CARTESIAN_POINT ( 'NONE',  ( 0.006303098004689107643, 0.3922539627124311812, -1.220472440944881720 ) ) ;
#23971=CARTESIAN_POINT ( 'NONE',  ( 0.1998031496062992463, 0.3460692066303959202, -2.583333333333333481 ) ) ;
#23973=CARTESIAN_POINT ( 'NONE',  ( -0.3460692066303958092, -0.1998031496062994683, -0.9973753280839895430 ) ) ;
#23976=CARTESIAN_POINT ( 'NONE',  ( -0.3392501089628019995, 0.1958661417322832277, -2.538057742782152015 ) ) ;
#23987=CARTESIAN_POINT ( 'NONE',  ( -0.3392501089628019439, 0.1958661417322832554, -1.996043676344145146 ) ) ;
#23990=CARTESIAN_POINT ( 'NONE',  ( 0.3917322834645670104, 2.398668435337828261E-17, -2.722440944881889369 ) ) ;
#23993=CARTESIAN_POINT ( 'NONE',  ( 0.3420746716998660508, -0.1974969037888703871, -0.2624671916010499206 ) ) ;
#23997=CARTESIAN_POINT ( 'NONE',  ( 0.4724409448818898682, 2.892866454678787531E-17, -0.1181102362204724532 ) ) ;
#24001=CARTESIAN_POINT ( 'NONE',  ( -0.3392501089628017219, -0.1958661417322836995, -1.151594118931445365 ) ) ;
#24003=CARTESIAN_POINT ( 'NONE',  ( 0.3917322834645670104, -0.1049643490035303411, -2.715879265091863726 ) ) ;
#24008=CARTESIAN_POINT ( 'NONE',  ( 0.1070741851644054915, -0.3996062992125986035, -0.8727034120734907807 ) ) ;
#24010=CARTESIAN_POINT ( 'NONE',  ( 4.893765752498283308E-17, -0.3996062992125985480, -0.1555118110236220763 ) ) ;
#24012=CARTESIAN_POINT ( 'NONE',  ( 0.3996062992125986035, 2.446882876249141962E-17, -2.165354330708661568 ) ) ;
#24016=CARTESIAN_POINT ( 'NONE',  ( 0.3458507752293908943, 0.3458507752293908943, -1.001968503937007871 ) ) ;
#24019=CARTESIAN_POINT ( 'NONE',  ( 0.3420746716998660508, -0.1974969037888704149, -1.126640419947506633 ) ) ;
#24030=CARTESIAN_POINT ( 'NONE',  ( 0.2925321140481932369, 0.2925321140481932369, -1.789370078740157410 ) ) ;
#24032=CARTESIAN_POINT ( 'NONE',  ( 0.3917322834645670104, -0.1049643490035303411, -1.520997375328083656 ) ) ;
#24045=CARTESIAN_POINT ( 'NONE',  ( 0.3917322834645669549, 0.1049643490035304660, -1.154199475065616820 ) ) ;
#24063=CARTESIAN_POINT ( 'NONE',  ( -0.3996062992125986035, -7.340648628747425578E-17, -1.141732283464566899 ) ) ;
#24064=CARTESIAN_POINT ( 'NONE',  ( 0.2952755905511810774, 0.000000000000000000, -1.929133858267716661 ) ) ;
#24065=CARTESIAN_POINT ( 'NONE',  ( 0.1049643490035303689, 0.3917322834645670104, -2.190288713910760965 ) ) ;
#24068=CARTESIAN_POINT ( 'NONE',  ( -0.2362204724409447953, -0.4091458600556404646, -0.3805774278215223183 ) ) ;
#24069=CARTESIAN_POINT ( 'NONE',  ( -0.1058382717557497937, -0.3949938075777411628, -2.591863517060367883 ) ) ;
#24070=ORIENTED_EDGE ( 'NONE', *, *, #62908, .F. ) ;
#24072=CARTESIAN_POINT ( 'NONE',  ( 0.2867679344610365999, 0.2867679344610365999, -1.389763779527558807 ) ) ;
#24074=CARTESIAN_POINT ( 'NONE',  ( -0.4724409448818899238, 0.1265901696524986686, -2.552493438320210029 ) ) ;
#24075=CARTESIAN_POINT ( 'NONE',  ( -1.157146581871515012E-16, 0.4724409448818898682, -0.8641732283464567121 ) ) ;
#24080=CARTESIAN_POINT ( 'NONE',  ( -0.2867679344610366554, 0.2867679344610365444, -0.5721591619084497315 ) ) ;
#24088=CARTESIAN_POINT ( 'NONE',  ( -0.1049643490035307158, 0.3917322834645670104, -1.893063935204411186 ) ) ;
#24095=CARTESIAN_POINT ( 'NONE',  ( -0.3392501089628017219, -0.1958661417322836718, -1.554461942257217899 ) ) ;
#24105=CARTESIAN_POINT ( 'NONE',  ( 0.3917322834645670104, 2.398668435337828261E-17, -2.629921259842519898 ) ) ;
#24112=CARTESIAN_POINT ( 'NONE',  ( -0.1958661417322836718, 0.3392501089628017219, -0.8851706036745407014 ) ) ;
#24113=CARTESIAN_POINT ( 'NONE',  ( 0.4724409448818897572, -0.1265901696524988906, 0.1266404199475065218 ) ) ;
#24115=CARTESIAN_POINT ( 'NONE',  ( -0.3949938075777409963, -7.255918531996591613E-17, 0.1988188976377952832 ) ) ;
#24124=CARTESIAN_POINT ( 'NONE',  ( -0.1998031496062991630, -0.3460692066303959202, -0.6148293963254594097 ) ) ;
#24126=CARTESIAN_POINT ( 'NONE',  ( -0.2867679344610364334, -0.2867679344610367109, -0.2086614173228345248 ) ) ;
#24133=CARTESIAN_POINT ( 'NONE',  ( -0.3917322834645670659, 0.1049643490035301607, -1.845125041173541369 ) ) ;
#24142=CARTESIAN_POINT ( 'NONE',  ( -9.594673741351313045E-17, 0.3917322834645670659, -0.7841400506899758316 ) ) ;
#24147=CARTESIAN_POINT ( 'NONE',  ( -0.3458507752293906723, -0.3458507752293910609, -1.868110236220472453 ) ) ;
#24167=CARTESIAN_POINT ( 'NONE',  ( -0.1998031496062991907, -0.3460692066303959757, -0.06561679790026248016 ) ) ;
#24168=CARTESIAN_POINT ( 'NONE',  ( 0.3996062992125986035, -0.1070741851644052972, -2.550524934383202158 ) ) ;
#24173=CARTESIAN_POINT ( 'NONE',  ( 0.3996062992125986035, 0.1070741851644054776, -2.014435695538057569 ) ) ;
#24174=CARTESIAN_POINT ( 'NONE',  ( 0.3420746716998660508, -0.1974969037888703871, -1.364829396325459410 ) ) ;
#24175=CARTESIAN_POINT ( 'NONE',  ( 0.2925321140481932369, -0.2925321140481932369, -2.775590551181101429 ) ) ;
#24177=CARTESIAN_POINT ( 'NONE',  ( -0.3392501089628019995, 0.1958661417322832277, -0.8057742782152230721 ) ) ;
#24181=CARTESIAN_POINT ( 'NONE',  ( -9.674558042662122972E-17, 0.3949938075777409963, -2.753937007874016185 ) ) ;
#24185=CARTESIAN_POINT ( 'NONE',  ( 5.785732909357575061E-17, -0.4724409448818898682, -2.598425196850393970 ) ) ;
#24186=CARTESIAN_POINT ( 'NONE',  ( 0.2925321140481932369, -0.2925321140481932369, -2.303149606299212060 ) ) ;
#24193=CARTESIAN_POINT ( 'NONE',  ( 0.1049643490035303689, 0.3917322834645668994, -2.750636852197163584 ) ) ;
#24199=CARTESIAN_POINT ( 'NONE',  ( -0.3917322834645669549, -0.1049643490035306603, -0.6030183727034120755 ) ) ;
#24200=CARTESIAN_POINT ( 'NONE',  ( 0.3392501089628018884, -0.1958661417322834220, -1.356955380577427928 ) ) ;
#24201=CARTESIAN_POINT ( 'NONE',  ( -0.2867679344610364334, -0.2867679344610367109, -2.413385826771653253 ) ) ;
#24204=CARTESIAN_POINT ( 'NONE',  ( 0.3949938075777411073, -0.1058382717557499464, -2.631233595800525293 ) ) ;
#24208=CARTESIAN_POINT ( 'NONE',  ( 4.893765752498283924E-17, -0.3996062992125986035, -1.653543307086614123 ) ) ;
#24209=CARTESIAN_POINT ( 'NONE',  ( 0.03757601356357168076, -0.4709442531824368783, -4.620136098463503353E-16 ) ) ;
#24211=CARTESIAN_POINT ( 'NONE',  ( 0.000000000000000000, 0.000000000000000000, -2.755905511811024056 ) ) ;
#24213=CARTESIAN_POINT ( 'NONE',  ( 0.3392501089628018329, 0.1958661417322835607, -0.3733595800524935338 ) ) ;
#24219=CARTESIAN_POINT ( 'NONE',  ( -0.3917322834645670104, -7.196005306013484475E-17, -0.1889763779527558474 ) ) ;
#24224=CARTESIAN_POINT ( 'NONE',  ( 0.4724409448818897572, -0.1265901696524988906, -1.843832020997375309 ) ) ;
#24234=CARTESIAN_POINT ( 'NONE',  ( -0.1049643490035301746, -0.3917322834645670659, -0.3096919703073997554 ) ) ;
#24236=CARTESIAN_POINT ( 'NONE',  ( 0.2867679344610366554, -0.2867679344610365444, -0.6555118110236221041 ) ) ;
#24241=CARTESIAN_POINT ( 'NONE',  ( -0.3392501089628019995, 0.1958661417322832277, -2.380577427821522374 ) ) ;
#24244=CARTESIAN_POINT ( 'NONE',  ( 0.2362204724409449064, 0.4091458600556404646, -0.8510498687664042050 ) ) ;
#24256=CARTESIAN_POINT ( 'NONE',  ( 0.1998031496062994128, -0.3460692066303957537, -2.058398950131233640 ) ) ;
#24264=CARTESIAN_POINT ( 'NONE',  ( 0.3996062992125985480, -0.1070741851644052972, -0.8182414698162728817 ) ) ;
#24265=CARTESIAN_POINT ( 'NONE',  ( -0.1998031496062991907, -0.3460692066303959757, -1.010498687664042050 ) ) ;
#24266=CARTESIAN_POINT ( 'NONE',  ( 4.837279021331060870E-17, -0.3949938075777409963, -0.3937007874015748810 ) ) ;
#24274=CARTESIAN_POINT ( 'NONE',  ( -0.1974969037888706924, 0.3420746716998658843, -1.192257217847769279 ) ) ;
#24279=CARTESIAN_POINT ( 'NONE',  ( -0.1265901696524993347, 0.4724409448818895907, -1.108923884514435798 ) ) ;
#24280=CARTESIAN_POINT ( 'NONE',  ( 0.1998031496062992740, 0.3460692066303959757, -2.506561679790026087 ) ) ;
#24283=CARTESIAN_POINT ( 'NONE',  ( -0.3392501089628017219, -0.1958661417322836995, -0.6791531740495557745 ) ) ;
#24284=ORIENTED_EDGE ( 'NONE', *, *, #73965, .T. ) ;
#24295=CARTESIAN_POINT ( 'NONE',  ( 0.2867679344610365999, 0.2867679344610365999, -0.9173228346456693272 ) ) ;
#24298=CARTESIAN_POINT ( 'NONE',  ( -0.3949938075777409963, -7.255918531996591613E-17, -1.614173228346456934 ) ) ;
#24310=CARTESIAN_POINT ( 'NONE',  ( 0.1958661417322836440, -0.3392501089628017219, -0.01902887139107619849 ) ) ;
#24316=CARTESIAN_POINT ( 'NONE',  ( 0.3996062992125986035, 0.1070741851644054776, -2.171916010498687211 ) ) ;
#24319=CARTESIAN_POINT ( 'NONE',  ( 0.3996062992125984925, 0.1070741851644054637, -1.776246719160104570 ) ) ;
#24324=CARTESIAN_POINT ( 'NONE',  ( 0.2362204724409451007, -0.4091458600556402980, -0.2493438320209973857 ) ) ;
#24325=CARTESIAN_POINT ( 'NONE',  ( 0.2017716535433070613, -0.2017716535433070890, 0.000000000000000000 ) ) ;
#24326=CARTESIAN_POINT ( 'NONE',  ( -0.1049643490035302024, -0.3917322834645671215, 0.09317585301837273681 ) ) ;
#24332=CARTESIAN_POINT ( 'NONE',  ( 5.785732909357575061E-17, -0.4724409448818898682, -2.517716535433071279 ) ) ;
#24334=CARTESIAN_POINT ( 'NONE',  ( -9.674558042662122972E-17, 0.3949938075777409963, -2.124015748031495843 ) ) ;
#24348=CARTESIAN_POINT ( 'NONE',  ( 0.000000000000000000, 0.000000000000000000, -2.755905511811024056 ) ) ;
#24357=CARTESIAN_POINT ( 'NONE',  ( 0.1070741851644053388, 0.3996062992125986035, -0.7001312335958002064 ) ) ;
#24358=CARTESIAN_POINT ( 'NONE',  ( -0.1049643490035307020, 0.3917322834645669549, -2.138451443569553412 ) ) ;
#24367=CARTESIAN_POINT ( 'NONE',  ( -1.157146581871515012E-16, 0.4724409448818898682, -2.596456692913385655 ) ) ;
#24374=CARTESIAN_POINT ( 'NONE',  ( 0.3392501089628018884, -0.1958661417322834220, -1.606955380577427928 ) ) ;
#24375=CARTESIAN_POINT ( 'NONE',  ( -0.3204081651523081331, 0.2263583204867674892, -1.220472440944882164 ) ) ;
#24378=CARTESIAN_POINT ( 'NONE',  ( -0.2952755905511810774, 3.616083068348483797E-17, -1.929133858267716661 ) ) ;
#24379=CARTESIAN_POINT ( 'NONE',  ( -0.3996062992125984925, -0.1070741851644056719, -2.484908136482939955 ) ) ;
#24381=CARTESIAN_POINT ( 'NONE',  ( 0.3996062992125986035, 2.446882876249141962E-17, -0.9055118110236221041 ) ) ;
#24384=CARTESIAN_POINT ( 'NONE',  ( -0.1049643490035307020, 0.3917322834645669549, -2.518372703412073754 ) ) ;
#24385=VERTEX_POINT ( 'NONE', #45947 ) ;
#24397=CARTESIAN_POINT ( 'NONE',  ( 0.1049643490035304938, -0.3917322834645669549, -2.689632545931758489 ) ) ;
#24400=CARTESIAN_POINT ( 'NONE',  ( -0.3420746716998659953, -0.1974969037888706647, -0.2099737532808399476 ) ) ;
#24407=CARTESIAN_POINT ( 'NONE',  ( 0.1958661417322834775, 0.3392501089628018884, -1.558418265913072309 ) ) ;
#24409=CARTESIAN_POINT ( 'NONE',  ( 0.1958661417322834775, 0.3392501089628018884, -2.591207349081364519 ) ) ;
#24414=CARTESIAN_POINT ( 'NONE',  ( -0.3460692066303958092, -0.1998031496062994683, -0.9973753280839895430 ) ) ;
#24416=CARTESIAN_POINT ( 'NONE',  ( 0.3996062992125986035, -0.1070741851644052972, -0.3458005249343831244 ) ) ;
#24418=CARTESIAN_POINT ( 'NONE',  ( -0.3996062992125986035, -0.1070741851644056997, -2.408136482939632561 ) ) ;
#24419=CARTESIAN_POINT ( 'NONE',  ( 0.1049643490035304938, -0.3917322834645669549, -1.744750656167979308 ) ) ;
#24423=CARTESIAN_POINT ( 'NONE',  ( -0.4724409448818898682, -8.678599364036362592E-17, -1.061023622047243986 ) ) ;
#24427=CARTESIAN_POINT ( 'NONE',  ( -0.1058382717557497660, -0.3949938075777411073, -1.093832020997375309 ) ) ;
#24440=CARTESIAN_POINT ( 'NONE',  ( 0.3460692066303958092, 0.1998031496062993018, -1.782808398950131323 ) ) ;
#24456=CARTESIAN_POINT ( 'NONE',  ( -0.1049643490035307020, 0.3917322834645669549, -1.036089238845144589 ) ) ;
#24477=CARTESIAN_POINT ( 'NONE',  ( -0.3392501089628017219, -0.1958661417322836718, -1.934383202099737575 ) ) ;
#24480=CARTESIAN_POINT ( 'NONE',  ( -0.1265901696524986964, -0.4724409448818899238, -0.5446194225721783244 ) ) ;
#24481=CARTESIAN_POINT ( 'NONE',  ( 0.3420746716998660508, -0.1974969037888703871, -2.624671916010498318 ) ) ;
#24484=CARTESIAN_POINT ( 'NONE',  ( 0.3392501089628018884, -0.1958661417322834220, -1.514435695538058013 ) ) ;
#24486=CARTESIAN_POINT ( 'NONE',  ( -0.4091458600556405756, 0.2362204724409446288, -2.388451443569553856 ) ) ;
#24493=CARTESIAN_POINT ( 'NONE',  ( -9.594673741351310580E-17, 0.3917322834645669549, -0.7099544374990010009 ) ) ;
#24501=CARTESIAN_POINT ( 'NONE',  ( -0.1958661417322836995, 0.3392501089628017219, -1.899625614994437495 ) ) ;
#24503=VERTEX_POINT ( 'NONE', #24325 ) ;
#24508=CARTESIAN_POINT ( 'NONE',  ( -0.1958661417322836718, 0.3392501089628017219, -1.357611548556430625 ) ) ;
#24518=CARTESIAN_POINT ( 'NONE',  ( -0.1049643490035302024, -0.3917322834645671215, -2.741469816272964710 ) ) ;
#24525=CARTESIAN_POINT ( 'NONE',  ( -0.1049643490035302024, -0.3917322834645671215, -1.101706036745407014 ) ) ;
#24526=CARTESIAN_POINT ( 'NONE',  ( 0.4091458600556403535, 0.2362204724409449896, 0.1069553805774278027 ) ) ;
#24529=CARTESIAN_POINT ( 'NONE',  ( 4.837279021331061486E-17, -0.3949938075777409963, 0.1594488188976377896 ) ) ;
#24539=CARTESIAN_POINT ( 'NONE',  ( 4.893765752498283308E-17, -0.3996062992125985480, -0.6279527559055118058 ) ) ;
#24542=CARTESIAN_POINT ( 'NONE',  ( -0.3392501089628019995, 0.1958661417322832277, -0.3333333333333333148 ) ) ;
#24545=FACE_OUTER_BOUND ( 'NONE', #31509, .T. ) ;
#24557=CARTESIAN_POINT ( 'NONE',  ( -0.3917322834645670104, -0.1049643490035307020, -0.9875521241807894146 ) ) ;
#24561=CARTESIAN_POINT ( 'NONE',  ( -0.4091458600556402980, -0.2362204724409451284, -1.861548556430446144 ) ) ;
#24580=CARTESIAN_POINT ( 'NONE',  ( -0.1998031496062994405, 0.3460692066303957537, -2.452099737532808188 ) ) ;
#24585=CARTESIAN_POINT ( 'NONE',  ( -0.3460692066303958092, -0.1998031496062994683, -2.257217847769029007 ) ) ;
#24586=CARTESIAN_POINT ( 'NONE',  ( 0.3949938075777409408, 0.1058382717557500574, -1.699475065616798064 ) ) ;
#24588=CARTESIAN_POINT ( 'NONE',  ( 0.4091458600556403535, 0.2362204724409449896, -2.493438320209973469 ) ) ;
#24589=CARTESIAN_POINT ( 'NONE',  ( 0.3392501089628018884, -0.1958661417322834220, -0.5695538057742781657 ) ) ;
#24593=CARTESIAN_POINT ( 'NONE',  ( 0.3949938075777409408, -0.1058382717557499186, -2.393044619422572072 ) ) ;
#24597=CARTESIAN_POINT ( 'NONE',  ( 0.4091458600556403535, 0.2362204724409449896, -2.808398950131233640 ) ) ;
#24598=CARTESIAN_POINT ( 'NONE',  ( 0.3996062992125986035, 0.1070741851644054776, -2.329396325459317296 ) ) ;
#24604=CARTESIAN_POINT ( 'NONE',  ( 0.3392501089628018884, -0.1958661417322834220, -0.1896325459317586282 ) ) ;
#24608=CARTESIAN_POINT ( 'NONE',  ( 0.4724409448818898682, 2.892866454678787531E-17, -2.007874015748031482 ) ) ;
#24612=CARTESIAN_POINT ( 'NONE',  ( -0.1958661417322834220, -0.3392501089628018884, -0.6227034120734910028 ) ) ;
#24613=CARTESIAN_POINT ( 'NONE',  ( -0.3917322834645671215, 0.1049643490035301469, -1.599737532808399143 ) ) ;
#24614=CARTESIAN_POINT ( 'NONE',  ( -0.1049643490035307020, 0.3917322834645669549, -2.833333333333333037 ) ) ;
#24617=CARTESIAN_POINT ( 'NONE',  ( 0.1058382717557499880, 0.3949938075777411073, -2.513123359580052174 ) ) ;
#24621=CARTESIAN_POINT ( 'NONE',  ( -0.1998031496062994683, 0.3460692066303958092, -1.272965879265091749 ) ) ;
#24623=CARTESIAN_POINT ( 'NONE',  ( -0.4091458600556402980, -0.2362204724409451284, -0.7591863517060367661 ) ) ;
#24626=CARTESIAN_POINT ( 'NONE',  ( -0.3392501089628019995, 0.1958661417322832277, -0.5833333333333334814 ) ) ;
#24633=ORIENTED_EDGE ( 'NONE', *, *, #37682, .F. ) ;
#24636=CARTESIAN_POINT ( 'NONE',  ( -0.1265901696524993347, 0.4724409448818895907, -2.211286089238845065 ) ) ;
#24646=CARTESIAN_POINT ( 'NONE',  ( 0.3917322834645669549, 2.398668435337827645E-17, -0.5131040437982135050 ) ) ;
#24648=CARTESIAN_POINT ( 'NONE',  ( 0.1049643490035303689, 0.3917322834645670104, -0.8654855643044619962 ) ) ;
#24653=CARTESIAN_POINT ( 'NONE',  ( -0.2867679344610364334, -0.2867679344610367109, -2.728346456692912536 ) ) ;
#24656=CARTESIAN_POINT ( 'NONE',  ( 0.3458507752293908943, -0.3458507752293908943, -0.9625984251968502381 ) ) ;
#24668=ORIENTED_EDGE ( 'NONE', *, *, #51709, .T. ) ;
#24669=CARTESIAN_POINT ( 'NONE',  ( -0.3996062992125986590, 0.1070741851644051723, -2.156824146981627166 ) ) ;
#24677=CARTESIAN_POINT ( 'NONE',  ( 4.893765752498283308E-17, -0.3996062992125985480, -0.7854330708661416693 ) ) ;
#24678=CARTESIAN_POINT ( 'NONE',  ( -0.2925321140481932924, 0.2925321140481931814, -0.8070866141732284671 ) ) ;
#24680=CARTESIAN_POINT ( 'NONE',  ( -0.1058382717557503211, 0.3949938075777409408, -0.3215223097112862027 ) ) ;
#24681=CARTESIAN_POINT ( 'NONE',  ( 0.3841287887292355596, 0.08106202739151233128, -1.220472440944881942 ) ) ;
#24686=CARTESIAN_POINT ( 'NONE',  ( 0.2891555358219910499, -0.2891555358219909944, -1.435039370078739829 ) ) ;
#24691=CARTESIAN_POINT ( 'NONE',  ( 0.1265901696524989462, 0.4724409448818897572, -1.725721784776903078 ) ) ;
#24692=CARTESIAN_POINT ( 'NONE',  ( -0.1070741851644051862, -0.3996062992125986590, -2.591863517060367439 ) ) ;
#24705=CARTESIAN_POINT ( 'NONE',  ( -0.3917322834645671215, 0.1049643490035301469, -1.284776902887139194 ) ) ;
#24708=CARTESIAN_POINT ( 'NONE',  ( 0.2891555358219910499, -0.2891555358219909944, -1.358267716535433101 ) ) ;
#24713=CARTESIAN_POINT ( 'NONE',  ( -0.1070741851644056997, 0.3996062992125986035, -0.1640419947506561726 ) ) ;
#24720=CARTESIAN_POINT ( 'NONE',  ( 4.797336870675656522E-17, -0.3917322834645670104, -0.005905511811023714773 ) ) ;
#24727=CARTESIAN_POINT ( 'NONE',  ( -0.3460692066303960868, 0.1998031496062990242, -2.073490813648294129 ) ) ;
#24730=CARTESIAN_POINT ( 'NONE',  ( -0.3996062992125984925, -0.1070741851644056858, -1.382545931758530022 ) ) ;
#24734=CARTESIAN_POINT ( 'NONE',  ( 0.3458507752293908943, -0.3458507752293908943, -1.043307086614173151 ) ) ;
#24736=CARTESIAN_POINT ( 'NONE',  ( -0.3392501089628019995, 0.1958661417322832277, -0.01837270341207344546 ) ) ;
#24738=CARTESIAN_POINT ( 'NONE',  ( -0.2867679344610366554, 0.2867679344610365444, -1.994094488188976388 ) ) ;
#24742=CARTESIAN_POINT ( 'NONE',  ( 4.893765752498283308E-17, -0.3996062992125985480, 0.1594488188976377896 ) ) ;
#24745=CARTESIAN_POINT ( 'NONE',  ( -0.1974969037888706924, 0.3420746716998658843, -2.452099737532808632 ) ) ;
#24754=CARTESIAN_POINT ( 'NONE',  ( 0.000000000000000000, 0.000000000000000000, -2.755905511811024056 ) ) ;
#24756=CYLINDRICAL_SURFACE ( 'NONE', #15614, 0.4724409448818898682 ) ;
#24764=CARTESIAN_POINT ( 'NONE',  ( -0.3996062992125984925, -0.1070741851644056858, -0.9101049868766404316 ) ) ;
#24765=CARTESIAN_POINT ( 'NONE',  ( -9.594673741351313045E-17, 0.3917322834645670104, -2.131889763779527769 ) ) ;
#24781=CARTESIAN_POINT ( 'NONE',  ( 0.1049643490035303689, 0.3917322834645670104, -1.967847769028871374 ) ) ;
#24785=CARTESIAN_POINT ( 'NONE',  ( -0.4724409448818904234, 0.1265901696524979470, -0.5052493438320210251 ) ) ;
#24788=CARTESIAN_POINT ( 'NONE',  ( 0.3460692066303959757, -0.1998031496062991907, -0.7349081364829396223 ) ) ;
#24789=EDGE_LOOP ( 'NONE', ( #23812, #28647, #66413, #44058 ) ) ;
#24791=CARTESIAN_POINT ( 'NONE',  ( 0.3917322834645670104, 2.398668435337828261E-17, -2.787401574803149096 ) ) ;
#24804=CARTESIAN_POINT ( 'NONE',  ( 0.1958661417322836440, -0.3392501089628017219, -2.696194225721784576 ) ) ;
#24807=CARTESIAN_POINT ( 'NONE',  ( 4.837279021331060870E-17, -0.3949938075777409963, -0.2362204724409449619 ) ) ;
#24814=CARTESIAN_POINT ( 'NONE',  ( -0.3917322834645671770, 0.1049643490035302024, -1.761830339403886336 ) ) ;
#24816=CARTESIAN_POINT ( 'NONE',  ( -0.3917322834645669549, -0.1049643490035306603, -2.492782152230970993 ) ) ;
#24821=CARTESIAN_POINT ( 'NONE',  ( 0.1998031496062994405, -0.3460692066303958092, -0.8792650918635170898 ) ) ;
#24823=CARTESIAN_POINT ( 'NONE',  ( -9.787531504996566615E-17, 0.3996062992125985480, -0.3917322834645669549 ) ) ;
#24825=CARTESIAN_POINT ( 'NONE',  ( -0.3996062992125987146, 0.1070741851644051862, -2.395013123359580387 ) ) ;
#24826=CARTESIAN_POINT ( 'NONE',  ( -0.3917322834645671215, 0.1049643490035301469, -1.849737532808399143 ) ) ;
#24830=CARTESIAN_POINT ( 'NONE',  ( -0.2362204724409447953, -0.4091458600556404646, -0.9297900262467192478 ) ) ;
#24833=CARTESIAN_POINT ( 'NONE',  ( -0.1974969037888706924, 0.3420746716998658843, -1.192257217847769279 ) ) ;
#24838=DIRECTION ( 'NONE',  ( 1.000000000000000000, 0.000000000000000000, 0.000000000000000000 ) ) ;
#24845=CARTESIAN_POINT ( 'NONE',  ( -0.1998031496062991630, -0.3460692066303959202, -1.874671916010498762 ) ) ;
#24858=EDGE_CURVE ( 'NONE', #36386, #24503, #55891, .T. ) ;
#24861=CARTESIAN_POINT ( 'NONE',  ( 0.1049643490035304938, -0.3917322834645669549, -1.114829396325459410 ) ) ;
#24870=CARTESIAN_POINT ( 'NONE',  ( 0.1265901696524990572, -0.4724409448818897017, -2.604986876640420057 ) ) ;
#24877=CARTESIAN_POINT ( 'NONE',  ( 5.785732909357575061E-17, -0.4724409448818898682, -0.5511811023622047445 ) ) ;
#24881=CARTESIAN_POINT ( 'NONE',  ( 4.797336870675656522E-17, -0.3917322834645670104, -1.960629921259842368 ) ) ;
#24884=CARTESIAN_POINT ( 'NONE',  ( -0.3458507752293909498, 0.3458507752293907833, -0.4921259842519684624 ) ) ;
#24885=CARTESIAN_POINT ( 'NONE',  ( -0.3420746716998659953, -0.1974969037888706647, -2.572178477690288734 ) ) ;
#24888=CARTESIAN_POINT ( 'NONE',  ( 4.797336870675656522E-17, -0.3917322834645670104, -1.173228346456692828 ) ) ;
#24890=CARTESIAN_POINT ( 'NONE',  ( -0.4724409448818899238, 0.1265901696524986686, -2.867454068241469756 ) ) ;
#24897=CARTESIAN_POINT ( 'NONE',  ( -0.1958661417322836440, 0.3392501089628016664, -0.8805581120396831496 ) ) ;
#24904=CARTESIAN_POINT ( 'NONE',  ( 0.3392501089628018884, -0.1958661417322833942, -2.148969447015434575 ) ) ;
#24912=CARTESIAN_POINT ( 'NONE',  ( 0.2867679344610365999, 0.2867679344610365999, -1.324803149606299302 ) ) ;
#24922=CARTESIAN_POINT ( 'NONE',  ( 0.2867679344610365999, 0.2867679344610365999, -2.807086614173227357 ) ) ;
#24928=CARTESIAN_POINT ( 'NONE',  ( -0.1958661417322836718, 0.3392501089628017219, -1.200131233595800540 ) ) ;
#24929=CARTESIAN_POINT ( 'NONE',  ( -0.4724409448818895907, -0.1265901696524993070, 0.03477690288713909672 ) ) ;
#24930=CARTESIAN_POINT ( 'NONE',  ( 0.1058382717557500852, -0.3949938075777408852, 0.1528871391076115638 ) ) ;
#24939=CARTESIAN_POINT ( 'NONE',  ( -0.1998031496062994405, 0.3460692066303957537, -0.4048556430446194621 ) ) ;
#24941=CARTESIAN_POINT ( 'NONE',  ( -0.3917322834645669549, -0.1049643490035306603, -0.3530183727034120755 ) ) ;
#24955=CARTESIAN_POINT ( 'NONE',  ( 4.797336870675656522E-17, -0.3917322834645670659, -0.7053998932096606778 ) ) ;
#24960=CARTESIAN_POINT ( 'NONE',  ( -0.4724409448818895907, -0.1265901696524993070, -2.327427821522309426 ) ) ;
#24975=ORIENTED_EDGE ( 'NONE', *, *, #63009, .F. ) ;
#24977=( BOUNDED_CURVE ( )  B_SPLINE_CURVE ( 2, ( #10413, #11649, #36070, #30978, #44015, #61742, #4907, #23022, #29746, #68477, #17553, #68882, #75209 ),
 .UNSPECIFIED., .F., .F. ) 
 B_SPLINE_CURVE_WITH_KNOTS ( ( 3, 2, 2, 2, 2, 2, 3 ),
 ( 0.1375000000000000111, 0.1416666666666666630, 0.1458333333333333426, 0.1499999999999999944, 0.1541666666666666741, 0.1583333333333333259, 0.1625000000000000056 ),
 .UNSPECIFIED. ) 
 CURVE ( )  GEOMETRIC_REPRESENTATION_ITEM ( )  RATIONAL_B_SPLINE_CURVE ( ( 1.000000000000000000, 0.9659258262890683122, 1.000000000000000000, 0.9659258262890683122, 1.000000000000000000, 0.9659258262890683122, 1.000000000000000000, 0.9659258262890683122, 1.000000000000000000, 0.9659258262890683122, 1.000000000000000000, 0.9659258262890683122, 1.000000000000000000 ) ) 
 REPRESENTATION_ITEM ( '' )  );
#24980=CARTESIAN_POINT ( 'NONE',  ( -0.3460692066303960868, 0.1998031496062990242, -0.1837270341207349333 ) ) ;
#24981=CARTESIAN_POINT ( 'NONE',  ( -0.2925321140481930149, -0.2925321140481933480, -2.812992125984251857 ) ) ;
#24987=CARTESIAN_POINT ( 'NONE',  ( 0.1998031496062994405, -0.3460692066303958092, -2.139107611548556331 ) ) ;
#24988=CARTESIAN_POINT ( 'NONE',  ( -0.2891555358219908833, -0.2891555358219912164, -1.633858267716535195 ) ) ;
#24989=CARTESIAN_POINT ( 'NONE',  ( 0.3996062992125986590, -0.1070741851644053111, -2.946194225721785465 ) ) ;
#24991=CARTESIAN_POINT ( 'NONE',  ( -0.1049643490035301885, -0.3917322834645671215, -0.5367454068241467313 ) ) ;
#24995=CARTESIAN_POINT ( 'NONE',  ( 0.1058382717557499880, 0.3949938075777409408, -2.432414698162729927 ) ) ;
#24999=CARTESIAN_POINT ( 'NONE',  ( -0.4091458600556402980, -0.2362204724409451284, -2.887139107611548461 ) ) ;
#25001=CARTESIAN_POINT ( 'NONE',  ( 0.1998031496062994405, -0.3460692066303958092, -1.981627296587926690 ) ) ;
#25009=CARTESIAN_POINT ( 'NONE',  ( -0.3917322834645671215, 0.1049643490035301469, -0.1174540682414699083 ) ) ;
#25016=CARTESIAN_POINT ( 'NONE',  ( -0.1049643490035307020, 0.3917322834645669549, -0.7211286089238846397 ) ) ;
#25017=CARTESIAN_POINT ( 'NONE',  ( 0.3392501089628018884, -0.1958661417322834220, -1.514435695538058013 ) ) ;
#25018=CARTESIAN_POINT ( 'NONE',  ( -0.2867679344610365999, 0.2867679344610364889, -2.531496062992125484 ) ) ;
#25020=CARTESIAN_POINT ( 'NONE',  ( -9.787531504996567848E-17, 0.3996062992125986035, -1.920830620545185230E-17 ) ) ;
#25021=ORIENTED_EDGE ( 'NONE', *, *, #13910, .F. ) ;
#25025=CARTESIAN_POINT ( 'NONE',  ( -0.1998031496062994683, 0.3460692066303958092, -1.587926509186351698 ) ) ;
#25030=CARTESIAN_POINT ( 'NONE',  ( 0.1049643490035304938, -0.3917322834645669549, -0.3274278215223098143 ) ) ;
#25039=CARTESIAN_POINT ( 'NONE',  ( -0.4724409448818898682, -8.678599364036362592E-17, -2.244094488188976388 ) ) ;
#25045=CARTESIAN_POINT ( 'NONE',  ( 0.4724409448818898682, 2.892866454678787531E-17, -2.322834645669291209 ) ) ;
#25049=CARTESIAN_POINT ( 'NONE',  ( 0.1958661417322836162, -0.3392501089628018329, -0.4868573246381086017 ) ) ;
#25051=CARTESIAN_POINT ( 'NONE',  ( 0.3392501089628018329, 0.1958661417322835607, -0.8458005249343831800 ) ) ;
#25056=CARTESIAN_POINT ( 'NONE',  ( 0.3917322834645670104, 2.398668435337828261E-17, -2.944881889763779181 ) ) ;
#25060=CARTESIAN_POINT ( 'NONE',  ( -0.2362204724409447953, -0.4091458600556404646, -1.402230971128609172 ) ) ;
#25073=CARTESIAN_POINT ( 'NONE',  ( -0.3460692066303960313, 0.1998031496062989965, -2.465223097112860806 ) ) ;
#25077=CARTESIAN_POINT ( 'NONE',  ( -0.1998031496062991630, -0.3460692066303959202, -1.559711286089239035 ) ) ;
#25083=CARTESIAN_POINT ( 'NONE',  ( 0.3460692066303959202, -0.1998031496062991630, -0.4967191601049869010 ) ) ;
#25085=CARTESIAN_POINT ( 'NONE',  ( -0.2925321140481932924, 0.2925321140481931814, -1.122047244094488194 ) ) ;
#25086=CARTESIAN_POINT ( 'NONE',  ( -0.1058382717557503211, 0.3949938075777409408, -0.1640419947506562559 ) ) ;
#25091=CARTESIAN_POINT ( 'NONE',  ( -0.4724409448818898682, -8.678599364036362592E-17, -2.320866141732283783 ) ) ;
#25093=CARTESIAN_POINT ( 'NONE',  ( -0.3949938075777408852, -0.1058382717557502933, -1.225065616797900159 ) ) ;
#25098=CARTESIAN_POINT ( 'NONE',  ( 0.2362204724409449064, 0.4091458600556404646, -1.561679790026246684 ) ) ;
#25099=CARTESIAN_POINT ( 'NONE',  ( -0.3460692066303960868, 0.1998031496062990242, -2.703412073490813583 ) ) ;
#25100=ORIENTED_EDGE ( 'NONE', *, *, #30797, .F. ) ;
#25112=CARTESIAN_POINT ( 'NONE',  ( -0.1049643490035307020, 0.3917322834645669549, -1.258530183727033958 ) ) ;
#25115=CARTESIAN_POINT ( 'NONE',  ( -0.2891555358219911054, 0.2891555358219909388, -2.066929133858268042 ) ) ;
#25116=ORIENTED_EDGE ( 'NONE', *, *, #26304, .F. ) ;
#25122=CARTESIAN_POINT ( 'NONE',  ( -0.1070741851644051862, -0.3996062992125987146, -0.2296587926509186250 ) ) ;
#25129=CARTESIAN_POINT ( 'NONE',  ( -0.3917322834645671215, 0.1049643490035301469, -0.1174540682414699083 ) ) ;
#25137=CARTESIAN_POINT ( 'NONE',  ( -0.1998031496062991630, -0.3460692066303959202, -1.402230971128609172 ) ) ;
#25142=CARTESIAN_POINT ( 'NONE',  ( 0.4724409448818897572, -0.1265901696524988906, -1.056430446194225992 ) ) ;
#25145=CARTESIAN_POINT ( 'NONE',  ( 0.3917322834645670104, 2.398668435337828261E-17, -2.879921259842519454 ) ) ;
#25147=CARTESIAN_POINT ( 'NONE',  ( 0.3392501089628018884, -0.1958661417322834220, -2.079396325459317740 ) ) ;
#25151=CARTESIAN_POINT ( 'NONE',  ( 0.3458507752293908943, -0.3458507752293908943, -2.694881889763780070 ) ) ;
#25154=CARTESIAN_POINT ( 'NONE',  ( 0.1974969037888706092, -0.3420746716998660508, -2.215879265091863726 ) ) ;
#25163=CARTESIAN_POINT ( 'NONE',  ( -1.157146581871515012E-16, 0.4724409448818898682, 0.2381889763779527491 ) ) ;
#25176=CARTESIAN_POINT ( 'NONE',  ( 0.3460692066303958092, 0.1998031496062993018, -0.6804461942257218343 ) ) ;
#25178=CARTESIAN_POINT ( 'NONE',  ( -9.594673741351313045E-17, 0.3917322834645670104, -2.446850393700787496 ) ) ;
#25188=DIRECTION ( 'NONE',  ( 0.000000000000000000, 0.000000000000000000, 1.000000000000000000 ) ) ;
#25190=CARTESIAN_POINT ( 'NONE',  ( -0.1049643490035302301, -0.3917322834645671770, -2.273641363025933781 ) ) ;
#25196=CARTESIAN_POINT ( 'NONE',  ( 0.3392501089628018884, -0.1958661417322834220, -2.079396325459317740 ) ) ;
#25197=CARTESIAN_POINT ( 'NONE',  ( -0.02544847934398350789, 0.3910482532979367432, -1.220472440944882164 ) ) ;
#25200=LINE ( 'NONE', #82470, #5932 ) ;
#25201=CARTESIAN_POINT ( 'NONE',  ( 0.3996062992125984925, 0.1070741851644054499, -2.721128608923884862 ) ) ;
#25203=CARTESIAN_POINT ( 'NONE',  ( -0.3460692066303960868, 0.1998031496062990242, -1.443569553805774230 ) ) ;
#25205=CARTESIAN_POINT ( 'NONE',  ( -0.1049643490035307158, 0.3917322834645670104, 0.1541801592837776513 ) ) ;
#25217=CARTESIAN_POINT ( 'NONE',  ( -0.3917322834645671215, 0.1049643490035301469, -0.02493438320209968861 ) ) ;
#25220=CARTESIAN_POINT ( 'NONE',  ( 0.3949938075777411073, -0.1058382717557499464, -0.1115485564304462551 ) ) ;
#25223=LINE ( 'NONE', #50889, #60987 ) ;
#25228=CARTESIAN_POINT ( 'NONE',  ( -9.594673741351313045E-17, 0.3917322834645670659, -1.886502255414385099 ) ) ;
#25230=CARTESIAN_POINT ( 'NONE',  ( -0.1958661417322836718, 0.3392501089628017219, -2.617454068241469756 ) ) ;
#25234=CARTESIAN_POINT ( 'NONE',  ( -0.3996062992125986035, -7.340648628747425578E-17, -0.9842519685039369248 ) ) ;
#25236=CARTESIAN_POINT ( 'NONE',  ( 0.3996062992125984925, 0.1070741851644054637, -0.5164041994750655507 ) ) ;
#25237=CARTESIAN_POINT ( 'NONE',  ( 0.2925321140481932369, -0.2925321140481931814, -0.01771653543307089712 ) ) ;
#25239=CARTESIAN_POINT ( 'NONE',  ( -0.3460692066303958092, -0.1998031496062994683, -2.729658792650918375 ) ) ;
#25240=CARTESIAN_POINT ( 'NONE',  ( -0.3392501089628019995, 0.1958661417322832277, -1.843175853018372834 ) ) ;
#25246=CARTESIAN_POINT ( 'NONE',  ( -1.157146581871515012E-16, 0.4724409448818898682, -1.494094488188976388 ) ) ;
#25249=CARTESIAN_POINT ( 'NONE',  ( -0.1058382717557503072, 0.3949938075777408852, -1.028215223097112885 ) ) ;
#25259=CARTESIAN_POINT ( 'NONE',  ( -0.3460692066303960313, 0.1998031496062989965, -1.992782152230971437 ) ) ;
#25273=CARTESIAN_POINT ( 'NONE',  ( -0.3917322834645670104, -7.196005306013484475E-17, -0.9114173228346457156 ) ) ;
#25289=CARTESIAN_POINT ( 'NONE',  ( -0.2362204724409447953, -0.4091458600556404646, -0.5380577427821522374 ) ) ;
#25293=CARTESIAN_POINT ( 'NONE',  ( -0.2867679344610364334, -0.2867679344610367109, -2.098425196850393970 ) ) ;
#25296=CARTESIAN_POINT ( 'NONE',  ( 0.4724409448818898682, 2.892866454678787531E-17, -0.2755905511811023723 ) ) ;
#25297=CARTESIAN_POINT ( 'NONE',  ( 4.837279021331060870E-17, -0.3949938075777409963, -2.598425196850393970 ) ) ;
#25300=CARTESIAN_POINT ( 'NONE',  ( 0.3917322834645670104, -0.1049643490035303411, -1.520997375328083656 ) ) ;
#25303=CARTESIAN_POINT ( 'NONE',  ( -0.02190130575838357754, 0.3959418824714266427, -2.755905511811024500 ) ) ;
#25306=CARTESIAN_POINT ( 'NONE',  ( -9.787531504996567848E-17, 0.3996062992125986035, -1.920830620545185230E-17 ) ) ;
#25311=CARTESIAN_POINT ( 'NONE',  ( -0.1958661417322836440, 0.3392501089628016664, -0.5655974821184234225 ) ) ;
#25316=CARTESIAN_POINT ( 'NONE',  ( -0.2017716535433071445, -0.2017716535433071445, -0.3937007874015748254 ) ) ;
#25317=VERTEX_POINT ( 'NONE', #79853 ) ;
#25318=CARTESIAN_POINT ( 'NONE',  ( -0.1958661417322836995, 0.3392501089628017219, -2.057105929955067580 ) ) ;
#25325=CARTESIAN_POINT ( 'NONE',  ( 0.1958661417322834775, 0.3392501089628018884, -1.331364829396325611 ) ) ;
#25335=CARTESIAN_POINT ( 'NONE',  ( 0.1958661417322834775, 0.3392501089628018884, -2.813648293963254776 ) ) ;
#25342=DIRECTION ( 'NONE',  ( 1.000000000000000000, 0.000000000000000000, -0.000000000000000000 ) ) ;
#25343=CARTESIAN_POINT ( 'NONE',  ( 4.797336870675656522E-17, -0.3917322834645670104, -1.265748031496062964 ) ) ;
#25344=CARTESIAN_POINT ( 'NONE',  ( 0.3458507752293908943, 0.3458507752293908943, -0.2145669291338583029 ) ) ;
#25347=CARTESIAN_POINT ( 'NONE',  ( -0.1998031496062994405, 0.3460692066303957537, -2.767060367454068359 ) ) ;
#25352=CARTESIAN_POINT ( 'NONE',  ( 0.3949938075777408852, 0.1058382717557500435, -0.04396325459317585588 ) ) ;
#25356=CARTESIAN_POINT ( 'NONE',  ( -0.4724409448818898682, -8.678599364036362592E-17, -0.9842519685039369248 ) ) ;
#25359=CARTESIAN_POINT ( 'NONE',  ( 0.3996062992125985480, 2.446882876249141654E-17, -0.3523622047244094335 ) ) ;
#25361=CARTESIAN_POINT ( 'NONE',  ( 0.3392501089628018329, 0.1958661417322835607, -0.2808398950131232863 ) ) ;
#25374=CARTESIAN_POINT ( 'NONE',  ( -0.2867679344610367109, 0.2867679344610365444, -0.8038250900600545368 ) ) ;
#25378=CARTESIAN_POINT ( 'NONE',  ( 0.3458507752293908943, 0.3458507752293908943, -2.419291338582676865 ) ) ;
#25396=CARTESIAN_POINT ( 'NONE',  ( -0.2925321140481932369, 0.2925321140481931814, -0.4921259842519684624 ) ) ;
#25397=CARTESIAN_POINT ( 'NONE',  ( 0.1070741851644054776, -0.3996062992125984925, -2.839238845144356649 ) ) ;
#25403=CARTESIAN_POINT ( 'NONE',  ( 0.3996062992125986035, 0.1070741851644054776, -2.171916010498687211 ) ) ;
#25404=CARTESIAN_POINT ( 'NONE',  ( 0.3420746716998660508, -0.1974969037888703871, -1.522309711286089273 ) ) ;
#25405=CARTESIAN_POINT ( 'NONE',  ( -0.3996062992125986035, -7.340648628747425578E-17, -2.874015748031495843 ) ) ;
#25407=CARTESIAN_POINT ( 'NONE',  ( -0.2867679344610364334, -0.2867679344610367109, -0.8385826771653541734 ) ) ;
#25410=CARTESIAN_POINT ( 'NONE',  ( 0.2891555358219910499, -0.2891555358219909944, -2.537401574803150428 ) ) ;
#25414=CARTESIAN_POINT ( 'NONE',  ( -0.1265901696524986964, -0.4724409448818899238, -2.906824146981627610 ) ) ;
#25415=CARTESIAN_POINT ( 'NONE',  ( 0.1998031496062992740, 0.3460692066303959757, -2.034120734908136718 ) ) ;
#25421=CARTESIAN_POINT ( 'NONE',  ( -0.1049643490035307020, 0.3917322834645669549, -0.09120734908136493568 ) ) ;
#25429=CARTESIAN_POINT ( 'NONE',  ( -0.3392501089628019995, 0.1958661417322832277, -0.4258530183727035068 ) ) ;
#25430=CARTESIAN_POINT ( 'NONE',  ( -0.3917322834645669549, -0.1049643490035306603, -1.612860892388451539 ) ) ;
#25431=CARTESIAN_POINT ( 'NONE',  ( -0.3392501089628019995, 0.1958661417322832277, -2.538057742782152015 ) ) ;
#25433=CARTESIAN_POINT ( 'NONE',  ( -0.3996062992125987146, 0.1070741851644051862, -0.03280839895013124702 ) ) ;
#25434=ORIENTED_EDGE ( 'NONE', *, *, #33217, .T. ) ;
#25437=CARTESIAN_POINT ( 'NONE',  ( -0.3996062992125986035, -7.340648628747425578E-17, -1.614173228346456712 ) ) ;
#25441=CARTESIAN_POINT ( 'NONE',  ( 0.3808816823641231752, -0.09156050430092187165, -1.929133858267716661 ) ) ;
#25442=CARTESIAN_POINT ( 'NONE',  ( -0.1958661417322836718, 0.3392501089628017219, -0.8851706036745407014 ) ) ;
#25445=EDGE_CURVE ( 'NONE', #37037, #25602, #79025, .T. ) ;
#25451=CARTESIAN_POINT ( 'NONE',  ( -0.2362204724409447953, -0.4091458600556404646, -1.955380577427821454 ) ) ;
#25462=CARTESIAN_POINT ( 'NONE',  ( 0.1958661417322834497, 0.3392501089628018329, -1.011791707840208332 ) ) ;
#25464=CARTESIAN_POINT ( 'NONE',  ( 0.3917322834645670104, 2.398668435337828261E-17, -0.6751968503937009203 ) ) ;
#25470=CARTESIAN_POINT ( 'NONE',  ( 0.3917322834645670104, -0.1049643490035303411, -2.623359580052493367 ) ) ;
#25473=CARTESIAN_POINT ( 'NONE',  ( 0.2362204724409451007, -0.4091458600556402980, -1.113517060367454015 ) ) ;
#25480=CARTESIAN_POINT ( 'NONE',  ( 0.000000000000000000, 0.000000000000000000, -2.755905511811024056 ) ) ;
#25486=CARTESIAN_POINT ( 'NONE',  ( 0.2925321140481932369, -0.2925321140481931814, -2.379921259842520342 ) ) ;
#25490=CARTESIAN_POINT ( 'NONE',  ( -9.787531504996566615E-17, 0.3996062992125985480, -1.494094488188976610 ) ) ;
#25496=CARTESIAN_POINT ( 'NONE',  ( 0.1070741851644053527, 0.3996062992125985480, -0.7001312335958003175 ) ) ;
#25497=CARTESIAN_POINT ( 'NONE',  ( -0.1070741851644051862, -0.3996062992125987146, -0.8595800524934383846 ) ) ;
#25499=CARTESIAN_POINT ( 'NONE',  ( -0.3949938075777411628, 0.1058382717557497937, -0.1902887139107612702 ) ) ;
#25505=CARTESIAN_POINT ( 'NONE',  ( 0.1058382717557500852, -0.3949938075777408852, -1.421916010498688099 ) ) ;
#25511=CARTESIAN_POINT ( 'NONE',  ( -0.4091458600556402980, -0.2362204724409451284, -1.469816272965879245 ) ) ;
#25512=CARTESIAN_POINT ( 'NONE',  ( -0.1998031496062991907, -0.3460692066303959757, -2.585301837270341352 ) ) ;
#25519=CARTESIAN_POINT ( 'NONE',  ( -0.3392501089628019439, 0.1958661417322832554, -1.838563361383515504 ) ) ;
#25526=CARTESIAN_POINT ( 'NONE',  ( -0.3917322834645669549, -0.1049643490035306603, -1.612860892388451539 ) ) ;
#25529=CARTESIAN_POINT ( 'NONE',  ( 0.3420746716998659953, 0.1974969037888705536, -1.706036745406824151 ) ) ;
#25534=CARTESIAN_POINT ( 'NONE',  ( -0.3996062992125986035, -0.1070741851644056997, -0.2034120734908136108 ) ) ;
#25541=CARTESIAN_POINT ( 'NONE',  ( 0.1049643490035303689, 0.3917322834645670104, -0.3930446194225722945 ) ) ;
#25548=CARTESIAN_POINT ( 'NONE',  ( -0.1998031496062994405, 0.3460692066303957537, -1.822178477690288512 ) ) ;
#25553=CARTESIAN_POINT ( 'NONE',  ( -0.3458507752293909498, 0.3458507752293907833, -0.9645669291338579976 ) ) ;
#25555=CARTESIAN_POINT ( 'NONE',  ( -0.1958661417322836718, 0.3392501089628017219, 0.1522309711286089495 ) ) ;
#25556=CARTESIAN_POINT ( 'NONE',  ( -0.3392501089628017219, -0.1958661417322836718, -2.026902887139107712 ) ) ;
#25560=CARTESIAN_POINT ( 'NONE',  ( 0.4724409448818898682, 2.892866454678787531E-17, -2.714566929133858331 ) ) ;
#25565=CARTESIAN_POINT ( 'NONE',  ( -0.3949938075777409963, -7.255918531996591613E-17, -2.635826771653543954 ) ) ;
#25567=APPLICATION_CONTEXT ( 'automotive_design' ) ;
#25573=CARTESIAN_POINT ( 'NONE',  ( 0.1958661417322834775, 0.3392501089628018884, -1.396325459317585338 ) ) ;
#25576=CARTESIAN_POINT ( 'NONE',  ( 0.4724409448818898682, 2.892866454678787531E-17, -0.03740157480314962313 ) ) ;
#25589=CARTESIAN_POINT ( 'NONE',  ( 0.2925321140481932369, 0.2925321140481932369, -1.001968503937007871 ) ) ;
#25590=CARTESIAN_POINT ( 'NONE',  ( 4.797336870675656522E-17, -0.3917322834645670104, -2.368110236220472675 ) ) ;
#25601=CARTESIAN_POINT ( 'NONE',  ( -9.594673741351313045E-17, 0.3917322834645670659, -2.043982570375014962 ) ) ;
#25602=VERTEX_POINT ( 'NONE', #23819 ) ;
#25607=CARTESIAN_POINT ( 'NONE',  ( -0.3917322834645670104, -7.196005306013484475E-17, -2.013779527559055094 ) ) ;
#25608=CARTESIAN_POINT ( 'NONE',  ( -0.1778467755331564759, 0.3496712940256280211, -1.220472440944882164 ) ) ;
#25611=CARTESIAN_POINT ( 'NONE',  ( 0.4724409448818898682, 2.892866454678787531E-17, -2.557086614173228689 ) ) ;
#25612=CARTESIAN_POINT ( 'NONE',  ( 0.1998031496062994128, -0.3460692066303957537, -2.688320209973753538 ) ) ;
#25614=CARTESIAN_POINT ( 'NONE',  ( -9.787531504996567848E-17, 0.3996062992125986035, -1.259842519685039353 ) ) ;
#25616=CARTESIAN_POINT ( 'NONE',  ( -0.2867679344610364334, -0.2867679344610367109, -2.885826771653543066 ) ) ;
#25630=CARTESIAN_POINT ( 'NONE',  ( 0.3917322834645670104, -0.1049643490035303411, -0.1036745406824146343 ) ) ;
#25633=CARTESIAN_POINT ( 'NONE',  ( -0.2891555358219911054, 0.2891555358219909388, -0.6496062992125984925 ) ) ;
#25641=CARTESIAN_POINT ( 'NONE',  ( 0.3392501089628018884, -0.1958661417322833942, -1.676528502133545206 ) ) ;
#25643=CARTESIAN_POINT ( 'NONE',  ( -0.1049643490035307020, 0.3917322834645669549, -2.610892388451443225 ) ) ;
#25648=CARTESIAN_POINT ( 'NONE',  ( 0.3460692066303959202, 0.1998031496062993295, -0.7611548556430446366 ) ) ;
#25650=CARTESIAN_POINT ( 'NONE',  ( 0.3460692066303958092, 0.1998031496062993018, -0.8379265091863516979 ) ) ;
#25651=CARTESIAN_POINT ( 'NONE',  ( -0.1998031496062994405, 0.3460692066303957537, 0.06758530183727032292 ) ) ;
#25653=CARTESIAN_POINT ( 'NONE',  ( -0.1998031496062994683, 0.3460692066303958092, -2.532808398950130879 ) ) ;
#25654=CARTESIAN_POINT ( 'NONE',  ( 0.1958661417322834775, 0.3392501089628018884, -1.803805774278215202 ) ) ;
#25660=CARTESIAN_POINT ( 'NONE',  ( 5.785732909357575061E-17, -0.4724409448818898682, -1.415354330708661346 ) ) ;
#25664=CARTESIAN_POINT ( 'NONE',  ( -9.674558042662122972E-17, 0.3949938075777409963, -1.021653543307086798 ) ) ;
#25674=CARTESIAN_POINT ( 'NONE',  ( -0.3460692066303957537, -0.1998031496062994405, -2.176509186351706315 ) ) ;
#25676=CARTESIAN_POINT ( 'NONE',  ( -0.3917322834645668994, -0.1049643490035306742, -1.700768085792964346 ) ) ;
#25687=CARTESIAN_POINT ( 'NONE',  ( 0.3460692066303958092, 0.1998031496062993018, -0.05052493438320210251 ) ) ;
#25689=CARTESIAN_POINT ( 'NONE',  ( -0.3917322834645669549, -0.1049643490035306603, -0.9179790026246721357 ) ) ;
#25710=CARTESIAN_POINT ( 'NONE',  ( 0.3392501089628018884, -0.1958661417322834220, -2.616797900262466836 ) ) ;
#25713=CARTESIAN_POINT ( 'NONE',  ( 0.3458507752293908943, 0.3458507752293908943, -0.9251968503937008093 ) ) ;
#25714=CARTESIAN_POINT ( 'NONE',  ( 0.2925321140481932369, 0.2925321140481932369, 0.01968503937007872254 ) ) ;
#25717=CARTESIAN_POINT ( 'NONE',  ( -0.2867679344610365999, 0.2867679344610364889, -1.744094488188976610 ) ) ;
#25718=VERTEX_POINT ( 'NONE', #49489 ) ;
#25720=CARTESIAN_POINT ( 'NONE',  ( -0.2362204724409447953, -0.4091458600556404646, -2.742782152230971437 ) ) ;
#25727=CARTESIAN_POINT ( 'NONE',  ( 0.3392501089628018329, -0.1958661417322834497, -0.9724216291000506995 ) ) ;
#25734=CARTESIAN_POINT ( 'NONE',  ( -0.3917322834645671770, 0.1049643490035302024, -2.391751599246406457 ) ) ;
#25742=CARTESIAN_POINT ( 'NONE',  ( 4.797336870675656522E-17, -0.3917322834645670104, -1.423228346456693050 ) ) ;
#25746=CARTESIAN_POINT ( 'NONE',  ( -0.001150535885505079474, 0.3985446848723406821, -3.148631409696655085E-18 ) ) ;
#25750=LINE ( 'NONE', #13566, #9338 ) ;
#25753=VERTEX_POINT ( 'NONE', #48659 ) ;
#25758=CARTESIAN_POINT ( 'NONE',  ( -0.2867679344610365999, 0.2867679344610364889, -1.049212598425196763 ) ) ;
#25759=CARTESIAN_POINT ( 'NONE',  ( -0.1265901696524993347, 0.4724409448818895907, -0.3982939632545932085 ) ) ;
#25762=CARTESIAN_POINT ( 'NONE',  ( -9.674558042662122972E-17, 0.3949938075777409963, 0.08070866141732281618 ) ) ;
#25768=CARTESIAN_POINT ( 'NONE',  ( 0.3420746716998660508, -0.1974969037888704149, -0.1817585301837270073 ) ) ;
#25775=CARTESIAN_POINT ( 'NONE',  ( -9.787531504996566615E-17, 0.3996062992125985480, -0.8641732283464567121 ) ) ;
#25777=CARTESIAN_POINT ( 'NONE',  ( -0.2867679344610364334, -0.2867679344610367109, -0.6811023622047243098 ) ) ;
#25795=CARTESIAN_POINT ( 'NONE',  ( 0.4724409448818896462, 0.1265901696524990294, -2.406167979002624246 ) ) ;
#25812=CARTESIAN_POINT ( 'NONE',  ( -0.1070741851644057135, 0.3996062992125985480, -0.1640419947506562004 ) ) ;
#25813=CARTESIAN_POINT ( 'NONE',  ( -0.1998031496062991630, -0.3460692066303959202, -2.662073490813648746 ) ) ;
#25818=CARTESIAN_POINT ( 'NONE',  ( -0.3460692066303958092, -0.1998031496062994683, -2.099737532808398921 ) ) ;
#25819=CARTESIAN_POINT ( 'NONE',  ( 0.2891555358219910499, -0.2891555358219909944, -1.988188976377952777 ) ) ;
#25820=CARTESIAN_POINT ( 'NONE',  ( -0.3917322834645669549, -0.1049643490035306603, -0.3530183727034120755 ) ) ;
#25822=CARTESIAN_POINT ( 'NONE',  ( -0.1049643490035301885, -0.3917322834645671215, -1.009186351706036433 ) ) ;
#25826=CARTESIAN_POINT ( 'NONE',  ( -0.2891555358219911054, 0.2891555358219909388, -2.458661417322835163 ) ) ;
#25830=CARTESIAN_POINT ( 'NONE',  ( -0.2362204724409451284, 0.4091458600556402425, -2.690288713910760965 ) ) ;
#25831=CARTESIAN_POINT ( 'NONE',  ( 0.1998031496062992740, 0.3460692066303959757, -2.191601049868766360 ) ) ;
#25832=CARTESIAN_POINT ( 'NONE',  ( 0.3392501089628018329, 0.1958661417322835607, -0.6004130165692406207 ) ) ;
#25838=CARTESIAN_POINT ( 'NONE',  ( 0.1049643490035304938, -0.3917322834645669549, -0.3274278215223098143 ) ) ;
#25846=CARTESIAN_POINT ( 'NONE',  ( -0.3917322834645669549, -0.1049643490035306603, -0.7604986876640419391 ) ) ;
#25847=CARTESIAN_POINT ( 'NONE',  ( 4.797336870675656522E-17, -0.3917322834645670104, -1.488188976377952777 ) ) ;
#25848=CARTESIAN_POINT ( 'NONE',  ( -0.3917322834645670104, -7.196005306013484475E-17, -2.866141732283464361 ) ) ;
#25850=CARTESIAN_POINT ( 'NONE',  ( -0.3996062992125986035, -0.1070741851644056997, -0.04593175853018374721 ) ) ;
#25854=CARTESIAN_POINT ( 'NONE',  ( -0.2925321140481932924, 0.2925321140481931814, -1.437007874015747921 ) ) ;
#25859=CARTESIAN_POINT ( 'NONE',  ( -0.1265901696524986964, -0.4724409448818899238, -1.174540682414698445 ) ) ;
#25860=CARTESIAN_POINT ( 'NONE',  ( 0.3917322834645670104, 2.398668435337828261E-17, -0.8326771653543307838 ) ) ;
#25867=CARTESIAN_POINT ( 'NONE',  ( -0.4724409448818895907, -0.1265901696524993070, -2.093175853018372834 ) ) ;
#25873=ORIENTED_EDGE ( 'NONE', *, *, #15671, .F. ) ;
#25878=CARTESIAN_POINT ( 'NONE',  ( -0.1049643490035301746, -0.3917322834645670659, -0.7821329151892896236 ) ) ;
#25882=CARTESIAN_POINT ( 'NONE',  ( 0.2867679344610366554, -0.2867679344610365444, -0.9704724409448819422 ) ) ;
#25888=CARTESIAN_POINT ( 'NONE',  ( 0.1958661417322836440, -0.3392501089628017219, -2.603674540682414218 ) ) ;
#25892=CARTESIAN_POINT ( 'NONE',  ( -0.3458507752293906723, -0.3458507752293910609, -1.080708661417322691 ) ) ;
#25904=CARTESIAN_POINT ( 'NONE',  ( 0.3996062992125986035, -0.1070741851644052972, -2.550524934383202158 ) ) ;
#25909=CARTESIAN_POINT ( 'NONE',  ( -0.2925321140481932369, 0.2925321140481931259, -1.356299212598425452 ) ) ;
#25916=CARTESIAN_POINT ( 'NONE',  ( -0.1070741851644051862, -0.3996062992125986035, -0.7788713910761155823 ) ) ;
#25917=CARTESIAN_POINT ( 'NONE',  ( 0.3460692066303959202, 0.1998031496062993295, -0.9186351706036745002 ) ) ;
#25918=CARTESIAN_POINT ( 'NONE',  ( 0.1974969037888706369, -0.3420746716998659953, -0.2493438320209974690 ) ) ;
#25926=CARTESIAN_POINT ( 'NONE',  ( 0.3420746716998660508, 0.1974969037888705814, -1.467847769028871374 ) ) ;
#25931=CARTESIAN_POINT ( 'NONE',  ( 0.4724409448818898682, 2.892866454678787531E-17, -1.535433070866141669 ) ) ;
#25932=CARTESIAN_POINT ( 'NONE',  ( 0.3996062992125985480, 0.1070741851644054637, -2.644356955380577467 ) ) ;
#25934=ORIENTED_EDGE ( 'NONE', *, *, #13593, .F. ) ;
#25939=CARTESIAN_POINT ( 'NONE',  ( -0.3917322834645670659, 0.1049643490035301607, -2.002605356134171455 ) ) ;
#25946=CARTESIAN_POINT ( 'NONE',  ( 0.2867679344610365999, 0.2867679344610365999, -1.547244094488189115 ) ) ;
#25949=CARTESIAN_POINT ( 'NONE',  ( 4.837279021331060870E-17, -0.3949938075777409963, -1.968503937007873850 ) ) ;
#25954=CARTESIAN_POINT ( 'NONE',  ( -0.3460692066303960868, 0.1998031496062990242, -0.3412073490813647969 ) ) ;
#25957=( NAMED_UNIT ( * ) SI_UNIT ( $, .STERADIAN. ) SOLID_ANGLE_UNIT ( ) );
#25961=CARTESIAN_POINT ( 'NONE',  ( 0.3917322834645670104, -0.1049643490035303411, -0.1961942257217848817 ) ) ;
#25968=CARTESIAN_POINT ( 'NONE',  ( 0.2925321140481932369, 0.2925321140481932369, -2.104330708661417138 ) ) ;
#25973=CARTESIAN_POINT ( 'NONE',  ( 0.4091458600556404646, -0.2362204724409448231, -0.7349081364829396223 ) ) ;
#25976=CARTESIAN_POINT ( 'NONE',  ( 0.1958661417322834775, 0.3392501089628018884, -0.1364829396325459021 ) ) ;
#25981=CARTESIAN_POINT ( 'NONE',  ( 0.4724409448818896462, 0.1265901696524990294, -2.721128608923884418 ) ) ;
#25985=CARTESIAN_POINT ( 'NONE',  ( 0.1974969037888704704, 0.3420746716998660508, -2.740813648293963567 ) ) ;
#25995=CARTESIAN_POINT ( 'NONE',  ( -0.1958661417322834220, -0.3392501089628018884, -1.317585301837270295 ) ) ;
#25999=CARTESIAN_POINT ( 'NONE',  ( 0.4091458600556404646, -0.2362204724409448231, 0.1332020997375328031 ) ) ;
#26011=CARTESIAN_POINT ( 'NONE',  ( 0.1998031496062994128, -0.3460692066303957537, -1.113517060367454015 ) ) ;
#26012=CARTESIAN_POINT ( 'NONE',  ( 0.3917322834645670104, 2.398668435337828261E-17, -2.564960629921259727 ) ) ;
#26021=CARTESIAN_POINT ( 'NONE',  ( -0.3996062992125986035, -7.340648628747425578E-17, 0.1181102362204724254 ) ) ;
#26022=CARTESIAN_POINT ( 'NONE',  ( 0.3917322834645670104, 0.1049643490035304660, -2.011174171424884083 ) ) ;
#26028=CARTESIAN_POINT ( 'NONE',  ( -0.2867679344610364334, -0.2867679344610367109, -2.190944881889763440 ) ) ;
#26036=CARTESIAN_POINT ( 'NONE',  ( -9.787531504996567848E-17, 0.3996062992125986035, -1.417322834645669216 ) ) ;
#26038=CARTESIAN_POINT ( 'NONE',  ( -0.2867679344610365444, -0.2867679344610367664, -0.05579359399706226158 ) ) ;
#26053=CARTESIAN_POINT ( 'NONE',  ( -0.3392501089628017219, -0.1958661417322836718, -0.04461942257217842850 ) ) ;
#26055=ORIENTED_EDGE ( 'NONE', *, *, #63009, .T. ) ;
#26056=CARTESIAN_POINT ( 'NONE',  ( 0.3949938075777411073, -0.1058382717557499464, -0.5839895013123359568 ) ) ;
#26064=CARTESIAN_POINT ( 'NONE',  ( -9.594673741351313045E-17, 0.3917322834645670659, -1.729021940453755013 ) ) ;
#26066=CARTESIAN_POINT ( 'NONE',  ( 0.3917322834645670104, 2.398668435337828261E-17, -2.879921259842519454 ) ) ;
#26070=CARTESIAN_POINT ( 'NONE',  ( 0.2925321140481932369, 0.2925321140481932369, -1.397637795275590067 ) ) ;
#26072=CARTESIAN_POINT ( 'NONE',  ( 0.2925321140481932369, -0.2925321140481931814, -0.6476377952755905110 ) ) ;
#26073=CARTESIAN_POINT ( 'NONE',  ( -0.2925321140481930149, -0.2925321140481933480, -0.2933070866141732069 ) ) ;
#26075=CARTESIAN_POINT ( 'NONE',  ( -0.3996062992125986035, -0.1070741851644056997, -2.880577427821522374 ) ) ;
#26076=CARTESIAN_POINT ( 'NONE',  ( 0.2867679344610365999, 0.2867679344610365999, -1.954724409448818978 ) ) ;
#26082=CARTESIAN_POINT ( 'NONE',  ( 0.2362204724409449064, 0.4091458600556404646, -1.638451443569553634 ) ) ;
#26085=CARTESIAN_POINT ( 'NONE',  ( -0.2891555358219911054, 0.2891555358219909388, -1.356299212598425230 ) ) ;
#26095=CARTESIAN_POINT ( 'NONE',  ( -0.1998031496062994405, 0.3460692066303957537, -2.294619422572178546 ) ) ;
#26097=CARTESIAN_POINT ( 'NONE',  ( 0.1958661417322836162, -0.3392501089628018329, -1.589219529362517758 ) ) ;
#26105=CARTESIAN_POINT ( 'NONE',  ( -1.157146581871515012E-16, 0.4724409448818898682, -2.362204724409448620 ) ) ;
#26109=CARTESIAN_POINT ( 'NONE',  ( -0.1070741851644056997, 0.3996062992125984925, 0.07414698162729659037 ) ) ;
#26111=CARTESIAN_POINT ( 'NONE',  ( 0.1958661417322836440, -0.3392501089628017219, -1.278871391076115582 ) ) ;
#26115=CARTESIAN_POINT ( 'NONE',  ( -0.4709442531824371558, -0.03757601356356778805, -1.220472440944882164 ) ) ;
#26121=CYLINDRICAL_SURFACE ( 'NONE', #82439, 0.4724409448818898682 ) ;
#26131=CARTESIAN_POINT ( 'NONE',  ( 0.3917322834645669549, 0.1049643490035304660, -2.321522309711285814 ) ) ;
#26134=CARTESIAN_POINT ( 'NONE',  ( 0.3458507752293908943, -0.3458507752293908943, -0.7283464566929134243 ) ) ;
#26136=CARTESIAN_POINT ( 'NONE',  ( 0.3996062992125986590, -0.1070741851644053111, 0.04593175853018371252 ) ) ;
#26137=ORIENTED_EDGE ( 'NONE', *, *, #52927, .T. ) ;
#26139=CARTESIAN_POINT ( 'NONE',  ( 0.3392501089628018329, 0.1958661417322835607, -1.855643044619422533 ) ) ;
#26143=CARTESIAN_POINT ( 'NONE',  ( 0.1265901696524990294, -0.4724409448818896462, -2.919947506561679784 ) ) ;
#26150=CARTESIAN_POINT ( 'NONE',  ( -0.3392501089628019439, 0.1958661417322832554, -1.051161786580365742 ) ) ;
#26157=CARTESIAN_POINT ( 'NONE',  ( 4.797336870675656522E-17, -0.3917322834645670659, -2.595163672737219596 ) ) ;
#26166=CARTESIAN_POINT ( 'NONE',  ( 0.3392501089628018884, -0.1958661417322834220, -1.606955380577427928 ) ) ;
#26182=CARTESIAN_POINT ( 'NONE',  ( -0.2362204724409447953, -0.4091458600556404646, -0.2998687664041995160 ) ) ;
#26186=CARTESIAN_POINT ( 'NONE',  ( 0.1058382717557500852, -0.3949938075777408852, -0.3195538057742782212 ) ) ;
#26191=CARTESIAN_POINT ( 'NONE',  ( 0.3949938075777409963, 2.418639510665530743E-17, -0.03740157480314962313 ) ) ;
#26198=CARTESIAN_POINT ( 'NONE',  ( 0.3460692066303958092, 0.1998031496062993018, -0.8379265091863516979 ) ) ;
#26200=CARTESIAN_POINT ( 'NONE',  ( 0.3917322834645670104, -0.1049643490035303411, -0.5761154855643042527 ) ) ;
#26216=CARTESIAN_POINT ( 'NONE',  ( 0.1265901696524989462, 0.4724409448818897572, -2.589895013123359568 ) ) ;
#26233=CARTESIAN_POINT ( 'NONE',  ( -0.1998031496062991907, -0.3460692066303959757, -0.3805774278215223183 ) ) ;
#26239=CARTESIAN_POINT ( 'NONE',  ( 0.3996062992125986035, 2.446882876249141962E-17, -2.795275590551181022 ) ) ;
#26241=CARTESIAN_POINT ( 'NONE',  ( -0.1058382717557497937, -0.3949938075777411628, -1.804461942257217899 ) ) ;
#26242=CARTESIAN_POINT ( 'NONE',  ( -0.1049643490035302024, -0.3917322834645671215, -0.3792650918635169233 ) ) ;
#26245=CARTESIAN_POINT ( 'NONE',  ( -0.1049643490035301885, -0.3917322834645671215, -1.166666666666666519 ) ) ;
#26247=CARTESIAN_POINT ( 'NONE',  ( 0.1958661417322834775, 0.3392501089628018884, -0.9238845144356954142 ) ) ;
#26249=CARTESIAN_POINT ( 'NONE',  ( -0.3420746716998660508, -0.1974969037888706924, -2.806430446194226214 ) ) ;
#26254=CARTESIAN_POINT ( 'NONE',  ( -0.4724409448818899238, 0.1265901696524986686, -2.867454068241469756 ) ) ;
#26255=CARTESIAN_POINT ( 'NONE',  ( 0.3460692066303959202, 0.1998031496062993295, -2.650918635170603554 ) ) ;
#26256=CARTESIAN_POINT ( 'NONE',  ( -0.3917322834645670104, -0.1049643490035307020, -1.145032439141419500 ) ) ;
#26262=CARTESIAN_POINT ( 'NONE',  ( -0.3917322834645671215, 0.1049643490035301469, -0.5898950131233595684 ) ) ;
#26270=CARTESIAN_POINT ( 'NONE',  ( 0.05722014594059725984, -0.3876764156947919981, -1.929133858267717549 ) ) ;
#26271=CARTESIAN_POINT ( 'NONE',  ( 0.1049643490035303689, 0.3917322834645670104, -1.875328083989501460 ) ) ;
#26272=CARTESIAN_POINT ( 'NONE',  ( 4.797336870675656522E-17, -0.3917322834645670104, -2.748031496062991685 ) ) ;
#26274=CARTESIAN_POINT ( 'NONE',  ( -9.787531504996567848E-17, 0.3996062992125986035, 0.1574803149606298913 ) ) ;
#26281=CARTESIAN_POINT ( 'NONE',  ( 0.1958661417322836440, -0.3392501089628017219, -0.8064304461942258806 ) ) ;
#26284=CARTESIAN_POINT ( 'NONE',  ( -0.3960428127060340864, -0.01218835185216879564, -1.929133858267718660 ) ) ;
#26302=CARTESIAN_POINT ( 'NONE',  ( 0.1958661417322836162, -0.3392501089628018329, -0.6443376395987383543 ) ) ;
#26304=EDGE_CURVE ( 'NONE', #52886, #49832, #37600, .T. ) ;
#26311=CARTESIAN_POINT ( 'NONE',  ( 0.3392501089628018884, -0.1958661417322833942, -0.1017253525272460019 ) ) ;
#26314=CARTESIAN_POINT ( 'NONE',  ( -0.4724409448818899238, 0.1265901696524986686, -1.054461942257217899 ) ) ;
#26327=CARTESIAN_POINT ( 'NONE',  ( 0.1998031496062992463, 0.3460692066303959202, -2.425853018372703396 ) ) ;
#26331=CARTESIAN_POINT ( 'NONE',  ( -0.3996062992125984925, -0.1070741851644056858, -1.854986876640420057 ) ) ;
#26338=CARTESIAN_POINT ( 'NONE',  ( -0.3996062992125986035, 0.1070741851644051584, -0.8969816272965878134 ) ) ;
#26339=CARTESIAN_POINT ( 'NONE',  ( 0.3996062992125986035, 2.446882876249141962E-17, -1.377952755905511806 ) ) ;
#26340=CARTESIAN_POINT ( 'NONE',  ( 0.3949938075777411073, -0.1058382717557499464, -0.5839895013123359568 ) ) ;
#26346=CARTESIAN_POINT ( 'NONE',  ( 0.3420746716998660508, -0.1974969037888704149, -1.914041994750656395 ) ) ;
#26351=CARTESIAN_POINT ( 'NONE',  ( 0.4724409448818896462, 0.1265901696524990294, -1.699475065616798064 ) ) ;
#26360=CARTESIAN_POINT ( 'NONE',  ( 0.3917322834645668994, -0.1049643490035303134, -1.923865198653856634 ) ) ;
#26369=CARTESIAN_POINT ( 'NONE',  ( -0.3392501089628019995, 0.1958661417322832277, -1.278215223097112885 ) ) ;
#26372=CARTESIAN_POINT ( 'NONE',  ( -0.3949938075777411628, 0.1058382717557497937, -1.765091863517060267 ) ) ;
#26373=ORIENTED_EDGE ( 'NONE', *, *, #34764, .F. ) ;
#26377=CARTESIAN_POINT ( 'NONE',  ( -0.3460692066303958092, -0.1998031496062994683, -0.3674540682414698112 ) ) ;
#26382=LENGTH_MEASURE_WITH_UNIT ( LENGTH_MEASURE( 0.02539999999999999897 ), #32277 );
#26386=CARTESIAN_POINT ( 'NONE',  ( 0.3917322834645670104, 2.398668435337828261E-17, -0.5177165354330709457 ) ) ;
#26393=CARTESIAN_POINT ( 'NONE',  ( -0.1998031496062994405, 0.3460692066303957537, -1.979658792650918597 ) ) ;
#26397=CARTESIAN_POINT ( 'NONE',  ( 0.4724409448818897572, -0.1265901696524988906, -0.7414698162729659314 ) ) ;
#26400=CARTESIAN_POINT ( 'NONE',  ( -0.1049643490035307020, 0.3917322834645669549, -0.3136482939632545541 ) ) ;
#26402=DIRECTION ( 'NONE',  ( 1.000000000000000000, 0.000000000000000000, 0.000000000000000000 ) ) ;
#26408=CARTESIAN_POINT ( 'NONE',  ( -0.2925321140481932369, 0.2925321140481931259, 0.2185039370078740162 ) ) ;
#26413=CARTESIAN_POINT ( 'NONE',  ( 0.3949938075777408852, 0.1058382717557500435, -2.563648293963254776 ) ) ;
#26415=CARTESIAN_POINT ( 'NONE',  ( 0.1958661417322836440, -0.3392501089628017219, -0.1765091863517061210 ) ) ;
#26420=CARTESIAN_POINT ( 'NONE',  ( -0.3392501089628019995, 0.1958661417322832277, -1.593175853018372612 ) ) ;
#26424=CARTESIAN_POINT ( 'NONE',  ( 0.4724409448818897572, -0.1265901696524988906, 0.1266404199475065218 ) ) ;
#26437=CARTESIAN_POINT ( 'NONE',  ( -0.3460692066303957537, -0.1998031496062994405, -1.074146981627296604 ) ) ;
#26438=CARTESIAN_POINT ( 'NONE',  ( 0.3917322834645669549, 0.1049643490035304660, -2.729002624671915900 ) ) ;
#26448=CARTESIAN_POINT ( 'NONE',  ( 0.3917322834645670659, 2.398668435337828261E-17, -2.477053436516747364 ) ) ;
#26456=CARTESIAN_POINT ( 'NONE',  ( 0.3917322834645670104, 2.398668435337828261E-17, -2.092519685039370358 ) ) ;
#26463=CARTESIAN_POINT ( 'NONE',  ( -0.3996062992125984925, -0.1070741851644056719, -2.642388451443570041 ) ) ;
#26465=CARTESIAN_POINT ( 'NONE',  ( -0.1998031496062994683, 0.3460692066303958092, -1.430446194225721834 ) ) ;
#26467=CARTESIAN_POINT ( 'NONE',  ( 0.1958661417322834775, 0.3392501089628018884, -0.1410954312674034816 ) ) ;
#26480=CARTESIAN_POINT ( 'NONE',  ( 4.797336870675656522E-17, -0.3917322834645670104, -0.3858267716535432879 ) ) ;
#26483=CARTESIAN_POINT ( 'NONE',  ( 0.1058382717557500713, -0.3949938075777409408, -0.5577427821522310536 ) ) ;
#26497=CARTESIAN_POINT ( 'NONE',  ( 0.1998031496062992740, 0.3460692066303959757, -1.404199475065616820 ) ) ;
#26499=CARTESIAN_POINT ( 'NONE',  ( -9.787531504996566615E-17, 0.3996062992125985480, -0.7066929133858268486 ) ) ;
#26500=CARTESIAN_POINT ( 'NONE',  ( 0.3996062992125986035, -0.1070741851644052972, -0.03083989501312338344 ) ) ;
#26502=CARTESIAN_POINT ( 'NONE',  ( -0.3460692066303958092, -0.1998031496062994683, -2.572178477690288734 ) ) ;
#26503=CARTESIAN_POINT ( 'NONE',  ( -0.3392501089628017219, -0.1958661417322836718, -2.026902887139107712 ) ) ;
#26509=CARTESIAN_POINT ( 'NONE',  ( 0.1265901696524989462, 0.4724409448818897572, -1.645013123359579943 ) ) ;
#26512=CARTESIAN_POINT ( 'NONE',  ( -9.674558042662122972E-17, 0.3949938075777409963, -1.336614173228346081 ) ) ;
#26518=CARTESIAN_POINT ( 'NONE',  ( 0.000000000000000000, 0.000000000000000000, -1.929133858267716661 ) ) ;
#26522=CARTESIAN_POINT ( 'NONE',  ( -0.3996062992125985480, -7.340648628747423112E-17, -2.163385826771653697 ) ) ;
#26525=CARTESIAN_POINT ( 'NONE',  ( 0.3917322834645668994, 0.1049643490035304522, -1.936988558233908808 ) ) ;
#26541=CARTESIAN_POINT ( 'NONE',  ( 0.1049643490035303689, 0.3917322834645670104, -1.337926509186352142 ) ) ;
#26550=CARTESIAN_POINT ( 'NONE',  ( -0.1265901696524986964, -0.4724409448818899238, -2.591863517060367439 ) ) ;
#26562=CARTESIAN_POINT ( 'NONE',  ( -9.594673741351313045E-17, 0.3917322834645670104, -2.669291338582676865 ) ) ;
#26565=CARTESIAN_POINT ( 'NONE',  ( 0.4091458600556404646, -0.2362204724409448231, -0.7349081364829396223 ) ) ;
#26566=CARTESIAN_POINT ( 'NONE',  ( -0.3460692066303960868, 0.1998031496062990242, -0.02624671916010500733 ) ) ;
#26570=CARTESIAN_POINT ( 'NONE',  ( -0.1958661417322834220, -0.3392501089628018884, -1.632545931758530244 ) ) ;
#26574=CARTESIAN_POINT ( 'NONE',  ( -0.02578378529929148399, 0.3963884504522700580, -2.755905511811024056 ) ) ;
#26581=CARTESIAN_POINT ( 'NONE',  ( -0.1049643490035306742, 0.3917322834645668994, -1.346437377131546764 ) ) ;
#26587=CARTESIAN_POINT ( 'NONE',  ( 0.3917322834645670104, 0.1049643490035304660, -2.483615116306773452 ) ) ;
#26596=CARTESIAN_POINT ( 'NONE',  ( -0.1958661417322836718, 0.3392501089628017219, -1.987532808398950079 ) ) ;
#26611=CARTESIAN_POINT ( 'NONE',  ( -0.3458507752293906723, -0.3458507752293910609, -0.1358267716535432879 ) ) ;
#26614=CARTESIAN_POINT ( 'NONE',  ( -0.3949938075777408852, -0.1058382717557502933, 0.03477690288713909672 ) ) ;
#26619=CARTESIAN_POINT ( 'NONE',  ( -0.1058382717557497660, -0.3949938075777411073, -0.1489501312335957950 ) ) ;
#26626=CARTESIAN_POINT ( 'NONE',  ( -0.1070741851644051862, -0.3996062992125986590, -1.093832020997375087 ) ) ;
#26628=CARTESIAN_POINT ( 'NONE',  ( 0.3392501089628018329, 0.1958661417322835607, -0.7532808398950130435 ) ) ;
#26641=CARTESIAN_POINT ( 'NONE',  ( -0.3957358693849766240, -0.01930322177395251207, -1.220472440945443493 ) ) ;
#26643=CARTESIAN_POINT ( 'NONE',  ( 0.1265901696524990294, -0.4724409448818896462, -2.681758530183727895 ) ) ;
#26660=CARTESIAN_POINT ( 'NONE',  ( -0.2925321140481932369, 0.2925321140481931814, -0.1771653543307086798 ) ) ;
#26664=CARTESIAN_POINT ( 'NONE',  ( 0.3996062992125986590, -0.1070741851644053111, -2.473753280839894764 ) ) ;
#26665=CARTESIAN_POINT ( 'NONE',  ( -0.2891555358219908833, -0.2891555358219912164, -2.106299212598425452 ) ) ;
#26666=CARTESIAN_POINT ( 'NONE',  ( -0.3392501089628019995, 0.1958661417322832277, -0.4908136482939632339 ) ) ;
#26668=CARTESIAN_POINT ( 'NONE',  ( 0.1049643490035304799, -0.3917322834645669549, -1.022309711286089051 ) ) ;
#26670=CARTESIAN_POINT ( 'NONE',  ( 0.3392501089628018884, -0.1958661417322834220, -0.8845144356955378928 ) ) ;
#26672=CARTESIAN_POINT ( 'NONE',  ( 0.2867679344610365999, -0.2867679344610365999, -0.02097805954624490030 ) ) ;
#26678=CARTESIAN_POINT ( 'NONE',  ( -0.3996062992125986035, -0.1070741851644056997, -2.565616797900262647 ) ) ;
#26679=CARTESIAN_POINT ( 'NONE',  ( 0.3917322834645670104, 0.1049643490035304660, -1.066292281661104457 ) ) ;
#26685=CARTESIAN_POINT ( 'NONE',  ( 0.1958661417322834775, 0.3392501089628018884, -0.5439632545931759600 ) ) ;
#26694=CARTESIAN_POINT ( 'NONE',  ( -0.3917322834645671215, 0.1049643490035301469, -2.072178477690288734 ) ) ;
#26696=CARTESIAN_POINT ( 'NONE',  ( -0.1070741851644056997, 0.3996062992125986035, -0.1640419947506562004 ) ) ;
#26703=CARTESIAN_POINT ( 'NONE',  ( 0.1049643490035303689, 0.3917322834645670104, -0.7080052493438320216 ) ) ;
#26716=DIRECTION ( 'NONE',  ( 0.000000000000000000, 0.000000000000000000, 1.000000000000000000 ) ) ;
#26723=CARTESIAN_POINT ( 'NONE',  ( -0.1958661417322834497, -0.3392501089628018884, -0.7755712353992633146 ) ) ;
#26726=CARTESIAN_POINT ( 'NONE',  ( 0.3458507752293908943, 0.3458507752293908943, -0.7677165354330708347 ) ) ;
#26732=CARTESIAN_POINT ( 'NONE',  ( -0.1958661417322836995, 0.3392501089628017219, -0.1673421504275084681 ) ) ;
#26735=CARTESIAN_POINT ( 'NONE',  ( -1.157146581871515012E-16, 0.4724409448818898682, -1.336614173228346303 ) ) ;
#26749=CARTESIAN_POINT ( 'NONE',  ( -0.3460692066303957537, -0.1998031496062994405, -2.491469816272966042 ) ) ;
#26753=CARTESIAN_POINT ( 'NONE',  ( 0.3996062992125984925, 0.1070741851644054637, -1.618766404199474929 ) ) ;
#26759=CARTESIAN_POINT ( 'NONE',  ( -0.1998031496062994405, 0.3460692066303957537, -1.034776902887139194 ) ) ;
#26760=CARTESIAN_POINT ( 'NONE',  ( 4.893765752498283924E-17, -0.3996062992125986035, -1.338582677165354173 ) ) ;
#26761=CARTESIAN_POINT ( 'NONE',  ( 0.3949938075777409963, 2.418639510665530435E-17, -0.5905511811023622659 ) ) ;
#26767=CARTESIAN_POINT ( 'NONE',  ( 0.2891555358219910499, -0.2891555358219909944, -1.907480314960629419 ) ) ;
#26772=CARTESIAN_POINT ( 'NONE',  ( 0.4724409448818896462, 0.1265901696524990294, -1.856955380577427928 ) ) ;
#26773=CARTESIAN_POINT ( 'NONE',  ( 0.3272402980636514580, -0.2155943732411718938, -2.755905511811024944 ) ) ;
#26779=CARTESIAN_POINT ( 'NONE',  ( -0.3392501089628019439, 0.1958661417322832554, -2.468484621226035181 ) ) ;
#26785=CARTESIAN_POINT ( 'NONE',  ( -0.3917322834645668994, -0.1049643490035306742, -2.645649975556744415 ) ) ;
#26787=CARTESIAN_POINT ( 'NONE',  ( -0.3917322834645671215, 0.1049643490035301469, -2.072178477690288734 ) ) ;
#26790=CARTESIAN_POINT ( 'NONE',  ( -0.3949938075777409408, -0.1058382717557502933, -1.935695538057742748 ) ) ;
#26795=CARTESIAN_POINT ( 'NONE',  ( 0.3996062992125986035, 2.446882876249141962E-17, -0.4330708661417322913 ) ) ;
#26804=CARTESIAN_POINT ( 'NONE',  ( -0.3392501089628019995, 0.1958661417322832277, -0.4258530183727035068 ) ) ;
#26811=CARTESIAN_POINT ( 'NONE',  ( 0.1998031496062994128, -0.3460692066303957537, -1.900918635170603554 ) ) ;
#26814=FACE_OUTER_BOUND ( 'NONE', #82794, .T. ) ;
#26816=CARTESIAN_POINT ( 'NONE',  ( 0.1265901696524989462, 0.4724409448818897572, -1.410761154855643129 ) ) ;
#26818=CARTESIAN_POINT ( 'NONE',  ( -9.594673741351313045E-17, 0.3917322834645670104, -0.1496062992125983815 ) ) ;
#26819=CARTESIAN_POINT ( 'NONE',  ( -0.3392501089628019995, 0.1958661417322832277, -2.630577427821522374 ) ) ;
#26823=CARTESIAN_POINT ( 'NONE',  ( 4.893765752498283308E-17, -0.3996062992125985480, -0.1555118110236220763 ) ) ;
#26828=CARTESIAN_POINT ( 'NONE',  ( -0.1058382717557497660, -0.3949938075777411073, -2.826115485564304475 ) ) ;
#26830=CARTESIAN_POINT ( 'NONE',  ( 0.3917322834645669549, 0.1049643490035304660, -0.2093175853018373889 ) ) ;
#26835=CARTESIAN_POINT ( 'NONE',  ( -0.3917322834645669549, -0.1049643490035306603, -1.927821522309711044 ) ) ;
#26838=CARTESIAN_POINT ( 'NONE',  ( -0.1265901696524993347, 0.4724409448818895907, 0.07414698162729659037 ) ) ;
#26851=CARTESIAN_POINT ( 'NONE',  ( 0.1070741851644054776, -0.3996062992125984925, -1.264435695538057569 ) ) ;
#26852=CARTESIAN_POINT ( 'NONE',  ( 0.1049643490035304938, -0.3917322834645669549, -2.847112860892388131 ) ) ;
#26861=CARTESIAN_POINT ( 'NONE',  ( -0.3460692066303960868, 0.1998031496062990242, -0.1837270341207349056 ) ) ;
#26862=CARTESIAN_POINT ( 'NONE',  ( 0.1958661417322834775, 0.3392501089628018884, -2.503300155676852157 ) ) ;
#26868=CARTESIAN_POINT ( 'NONE',  ( 4.797336870675656522E-17, -0.3917322834645670104, -2.368110236220472675 ) ) ;
#26876=CARTESIAN_POINT ( 'NONE',  ( -0.2925321140481930704, -0.2925321140481933480, -1.476377952755905554 ) ) ;
#26878=CARTESIAN_POINT ( 'NONE',  ( -9.594673741351313045E-17, 0.3917322834645670659, -0.1542187908474559610 ) ) ;
#26890=CARTESIAN_POINT ( 'NONE',  ( 0.1049643490035303689, 0.3917322834645670104, -0.6154855643044617741 ) ) ;
#26893=CARTESIAN_POINT ( 'NONE',  ( 0.1058382717557499880, 0.3949938075777411073, -0.7808398950131234528 ) ) ;
#26894=ORIENTED_EDGE ( 'NONE', *, *, #38729, .F. ) ;
#26908=CARTESIAN_POINT ( 'NONE',  ( -0.2925321140481932924, 0.2925321140481931814, -1.279527559055118058 ) ) ;
#26910=CARTESIAN_POINT ( 'NONE',  ( 0.2925321140481932369, -0.2925321140481931814, -0.8051181102362205966 ) ) ;
#26911=CARTESIAN_POINT ( 'NONE',  ( -0.3460692066303957537, -0.1998031496062994405, -0.1292650918635170898 ) ) ;
#26913=CARTESIAN_POINT ( 'NONE',  ( -9.787531504996567848E-17, 0.3996062992125986035, -2.834645669291338432 ) ) ;
#26914=CARTESIAN_POINT ( 'NONE',  ( 0.2867679344610365999, -0.2867679344610365444, -2.072834645669291209 ) ) ;
#26920=CARTESIAN_POINT ( 'NONE',  ( -0.1265901696524986964, -0.4724409448818899238, -2.038713910761154491 ) ) ;
#26923=CARTESIAN_POINT ( 'NONE',  ( -0.3949938075777411073, 0.1058382717557497660, -1.369422572178477848 ) ) ;
#26934=CARTESIAN_POINT ( 'NONE',  ( 4.893765752498283308E-17, -0.3996062992125985480, -2.360236220472441193 ) ) ;
#26935=CARTESIAN_POINT ( 'NONE',  ( -0.1958661417322834497, -0.3392501089628018884, -2.192894070044932420 ) ) ;
#26948=CARTESIAN_POINT ( 'NONE',  ( 0.1998031496062992463, 0.3460692066303959202, -0.06364829396325459576 ) ) ;
#26950=CARTESIAN_POINT ( 'NONE',  ( -0.1958661417322834220, -0.3392501089628018884, -1.252624671916010568 ) ) ;
#26971=CARTESIAN_POINT ( 'NONE',  ( -0.2867679344610366554, 0.2867679344610365444, -2.531496062992125484 ) ) ;
#26974=CARTESIAN_POINT ( 'NONE',  ( 0.4091458600556403535, 0.2362204724409449896, -0.7611548556430446366 ) ) ;
#26975=CARTESIAN_POINT ( 'NONE',  ( -0.1998031496062991907, -0.3460692066303959757, -0.2230971128608923992 ) ) ;
#26978=CARTESIAN_POINT ( 'NONE',  ( -0.3392501089628019995, 0.1958661417322832277, -1.750656167979002698 ) ) ;
#26990=CARTESIAN_POINT ( 'NONE',  ( -0.1049643490035301746, -0.3917322834645670659, -1.254573860071179103 ) ) ;
#26996=CARTESIAN_POINT ( 'NONE',  ( 0.1958661417322834775, 0.3392501089628018884, -2.660780470637482242 ) ) ;
#27005=CARTESIAN_POINT ( 'NONE',  ( -9.594673741351313045E-17, 0.3917322834645670104, -1.816929133858267820 ) ) ;
#27008=ADVANCED_FACE ( 'NONE', ( #1662 ), #27319, .T. ) ;
#27020=CARTESIAN_POINT ( 'NONE',  ( -0.4724409448818899238, 0.1265901696524986686, -0.2670603674540683037 ) ) ;
#27023=CARTESIAN_POINT ( 'NONE',  ( 0.3949938075777409963, 2.418639510665530743E-17, -0.1948818897637795700 ) ) ;
#27028=CARTESIAN_POINT ( 'NONE',  ( 0.1058382717557499880, 0.3949938075777409408, -0.2276902887139107823 ) ) ;
#27036=CARTESIAN_POINT ( 'NONE',  ( -9.787531504996566615E-17, 0.3996062992125985480, -1.021653543307086576 ) ) ;
#27038=CARTESIAN_POINT ( 'NONE',  ( 0.3917322834645669549, 0.1049643490035304660, -0.5892388451443569819 ) ) ;
#27049=( GEOMETRIC_REPRESENTATION_CONTEXT ( 3 ) GLOBAL_UNCERTAINTY_ASSIGNED_CONTEXT ( ( #22601 ) ) GLOBAL_UNIT_ASSIGNED_CONTEXT ( ( #12933, #45728, #25957 ) ) REPRESENTATION_CONTEXT ( 'NONE', 'WORKASPACE' ) );
#27055=CARTESIAN_POINT ( 'NONE',  ( 5.785732909357575061E-17, -0.4724409448818898682, -2.675196850393700920 ) ) ;
#27072=CARTESIAN_POINT ( 'NONE',  ( -0.1998031496062994683, 0.3460692066303958092, -0.9580052493438320216 ) ) ;
#27073=CARTESIAN_POINT ( 'NONE',  ( -0.3458507752293909498, 0.3458507752293908388, -1.198818897637795367 ) ) ;
#27077=CARTESIAN_POINT ( 'NONE',  ( -0.2925321140481930704, -0.2925321140481933480, -2.736220472440944018 ) ) ;
#27078=CARTESIAN_POINT ( 'NONE',  ( 0.1974969037888704704, 0.3420746716998660508, -1.876640419947506633 ) ) ;
#27079=CARTESIAN_POINT ( 'NONE',  ( 0.2867679344610365999, -0.2867679344610365444, -0.4055118110236220486 ) ) ;
#27080=CARTESIAN_POINT ( 'NONE',  ( 0.3726288332213487653, 0.1208384647389236927, -1.220472440944882164 ) ) ;
#27082=CARTESIAN_POINT ( 'NONE',  ( 0.3917322834645670104, 2.398668435337828261E-17, -1.212598425196850238 ) ) ;
#27084=CARTESIAN_POINT ( 'NONE',  ( 0.1958661417322836162, -0.3392501089628018329, 0.1430639352044112689 ) ) ;
#27090=CARTESIAN_POINT ( 'NONE',  ( -0.3996062992125986035, -7.340648628747425578E-17, -2.401574803149606474 ) ) ;
#27091=CARTESIAN_POINT ( 'NONE',  ( 0.3917322834645670104, 0.1049643490035304660, -1.223772596621734321 ) ) ;
#27098=CARTESIAN_POINT ( 'NONE',  ( 0.3917322834645670104, 2.398668435337828261E-17, -0.6751968503937009203 ) ) ;
#27106=CARTESIAN_POINT ( 'NONE',  ( 0.3458507752293908943, 0.3458507752293908943, -0.5295275590551181688 ) ) ;
#27107=CARTESIAN_POINT ( 'NONE',  ( 4.797336870675656522E-17, -0.3917322834645670104, -1.803149606299212726 ) ) ;
#27109=CARTESIAN_POINT ( 'NONE',  ( 0.3460692066303959757, -0.1998031496062991907, -0.2624671916010499206 ) ) ;
#27115=CARTESIAN_POINT ( 'NONE',  ( -0.4724409448818898682, -8.678599364036362592E-17, -1.141732283464566899 ) ) ;
#27116=CARTESIAN_POINT ( 'NONE',  ( 0.2867679344610365999, -0.2867679344610365444, -0.9704724409448820532 ) ) ;
#27118=CARTESIAN_POINT ( 'NONE',  ( -0.3841287887292183512, -0.08106202739158083204, -1.929133858267717105 ) ) ;
#27131=CARTESIAN_POINT ( 'NONE',  ( 0.4724409448818915891, -0.1265901696524958653, -2.550524934383202158 ) ) ;
#27135=CARTESIAN_POINT ( 'NONE',  ( 0.1049643490035303689, 0.3917322834645668994, -0.7033927577089746919 ) ) ;
#27144=CARTESIAN_POINT ( 'NONE',  ( 0.3917322834645670659, -0.1049643490035303273, -0.1082870323172722415 ) ) ;
#27146=CARTESIAN_POINT ( 'NONE',  ( -0.4724409448818896462, -0.1265901696524993070, -0.2034120734908136108 ) ) ;
#27147=CARTESIAN_POINT ( 'NONE',  ( -0.4724409448818898682, -8.678599364036362592E-17, -1.533464566929133799 ) ) ;
#27164=CARTESIAN_POINT ( 'NONE',  ( 4.893765752498283308E-17, -0.3996062992125985480, -2.675196850393700920 ) ) ;
#27169=CARTESIAN_POINT ( 'NONE',  ( -0.3996062992125985480, -7.340648628747423112E-17, -1.690944881889763884 ) ) ;
#27175=CARTESIAN_POINT ( 'NONE',  ( -0.2925321140481930704, -0.2925321140481933480, -1.476377952755905554 ) ) ;
#27176=CARTESIAN_POINT ( 'NONE',  ( 0.1058382717557500713, -0.3949938075777409408, -0.7152230971128611392 ) ) ;
#27181=CARTESIAN_POINT ( 'NONE',  ( -0.1974969037888704149, -0.3420746716998661063, -1.717191601049868677 ) ) ;
#27186=CARTESIAN_POINT ( 'NONE',  ( 0.4091458600556403535, 0.2362204724409449896, -2.178477690288713742 ) ) ;
#27194=CARTESIAN_POINT ( 'NONE',  ( 0.3917322834645668994, -0.1049643490035303134, -2.238825828575116805 ) ) ;
#27195=CARTESIAN_POINT ( 'NONE',  ( -0.1070741851644056997, 0.3996062992125984925, -2.760498687664041384 ) ) ;
#27200=CARTESIAN_POINT ( 'NONE',  ( -0.3917322834645668994, -0.1049643490035306742, -2.803130290517373613 ) ) ;
#27203=CARTESIAN_POINT ( 'NONE',  ( 0.2867679344610365999, 0.2867679344610365999, -2.019685039370078261 ) ) ;
#27206=CARTESIAN_POINT ( 'NONE',  ( -0.2891555358219911054, 0.2891555358219909388, -2.224409448818897683 ) ) ;
#27211=CARTESIAN_POINT ( 'NONE',  ( -0.2925321140481930704, -0.2925321140481933480, -0.5314960629921260393 ) ) ;
#27215=SURFACE_STYLE_FILL_AREA ( #32694 ) ;
#27220=CARTESIAN_POINT ( 'NONE',  ( 0.1958661417322834775, 0.3392501089628018884, -0.3864829396325459854 ) ) ;
#27232=CARTESIAN_POINT ( 'NONE',  ( 0.4724409448818898682, 2.892866454678787531E-17, -1.220472440944881942 ) ) ;
#27234=CARTESIAN_POINT ( 'NONE',  ( -0.1958661417322836718, 0.3392501089628017219, -0.3202099737532808077 ) ) ;
#27235=CARTESIAN_POINT ( 'NONE',  ( 0.1049643490035304799, -0.3917322834645669549, -2.374671916010498762 ) ) ;
#27238=CARTESIAN_POINT ( 'NONE',  ( 0.3996062992125984925, 0.1070741851644054637, -0.04396325459317587669 ) ) ;
#27243=CARTESIAN_POINT ( 'NONE',  ( 0.1974969037888706092, -0.3420746716998660508, -2.845800524934383624 ) ) ;
#27245=CARTESIAN_POINT ( 'NONE',  ( 0.3917322834645670104, -0.1049643490035303273, -0.03871391076115493490 ) ) ;
#27250=CARTESIAN_POINT ( 'NONE',  ( -0.3917322834645670104, -7.196005306013484475E-17, -1.763779527559055094 ) ) ;
#27253=CARTESIAN_POINT ( 'NONE',  ( -0.3458507752293909498, 0.3458507752293907833, -0.2539370078740156855 ) ) ;
#27257=CARTESIAN_POINT ( 'NONE',  ( -0.4724409448818898682, -8.678599364036362592E-17, -0.7460629921259841479 ) ) ;
#27261=CARTESIAN_POINT ( 'NONE',  ( 0.000000000000000000, 0.000000000000000000, -2.755905511811024056 ) ) ;
#27266=CARTESIAN_POINT ( 'NONE',  ( -0.3996062992125985480, -7.340648628747423112E-17, -1.218503937007874072 ) ) ;
#27267=CARTESIAN_POINT ( 'NONE',  ( -0.2867679344610365999, 0.2867679344610364889, -2.624015748031495399 ) ) ;
#27276=CARTESIAN_POINT ( 'NONE',  ( 0.3996062992125986590, -0.1070741851644053111, -0.2690288713910760632 ) ) ;
#27278=CARTESIAN_POINT ( 'NONE',  ( -0.3392501089628019995, 0.1958661417322831999, -2.385189919456379926 ) ) ;
#27283=CARTESIAN_POINT ( 'NONE',  ( -9.594673741351313045E-17, 0.3917322834645670104, -2.446850393700787496 ) ) ;
#27290=CARTESIAN_POINT ( 'NONE',  ( 0.3996062992125986035, -0.1070741851644053111, -2.001312335958005395 ) ) ;
#27292=CARTESIAN_POINT ( 'NONE',  ( -0.2925321140481930704, -0.2925321140481933480, -1.791338582677165059 ) ) ;
#27294=CARTESIAN_POINT ( 'NONE',  ( -0.2867679344610367109, 0.2867679344610365444, -0.1739038302175346939 ) ) ;
#27306=CARTESIAN_POINT ( 'NONE',  ( 0.2867679344610365999, 0.2867679344610365999, -0.7598425196850391306 ) ) ;
#27309=CARTESIAN_POINT ( 'NONE',  ( 0.2891555358219910499, 0.2891555358219910499, -0.4527559055118110520 ) ) ;
#27319=CYLINDRICAL_SURFACE ( 'NONE', #37176, 0.4724409448818898682 ) ;
#27324=CARTESIAN_POINT ( 'NONE',  ( 0.1998031496062992740, 0.3460692066303959757, -1.089238845144356871 ) ) ;
#27326=CARTESIAN_POINT ( 'NONE',  ( -0.2925321140481932369, 0.2925321140481931259, -0.5688976377952755792 ) ) ;
#27327=CARTESIAN_POINT ( 'NONE',  ( -0.2925321140481932369, 0.2925321140481931259, -0.5688976377952755792 ) ) ;
#27329=CARTESIAN_POINT ( 'NONE',  ( -0.4724409448818895907, -0.1265901696524993070, -0.2034120734908136108 ) ) ;
#27330=CARTESIAN_POINT ( 'NONE',  ( 0.3917322834645670104, -0.1049643490035303411, -2.085958005249344271 ) ) ;
#27336=CARTESIAN_POINT ( 'NONE',  ( 0.3458507752293908943, 0.3458507752293908943, -1.789370078740157410 ) ) ;
#27341=CARTESIAN_POINT ( 'NONE',  ( 0.1974969037888704704, 0.3420746716998660508, -1.323490813648294129 ) ) ;
#27351=CARTESIAN_POINT ( 'NONE',  ( 0.3996062992125985480, 2.446882876249141654E-17, -2.714566929133858331 ) ) ;
#27352=CARTESIAN_POINT ( 'NONE',  ( 0.3392501089628018329, -0.1958661417322834497, -1.917303518863830103 ) ) ;
#27363=CARTESIAN_POINT ( 'NONE',  ( 0.2925321140481932369, 0.2925321140481932369, 0.1003937007874015769 ) ) ;
#27365=CARTESIAN_POINT ( 'NONE',  ( -0.3392501089628019995, 0.1958661417322832277, -1.370734908136483021 ) ) ;
#27374=CARTESIAN_POINT ( 'NONE',  ( -0.3996062992125986590, 0.1070741851644051723, -0.8969816272965877024 ) ) ;
#27388=CARTESIAN_POINT ( 'NONE',  ( 0.2867679344610366554, 0.2867679344610366554, -2.492125984251968518 ) ) ;
#27391=CARTESIAN_POINT ( 'NONE',  ( 0.1998031496062994405, -0.3460692066303958092, -0.2493438320209974135 ) ) ;
#27392=ORIENTED_EDGE ( 'NONE', *, *, #52169, .T. ) ;
#27395=CARTESIAN_POINT ( 'NONE',  ( -9.594673741351313045E-17, 0.3917322834645670104, -1.881889763779527769 ) ) ;
#27402=CARTESIAN_POINT ( 'NONE',  ( 0.4724409448818898682, 2.892866454678787531E-17, -2.084645669291338432 ) ) ;
#27406=CARTESIAN_POINT ( 'NONE',  ( -9.594673741351310580E-17, 0.3917322834645669549, -1.339875697341520455 ) ) ;
#27412=CARTESIAN_POINT ( 'NONE',  ( 0.3917322834645670659, 2.398668435337828261E-17, -2.634533751477377450 ) ) ;
#27420=CARTESIAN_POINT ( 'NONE',  ( -0.3392501089628019995, 0.1958661417322832277, -2.000656167979002920 ) ) ;
#27425=EDGE_CURVE ( 'NONE', #59512, #2851, #46203, .T. ) ;
#27429=CARTESIAN_POINT ( 'NONE',  ( 0.3460692066303959757, -0.1998031496062991907, -1.994750656167979086 ) ) ;
#27435=CARTESIAN_POINT ( 'NONE',  ( -0.3458507752293906723, -0.3458507752293910609, -0.7657480314960628531 ) ) ;
#27439=CARTESIAN_POINT ( 'NONE',  ( 0.2891555358219910499, 0.2891555358219910499, -0.05708661417322836301 ) ) ;
#27445=CARTESIAN_POINT ( 'NONE',  ( -0.3420746716998662729, 0.1974969037888702206, -0.5754593175853018883 ) ) ;
#27452=CARTESIAN_POINT ( 'NONE',  ( -0.2925321140481930149, -0.2925321140481933480, -1.080708661417322691 ) ) ;
#27455=CARTESIAN_POINT ( 'NONE',  ( -0.1958661417322836718, 0.3392501089628017219, -0.7926509186351704539 ) ) ;
#27471=CARTESIAN_POINT ( 'NONE',  ( 0.2925321140481932369, 0.2925321140481932369, 0.1003937007874015491 ) ) ;
#27487=CARTESIAN_POINT ( 'NONE',  ( 0.3996062992125986035, -0.1070741851644053111, -0.7414698162729659314 ) ) ;
#27493=CARTESIAN_POINT ( 'NONE',  ( 0.1070741851644054915, -0.3996062992125986035, -2.447506561679789527 ) ) ;
#27494=CARTESIAN_POINT ( 'NONE',  ( 0.3949938075777411073, -0.1058382717557499464, -1.843832020997375309 ) ) ;
#27495=CARTESIAN_POINT ( 'NONE',  ( 0.3392501089628018884, -0.1958661417322834220, -0.4120734908136482466 ) ) ;
#27499=CARTESIAN_POINT ( 'NONE',  ( -0.3917322834645671215, 0.1049643490035301469, -1.127296587926509108 ) ) ;
#27501=CARTESIAN_POINT ( 'NONE',  ( 0.3917322834645668994, 0.1049643490035304522, -0.04722477870634988334 ) ) ;
#27502=EDGE_CURVE ( 'NONE', #59098, #47997, #54811, .T. ) ;
#27508=CARTESIAN_POINT ( 'NONE',  ( -0.2925321140481930704, -0.2925321140481933480, -2.421259842519684735 ) ) ;
#27509=CARTESIAN_POINT ( 'NONE',  ( 0.3392501089628018329, 0.1958661417322835607, -1.072853961451130544 ) ) ;
#27515=CARTESIAN_POINT ( 'NONE',  ( -0.2867679344610365999, 0.2867679344610364889, -0.4192913385826772532 ) ) ;
#27523=CARTESIAN_POINT ( 'NONE',  ( -0.2417350488504524941, -0.3089825338629034746, -1.929133858267717772 ) ) ;
#27524=CARTESIAN_POINT ( 'NONE',  ( -0.2867679344610364334, -0.2867679344610367109, -1.783464566929133577 ) ) ;
#27526=ORIENTED_EDGE ( 'NONE', *, *, #46673, .F. ) ;
#27527=CARTESIAN_POINT ( 'NONE',  ( 0.3996062992125986035, 0.1070741851644054776, -0.2821522309711286258 ) ) ;
#27532=CARTESIAN_POINT ( 'NONE',  ( 0.2362204724409451007, -0.4091458600556402980, -0.01115485564304462100 ) ) ;
#27534=CARTESIAN_POINT ( 'NONE',  ( -0.1049643490035307020, 0.3917322834645669549, -1.193569553805774452 ) ) ;
#27554=CARTESIAN_POINT ( 'NONE',  ( -0.2867679344610366554, 0.2867679344610365444, -1.202080421750969741 ) ) ;
#27557=CARTESIAN_POINT ( 'NONE',  ( 0.2362204724409449064, 0.4091458600556404646, -0.7742782152230971437 ) ) ;
#27564=CARTESIAN_POINT ( 'NONE',  ( 0.3392501089628018329, 0.1958661417322835607, -0.1279720716873509745 ) ) ;
#27567=CARTESIAN_POINT ( 'NONE',  ( -0.2362204724409451284, 0.4091458600556402425, -1.822178477690288512 ) ) ;
#27585=CARTESIAN_POINT ( 'NONE',  ( -0.3949938075777408852, -0.1058382717557502933, 0.1922572178477690297 ) ) ;
#27590=CARTESIAN_POINT ( 'NONE',  ( -0.3996062992125985480, -7.340648628747423112E-17, -2.005905511811023612 ) ) ;
#27596=CARTESIAN_POINT ( 'NONE',  ( -9.787531504996566615E-17, 0.3996062992125985480, -1.021653543307086576 ) ) ;
#27597=CARTESIAN_POINT ( 'NONE',  ( 0.3996062992125986035, 0.1070741851644054776, -1.541994750656167978 ) ) ;
#27598=CARTESIAN_POINT ( 'NONE',  ( -0.1974969037888706647, 0.3420746716998658843, -0.8005249343832020470 ) ) ;
#27603=CARTESIAN_POINT ( 'NONE',  ( 0.2891555358219910499, -0.2891555358219909944, -1.592519685039370581 ) ) ;
#27607=CARTESIAN_POINT ( 'NONE',  ( -0.4091458600556402980, -0.2362204724409451284, -1.942257217847769057 ) ) ;
#27608=CARTESIAN_POINT ( 'NONE',  ( 0.3876764156950328055, 0.05722014593897428725, -2.755905511811027164 ) ) ;
#27614=CARTESIAN_POINT ( 'NONE',  ( -0.1958661417322836440, 0.3392501089628016664, -2.297880946685352033 ) ) ;
#27620=CARTESIAN_POINT ( 'NONE',  ( -0.3917322834645669549, -0.1049643490035306603, 0.1843832020997374643 ) ) ;
#27622=CARTESIAN_POINT ( 'NONE',  ( -0.2867679344610365999, 0.2867679344610364889, -2.059055118110236116 ) ) ;
#27625=CARTESIAN_POINT ( 'NONE',  ( -0.3420746716998659953, -0.1974969037888706647, -2.414698162729658648 ) ) ;
#27631=CARTESIAN_POINT ( 'NONE',  ( 0.2925321140481932369, -0.2925321140481932369, -0.4133858267716534196 ) ) ;
#27636=CARTESIAN_POINT ( 'NONE',  ( 0.3917322834645670104, -0.1049643490035303411, -0.1961942257217848817 ) ) ;
#27638=CARTESIAN_POINT ( 'NONE',  ( -0.3392501089628019995, 0.1958661417322832277, -0.5833333333333334814 ) ) ;
#27649=CARTESIAN_POINT ( 'NONE',  ( 0.4724409448818896462, 0.1265901696524990294, -1.384514435695537671 ) ) ;
#27651=CARTESIAN_POINT ( 'NONE',  ( -0.3917322834645669549, -0.1049643490035306603, -0.5104986876640419391 ) ) ;
#27652=CARTESIAN_POINT ( 'NONE',  ( 0.3392501089628018329, 0.1958661417322835607, -2.578083989501311901 ) ) ;
#27655=CARTESIAN_POINT ( 'NONE',  ( -0.3996062992125985480, -7.340648628747423112E-17, -0.1161417322834645965 ) ) ;
#27660=CARTESIAN_POINT ( 'NONE',  ( 0.3917322834645669549, 2.398668435337827645E-17, -0.04066309891632365059 ) ) ;
#27662=CARTESIAN_POINT ( 'NONE',  ( -0.3392501089628019995, 0.1958661417322832277, -0.1108923884514436548 ) ) ;
#27667=CARTESIAN_POINT ( 'NONE',  ( -9.594673741351313045E-17, 0.3917322834645670104, -2.039370078740157410 ) ) ;
#27671=CARTESIAN_POINT ( 'NONE',  ( -0.3458507752293909498, 0.3458507752293907833, -0.4114173228346455491 ) ) ;
#27677=CARTESIAN_POINT ( 'NONE',  ( -1.157146581871515012E-16, 0.4724409448818898682, -0.7066929133858268486 ) ) ;
#27686=CARTESIAN_POINT ( 'NONE',  ( -0.3996062992125984925, -0.1070741851644056858, -1.540026246719159886 ) ) ;
#27687=CARTESIAN_POINT ( 'NONE',  ( 0.1958661417322836440, -0.3392501089628017219, -2.853674540682414662 ) ) ;
#27697=CARTESIAN_POINT ( 'NONE',  ( -9.787531504996567848E-17, 0.3996062992125986035, -8.919671568592925241E-18 ) ) ;
#27698=CARTESIAN_POINT ( 'NONE',  ( -0.2867679344610365444, -0.2867679344610367664, -2.575478633367141779 ) ) ;
#27703=CARTESIAN_POINT ( 'NONE',  ( -0.3392501089628017219, -0.1958661417322836718, -2.499343832020997080 ) ) ;
#27711=CARTESIAN_POINT ( 'NONE',  ( 0.2867679344610366554, -0.2867679344610365999, -0.2526439876978496257 ) ) ;
#27724=CARTESIAN_POINT ( 'NONE',  ( -0.1049643490035307020, 0.3917322834645669549, -0.7860892388451442558 ) ) ;
#27727=CARTESIAN_POINT ( 'NONE',  ( -0.2891555358219908833, -0.2891555358219912164, -1.003937007874015741 ) ) ;
#27745=CARTESIAN_POINT ( 'NONE',  ( 0.3460692066303959202, 0.1998031496062993295, -1.863517060367454015 ) ) ;
#27747=CARTESIAN_POINT ( 'NONE',  ( 0.1070741851644053388, 0.3996062992125986035, -1.015091863517060267 ) ) ;
#27748=CARTESIAN_POINT ( 'NONE',  ( 0.3996062992125986035, -0.1070741851644052972, -0.3458005249343831244 ) ) ;
#27750=CARTESIAN_POINT ( 'NONE',  ( 0.1265901696524990294, -0.4724409448818896462, -0.08530183727034119923 ) ) ;
#27751=CARTESIAN_POINT ( 'NONE',  ( 0.3917322834645669549, 0.1049643490035304660, -2.256561679790026531 ) ) ;
#27757=CARTESIAN_POINT ( 'NONE',  ( 0.1265901696524989462, 0.4724409448818897572, -1.802493438320209584 ) ) ;
#27760=CARTESIAN_POINT ( 'NONE',  ( -0.3420746716998660508, -0.1974969037888706924, -1.231627296587926468 ) ) ;
#27766=CARTESIAN_POINT ( 'NONE',  ( -1.157146581871515012E-16, 0.4724409448818898682, -2.281496062992125928 ) ) ;
#27770=CARTESIAN_POINT ( 'NONE',  ( -0.2925321140481932369, 0.2925321140481931259, -2.616141732283464805 ) ) ;
#27772=CARTESIAN_POINT ( 'NONE',  ( 0.1049643490035304522, -0.3917322834645668994, -1.897618479493751398 ) ) ;
#27785=CARTESIAN_POINT ( 'NONE',  ( 4.893765752498283308E-17, -0.3996062992125985480, -0.4704724409448819422 ) ) ;
#27788=CARTESIAN_POINT ( 'NONE',  ( 0.3917322834645670104, 2.398668435337828261E-17, -1.620078740157480324 ) ) ;
#27799=CARTESIAN_POINT ( 'NONE',  ( 0.1998031496062994128, -0.3460692066303957537, -1.113517060367454015 ) ) ;
#27811=CARTESIAN_POINT ( 'NONE',  ( -0.3917322834645669549, -0.1049643490035306603, -2.715223097112860806 ) ) ;
#27814=CARTESIAN_POINT ( 'NONE',  ( 0.1998031496062992740, 0.3460692066303959757, -0.4593175853018372501 ) ) ;
#27817=CARTESIAN_POINT ( 'NONE',  ( -0.1958661417322834220, -0.3392501089628018884, -2.262467191601049699 ) ) ;
#27828=CARTESIAN_POINT ( 'NONE',  ( -0.3392501089628018329, -0.1958661417322836440, -1.707329765582990211 ) ) ;
#27833=ORIENTED_EDGE ( 'NONE', *, *, #15253, .F. ) ;
#27834=CARTESIAN_POINT ( 'NONE',  ( 0.1974969037888706369, -0.3420746716998659953, 0.06561679790026241077 ) ) ;
#27844=CARTESIAN_POINT ( 'NONE',  ( -0.3917322834645669549, -0.1049643490035306603, -1.705380577427821898 ) ) ;
#27854=CARTESIAN_POINT ( 'NONE',  ( 0.1070741851644053527, 0.3996062992125986590, -2.040682414698162361 ) ) ;
#27860=CARTESIAN_POINT ( 'NONE',  ( 0.2362204724409451007, -0.4091458600556402980, -0.7985564304461942875 ) ) ;
#27863=CARTESIAN_POINT ( 'NONE',  ( 0.3420746716998660508, 0.1974969037888705814, -0.2080052493438320771 ) ) ;
#27868=CARTESIAN_POINT ( 'NONE',  ( -0.2891555358219911054, 0.2891555358219909388, -0.5688976377952756902 ) ) ;
#27875=CARTESIAN_POINT ( 'NONE',  ( 0.3460692066303958092, 0.1998031496062993018, -1.152887139107611425 ) ) ;
#27877=CARTESIAN_POINT ( 'NONE',  ( -0.1049643490035307020, 0.3917322834645669549, -1.258530183727033958 ) ) ;
#27890=CARTESIAN_POINT ( 'NONE',  ( 0.3458507752293908943, 0.3458507752293908943, -2.734251968503936148 ) ) ;
#27906=CARTESIAN_POINT ( 'NONE',  ( 0.2925321140481932369, -0.2925321140481931814, -0.7283464566929134243 ) ) ;
#27911=CARTESIAN_POINT ( 'NONE',  ( -0.2925321140481930704, -0.2925321140481933480, -2.578740157480315265 ) ) ;
#27912=CARTESIAN_POINT ( 'NONE',  ( 0.3420746716998659953, 0.1974969037888705536, -2.178477690288714186 ) ) ;
#27914=CARTESIAN_POINT ( 'NONE',  ( 0.1049643490035304938, -0.3917322834645669549, -0.8648293963254591876 ) ) ;
#27917=CARTESIAN_POINT ( 'NONE',  ( -0.1049643490035302024, -0.3917322834645671215, -1.166666666666666519 ) ) ;
#27919=CARTESIAN_POINT ( 'NONE',  ( 0.3949938075777409963, 2.418639510665530743E-17, -2.872047244094488416 ) ) ;
#27926=CARTESIAN_POINT ( 'NONE',  ( 0.3996062992125986035, 2.446882876249141962E-17, -2.637795275590551380 ) ) ;
#27927=CARTESIAN_POINT ( 'NONE',  ( 0.2867679344610366554, 0.2867679344610366554, -1.394376271162416359 ) ) ;
#27933=CARTESIAN_POINT ( 'NONE',  ( -0.1049643490035302024, -0.3917322834645671215, -0.6292650918635172008 ) ) ;
#27941=CARTESIAN_POINT ( 'NONE',  ( -0.2362204724409451284, 0.4091458600556402425, -0.5623359580052492701 ) ) ;
#27942=CARTESIAN_POINT ( 'NONE',  ( 0.2867679344610365999, -0.2867679344610365444, -1.980314960629921073 ) ) ;
#27944=CARTESIAN_POINT ( 'NONE',  ( 4.893765752498283924E-17, -0.3996062992125986035, -0.3937007874015748254 ) ) ;
#27951=CARTESIAN_POINT ( 'NONE',  ( -0.2867679344610364334, -0.2867679344610367109, -1.403543307086614123 ) ) ;
#27960=CARTESIAN_POINT ( 'NONE',  ( 0.3983403474834781299, 0.03178304480585100733, -1.929133858267716661 ) ) ;
#27971=CARTESIAN_POINT ( 'NONE',  ( -0.3917322834645669549, -7.196005306013483243E-17, -1.221765461121048224 ) ) ;
#27974=CARTESIAN_POINT ( 'NONE',  ( 0.4724409448818889246, 0.1265901696525005560, -0.7545931758530183275 ) ) ;
#27980=CARTESIAN_POINT ( 'NONE',  ( -0.2867679344610365444, -0.2867679344610367664, -0.05579359399706226158 ) ) ;
#27982=CARTESIAN_POINT ( 'NONE',  ( -0.4091458600556402980, -0.2362204724409451284, -0.2099737532808398921 ) ) ;
#27983=CARTESIAN_POINT ( 'NONE',  ( 0.4091458600556404646, -0.2362204724409448231, -1.441601049868766582 ) ) ;
#27999=CARTESIAN_POINT ( 'NONE',  ( 0.1998031496062994128, -0.3460692066303957537, -2.845800524934383624 ) ) ;
#28004=CARTESIAN_POINT ( 'NONE',  ( -0.3996062992125986590, 0.1070741851644051723, -1.841863517060367661 ) ) ;
#28009=CARTESIAN_POINT ( 'NONE',  ( 0.2925321140481931814, 0.2925321140481931814, -1.159448818897637734 ) ) ;
#28010=CARTESIAN_POINT ( 'NONE',  ( 0.1998031496062992740, 0.3460692066303959757, -1.404199475065616820 ) ) ;
#28011=CARTESIAN_POINT ( 'NONE',  ( -0.1974969037888706647, 0.3420746716998658843, -1.115485564304461885 ) ) ;
#28012=CARTESIAN_POINT ( 'NONE',  ( 0.2867679344610366554, -0.2867679344610365444, -0.2480314960629920740 ) ) ;
#28016=CARTESIAN_POINT ( 'NONE',  ( 0.3949938075777408852, 0.1058382717557500435, -1.618766404199474929 ) ) ;
#28021=CARTESIAN_POINT ( 'NONE',  ( 0.4724409448818897572, -0.1265901696524988906, -2.158792650918635037 ) ) ;
#28030=CARTESIAN_POINT ( 'NONE',  ( -9.594673741351310580E-17, 0.3917322834645669549, -2.599718217026559586 ) ) ;
#28037=CARTESIAN_POINT ( 'NONE',  ( -9.594673741351313045E-17, 0.3917322834645670104, 0.2303149606299211838 ) ) ;
#28039=CARTESIAN_POINT ( 'NONE',  ( -0.3392501089628019995, 0.1958661417322832277, -2.065616797900262647 ) ) ;
#28042=CARTESIAN_POINT ( 'NONE',  ( -0.2891555358219908833, -0.2891555358219912164, -2.106299212598425452 ) ) ;
#28047=CARTESIAN_POINT ( 'NONE',  ( 0.3996062992125986035, 2.446882876249141962E-17, -0.5905511811023621549 ) ) ;
#28053=CARTESIAN_POINT ( 'NONE',  ( -0.2867679344610365999, 0.2867679344610364889, 0.05314960629921249707 ) ) ;
#28060=CARTESIAN_POINT ( 'NONE',  ( -0.1958661417322834220, -0.3392501089628018884, 0.09973753280839897650 ) ) ;
#28064=DIRECTION ( 'NONE',  ( 1.000000000000000000, 0.000000000000000000, 0.000000000000000000 ) ) ;
#28065=CARTESIAN_POINT ( 'NONE',  ( -0.1265901696524993347, 0.4724409448818895907, -1.423884514435695525 ) ) ;
#28066=DIRECTION ( 'NONE',  ( -0.000000000000000000, -0.000000000000000000, 1.000000000000000000 ) ) ;
#28067=CARTESIAN_POINT ( 'NONE',  ( 0.3917322834645670104, 2.398668435337828261E-17, -0.7401574803149605364 ) ) ;
#28068=CARTESIAN_POINT ( 'NONE',  ( 0.1958661417322834775, 0.3392501089628018884, -2.433727034120734878 ) ) ;
#28071=CARTESIAN_POINT ( 'NONE',  ( 0.1998031496062992463, 0.3460692066303959202, -0.06364829396325462352 ) ) ;
#28076=CARTESIAN_POINT ( 'NONE',  ( 4.797336870675655290E-17, -0.3917322834645669549, -0.001293020176166160412 ) ) ;
#28078=CARTESIAN_POINT ( 'NONE',  ( 0.1049643490035303689, 0.3917322834645670104, -0.07808398950131241467 ) ) ;
#28083=CARTESIAN_POINT ( 'NONE',  ( -0.2867679344610364334, -0.2867679344610367109, -2.098425196850393526 ) ) ;
#28088=CARTESIAN_POINT ( 'NONE',  ( 0.4724409448818897572, -0.1265901696524988906, -0.5032808398950130435 ) ) ;
#28099=CARTESIAN_POINT ( 'NONE',  ( -0.2362204724409451284, 0.4091458600556402425, -1.979658792650918597 ) ) ;
#28102=CARTESIAN_POINT ( 'NONE',  ( -0.2925321140481930149, -0.2925321140481933480, -1.553149606299212726 ) ) ;
#28111=CYLINDRICAL_SURFACE ( 'NONE', #80269, 0.4724409448818898682 ) ;
#28112=CARTESIAN_POINT ( 'NONE',  ( 0.3460692066303959757, -0.1998031496062991907, 0.05249343832020996609 ) ) ;
#28113=CARTESIAN_POINT ( 'NONE',  ( 0.1049643490035303967, 0.3917322834645670659, -2.352381520506248602 ) ) ;
#28118=CARTESIAN_POINT ( 'NONE',  ( -0.1049643490035307020, 0.3917322834645669549, -2.453412073490813139 ) ) ;
#28123=CARTESIAN_POINT ( 'NONE',  ( 0.1998031496062992740, 0.3460692066303959757, -2.034120734908136718 ) ) ;
#28127=CARTESIAN_POINT ( 'NONE',  ( 0.2867679344610366554, -0.2867679344610365999, -0.5676046176191095194 ) ) ;
#28128=ORIENTED_EDGE ( 'NONE', *, *, #15253, .T. ) ;
#28140=CARTESIAN_POINT ( 'NONE',  ( 0.1958661417322834775, 0.3392501089628018884, -0.6089238845144356871 ) ) ;
#28142=ORIENTED_EDGE ( 'NONE', *, *, #28554, .F. ) ;
#28143=CARTESIAN_POINT ( 'NONE',  ( -0.2891555358219911054, 0.2891555358219909388, -1.122047244094488194 ) ) ;
#28160=CARTESIAN_POINT ( 'NONE',  ( 0.2925321140481932369, 0.2925321140481932369, -1.555118110236220597 ) ) ;
#28162=CARTESIAN_POINT ( 'NONE',  ( 0.2925321140481932369, -0.2925321140481931814, -1.277559055118109965 ) ) ;
#28163=CARTESIAN_POINT ( 'NONE',  ( 0.2925321140481932369, -0.2925321140481931814, -0.4901574803149606474 ) ) ;
#28165=CARTESIAN_POINT ( 'NONE',  ( 0.1265901696524990294, -0.4724409448818896462, 0.07217847769028870597 ) ) ;
#28166=CARTESIAN_POINT ( 'NONE',  ( -0.3392501089628017219, -0.1958661417322836718, -2.341863517060367439 ) ) ;
#28172=CARTESIAN_POINT ( 'NONE',  ( 0.1265901696524990294, -0.4724409448818896462, -1.736876640419947604 ) ) ;
#28175=CARTESIAN_POINT ( 'NONE',  ( -0.2891555358219909388, -0.2891555358219912164, -1.710629921259842590 ) ) ;
#28185=CARTESIAN_POINT ( 'NONE',  ( 0.3996062992125984925, 0.1070741851644054637, -2.406167979002624246 ) ) ;
#28186=CARTESIAN_POINT ( 'NONE',  ( -0.3917322834645669549, -7.196005306013483243E-17, -2.481607980806087799 ) ) ;
#28198=CARTESIAN_POINT ( 'NONE',  ( 0.1070741851644054776, -0.3996062992125984925, -0.1620734908136483021 ) ) ;
#28200=CARTESIAN_POINT ( 'NONE',  ( -0.3917322834645671215, 0.1049643490035301469, -2.007217847769029007 ) ) ;
#28209=CARTESIAN_POINT ( 'NONE',  ( 0.2925321140481932369, 0.2925321140481932369, -0.8444881889763780070 ) ) ;
#28215=CARTESIAN_POINT ( 'NONE',  ( 0.3948464311378731550, 0.01987007963502800123, -1.220472440944882608 ) ) ;
#28225=CARTESIAN_POINT ( 'NONE',  ( 0.2925321140481932369, -0.2925321140481932369, -0.4133858267716534196 ) ) ;
#28228=CARTESIAN_POINT ( 'NONE',  ( -0.3917322834645671215, 0.1049643490035301469, -2.072178477690288734 ) ) ;
#28239=CARTESIAN_POINT ( 'NONE',  ( -0.3917322834645668994, -0.1049643490035306742, -1.700768085792964346 ) ) ;
#28245=CARTESIAN_POINT ( 'NONE',  ( 0.3917322834645670659, -0.1049643490035303273, -2.785452386647981449 ) ) ;
#28254=CARTESIAN_POINT ( 'NONE',  ( 0.3917322834645669549, 0.1049643490035304660, -2.099081364829396446 ) ) ;
#28259=CARTESIAN_POINT ( 'NONE',  ( 0.2867679344610365999, -0.2867679344610365444, -2.925196850393700920 ) ) ;
#28261=CARTESIAN_POINT ( 'NONE',  ( -0.1998031496062991630, -0.3460692066303959202, 0.01509186351706036204 ) ) ;
#28263=CARTESIAN_POINT ( 'NONE',  ( -0.1998031496062994683, 0.3460692066303958092, -2.060367454068241511 ) ) ;
#28269=CARTESIAN_POINT ( 'NONE',  ( 0.4091458600556403535, 0.2362204724409449896, -0.5229658792650918597 ) ) ;
#28272=CARTESIAN_POINT ( 'NONE',  ( 0.1058382717557500852, -0.3949938075777408852, -0.6345144356955381149 ) ) ;
#28277=CARTESIAN_POINT ( 'NONE',  ( 0.3420746716998660508, -0.1974969037888704149, -0.4967191601049869010 ) ) ;
#28281=CARTESIAN_POINT ( 'NONE',  ( -0.2362204724409447953, -0.4091458600556404646, -0.1423884514435695414 ) ) ;
#28284=CARTESIAN_POINT ( 'NONE',  ( -0.3460692066303960313, 0.1998031496062989965, -1.205380577427821454 ) ) ;
#28286=CARTESIAN_POINT ( 'NONE',  ( -0.2867679344610364334, -0.2867679344610367109, -0.9960629921259842590 ) ) ;
#28299=CARTESIAN_POINT ( 'NONE',  ( -9.787531504996566615E-17, 0.3996062992125985480, 0.2381889763779527491 ) ) ;
#28318=CARTESIAN_POINT ( 'NONE',  ( -0.1070741851644051862, -0.3996062992125986590, -0.7020997375328084100 ) ) ;
#28322=CARTESIAN_POINT ( 'NONE',  ( -0.4724409448818899238, 0.1265901696524986686, 0.1246719160104986929 ) ) ;
#28323=CARTESIAN_POINT ( 'NONE',  ( -9.674558042662121740E-17, 0.3949938075777409963, -2.362204724409449064 ) ) ;
#28326=CARTESIAN_POINT ( 'NONE',  ( -0.3917322834645669549, -0.1049643490035306603, -0.8254593175853015552 ) ) ;
#28332=CARTESIAN_POINT ( 'NONE',  ( -0.3392501089628019439, 0.1958661417322832554, -0.2637602117772160915 ) ) ;
#28338=DIRECTION ( 'NONE',  ( 0.000000000000000000, 0.000000000000000000, 1.000000000000000000 ) ) ;
#28339=CARTESIAN_POINT ( 'NONE',  ( -0.3996062992125987146, 0.1070741851644051862, -2.867454068241469756 ) ) ;
#28340=CARTESIAN_POINT ( 'NONE',  ( 0.3917322834645670104, 0.1049643490035304660, -1.538733226542994048 ) ) ;
#28346=CARTESIAN_POINT ( 'NONE',  ( -0.3917322834645669549, -0.1049643490035306603, -1.075459317585301777 ) ) ;
#28355=CARTESIAN_POINT ( 'NONE',  ( 0.3917322834645670104, -0.1049643490035303411, -2.465879265091863282 ) ) ;
#28356=ORIENTED_EDGE ( 'NONE', *, *, #76928, .F. ) ;
#28363=CARTESIAN_POINT ( 'NONE',  ( -9.594673741351313045E-17, 0.3917322834645670104, -1.187007874015748143 ) ) ;
#28364=CARTESIAN_POINT ( 'NONE',  ( -0.3460692066303960313, 0.1998031496062989965, -2.150262467191601079 ) ) ;
#28373=CARTESIAN_POINT ( 'NONE',  ( 0.1998031496062992463, 0.3460692066303959202, -2.110892388451443669 ) ) ;
#28383=CARTESIAN_POINT ( 'NONE',  ( 0.3917322834645668994, -0.1049643490035303134, -1.293943938811336958 ) ) ;
#28393=CARTESIAN_POINT ( 'NONE',  ( -0.3917322834645671770, 0.1049643490035302024, -0.5019878197188469837 ) ) ;
#28397=CARTESIAN_POINT ( 'NONE',  ( 0.3458507752293908943, -0.3458507752293908943, -1.750000000000000222 ) ) ;
#28413=CARTESIAN_POINT ( 'NONE',  ( 0.1058382717557500852, -0.3949938075777408852, 0.1528871391076115638 ) ) ;
#28418=CARTESIAN_POINT ( 'NONE',  ( 0.1070741851644054776, -0.3996062992125984925, -2.209317585301837639 ) ) ;
#28424=CARTESIAN_POINT ( 'NONE',  ( 0.3996062992125986590, -0.1070741851644053111, -1.843832020997375309 ) ) ;
#28425=CARTESIAN_POINT ( 'NONE',  ( 4.837279021331060870E-17, -0.3949938075777409963, -1.181102362204724532 ) ) ;
#28426=CARTESIAN_POINT ( 'NONE',  ( -0.1070741851644056997, 0.3996062992125986035, -2.526246719160104792 ) ) ;
#28428=CARTESIAN_POINT ( 'NONE',  ( -0.3917322834645669549, -0.1049643490035306603, -0.3530183727034120755 ) ) ;
#28433=CARTESIAN_POINT ( 'NONE',  ( 0.1974969037888706092, -0.3420746716998660508, -2.215879265091863726 ) ) ;
#28437=CARTESIAN_POINT ( 'NONE',  ( -0.3458507752293909498, 0.3458507752293907833, -1.909448818897637512 ) ) ;
#28445=CARTESIAN_POINT ( 'NONE',  ( 0.1958661417322834497, 0.3392501089628018329, -2.271634227525247685 ) ) ;
#28448=CARTESIAN_POINT ( 'NONE',  ( 5.785732909357575061E-17, -0.4724409448818898682, -2.440944881889763884 ) ) ;
#28452=CARTESIAN_POINT ( 'NONE',  ( -0.1958661417322836718, 0.3392501089628017219, 0.2171916010498686767 ) ) ;
#28454=CARTESIAN_POINT ( 'NONE',  ( 0.3392501089628018329, 0.1958661417322835607, -1.855643044619422533 ) ) ;
#28457=CARTESIAN_POINT ( 'NONE',  ( 0.3420746716998659953, 0.1974969037888705536, -2.493438320209973469 ) ) ;
#28461=CARTESIAN_POINT ( 'NONE',  ( 0.3996062992125986035, 2.446882876249141962E-17, -0.9055118110236221041 ) ) ;
#28466=CARTESIAN_POINT ( 'NONE',  ( 4.797336870675656522E-17, -0.3917322834645670104, -0.005905511811023714773 ) ) ;
#28477=( CONVERSION_BASED_UNIT ( 'INCH', #10382 ) LENGTH_UNIT ( ) NAMED_UNIT ( #56680 ) );
#28478=CARTESIAN_POINT ( 'NONE',  ( 0.3458507752293908943, 0.3458507752293908943, -1.397637795275590067 ) ) ;
#28481=CARTESIAN_POINT ( 'NONE',  ( 0.2867679344610365999, 0.2867679344610365999, -0.7598425196850391306 ) ) ;
#28482=CARTESIAN_POINT ( 'NONE',  ( 0.3917322834645670104, 2.398668435337828261E-17, -2.564960629921259727 ) ) ;
#28485=CARTESIAN_POINT ( 'NONE',  ( 0.3460692066303958092, 0.1998031496062993018, -0.2080052493438320771 ) ) ;
#28490=CARTESIAN_POINT ( 'NONE',  ( -0.3917322834645670659, 0.1049643490035301607, -0.1128415766066123566 ) ) ;
#28492=CARTESIAN_POINT ( 'NONE',  ( 0.3392501089628018884, -0.1958661417322834220, -0.3471128608923885195 ) ) ;
#28499=CARTESIAN_POINT ( 'NONE',  ( -0.2867679344610364334, -0.2867679344610367109, -1.940944881889763884 ) ) ;
#28503=CARTESIAN_POINT ( 'NONE',  ( -1.157146581871515012E-16, 0.4724409448818898682, -0.5492125984251968740 ) ) ;
#28515=CARTESIAN_POINT ( 'NONE',  ( -0.1070741851644051862, -0.3996062992125986590, -1.723753280839894986 ) ) ;
#28524=CARTESIAN_POINT ( 'NONE',  ( 0.1070741851644053527, 0.3996062992125986590, -0.3083989501312335846 ) ) ;
#28525=CARTESIAN_POINT ( 'NONE',  ( -0.3949938075777411628, 0.1058382717557497937, -0.03280839895013128865 ) ) ;
#28527=CARTESIAN_POINT ( 'NONE',  ( -0.009287274676460672077, -0.3937527723457948658, -2.032323646524292649E-15 ) ) ;
#28531=CARTESIAN_POINT ( 'NONE',  ( -0.3917322834645671215, 0.1049643490035301469, -2.479658792650918375 ) ) ;
#28536=CARTESIAN_POINT ( 'NONE',  ( 0.2362204724409449064, 0.4091458600556404646, -0.7742782152230971437 ) ) ;
#28537=CARTESIAN_POINT ( 'NONE',  ( -0.3996062992125986035, -1.273259842764937629E-12, -1.929133858267794599 ) ) ;
#28540=CARTESIAN_POINT ( 'NONE',  ( 0.1958661417322834775, 0.3392501089628018884, -0.2985757462280333452 ) ) ;
#28554=EDGE_CURVE ( 'NONE', #53885, #21217, #61900, .T. ) ;
#28556=CARTESIAN_POINT ( 'NONE',  ( -9.594673741351313045E-17, 0.3917322834645670104, -0.4645669291338582751 ) ) ;
#28559=CARTESIAN_POINT ( 'NONE',  ( -0.3949938075777409408, -0.1058382717557502933, -0.9908136482939633449 ) ) ;
#28575=CARTESIAN_POINT ( 'NONE',  ( -0.3460692066303960868, 0.1998031496062990242, -1.758530183727034180 ) ) ;
#28578=CARTESIAN_POINT ( 'NONE',  ( -0.1070741851644051862, -0.3996062992125986590, -1.251312335958005173 ) ) ;
#28579=CARTESIAN_POINT ( 'NONE',  ( 4.893765752498283308E-17, -0.3996062992125985480, -0.6279527559055118058 ) ) ;
#28582=CARTESIAN_POINT ( 'NONE',  ( 0.4724409448818897572, -0.1265901696524988906, 0.04593175853018372640 ) ) ;
#28584=CARTESIAN_POINT ( 'NONE',  ( -0.2867679344610364334, -0.2867679344610367109, -2.663385826771653253 ) ) ;
#28590=CARTESIAN_POINT ( 'NONE',  ( 0.2362204724409451007, -0.4091458600556402980, -1.743438320209973469 ) ) ;
#28593=CARTESIAN_POINT ( 'NONE',  ( -0.3949938075777408852, -0.1058382717557502933, -1.854986876640420501 ) ) ;
#28602=CARTESIAN_POINT ( 'NONE',  ( -0.1070741851644051862, -0.3996062992125986590, -2.668635170603674833 ) ) ;
#28603=CARTESIAN_POINT ( 'NONE',  ( 0.1958661417322836162, -0.3392501089628018329, -2.376621104165667298 ) ) ;
#28616=CARTESIAN_POINT ( 'NONE',  ( -0.3460692066303957537, -0.1998031496062994405, -0.1292650918635170620 ) ) ;
#28618=CARTESIAN_POINT ( 'NONE',  ( -0.1958661417322834220, -0.3392501089628018884, -1.725065616797900381 ) ) ;
#28628=CARTESIAN_POINT ( 'NONE',  ( -9.787531504996566615E-17, 0.3996062992125985480, -1.021653543307086576 ) ) ;
#28631=ORIENTED_EDGE ( 'NONE', *, *, #35272, .T. ) ;
#28643=CARTESIAN_POINT ( 'NONE',  ( -0.1998031496062991907, -0.3460692066303959757, -0.6955380577427822120 ) ) ;
#28644=VERTEX_POINT ( 'NONE', #39006 ) ;
#28646=CARTESIAN_POINT ( 'NONE',  ( -0.2867679344610364334, -0.2867679344610367109, -2.098425196850393526 ) ) ;
#28647=ORIENTED_EDGE ( 'NONE', *, *, #53516, .T. ) ;
#28652=AXIS2_PLACEMENT_3D ( 'NONE', #82345, #50332, #37709 ) ;
#28657=CARTESIAN_POINT ( 'NONE',  ( 0.1958661417322836162, -0.3392501089628018329, -1.589219529362517758 ) ) ;
#28663=CARTESIAN_POINT ( 'NONE',  ( 0.2891555358219910499, 0.2891555358219910499, 0.01968503937007868437 ) ) ;
#28673=CARTESIAN_POINT ( 'NONE',  ( 4.797336870675656522E-17, -0.3917322834645670104, -2.368110236220472675 ) ) ;
#28680=CARTESIAN_POINT ( 'NONE',  ( 0.2925321140481932369, 0.2925321140481932369, -0.05708661417322836301 ) ) ;
#28682=CARTESIAN_POINT ( 'NONE',  ( -0.1998031496062994683, 0.3460692066303958092, -1.902887139107611647 ) ) ;
#28687=CARTESIAN_POINT ( 'NONE',  ( 0.1265901696524990294, -0.4724409448818896462, -0.4770341207349080848 ) ) ;
#28690=CARTESIAN_POINT ( 'NONE',  ( 0.3420746716998660508, -0.1974969037888704149, -0.6541994750656167090 ) ) ;
#28695=CARTESIAN_POINT ( 'NONE',  ( 4.837279021331061486E-17, -0.3949938075777409963, -0.6279527559055118058 ) ) ;
#28702=CARTESIAN_POINT ( 'NONE',  ( 0.1998031496062994128, -0.3460692066303957537, -1.428477690288713964 ) ) ;
#28704=CARTESIAN_POINT ( 'NONE',  ( -0.2867679344610364334, -0.2867679344610367109, -1.153543307086613900 ) ) ;
#28706=CARTESIAN_POINT ( 'NONE',  ( -0.3272402980636380243, 0.2155943732411919889, 6.867566722516314874E-18 ) ) ;
#28719=CARTESIAN_POINT ( 'NONE',  ( 5.785732909357575061E-17, -0.4724409448818898682, -0.3129921259842520231 ) ) ;
#28734=CARTESIAN_POINT ( 'NONE',  ( 0.3996062992125985480, 0.1070741851644054637, -0.9120734908136483021 ) ) ;
#28738=CARTESIAN_POINT ( 'NONE',  ( 0.1265901696524990294, -0.4724409448818896462, 0.07217847769028870597 ) ) ;
#28739=CARTESIAN_POINT ( 'NONE',  ( 0.2891555358219910499, -0.2891555358219909944, -2.303149606299212504 ) ) ;
#28742=CARTESIAN_POINT ( 'NONE',  ( 0.3392501089628018884, -0.1958661417322834220, -0.8845144356955378928 ) ) ;
#28749=CARTESIAN_POINT ( 'NONE',  ( 0.3392501089628018329, -0.1958661417322834497, -0.3425003692575309677 ) ) ;
#28754=CARTESIAN_POINT ( 'NONE',  ( -1.157146581871515012E-16, 0.4724409448818898682, 0.000000000000000000 ) ) ;
#28755=CARTESIAN_POINT ( 'NONE',  ( -0.1070741851644056997, 0.3996062992125986035, -2.841207349081364963 ) ) ;
#28756=CARTESIAN_POINT ( 'NONE',  ( 4.797336870675656522E-17, -0.3917322834645670659, -1.650281782973440192 ) ) ;
#28762=CARTESIAN_POINT ( 'NONE',  ( 0.3917322834645669549, 0.1049643490035304660, -1.154199475065616820 ) ) ;
#28772=CARTESIAN_POINT ( 'NONE',  ( -0.2867679344610364334, -0.2867679344610367109, -2.255905511811023612 ) ) ;
#28781=CARTESIAN_POINT ( 'NONE',  ( -0.2867679344610365999, 0.2867679344610364889, -1.206692913385826627 ) ) ;
#28783=CARTESIAN_POINT ( 'NONE',  ( 0.1998031496062994128, -0.3460692066303957537, -2.373359580052493367 ) ) ;
#28791=CARTESIAN_POINT ( 'NONE',  ( 0.1998031496062994128, -0.3460692066303957537, -2.058398950131233640 ) ) ;
#28793=CARTESIAN_POINT ( 'NONE',  ( 0.1958661417322834775, 0.3392501089628018884, 0.02099737532808403431 ) ) ;
#28800=CARTESIAN_POINT ( 'NONE',  ( 0.3392501089628018329, -0.1958661417322834497, -1.287382259021310427 ) ) ;
#28809=CARTESIAN_POINT ( 'NONE',  ( -9.594673741351313045E-17, 0.3917322834645670659, -0.4691794207687158269 ) ) ;
#28813=CARTESIAN_POINT ( 'NONE',  ( 0.3458507752293908943, 0.3458507752293908943, -1.789370078740157410 ) ) ;
#28833=CARTESIAN_POINT ( 'NONE',  ( 4.893765752498283308E-17, -0.3996062992125985480, -2.360236220472441193 ) ) ;
#28838=CARTESIAN_POINT ( 'NONE',  ( -0.3996062992125987146, 0.1070741851644051862, -1.922572178477689908 ) ) ;
#28840=CARTESIAN_POINT ( 'NONE',  ( -0.2891555358219911054, 0.2891555358219909388, -1.122047244094488194 ) ) ;
#28841=CARTESIAN_POINT ( 'NONE',  ( 0.3460692066303959202, 0.1998031496062993295, -2.335958005249343827 ) ) ;
#28843=CARTESIAN_POINT ( 'NONE',  ( -0.1049643490035301885, -0.3917322834645671215, -0.3792650918635169788 ) ) ;
#28847=CARTESIAN_POINT ( 'NONE',  ( 4.837279021331061486E-17, -0.3949938075777409963, -2.202755905511811108 ) ) ;
#28851=CARTESIAN_POINT ( 'NONE',  ( 0.4724409448818897572, -0.1265901696524988906, -2.473753280839894764 ) ) ;
#28852=CARTESIAN_POINT ( 'NONE',  ( -0.1998031496062994683, 0.3460692066303958092, -1.902887139107611647 ) ) ;
#28860=CARTESIAN_POINT ( 'NONE',  ( 0.2867679344610365999, -0.2867679344610365444, 0.1318897637795274913 ) ) ;
#28863=CARTESIAN_POINT ( 'NONE',  ( 0.4724409448818898682, 2.892866454678787531E-17, -2.480314960629921295 ) ) ;
#28867=CARTESIAN_POINT ( 'NONE',  ( 0.3392501089628018329, 0.1958661417322835607, -0.05839895013123368173 ) ) ;
#28869=CARTESIAN_POINT ( 'NONE',  ( 0.2867679344610365999, 0.2867679344610365999, -2.334645669291338432 ) ) ;
#28872=CARTESIAN_POINT ( 'NONE',  ( 0.2891555358219910499, -0.2891555358219909944, -2.460629921259842590 ) ) ;
#28876=CARTESIAN_POINT ( 'NONE',  ( -0.3460692066303958092, -0.1998031496062994683, -1.154855643044619518 ) ) ;
#28881=CARTESIAN_POINT ( 'NONE',  ( -0.3917322834645669549, -0.1049643490035306603, -0.1305774278215224293 ) ) ;
#28894=CARTESIAN_POINT ( 'NONE',  ( 0.1265901696524989462, 0.4724409448818897572, -1.883202099737532276 ) ) ;
#28896=CARTESIAN_POINT ( 'NONE',  ( -0.1049643490035302024, -0.3917322834645671215, -0.8517060367454066805 ) ) ;
#28897=CARTESIAN_POINT ( 'NONE',  ( -1.157146581871515012E-16, 0.4724409448818898682, -0.9448818897637796255 ) ) ;
#28901=CARTESIAN_POINT ( 'NONE',  ( 0.4724409448818898682, 2.892866454678787531E-17, -2.007874015748031482 ) ) ;
#28905=CARTESIAN_POINT ( 'NONE',  ( 0.2867679344610365999, -0.2867679344610365999, 0.1365022554143850153 ) ) ;
#28907=CARTESIAN_POINT ( 'NONE',  ( 0.2867679344610366554, -0.2867679344610365444, -0.4980314960629921850 ) ) ;
#28912=CARTESIAN_POINT ( 'NONE',  ( 4.797336870675656522E-17, -0.3917322834645670104, -2.433070866141732402 ) ) ;
#28915=CARTESIAN_POINT ( 'NONE',  ( -0.4724409448818898682, -8.678599364036362592E-17, -0.4311023622047244208 ) ) ;
#28922=CARTESIAN_POINT ( 'NONE',  ( 0.4091458600556403535, 0.2362204724409449896, -1.940288713910761187 ) ) ;
#28924=CARTESIAN_POINT ( 'NONE',  ( 0.3460692066303959202, -0.1998031496062991630, -1.756561679790026309 ) ) ;
#28933=CARTESIAN_POINT ( 'NONE',  ( 0.1070741851644054637, -0.3996062992125984925, -0.3195538057742782212 ) ) ;
#28934=CARTESIAN_POINT ( 'NONE',  ( -0.1998031496062994683, 0.3460692066303958092, -0.3280839895013123453 ) ) ;
#28935=CARTESIAN_POINT ( 'NONE',  ( -0.3917322834645670659, -7.196005306013484475E-17, -2.870754223918321912 ) ) ;
#28940=LINE ( 'NONE', #47461, #33192 ) ;
#28943=CARTESIAN_POINT ( 'NONE',  ( 0.3949938075777408852, 0.1058382717557500435, -0.9888451443569553634 ) ) ;
#28949=CARTESIAN_POINT ( 'NONE',  ( 0.4091458600556403535, 0.2362204724409449896, -1.391076115485564424 ) ) ;
#28950=CARTESIAN_POINT ( 'NONE',  ( 0.1070741851644054915, -0.3996062992125985480, -2.290026246719159886 ) ) ;
#28953=CARTESIAN_POINT ( 'NONE',  ( -0.3392501089628017219, -0.1958661417322836995, -0.5216728590889256889 ) ) ;
#28954=EDGE_LOOP ( 'NONE', ( #14606, #36619, #50375, #16544, #14397, #52794, #11910, #62392, #75531, #30623, #34804, #51278, #46315, #24975 ) ) ;
#28965=CARTESIAN_POINT ( 'NONE',  ( 4.797336870675656522E-17, -0.3917322834645670104, -0.8582677165354329896 ) ) ;
#28968=CARTESIAN_POINT ( 'NONE',  ( -0.3949938075777409963, -7.255918531996591613E-17, -1.141732283464566899 ) ) ;
#28972=CARTESIAN_POINT ( 'NONE',  ( 0.3460692066303959202, 0.1998031496062993295, 0.02624671916010497957 ) ) ;
#28984=CARTESIAN_POINT ( 'NONE',  ( -0.1070741851644051862, -0.3996062992125987146, -1.489501312335957950 ) ) ;
#28987=CARTESIAN_POINT ( 'NONE',  ( -0.2925321140481930149, -0.2925321140481933480, -1.080708661417322691 ) ) ;
#28988=CARTESIAN_POINT ( 'NONE',  ( -0.2925321140481932369, 0.2925321140481931259, -0.4114173228346455491 ) ) ;
#28991=CARTESIAN_POINT ( 'NONE',  ( -0.2362204724409451284, 0.4091458600556402425, -0.01312335958005249326 ) ) ;
#28992=CARTESIAN_POINT ( 'NONE',  ( 0.1958661417322836440, -0.3392501089628017219, -2.696194225721784576 ) ) ;
#28998=CARTESIAN_POINT ( 'NONE',  ( -0.4091458600556402980, -0.2362204724409451284, -2.176509186351706315 ) ) ;
#29001=CARTESIAN_POINT ( 'NONE',  ( -0.3949938075777411073, 0.1058382717557497660, -1.684383202099737575 ) ) ;
#29007=CARTESIAN_POINT ( 'NONE',  ( 0.1265901696524989184, 0.4724409448818898127, -2.274934383202099397 ) ) ;
#29012=CARTESIAN_POINT ( 'NONE',  ( -0.1958661417322834497, -0.3392501089628018884, -2.507854699966192147 ) ) ;
#29026=CARTESIAN_POINT ( 'NONE',  ( -0.2925321140481930149, -0.2925321140481933480, -0.1358267716535432879 ) ) ;
#29028=CARTESIAN_POINT ( 'NONE',  ( 0.1049643490035304938, -0.3917322834645669549, -1.744750656167979308 ) ) ;
#29033=DIRECTION ( 'NONE',  ( 0.000000000000000000, 0.000000000000000000, 1.000000000000000000 ) ) ;
#29037=CARTESIAN_POINT ( 'NONE',  ( -0.3996062992125984925, -0.1070741851644056858, -1.067585301837270517 ) ) ;
#29045=CARTESIAN_POINT ( 'NONE',  ( -0.1049643490035302024, -0.3917322834645671215, -1.731627296587926468 ) ) ;
#29046=CARTESIAN_POINT ( 'NONE',  ( 0.2579773093944593976, 0.2955417804206795784, -1.220472440944881942 ) ) ;
#29052=CARTESIAN_POINT ( 'NONE',  ( -0.1070741851644051862, -0.3996062992125986035, -2.511154855643044748 ) ) ;
#29054=CARTESIAN_POINT ( 'NONE',  ( -0.1070741851644056997, 0.3996062992125986035, -0.3215223097112860362 ) ) ;
#29057=CARTESIAN_POINT ( 'NONE',  ( -0.3917322834645671215, 0.1049643490035301469, -2.229658792650918819 ) ) ;
#29067=CARTESIAN_POINT ( 'NONE',  ( -0.3917322834645670659, 0.1049643490035301607, -1.687644726212911506 ) ) ;
#29073=CARTESIAN_POINT ( 'NONE',  ( 0.3392501089628018329, 0.1958661417322835607, -2.805137426018059710 ) ) ;
#29078=CARTESIAN_POINT ( 'NONE',  ( -1.157146581871515012E-16, 0.4724409448818898682, -0.1574803149606299191 ) ) ;
#29082=CARTESIAN_POINT ( 'NONE',  ( 0.3392501089628018884, -0.1958661417322833942, -1.204087557251655394 ) ) ;
#29084=CARTESIAN_POINT ( 'NONE',  ( -0.2867679344610364334, -0.2867679344610367109, -2.190944881889763440 ) ) ;
#29090=CARTESIAN_POINT ( 'NONE',  ( -0.1070741851644051862, -0.3996062992125986590, 0.008530183727034111943 ) ) ;
#29092=CARTESIAN_POINT ( 'NONE',  ( 4.893765752498283924E-17, -0.3996062992125986035, -1.811023622047244208 ) ) ;
#29097=CARTESIAN_POINT ( 'NONE',  ( 0.4091458600556404646, -0.2362204724409448231, -0.6541994750656167090 ) ) ;
#29101=CARTESIAN_POINT ( 'NONE',  ( -0.2891555358219911054, 0.2891555358219909388, -0.7263779527559056648 ) ) ;
#29107=CARTESIAN_POINT ( 'NONE',  ( 0.1974969037888706092, -0.3420746716998660508, -0.6410761154855643129 ) ) ;
#29111=CARTESIAN_POINT ( 'NONE',  ( -0.3726288332202236653, -0.1208384647423932784, -1.929133858267952473 ) ) ;
#29114=CARTESIAN_POINT ( 'NONE',  ( 0.3996062992125984925, 0.1070741851644054637, -1.461286089238845065 ) ) ;
#29116=AXIS2_PLACEMENT_3D ( 'NONE', #57955, #45747, #26402 ) ;
#29117=CARTESIAN_POINT ( 'NONE',  ( -0.1049643490035302024, -0.3917322834645671215, -1.166666666666666519 ) ) ;
#29121=CARTESIAN_POINT ( 'NONE',  ( -0.2898214735618663274, -0.2643935821217201498, -4.446769521226820888E-17 ) ) ;
#29147=CARTESIAN_POINT ( 'NONE',  ( 0.3996062992125985480, 0.1070741851644054637, -1.069553805774278166 ) ) ;
#29151=CARTESIAN_POINT ( 'NONE',  ( 0.3458507752293908943, -0.3458507752293908943, -0.09842519685039372024 ) ) ;
#29152=CARTESIAN_POINT ( 'NONE',  ( -0.3420746716998661618, 0.1974969037888702206, -2.545931758530183497 ) ) ;
#29155=CARTESIAN_POINT ( 'NONE',  ( 0.2867679344610365999, -0.2867679344610365444, -0.8779527559055116948 ) ) ;
#29157=CARTESIAN_POINT ( 'NONE',  ( -0.1265901696524993347, 0.4724409448818895907, -2.368766404199475151 ) ) ;
#29163=CARTESIAN_POINT ( 'NONE',  ( -0.1958661417322836440, 0.3392501089628016664, -0.2506368521971635843 ) ) ;
#29168=CARTESIAN_POINT ( 'NONE',  ( -0.4724409448818898682, -8.678599364036362592E-17, -0.2736220472440945017 ) ) ;
#29170=CARTESIAN_POINT ( 'NONE',  ( -0.1265901696524993347, 0.4724409448818896462, -1.108923884514435798 ) ) ;
#29171=CARTESIAN_POINT ( 'NONE',  ( -0.1958661417322833942, -0.3392501089628018884, -1.794638738354017660 ) ) ;
#29179=CARTESIAN_POINT ( 'NONE',  ( -0.3917322834645671215, 0.1049643490035301469, -1.062335958005249603 ) ) ;
#29188=CARTESIAN_POINT ( 'NONE',  ( -0.1958661417322836718, 0.3392501089628017219, -2.524934383202099397 ) ) ;
#29195=CARTESIAN_POINT ( 'NONE',  ( -0.3392501089628017219, -0.1958661417322836718, -0.9245406824146982228 ) ) ;
#29197=LINE ( 'NONE', #54443, #45891 ) ;
#29198=CARTESIAN_POINT ( 'NONE',  ( -0.3917322834645671215, 0.1049643490035301469, -1.219816272965879023 ) ) ;
#29200=CARTESIAN_POINT ( 'NONE',  ( 0.1070741851644053388, 0.3996062992125986035, -2.589895013123359568 ) ) ;
#29207=PRODUCT_CONTEXT ( 'NONE', #25567, 'mechanical' ) ;
#29209=CARTESIAN_POINT ( 'NONE',  ( -0.2952755905511810774, 3.616083068348483797E-17, -1.220472440944881942 ) ) ;
#29218=CARTESIAN_POINT ( 'NONE',  ( -0.3917322834645670659, 0.1049643490035301607, -1.057723466370391829 ) ) ;
#29226=CARTESIAN_POINT ( 'NONE',  ( -0.3392501089628017219, -0.1958661417322836995, -0.6791531740495557745 ) ) ;
#29231=CARTESIAN_POINT ( 'NONE',  ( 0.4724409448818898682, 2.892866454678787531E-17, -2.084645669291338432 ) ) ;
#29251=CARTESIAN_POINT ( 'NONE',  ( -0.3996062992125984925, -0.1070741851644056858, -2.012467191601049699 ) ) ;
#29256=CARTESIAN_POINT ( 'NONE',  ( -9.787531504996567848E-17, 0.3996062992125986035, -1.889763779527559251 ) ) ;
#29257=CARTESIAN_POINT ( 'NONE',  ( -0.3949938075777409963, -7.255918531996591613E-17, -1.141732283464566899 ) ) ;
#29258=CARTESIAN_POINT ( 'NONE',  ( -0.1998031496062994683, 0.3460692066303958092, -2.532808398950130879 ) ) ;
#29260=CARTESIAN_POINT ( 'NONE',  ( -0.3392501089628019995, 0.1958661417322832277, -0.1758530183727033402 ) ) ;
#29264=CARTESIAN_POINT ( 'NONE',  ( -0.2891555358219911054, 0.2891555358219909388, -2.143700787401574548 ) ) ;
#29268=CARTESIAN_POINT ( 'NONE',  ( 0.4724409448818896462, 0.1265901696524990294, -2.644356955380577912 ) ) ;
#29269=CARTESIAN_POINT ( 'NONE',  ( -0.3996062992125986035, -0.1070741851644056997, -1.935695538057742526 ) ) ;
#29277=CARTESIAN_POINT ( 'NONE',  ( -0.1958661417322834220, -0.3392501089628018884, 0.1646981627296586759 ) ) ;
#29284=CARTESIAN_POINT ( 'NONE',  ( -0.1958661417322834220, -0.3392501089628018884, -0.1502624671916011345 ) ) ;
#29287=CARTESIAN_POINT ( 'NONE',  ( -0.3392501089628017219, -0.1958661417322836718, -2.406824146981627166 ) ) ;
#29290=CARTESIAN_POINT ( 'NONE',  ( -0.1974969037888706647, 0.3420746716998658843, -2.532808398950130879 ) ) ;
#29295=CARTESIAN_POINT ( 'NONE',  ( -0.1998031496062991907, -0.3460692066303959757, -0.8530183727034120755 ) ) ;
#29299=CARTESIAN_POINT ( 'NONE',  ( 0.1208384647389237204, -0.3726288332213487653, -2.755905511811024056 ) ) ;
#29300=CARTESIAN_POINT ( 'NONE',  ( -0.1049643490035307020, 0.3917322834645669549, 0.06627296587926499727 ) ) ;
#29311=CARTESIAN_POINT ( 'NONE',  ( -0.4091458600556402980, -0.2362204724409451284, -1.627296587926509330 ) ) ;
#29313=CARTESIAN_POINT ( 'NONE',  ( 0.2867679344610365999, -0.2867679344610365444, -0.5629921259842519676 ) ) ;
#29321=CARTESIAN_POINT ( 'NONE',  ( -0.1049643490035301746, -0.3917322834645670659, 0.005268659613860090553 ) ) ;
#29323=CARTESIAN_POINT ( 'NONE',  ( -0.3917322834645670104, -7.196005306013484475E-17, -0.4389763779527560139 ) ) ;
#29328=CARTESIAN_POINT ( 'NONE',  ( 0.3917322834645670104, -0.1049643490035303411, -2.465879265091863282 ) ) ;
#29331=CARTESIAN_POINT ( 'NONE',  ( -0.3458507752293909498, 0.3458507752293907833, -0.7263779527559056648 ) ) ;
#29342=CARTESIAN_POINT ( 'NONE',  ( 0.3996062992125984925, 0.1070741851644054637, -1.618766404199474929 ) ) ;
#29351=CARTESIAN_POINT ( 'NONE',  ( -0.3460692066303960313, 0.1998031496062989965, -0.1030183727034120894 ) ) ;
#29352=CARTESIAN_POINT ( 'NONE',  ( -0.3996062992125986035, -0.1070741851644056997, -0.6758530183727035068 ) ) ;
#29353=CARTESIAN_POINT ( 'NONE',  ( -0.1974969037888703871, -0.3420746716998661063, 0.09186351706036739728 ) ) ;
#29359=CARTESIAN_POINT ( 'NONE',  ( -0.3949938075777409963, -7.255918531996591613E-17, -0.7460629921259843700 ) ) ;
#29364=CARTESIAN_POINT ( 'NONE',  ( -0.1265901696524986964, -0.4724409448818899238, -1.017060367454067915 ) ) ;
#29365=CARTESIAN_POINT ( 'NONE',  ( -0.3460692066303958092, -0.1998031496062994683, -2.414698162729658648 ) ) ;
#29367=VERTEX_POINT ( 'NONE', #53225 ) ;
#29368=CARTESIAN_POINT ( 'NONE',  ( 0.3917322834645670659, 2.398668435337828261E-17, -0.5872896569891882246 ) ) ;
#29380=CARTESIAN_POINT ( 'NONE',  ( 0.3917322834645670104, 2.398668435337828261E-17, -1.212598425196850238 ) ) ;
#29382=ORIENTED_EDGE ( 'NONE', *, *, #45564, .T. ) ;
#29383=CARTESIAN_POINT ( 'NONE',  ( -0.2891555358219908833, -0.2891555358219912164, -0.8464566929133858775 ) ) ;
#29394=CARTESIAN_POINT ( 'NONE',  ( 0.4091458600556404646, -0.2362204724409448231, -0.6541994750656167090 ) ) ;
#29398=EDGE_LOOP ( 'NONE', ( #25434, #26055, #70171, #15332, #9097, #56692 ) ) ;
#29399=CARTESIAN_POINT ( 'NONE',  ( -0.3996062992125987146, 0.1070741851644051862, -1.765091863517059823 ) ) ;
#29402=CARTESIAN_POINT ( 'NONE',  ( 0.3460692066303959202, -0.1998031496062991630, -1.284120734908136496 ) ) ;
#29403=CARTESIAN_POINT ( 'NONE',  ( -0.03175677952935525988, 0.3980111619244049992, -2.755905511811024500 ) ) ;
#29406=CARTESIAN_POINT ( 'NONE',  ( -0.4724409448818899238, 0.1265901696524986686, -0.3477690288713909950 ) ) ;
#29407=CARTESIAN_POINT ( 'NONE',  ( -0.2867679344610364334, -0.2867679344610367109, -2.505905511811023612 ) ) ;
#29413=CARTESIAN_POINT ( 'NONE',  ( 0.2362204724409451007, -0.4091458600556402980, -2.215879265091863726 ) ) ;
#29415=CARTESIAN_POINT ( 'NONE',  ( -0.2891555358219911054, 0.2891555358219909388, -1.671259842519685179 ) ) ;
#29426=CARTESIAN_POINT ( 'NONE',  ( -0.3917322834645669549, -7.196005306013483243E-17, -2.324127665845457713 ) ) ;
#29440=CARTESIAN_POINT ( 'NONE',  ( 0.3996062992125986035, -0.1070741851644052972, -0.3458005249343831244 ) ) ;
#29442=CARTESIAN_POINT ( 'NONE',  ( -0.3917322834645670104, -7.196005306013484475E-17, -1.698818897637795367 ) ) ;
#29452=CARTESIAN_POINT ( 'NONE',  ( 0.3996062992125986035, -0.1070741851644052972, -1.448162729658792669 ) ) ;
#29454=CARTESIAN_POINT ( 'NONE',  ( 0.3458507752293908943, 0.3458507752293908943, -2.576771653543307394 ) ) ;
#29459=CARTESIAN_POINT ( 'NONE',  ( 0.3392501089628018329, 0.1958661417322835607, -1.475721784776902856 ) ) ;
#29464=CARTESIAN_POINT ( 'NONE',  ( -0.3460692066303960313, 0.1998031496062989965, -2.307742782152231165 ) ) ;
#29466=CARTESIAN_POINT ( 'NONE',  ( 0.1070741851644054915, -0.3996062992125986035, -0.8727034120734907807 ) ) ;
#29469=CARTESIAN_POINT ( 'NONE',  ( 0.3917322834645669549, 0.1049643490035304660, -2.321522309711285814 ) ) ;
#29470=ORIENTED_EDGE ( 'NONE', *, *, #78723, .F. ) ;
#29478=CARTESIAN_POINT ( 'NONE',  ( 4.797336870675655290E-17, -0.3917322834645669549, -1.418615854821835276 ) ) ;
#29482=CARTESIAN_POINT ( 'NONE',  ( 0.3392501089628018884, -0.1958661417322834220, 0.06036745406824151755 ) ) ;
#29485=CARTESIAN_POINT ( 'NONE',  ( -0.1058382717557497937, -0.3949938075777411628, 0.08530183727034117147 ) ) ;
#29493=CARTESIAN_POINT ( 'NONE',  ( -0.2867679344610367109, 0.2867679344610365444, -1.433746349902574213 ) ) ;
#29495=CARTESIAN_POINT ( 'NONE',  ( -0.1958661417322834220, -0.3392501089628018884, -2.354986876640420057 ) ) ;
#29500=CARTESIAN_POINT ( 'NONE',  ( 0.1998031496062992740, 0.3460692066303959757, -0.3018372703412073865 ) ) ;
#29502=CARTESIAN_POINT ( 'NONE',  ( -0.3996062992125985480, -7.340648628747423112E-17, 0.1988188976377952832 ) ) ;
#29504=CARTESIAN_POINT ( 'NONE',  ( -0.3460692066303958092, -0.1998031496062994683, -2.099737532808398921 ) ) ;
#29509=CARTESIAN_POINT ( 'NONE',  ( -0.4091458600556402980, -0.2362204724409451284, -0.9166666666666666297 ) ) ;
#29512=CARTESIAN_POINT ( 'NONE',  ( -9.674558042662122972E-17, 0.3949938075777409963, -0.3917322834645669549 ) ) ;
#29521=CARTESIAN_POINT ( 'NONE',  ( -0.4724409448818898682, -8.678599364036362592E-17, -0.1161417322834645827 ) ) ;
#29525=CARTESIAN_POINT ( 'NONE',  ( -0.3996062992125984925, -0.1070741851644056858, -1.540026246719160108 ) ) ;
#29527=CARTESIAN_POINT ( 'NONE',  ( 0.1958661417322834775, 0.3392501089628018884, -0.9238845144356954142 ) ) ;
#29529=CARTESIAN_POINT ( 'NONE',  ( -0.3330030935778838797, 0.2065800153021834507, 1.128668216881735203E-17 ) ) ;
#29537=DIRECTION ( 'NONE',  ( 1.000000000000000000, 8.462065736472229849E-17, -0.000000000000000000 ) ) ;
#29549=CARTESIAN_POINT ( 'NONE',  ( -9.594673741351313045E-17, 0.3917322834645670659, -2.201462885335645048 ) ) ;
#29560=CARTESIAN_POINT ( 'NONE',  ( 0.4091458600556403535, 0.2362204724409449896, 0.02624671916010498651 ) ) ;
#29561=CARTESIAN_POINT ( 'NONE',  ( 0.2891555358219910499, 0.2891555358219910499, -2.185039370078740273 ) ) ;
#29562=ORIENTED_EDGE ( 'NONE', *, *, #10855, .T. ) ;
#29564=CARTESIAN_POINT ( 'NONE',  ( -0.3917322834645671215, 0.1049643490035301469, -0.8123359580052491591 ) ) ;
#29566=CARTESIAN_POINT ( 'NONE',  ( 0.1265901696524990294, -0.4724409448818896462, -2.447506561679789527 ) ) ;
#29567=CARTESIAN_POINT ( 'NONE',  ( 0.3458507752293908943, 0.3458507752293908943, -0.8444881889763780070 ) ) ;
#29573=CARTESIAN_POINT ( 'NONE',  ( 0.3917322834645668994, -0.1049643490035303134, -0.3490620490475572768 ) ) ;
#29579=CARTESIAN_POINT ( 'NONE',  ( -0.3996062992125986035, -7.340648628747425578E-17, -2.874015748031495843 ) ) ;
#29580=CARTESIAN_POINT ( 'NONE',  ( -0.3917322834645671770, 0.1049643490035302024, -1.446869709482626831 ) ) ;
#29586=CARTESIAN_POINT ( 'NONE',  ( 0.1049643490035304938, -0.3917322834645669549, -1.114829396325459410 ) ) ;
#29597=CARTESIAN_POINT ( 'NONE',  ( -0.3917322834645669549, -0.1049643490035306603, -2.557742782152230721 ) ) ;
#29598=ORIENTED_EDGE ( 'NONE', *, *, #4428, .T. ) ;
#29604=CARTESIAN_POINT ( 'NONE',  ( 0.3392501089628018884, -0.1958661417322834220, -0.9770341207349081403 ) ) ;
#29607=EDGE_CURVE ( 'NONE', #10673, #21899, #37105, .T. ) ;
#29608=CARTESIAN_POINT ( 'NONE',  ( -0.1998031496062991630, -0.3460692066303959202, -2.504593175853018661 ) ) ;
#29627=CARTESIAN_POINT ( 'NONE',  ( -0.3392501089628019439, 0.1958661417322832554, -1.523602731462254889 ) ) ;
#29637=CARTESIAN_POINT ( 'NONE',  ( -9.594673741351313045E-17, 0.3917322834645670659, -0.6266597357293457460 ) ) ;
#29640=CARTESIAN_POINT ( 'NONE',  ( -0.4724409448818898682, -8.678599364036362592E-17, -2.163385826771653697 ) ) ;
#29651=CARTESIAN_POINT ( 'NONE',  ( -0.2362204724409451284, 0.4091458600556402425, -2.137139107611548905 ) ) ;
#29660=CARTESIAN_POINT ( 'NONE',  ( -0.3996062992125986590, 0.1070741851644051862, -0.03280839895013124702 ) ) ;
#29661=CARTESIAN_POINT ( 'NONE',  ( -0.1998031496062994405, 0.3460692066303957537, -2.137139107611548905 ) ) ;
#29667=CARTESIAN_POINT ( 'NONE',  ( 0.1070741851644054915, -0.3996062992125986035, -1.817585301837270517 ) ) ;
#29668=CARTESIAN_POINT ( 'NONE',  ( 0.3949938075777409408, 0.1058382717557500574, -1.069553805774278388 ) ) ;
#29669=CARTESIAN_POINT ( 'NONE',  ( 0.3996062992125986035, 2.446882876249141962E-17, -2.480314960629921295 ) ) ;
#29670=CARTESIAN_POINT ( 'NONE',  ( 0.1049643490035304799, -0.3917322834645669549, -0.2349081364829395946 ) ) ;
#29674=CARTESIAN_POINT ( 'NONE',  ( 0.3420746716998660508, -0.1974969037888704149, -2.071522309711286258 ) ) ;
#29678=CARTESIAN_POINT ( 'NONE',  ( 0.4724409448818898682, 2.892866454678787531E-17, -2.322834645669291209 ) ) ;
#29679=CARTESIAN_POINT ( 'NONE',  ( -0.3996062992125987146, 0.1070741851644051862, -1.607611548556430403 ) ) ;
#29686=CARTESIAN_POINT ( 'NONE',  ( -0.3917322834645670659, 0.1049643490035301607, -2.790006930937320995 ) ) ;
#29694=CARTESIAN_POINT ( 'NONE',  ( -0.3917322834645670104, -7.196005306013484475E-17, -0.2814960629921260393 ) ) ;
#29696=CARTESIAN_POINT ( 'NONE',  ( 0.3917322834645670104, -0.1049643490035303411, -2.150918635170603554 ) ) ;
#29699=CARTESIAN_POINT ( 'NONE',  ( 0.3420746716998660508, -0.1974969037888703871, -2.624671916010498318 ) ) ;
#29703=CARTESIAN_POINT ( 'NONE',  ( 0.1998031496062992740, 0.3460692066303959757, -1.089238845144356871 ) ) ;
#29708=CARTESIAN_POINT ( 'NONE',  ( 0.3392501089628018329, 0.1958661417322835607, -0.5308398950131234528 ) ) ;
#29715=CARTESIAN_POINT ( 'NONE',  ( 0.1958661417322836440, -0.3392501089628017219, -0.08398950131233591521 ) ) ;
#29719=CARTESIAN_POINT ( 'NONE',  ( 0.4091458600556403535, 0.2362204724409449896, -1.548556430446194287 ) ) ;
#29721=CARTESIAN_POINT ( 'NONE',  ( -0.3917322834645669549, -0.1049643490035306603, -2.650262467191601079 ) ) ;
#29724=CARTESIAN_POINT ( 'NONE',  ( 0.2362204724409451007, -0.4091458600556402980, -2.296587926509186417 ) ) ;
#29725=CARTESIAN_POINT ( 'NONE',  ( 0.4724409448818898127, -0.1265901696524988629, -2.001312335958005395 ) ) ;
#29728=CARTESIAN_POINT ( 'NONE',  ( -0.3392501089628019439, 0.1958661417322832554, -0.5787208416984759296 ) ) ;
#29730=CARTESIAN_POINT ( 'NONE',  ( -9.594673741351313045E-17, 0.3917322834645670104, -0.2421259842519686289 ) ) ;
#29735=CARTESIAN_POINT ( 'NONE',  ( -0.2867679344610364334, -0.2867679344610367109, -2.413385826771653253 ) ) ;
#29738=CARTESIAN_POINT ( 'NONE',  ( 0.3458507752293908943, -0.3458507752293908943, -0.8051181102362205966 ) ) ;
#29746=CARTESIAN_POINT ( 'NONE',  ( -0.2362204724409451284, 0.4091458600556402425, -0.3280839895013123453 ) ) ;
#29750=CARTESIAN_POINT ( 'NONE',  ( -0.3460692066303960313, 0.1998031496062989965, -1.835301837270341352 ) ) ;
#29758=CARTESIAN_POINT ( 'NONE',  ( -9.787531504996566615E-17, 0.3996062992125985480, -0.07677165354330711677 ) ) ;
#29760=CARTESIAN_POINT ( 'NONE',  ( 4.893765752498283924E-17, -0.3996062992125986035, -0.5511811023622047445 ) ) ;
#29761=CARTESIAN_POINT ( 'NONE',  ( 0.1958661417322836718, -0.3392501089628017219, -2.765767347277902299 ) ) ;
#29767=CARTESIAN_POINT ( 'NONE',  ( -0.1974969037888706924, 0.3420746716998658843, -1.034776902887139194 ) ) ;
#29772=CARTESIAN_POINT ( 'NONE',  ( 0.4724409448818898682, 2.892866454678787531E-17, -1.220472440944881942 ) ) ;
#29773=CARTESIAN_POINT ( 'NONE',  ( 0.3996062992125985480, 0.1070741851644054637, -2.486876640419947382 ) ) ;
#29776=CARTESIAN_POINT ( 'NONE',  ( 0.2867679344610366554, 0.2867679344610366554, -0.6069746963592669298 ) ) ;
#29787=CARTESIAN_POINT ( 'NONE',  ( 0.3917322834645670104, -0.1049643490035303411, -0.8910761154855640909 ) ) ;
#29790=CARTESIAN_POINT ( 'NONE',  ( 0.1974969037888704704, 0.3420746716998660508, -1.404199475065616820 ) ) ;
#29794=CARTESIAN_POINT ( 'NONE',  ( -0.1070741851644051862, -0.3996062992125987146, 0.08530183727034119923 ) ) ;
#29801=CARTESIAN_POINT ( 'NONE',  ( 0.2867679344610365999, -0.2867679344610365444, -0.02559055118110245899 ) ) ;
#29806=CARTESIAN_POINT ( 'NONE',  ( -0.2925321140481932924, 0.2925321140481931814, -2.224409448818897239 ) ) ;
#29809=CARTESIAN_POINT ( 'NONE',  ( 0.1070741851644054776, -0.3996062992125984925, -1.421916010498687877 ) ) ;
#29810=CARTESIAN_POINT ( 'NONE',  ( -0.03178304480585582292, 0.3983403474834776858, -2.755905511811024500 ) ) ;
#29813=CARTESIAN_POINT ( 'NONE',  ( 5.785732909357575061E-17, -0.4724409448818898682, -0.2362204724409449064 ) ) ;
#29815=CARTESIAN_POINT ( 'NONE',  ( 0.3392501089628018329, 0.1958661417322835607, -2.578083989501311901 ) ) ;
#29821=CARTESIAN_POINT ( 'NONE',  ( 0.4724409448818897572, -0.1265901696524988906, -2.393044619422572072 ) ) ;
#29823=CARTESIAN_POINT ( 'NONE',  ( 0.3949938075777408852, 0.1058382717557500435, -1.618766404199474929 ) ) ;
#29833=CARTESIAN_POINT ( 'NONE',  ( 0.3392501089628018329, -0.1958661417322834497, -2.389744463745719916 ) ) ;
#29845=CARTESIAN_POINT ( 'NONE',  ( -0.1070741851644056997, 0.3996062992125984925, -0.7132545931758530466 ) ) ;
#29847=CARTESIAN_POINT ( 'NONE',  ( 0.1958661417322836440, -0.3392501089628017219, -1.908792650918635259 ) ) ;
#29856=CARTESIAN_POINT ( 'NONE',  ( -0.1070741851644056997, 0.3996062992125984925, -1.500656167979002253 ) ) ;
#29864=CARTESIAN_POINT ( 'NONE',  ( 0.3392501089628018884, -0.1958661417322834220, -1.764435695538057791 ) ) ;
#29869=CARTESIAN_POINT ( 'NONE',  ( 0.3460692066303959202, -0.1998031496062991630, -2.229002624671916344 ) ) ;
#29871=CARTESIAN_POINT ( 'NONE',  ( -0.2925321140481932924, 0.2925321140481931814, -0.9645669291338579976 ) ) ;
#29874=CARTESIAN_POINT ( 'NONE',  ( 0.3917322834645669549, 0.1049643490035304660, -2.793963254593175183 ) ) ;
#29884=CARTESIAN_POINT ( 'NONE',  ( -0.2867679344610366554, 0.2867679344610365444, -1.832001681593488751 ) ) ;
#29887=CARTESIAN_POINT ( 'NONE',  ( -0.3392501089628019995, 0.1958661417322832277, 0.1391076115485564701 ) ) ;
#29890=CARTESIAN_POINT ( 'NONE',  ( -0.1058382717557503211, 0.3949938075777409408, -0.006561679790026304741 ) ) ;
#29898=CARTESIAN_POINT ( 'NONE',  ( 0.1049643490035304799, -0.3917322834645670104, -1.184402517881576911 ) ) ;
#29900=CARTESIAN_POINT ( 'NONE',  ( 0.2867679344610365999, -0.2867679344610365444, -2.230314960629921295 ) ) ;
#29905=CARTESIAN_POINT ( 'NONE',  ( -0.1070741851644056997, 0.3996062992125986035, -0.3215223097112860362 ) ) ;
#29907=CARTESIAN_POINT ( 'NONE',  ( 0.3996062992125984925, 0.1070741851644054637, 0.1135170603674540563 ) ) ;
#29909=CARTESIAN_POINT ( 'NONE',  ( 0.3460692066303959757, -0.1998031496062991907, -2.152230971128608950 ) ) ;
#29914=CARTESIAN_POINT ( 'NONE',  ( -0.3458507752293906723, -0.3458507752293910609, -1.238188976377952999 ) ) ;
#29918=CARTESIAN_POINT ( 'NONE',  ( 0.1974969037888704704, 0.3420746716998660508, -0.6935695538057742304 ) ) ;
#29931=CARTESIAN_POINT ( 'NONE',  ( 0.2925321140481932369, -0.2925321140481931814, -1.592519685039370358 ) ) ;
#29933=CARTESIAN_POINT ( 'NONE',  ( 0.3917322834645670104, -0.1049643490035303411, -1.678477690288713964 ) ) ;
#29956=CARTESIAN_POINT ( 'NONE',  ( -0.3392501089628019995, 0.1958661417322831999, -2.227709604495750284 ) ) ;
#29964=CARTESIAN_POINT ( 'NONE',  ( -0.3917322834645671215, 0.1049643490035301469, -2.229658792650918819 ) ) ;
#29967=CARTESIAN_POINT ( 'NONE',  ( -0.3458507752293906723, -0.3458507752293910609, -0.05905511811023620578 ) ) ;
#29968=CARTESIAN_POINT ( 'NONE',  ( -0.1974969037888703871, -0.3420746716998661063, -2.742782152230970993 ) ) ;
#29972=CARTESIAN_POINT ( 'NONE',  ( -0.2867679344610365999, 0.2867679344610364889, -1.429133858267716661 ) ) ;
#29974=CARTESIAN_POINT ( 'NONE',  ( 0.4091458600556404646, -0.2362204724409448231, -2.624671916010498762 ) ) ;
#29981=CARTESIAN_POINT ( 'NONE',  ( 0.1958661417322834497, 0.3392501089628018329, -0.2243901330370585701 ) ) ;
#29989=CARTESIAN_POINT ( 'NONE',  ( -0.2867679344610367109, 0.2867679344610365444, -1.591226664863204077 ) ) ;
#29995=CARTESIAN_POINT ( 'NONE',  ( 0.1049643490035303689, 0.3917322834645670104, -1.022965879265091749 ) ) ;
#30013=CARTESIAN_POINT ( 'NONE',  ( -0.3917322834645671215, 0.1049643490035301469, -0.7473753280839893209 ) ) ;
#30016=CARTESIAN_POINT ( 'NONE',  ( -0.2925321140481932369, 0.2925321140481931259, -2.458661417322834719 ) ) ;
#30027=CARTESIAN_POINT ( 'NONE',  ( 0.1998031496062992463, 0.3460692066303959202, -0.6935695538057742304 ) ) ;
#30029=CARTESIAN_POINT ( 'NONE',  ( 0.4724409448818898682, 2.892866454678787531E-17, -2.084645669291338432 ) ) ;
#30036=CARTESIAN_POINT ( 'NONE',  ( -0.1049643490035306742, 0.3917322834645668994, -1.818878322013436355 ) ) ;
#30046=CARTESIAN_POINT ( 'NONE',  ( 0.3917322834645670659, -0.1049643490035303273, -0.4232476622385321074 ) ) ;
#30050=CARTESIAN_POINT ( 'NONE',  ( 0.3458507752293908943, 0.3458507752293908943, -2.104330708661417138 ) ) ;
#30062=CARTESIAN_POINT ( 'NONE',  ( -0.4724409448818898682, -8.678599364036362592E-17, -2.163385826771653697 ) ) ;
#30072=CARTESIAN_POINT ( 'NONE',  ( 0.1070741851644053388, 0.3996062992125986035, -2.117454068241469756 ) ) ;
#30077=CARTESIAN_POINT ( 'NONE',  ( -0.3460692066303958092, -0.1998031496062994683, -1.784776902887138972 ) ) ;
#30078=CARTESIAN_POINT ( 'NONE',  ( 0.2891555358219910499, -0.2891555358219909944, -1.515748031496063186 ) ) ;
#30079=CARTESIAN_POINT ( 'NONE',  ( -0.3996062992125986035, -0.1070741851644056997, -2.408136482939632561 ) ) ;
#30082=CARTESIAN_POINT ( 'NONE',  ( 0.3917322834645669549, 0.1049643490035304660, -0.5892388451443569819 ) ) ;
#30086=CARTESIAN_POINT ( 'NONE',  ( -0.1974969037888706924, 0.3420746716998658843, -2.137139107611548905 ) ) ;
#30089=CARTESIAN_POINT ( 'NONE',  ( -0.1265901696524986964, -0.4724409448818899238, -2.591863517060367439 ) ) ;
#30090=CARTESIAN_POINT ( 'NONE',  ( -9.787531504996567848E-17, 0.3996062992125986035, -1.574803149606299302 ) ) ;
#30098=CARTESIAN_POINT ( 'NONE',  ( -0.3917322834645670104, -7.196005306013484475E-17, 0.1909448818897636901 ) ) ;
#30105=CARTESIAN_POINT ( 'NONE',  ( 0.3917322834645669549, 0.1049643490035304660, -0.2093175853018373611 ) ) ;
#30107=CARTESIAN_POINT ( 'NONE',  ( 0.3392501089628018329, 0.1958661417322835607, -2.485564304461941987 ) ) ;
#30110=CARTESIAN_POINT ( 'NONE',  ( -0.1974969037888703871, -0.3420746716998661063, -2.900262467191600635 ) ) ;
#30114=CARTESIAN_POINT ( 'NONE',  ( -9.787531504996567848E-17, 0.3996062992125986035, -1.102362204724409489 ) ) ;
#30119=CARTESIAN_POINT ( 'NONE',  ( 0.2867679344610365999, 0.2867679344610365999, -0.2224409448818898127 ) ) ;
#30125=CARTESIAN_POINT ( 'NONE',  ( 0.3917322834645669549, 0.1049643490035304660, -0.1167979002624671692 ) ) ;
#30129=CARTESIAN_POINT ( 'NONE',  ( -0.4724409448818898682, -8.678599364036362592E-17, -1.614173228346456712 ) ) ;
#30131=CARTESIAN_POINT ( 'NONE',  ( 4.797336870675656522E-17, -0.3917322834645670104, -2.683070866141731958 ) ) ;
#30135=CARTESIAN_POINT ( 'NONE',  ( 5.785732909357575061E-17, -0.4724409448818898682, -1.968503937007873850 ) ) ;
#30139=CARTESIAN_POINT ( 'NONE',  ( 0.1049643490035303689, 0.3917322834645668994, -0.3884321277877147427 ) ) ;
#30141=CARTESIAN_POINT ( 'NONE',  ( 0.1049643490035303689, 0.3917322834645670104, -0.3930446194225722945 ) ) ;
#30148=CARTESIAN_POINT ( 'NONE',  ( -0.3917322834645671215, 0.1049643490035301469, -2.544619422572177658 ) ) ;
#30151=CARTESIAN_POINT ( 'NONE',  ( 0.1265901696524989462, 0.4724409448818897572, -0.8576115485564304031 ) ) ;
#30162=CARTESIAN_POINT ( 'NONE',  ( -0.1998031496062994405, 0.3460692066303957537, -1.822178477690288512 ) ) ;
#30170=CARTESIAN_POINT ( 'NONE',  ( 0.3996062992125985480, -0.1070741851644052972, -0.1883202099737532609 ) ) ;
#30171=CARTESIAN_POINT ( 'NONE',  ( 0.3996062992125986035, 2.446882876249141962E-17, -0.5905511811023621549 ) ) ;
#30172=CARTESIAN_POINT ( 'NONE',  ( 0.3949938075777409408, 0.1058382717557500574, 0.03280839895013118457 ) ) ;
#30178=CARTESIAN_POINT ( 'NONE',  ( 0.2891555358219910499, 0.2891555358219910499, -1.001968503937007871 ) ) ;
#30183=CARTESIAN_POINT ( 'NONE',  ( 5.785732909357575061E-17, -0.4724409448818898682, -1.181102362204724310 ) ) ;
#30184=CARTESIAN_POINT ( 'NONE',  ( 0.2925321140481932369, -0.2925321140481931814, -2.303149606299212060 ) ) ;
#30187=CARTESIAN_POINT ( 'NONE',  ( -0.3917322834645670659, -7.196005306013484475E-17, -0.8235101294301331309 ) ) ;
#30199=CARTESIAN_POINT ( 'NONE',  ( -0.3917322834645669549, -0.1049643490035306603, -1.140419947506561282 ) ) ;
#30202=CARTESIAN_POINT ( 'NONE',  ( -0.1058382717557503211, 0.3949938075777409408, -1.423884514435695969 ) ) ;
#30214=CARTESIAN_POINT ( 'NONE',  ( 0.1049643490035303689, 0.3917322834645670104, -0.07808398950131241467 ) ) ;
#30220=CARTESIAN_POINT ( 'NONE',  ( -0.1998031496062991907, -0.3460692066303959757, -1.955380577427821454 ) ) ;
#30223=CARTESIAN_POINT ( 'NONE',  ( 0.2925321140481932369, 0.2925321140481932369, -1.474409448818897683 ) ) ;
#30227=CARTESIAN_POINT ( 'NONE',  ( 5.785732909357575061E-17, -0.4724409448818898682, -0.5511811023622047445 ) ) ;
#30230=CARTESIAN_POINT ( 'NONE',  ( -9.594673741351313045E-17, 0.3917322834645670104, -2.761811023622046779 ) ) ;
#30236=CARTESIAN_POINT ( 'NONE',  ( 0.4091458600556404646, -0.2362204724409448231, -2.229002624671915900 ) ) ;
#30239=CARTESIAN_POINT ( 'NONE',  ( 0.1974969037888706092, -0.3420746716998660508, -2.058398950131233640 ) ) ;
#30259=CARTESIAN_POINT ( 'NONE',  ( -0.3996062992125985480, -7.340648628747423112E-17, -0.9035433070866141225 ) ) ;
#30260=CARTESIAN_POINT ( 'NONE',  ( -0.2867679344610364334, -0.2867679344610367109, -2.190944881889763440 ) ) ;
#30271=CARTESIAN_POINT ( 'NONE',  ( 0.4724409448818914781, 0.1265901696524960318, -2.171916010498687655 ) ) ;
#30277=CARTESIAN_POINT ( 'NONE',  ( 0.2867679344610365999, -0.2867679344610365444, -1.600393700787401619 ) ) ;
#30282=CARTESIAN_POINT ( 'NONE',  ( 0.3996062992125984925, 0.1070741851644054499, -2.406167979002624246 ) ) ;
#30284=CARTESIAN_POINT ( 'NONE',  ( 0.2925321140481932369, -0.2925321140481932369, -0.7283464566929134243 ) ) ;
#30287=CARTESIAN_POINT ( 'NONE',  ( -0.1049643490035307020, 0.3917322834645669549, -2.675853018372703396 ) ) ;
#30297=CARTESIAN_POINT ( 'NONE',  ( -0.1958661417322836440, 0.3392501089628016664, -1.982920316764092306 ) ) ;
#30300=CARTESIAN_POINT ( 'NONE',  ( 0.2867679344610365999, 0.2867679344610365999, 0.02755905511811028441 ) ) ;
#30303=CARTESIAN_POINT ( 'NONE',  ( -0.1974969037888706647, 0.3420746716998658843, -0.3280839895013124563 ) ) ;
#30311=CARTESIAN_POINT ( 'NONE',  ( 0.3917322834645670659, 2.398668435337828261E-17, -1.059730601871078148 ) ) ;
#30313=CARTESIAN_POINT ( 'NONE',  ( -0.3917322834645669549, -0.1049643490035306603, -2.807742782152229832 ) ) ;
#30318=CARTESIAN_POINT ( 'NONE',  ( 0.2925321140481932369, 0.2925321140481932369, -0.7677165354330709457 ) ) ;
#30320=CARTESIAN_POINT ( 'NONE',  ( 0.1070741851644054776, -0.3996062992125984925, -0.1620734908136483021 ) ) ;
#30322=CARTESIAN_POINT ( 'NONE',  ( -0.3996062992125986035, -7.340648628747425578E-17, -2.244094488188976388 ) ) ;
#30328=CARTESIAN_POINT ( 'NONE',  ( -0.4091458600556402980, -0.2362204724409451284, -1.074146981627296604 ) ) ;
#30332=CARTESIAN_POINT ( 'NONE',  ( 4.837279021331061486E-17, -0.3949938075777409963, -0.7854330708661416693 ) ) ;
#30344=CARTESIAN_POINT ( 'NONE',  ( 0.3996062992125986035, -0.1070741851644052972, -1.763123359580052174 ) ) ;
#30346=CARTESIAN_POINT ( 'NONE',  ( -0.3392501089628017219, -0.1958661417322836718, -1.461942257217847763 ) ) ;
#30359=CARTESIAN_POINT ( 'NONE',  ( 0.3392501089628018329, 0.1958661417322835607, -0.8458005249343831800 ) ) ;
#30377=CARTESIAN_POINT ( 'NONE',  ( 0.3996062992125986035, 2.446882876249141962E-17, -1.220472440944881942 ) ) ;
#30379=CARTESIAN_POINT ( 'NONE',  ( 0.3392501089628018884, -0.1958661417322834220, -1.986876640419947604 ) ) ;
#30383=CARTESIAN_POINT ( 'NONE',  ( 0.2362204724409451007, -0.4091458600556402980, -0.4068241469816273326 ) ) ;
#30384=CARTESIAN_POINT ( 'NONE',  ( 4.837279021331060870E-17, -0.3949938075777409963, -2.913385826771653253 ) ) ;
#30385=ORIENTED_EDGE ( 'NONE', *, *, #55825, .T. ) ;
#30387=CARTESIAN_POINT ( 'NONE',  ( -0.1958661417322836718, 0.3392501089628017219, -1.265091863517060489 ) ) ;
#30389=CARTESIAN_POINT ( 'NONE',  ( 0.3458507752293908943, 0.3458507752293908943, -2.657480314960630530 ) ) ;
#30395=CARTESIAN_POINT ( 'NONE',  ( -0.2867679344610364334, -0.2867679344610368219, -0.6115292406486071419 ) ) ;
#30404=CARTESIAN_POINT ( 'NONE',  ( 0.2867679344610366554, -0.2867679344610365999, -2.142407767225408932 ) ) ;
#30411=CARTESIAN_POINT ( 'NONE',  ( 0.3392501089628018884, -0.1958661417322834220, -1.449475065616798064 ) ) ;
#30421=CARTESIAN_POINT ( 'NONE',  ( 4.797336870675656522E-17, -0.3917322834645670104, -2.590551181102362044 ) ) ;
#30422=ORIENTED_EDGE ( 'NONE', *, *, #14203, .F. ) ;
#30431=CARTESIAN_POINT ( 'NONE',  ( -9.594673741351313045E-17, 0.3917322834645670104, -0.7145669291338584417 ) ) ;
#30432=CARTESIAN_POINT ( 'NONE',  ( -0.2362204724409447953, -0.4091458600556404646, 0.1725721784776902690 ) ) ;
#30434=CARTESIAN_POINT ( 'NONE',  ( -0.3460692066303960313, 0.1998031496062989965, -2.307742782152230721 ) ) ;
#30443=CARTESIAN_POINT ( 'NONE',  ( -0.3460692066303957537, -0.1998031496062994405, -0.6017060367454067915 ) ) ;
#30445=CARTESIAN_POINT ( 'NONE',  ( -0.3917322834645669549, -0.1049643490035306603, -0.03805774278215218187 ) ) ;
#30453=CARTESIAN_POINT ( 'NONE',  ( -9.594673741351310580E-17, 0.3917322834645669549, -1.497356012302150763 ) ) ;
#30463=CARTESIAN_POINT ( 'NONE',  ( 0.1958661417322836718, -0.3392501089628017219, -0.8760035677503431595 ) ) ;
#30467=CARTESIAN_POINT ( 'NONE',  ( 0.4724409448818896462, 0.1265901696524990294, -2.248687664041994605 ) ) ;
#30478=DIRECTION ( 'NONE',  ( 0.000000000000000000, 0.000000000000000000, 1.000000000000000000 ) ) ;
#30487=CARTESIAN_POINT ( 'NONE',  ( 0.3996062992125986035, -0.1070741851644053111, -0.1115485564304461857 ) ) ;
#30488=CARTESIAN_POINT ( 'NONE',  ( 0.2925321140481932369, 0.2925321140481932369, -2.734251968503936148 ) ) ;
#30495=CARTESIAN_POINT ( 'NONE',  ( 0.3996062992125986590, -0.1070741851644053111, -2.001312335958005395 ) ) ;
#30496=CARTESIAN_POINT ( 'NONE',  ( -0.1974969037888703871, -0.3420746716998661063, -1.482939632545931863 ) ) ;
#30499=CARTESIAN_POINT ( 'NONE',  ( -0.2867679344610366554, 0.2867679344610365444, -0.7992125984251967630 ) ) ;
#30504=CARTESIAN_POINT ( 'NONE',  ( -0.3949938075777411073, 0.1058382717557497660, -2.629265091863516979 ) ) ;
#30508=CARTESIAN_POINT ( 'NONE',  ( -0.4091458600556402980, -0.2362204724409451284, -2.572178477690288734 ) ) ;
#30509=CARTESIAN_POINT ( 'NONE',  ( -0.1070741851644051862, -0.3996062992125987146, -2.276902887139107268 ) ) ;
#30516=CARTESIAN_POINT ( 'NONE',  ( 0.3917322834645669549, 2.398668435337827645E-17, -2.875308768207662347 ) ) ;
#30523=CARTESIAN_POINT ( 'NONE',  ( 0.1049643490035304938, -0.3917322834645669549, -0.3274278215223098143 ) ) ;
#30524=CARTESIAN_POINT ( 'NONE',  ( -0.1049643490035302024, -0.3917322834645671215, -1.324146981627296826 ) ) ;
#30525=CARTESIAN_POINT ( 'NONE',  ( -0.1958661417322836718, 0.3392501089628017219, -2.367454068241469756 ) ) ;
#30528=CARTESIAN_POINT ( 'NONE',  ( 0.3949938075777411073, -0.1058382717557499464, -2.788713910761155379 ) ) ;
#30532=CARTESIAN_POINT ( 'NONE',  ( 0.1998031496062994405, -0.3460692066303958092, -1.509186351706036655 ) ) ;
#30535=CYLINDRICAL_SURFACE ( 'NONE', #70517, 0.4724409448818898682 ) ;
#30537=CARTESIAN_POINT ( 'NONE',  ( -0.1049643490035307020, 0.3917322834645669549, -0.2486876640419948270 ) ) ;
#30542=CARTESIAN_POINT ( 'NONE',  ( -9.594673741351313045E-17, 0.3917322834645670104, -0.1496062992125983815 ) ) ;
#30547=CARTESIAN_POINT ( 'NONE',  ( -0.4724409448818895907, -0.1265901696524993070, -1.778215223097112663 ) ) ;
#30559=CARTESIAN_POINT ( 'NONE',  ( -0.2867679344610364334, -0.2867679344610368219, -0.4540489256879772784 ) ) ;
#30561=CARTESIAN_POINT ( 'NONE',  ( 0.3917322834645669549, 0.1049643490035304660, -0.9967191601049869565 ) ) ;
#30567=CARTESIAN_POINT ( 'NONE',  ( 0.1049643490035303689, 0.3917322834645670104, -2.190288713910760521 ) ) ;
#30570=CARTESIAN_POINT ( 'NONE',  ( -0.4724409448818898682, -8.678599364036362592E-17, -0.5885826771653542844 ) ) ;
#30581=CARTESIAN_POINT ( 'NONE',  ( 0.3996062992125984925, 0.1070741851644054637, -1.933727034120735100 ) ) ;
#30589=CARTESIAN_POINT ( 'NONE',  ( -0.2925321140481930149, -0.2925321140481933480, -0.6082677165354329896 ) ) ;
#30590=CARTESIAN_POINT ( 'NONE',  ( -9.787531504996567848E-17, 0.3996062992125986035, -0.3149606299212598381 ) ) ;
#30591=CARTESIAN_POINT ( 'NONE',  ( -9.674558042662121740E-17, 0.3949938075777409963, -0.3149606299212598937 ) ) ;
#30597=CARTESIAN_POINT ( 'NONE',  ( -0.1058382717557497660, -0.3949938075777411073, -0.9363517060367456679 ) ) ;
#30602=CARTESIAN_POINT ( 'NONE',  ( 0.4724409448818897572, -0.1265901696524988906, -1.371391076115485053 ) ) ;
#30604=CARTESIAN_POINT ( 'NONE',  ( 0.1998031496062994405, -0.3460692066303958092, -2.296587926509186417 ) ) ;
#30608=CARTESIAN_POINT ( 'NONE',  ( -0.3917322834645671770, 0.1049643490035302024, -0.8169484496401069329 ) ) ;
#30619=CARTESIAN_POINT ( 'NONE',  ( 0.3917322834645670104, -0.1049643490035303411, -1.206036745406823707 ) ) ;
#30622=CARTESIAN_POINT ( 'NONE',  ( -0.1974969037888703871, -0.3420746716998661063, -1.325459317585301777 ) ) ;
#30623=ORIENTED_EDGE ( 'NONE', *, *, #16700, .F. ) ;
#30634=CARTESIAN_POINT ( 'NONE',  ( 0.1958661417322834775, 0.3392501089628018884, -0.07152230971128617498 ) ) ;
#30640=CARTESIAN_POINT ( 'NONE',  ( -0.1998031496062994683, 0.3460692066303958092, -2.217847769028871596 ) ) ;
#30643=CARTESIAN_POINT ( 'NONE',  ( -0.3460692066303957537, -0.1998031496062994405, -1.389107611548556553 ) ) ;
#30644=CARTESIAN_POINT ( 'NONE',  ( -0.02963302784744966181, 0.3970677821444046907, -2.755905511811023612 ) ) ;
#30647=CARTESIAN_POINT ( 'NONE',  ( -0.1265901696524993347, 0.4724409448818895907, -0.3215223097112860362 ) ) ;
#30650=CARTESIAN_POINT ( 'NONE',  ( -0.2867679344610365999, 0.2867679344610364889, 0.1456692913385827237 ) ) ;
#30656=CARTESIAN_POINT ( 'NONE',  ( 0.3458507752293908943, -0.3458507752293908943, -2.537401574803149984 ) ) ;
#30659=CARTESIAN_POINT ( 'NONE',  ( 0.1058382717557499880, 0.3949938075777409408, -2.274934383202099841 ) ) ;
#30672=LINE ( 'NONE', #37803, #22446 ) ;
#30682=CARTESIAN_POINT ( 'NONE',  ( -0.1070741851644051862, -0.3996062992125986590, -0.6213910761154856077 ) ) ;
#30683=CARTESIAN_POINT ( 'NONE',  ( 0.2867679344610365999, -0.2867679344610365444, -2.387795275590551380 ) ) ;
#30692=CARTESIAN_POINT ( 'NONE',  ( 0.4091458600556403535, 0.2362204724409449896, -2.178477690288713742 ) ) ;
#30698=CARTESIAN_POINT ( 'NONE',  ( 4.797336870675656522E-17, -0.3917322834645670104, -1.580708661417322913 ) ) ;
#30699=CARTESIAN_POINT ( 'NONE',  ( -0.2643935821217223148, 0.2898214735618642734, -1.220472440944881498 ) ) ;
#30703=CARTESIAN_POINT ( 'NONE',  ( 4.893765752498283308E-17, -0.3996062992125985480, -2.517716535433071279 ) ) ;
#30706=CARTESIAN_POINT ( 'NONE',  ( 0.3996062992125986035, 2.446882876249141962E-17, -1.062992125984252079 ) ) ;
#30709=CARTESIAN_POINT ( 'NONE',  ( -0.3917322834645670104, -7.196005306013484475E-17, -2.708661417322834275 ) ) ;
#30721=( BOUNDED_CURVE ( )  B_SPLINE_CURVE ( 2, ( #28537, #40751, #34445, #65619, #65193, #46225, #1631, #21806, #47470, #54194, #78242, #27290, #14686, #66435, #2465, #71921, #28123, #20983, #53778, #59275, #79910, #47882, #14271, #79491, #52948, #39505, #78662, #40343, #67269, #23047, #55434, #60935, #68907, #80326, #56269, #41987, #36096, #48300, #23874, #4936, #81965, #74829, #9602, #68501, #49123, #61767, #74412, #54615, #16344, #4515, #10440, #15932, #81143, #10017, #3285, #28950, #30604, #30184, #62177, #16756, #22640, #35270, #73997, #67681, #49540, #23458, #10841, #35682, #41579, #61348, #3702, #81555, #75235, #62593, #29365, #55025, #42395, #17174, #42807, #80733, #4107, #17578, #48714, #68094, #36501, #29773, #55846, #43211, #24280, #11259, #49951, #36917, #11677, #12487, #37738, #64247, #12907, #50360, #63412, #12080, #25512, #24692, #277, #64661, #32667, #50772, #19623, #38978, #82777, #25932, #31837, #76472, #76057, #5346, #77292, #5747, #6162, #63007, #25099, #75649, #18799, #6581, #38566, #44443, #31005, #45285, #17989 ),
 .UNSPECIFIED., .F., .F. ) 
 B_SPLINE_CURVE_WITH_KNOTS ( ( 3, 2, 2, 2, 2, 2, 2, 2, 2, 2, 2, 2, 2, 2, 2, 2, 2, 2, 2, 2, 2, 2, 2, 2, 2, 2, 2, 2, 2, 2, 2, 2, 2, 2, 2, 2, 2, 2, 2, 2, 2, 2, 2, 2, 2, 2, 2, 2, 2, 2, 2, 2, 2, 2, 2, 2, 2, 2, 2, 2, 2, 2, 2, 3 ),
 ( 0.6625000000000256239, 0.6666666666666918317, 0.6708333333333581505, 0.6750000000000244693, 0.6791666666666906771, 0.6833333333333569959, 0.6875000000000232037, 0.6916666666666894114, 0.6958333333333557302, 0.7000000000000219380, 0.7041666666666882568, 0.7083333333333545756, 0.7125000000000207834, 0.7166666666666869911, 0.7208333333333533099, 0.7250000000000195177, 0.7291666666666857255, 0.7333333333333520443, 0.7375000000000183631, 0.7416666666666845709, 0.7458333333333508897, 0.7500000000000170974, 0.7541666666666833052, 0.7583333333333496240, 0.7625000000000158318, 0.7666666666666821506, 0.7708333333333484694, 0.7750000000000146771, 0.7791666666666808849, 0.7833333333333472037, 0.7875000000000134115, 0.7916666666666796193, 0.7958333333333459381, 0.8000000000000122569, 0.8041666666666784646, 0.8083333333333446724, 0.8125000000000109912, 0.8166666666666771990, 0.8208333333333435178, 0.8250000000000097256, 0.8291666666666761554, 0.8333333333333423631, 0.8375000000000085709, 0.8416666666666747787, 0.8458333333333410975, 0.8500000000000073053, 0.8541666666666735130, 0.8583333333333398318, 0.8625000000000061506, 0.8666666666666723584, 0.8708333333333386772, 0.8750000000000048850, 0.8791666666666710928, 0.8833333333333374116, 0.8875000000000036193, 0.8916666666666699381, 0.8958333333333361459, 0.9000000000000024647, 0.9041666666666687835, 0.9083333333333349913, 0.9125000000000011990, 0.9166666666666674068, 0.9208333333333336146, 0.9250000000000000444 ),
 .UNSPECIFIED. ) 
 CURVE ( )  GEOMETRIC_REPRESENTATION_ITEM ( )  RATIONAL_B_SPLINE_CURVE ( ( 0.9999999999997902789, 0.9659258262892780333, 1.000000000000000000, 0.9659258262890683122, 1.000000000000000000, 0.9659258262890683122, 1.000000000000000000, 0.9659258262890683122, 1.000000000000000000, 0.9659258262890683122, 1.000000000000000000, 0.9659258262890683122, 1.000000000000000000, 0.9659258262890683122, 1.000000000000000000, 0.9659258262890683122, 1.000000000000000000, 0.9659258262890683122, 1.000000000000000000, 0.9659258262890683122, 1.000000000000000000, 0.9659258262890683122, 1.000000000000000000, 0.9659258262890683122, 1.000000000000000000, 0.9659258262890683122, 1.000000000000000000, 0.9659258262890683122, 1.000000000000000000, 0.9659258262890683122, 1.000000000000000000, 0.9659258262890683122, 1.000000000000000000, 0.9659258262890683122, 1.000000000000000000, 0.9659258262890683122, 1.000000000000000000, 0.9659258262890683122, 1.000000000000000000, 0.9659258262890683122, 1.000000000000000000, 0.9659258262890683122, 1.000000000000000000, 0.9659258262890683122, 1.000000000000000000, 0.9659258262890683122, 1.000000000000000000, 0.9659258262890683122, 1.000000000000000000, 0.9659258262890683122, 1.000000000000000000, 0.9659258262890683122, 1.000000000000000000, 0.9659258262890683122, 1.000000000000000000, 0.9659258262890683122, 1.000000000000000000, 0.9659258262890683122, 1.000000000000000000, 0.9659258262890683122, 1.000000000000000000, 0.9659258262890683122, 1.000000000000000000, 0.9659258262890683122, 1.000000000000000000, 0.9659258262890683122, 1.000000000000000000, 0.9659258262890683122, 1.000000000000000000, 0.9659258262890683122, 1.000000000000000000, 0.9659258262890683122, 1.000000000000000000, 0.9659258262890683122, 1.000000000000000000, 0.9659258262890683122, 1.000000000000000000, 0.9659258262890683122, 1.000000000000000000, 0.9659258262890683122, 1.000000000000000000, 0.9659258262890683122, 1.000000000000000000, 0.9659258262890683122, 1.000000000000000000, 0.9659258262890683122, 1.000000000000000000, 0.9659258262890683122, 1.000000000000000000, 0.9659258262890683122, 1.000000000000000000, 0.9659258262890683122, 1.000000000000000000, 0.9659258262890683122, 1.000000000000000000, 0.9659258262890683122, 1.000000000000000000, 0.9659258262890683122, 1.000000000000000000, 0.9659258262890683122, 1.000000000000000000, 0.9659258262890683122, 1.000000000000000000, 0.9659258262890683122, 1.000000000000000000, 0.9659258262890683122, 1.000000000000000000, 0.9659258262890683122, 1.000000000000000000, 0.9659258262890683122, 1.000000000000000000, 0.9659258262890683122, 1.000000000000000000, 0.9659258262890683122, 1.000000000000000000, 0.9659258262890683122, 1.000000000000000000, 0.9659258262890683122, 1.000000000000000000, 0.9659258262890683122, 1.000000000000000000, 0.9659258262890683122, 1.000000000000000000, 0.9659258262890683122, 1.000000000000000000, 0.9659258262890683122, 1.000000000000000000 ) ) 
 REPRESENTATION_ITEM ( '' )  );
#30722=CARTESIAN_POINT ( 'NONE',  ( -0.3917322834645669549, -0.1049643490035306603, -2.807742782152229832 ) ) ;
#30725=CARTESIAN_POINT ( 'NONE',  ( -0.3949938075777409408, -0.1058382717557502933, -0.3608923884514436686 ) ) ;
#30732=CARTESIAN_POINT ( 'NONE',  ( 0.1958661417322836718, -0.3392501089628017219, -1.505924827592862503 ) ) ;
#30734=CARTESIAN_POINT ( 'NONE',  ( 4.797336870675656522E-17, -0.3917322834645670104, -2.525590551181102317 ) ) ;
#30739=CARTESIAN_POINT ( 'NONE',  ( -0.2925321140481930704, -0.2925321140481933480, -0.6889763779527556808 ) ) ;
#30741=CARTESIAN_POINT ( 'NONE',  ( -0.3460692066303960313, 0.1998031496062989965, -0.4179790026246719137 ) ) ;
#30743=CARTESIAN_POINT ( 'NONE',  ( 0.1070741851644054915, -0.3996062992125986035, -2.290026246719159442 ) ) ;
#30744=CARTESIAN_POINT ( 'NONE',  ( 0.3917322834645670104, 2.398668435337828261E-17, -1.777559055118110409 ) ) ;
#30748=CARTESIAN_POINT ( 'NONE',  ( 0.4091458600556403535, 0.2362204724409449896, -0.9954068241469815614 ) ) ;
#30751=CARTESIAN_POINT ( 'NONE',  ( -0.3949938075777409963, -7.255918531996591613E-17, -1.061023622047243986 ) ) ;
#30763=CARTESIAN_POINT ( 'NONE',  ( 0.1070741851644053388, 0.3996062992125986035, -1.645013123359579943 ) ) ;
#30777=CARTESIAN_POINT ( 'NONE',  ( 0.3917322834645670104, -0.1049643490035303411, -0.9835958005249345604 ) ) ;
#30791=CARTESIAN_POINT ( 'NONE',  ( 4.893765752498283924E-17, -0.3996062992125986035, -1.023622047244094446 ) ) ;
#30793=DIRECTION ( 'NONE',  ( 0.000000000000000000, 0.000000000000000000, 1.000000000000000000 ) ) ;
#30796=CARTESIAN_POINT ( 'NONE',  ( 0.4724409448818896462, 0.1265901696524990294, -0.2821522309711286258 ) ) ;
#30797=EDGE_CURVE ( 'NONE', #49144, #45904, #22034, .T. ) ;
#30798=CARTESIAN_POINT ( 'NONE',  ( -0.2891555358219908833, -0.2891555358219912164, -2.736220472440944462 ) ) ;
#30801=CARTESIAN_POINT ( 'NONE',  ( 0.3392501089628018329, 0.1958661417322835607, -1.383202099737532942 ) ) ;
#30803=CARTESIAN_POINT ( 'NONE',  ( 0.2362204724409451007, -0.4091458600556402980, -2.296587926509186417 ) ) ;
#30804=CARTESIAN_POINT ( 'NONE',  ( -0.4724409448818898682, -8.678599364036362592E-17, -0.9035433070866141225 ) ) ;
#30809=CARTESIAN_POINT ( 'NONE',  ( 0.3392501089628018329, 0.1958661417322835052, -0.5262274033782657900 ) ) ;
#30816=CARTESIAN_POINT ( 'NONE',  ( -0.1958661417322833942, -0.3392501089628018884, -1.952119053314647523 ) ) ;
#30824=CARTESIAN_POINT ( 'NONE',  ( -0.2867679344610364334, -0.2867679344610367109, -1.403543307086614123 ) ) ;
#30833=CARTESIAN_POINT ( 'NONE',  ( -0.3392501089628019995, 0.1958661417322832277, -2.853018372703412187 ) ) ;
#30840=CARTESIAN_POINT ( 'NONE',  ( -0.3392501089628017219, -0.1958661417322836718, -1.082020997375328086 ) ) ;
#30843=CARTESIAN_POINT ( 'NONE',  ( -0.1974969037888706924, 0.3420746716998658843, 0.2250656167979003253 ) ) ;
#30853=CARTESIAN_POINT ( 'NONE',  ( 0.2925321140481932369, -0.2925321140481931814, -0.4901574803149606474 ) ) ;
#30855=CARTESIAN_POINT ( 'NONE',  ( -0.1958661417322836718, 0.3392501089628017219, -0.1627296587926508609 ) ) ;
#30870=CARTESIAN_POINT ( 'NONE',  ( -0.3917322834645671770, 0.1049643490035302024, -0.9744287646007369075 ) ) ;
#30874=CARTESIAN_POINT ( 'NONE',  ( -0.4091458600556405756, 0.2362204724409446288, -1.835301837270341352 ) ) ;
#30894=CARTESIAN_POINT ( 'NONE',  ( -0.1998031496062991630, -0.3460692066303959202, -2.504593175853018661 ) ) ;
#30899=CARTESIAN_POINT ( 'NONE',  ( 0.2925321140481932369, -0.2925321140481932369, -2.145669291338581974 ) ) ;
#30900=CARTESIAN_POINT ( 'NONE',  ( 0.2891555358219910499, -0.2891555358219909944, -1.673228346456693272 ) ) ;
#30901=CARTESIAN_POINT ( 'NONE',  ( -0.2925321140481932924, 0.2925321140481931814, -2.696850393700787052 ) ) ;
#30903=CARTESIAN_POINT ( 'NONE',  ( 0.3392501089628018329, 0.1958661417322835607, -0.4383202099737532609 ) ) ;
#30907=CARTESIAN_POINT ( 'NONE',  ( -0.1974969037888706924, 0.3420746716998658843, -2.767060367454068803 ) ) ;
#30912=CARTESIAN_POINT ( 'NONE',  ( -0.1998031496062991907, -0.3460692066303959757, -2.270341207349081181 ) ) ;
#30919=CARTESIAN_POINT ( 'NONE',  ( 0.3917322834645669549, 0.1049643490035304660, -0.05183727034120744204 ) ) ;
#30920=CARTESIAN_POINT ( 'NONE',  ( -0.4724409448818898682, -8.678599364036362592E-17, -0.9842519685039369248 ) ) ;
#30926=CARTESIAN_POINT ( 'NONE',  ( 0.1958661417322834775, 0.3392501089628018884, -0.5439632545931759600 ) ) ;
#30927=CARTESIAN_POINT ( 'NONE',  ( -9.594673741351313045E-17, 0.3917322834645670104, -1.566929133858267820 ) ) ;
#30928=CARTESIAN_POINT ( 'NONE',  ( -0.3917322834645671215, 0.1049643490035301469, -2.544619422572177658 ) ) ;
#30930=EDGE_LOOP ( 'NONE', ( #41583, #77964, #34652, #74847 ) ) ;
#30931=CARTESIAN_POINT ( 'NONE',  ( 0.1058382717557500713, -0.3949938075777409408, -2.919947506561680228 ) ) ;
#30935=CARTESIAN_POINT ( 'NONE',  ( -0.2925321140481932924, 0.2925321140481931814, -1.279527559055118058 ) ) ;
#30937=CARTESIAN_POINT ( 'NONE',  ( -0.2362204724409447953, -0.4091458600556404646, -0.7723097112860892732 ) ) ;
#30940=CARTESIAN_POINT ( 'NONE',  ( -0.3917322834645669549, -0.1049643490035306603, -0.2880577427821523484 ) ) ;
#30950=CARTESIAN_POINT ( 'NONE',  ( 0.3458507752293908943, 0.3458507752293908943, -2.185039370078739829 ) ) ;
#30956=CARTESIAN_POINT ( 'NONE',  ( -0.1265901696524986964, -0.4724409448818899238, -2.276902887139107268 ) ) ;
#30960=CARTESIAN_POINT ( 'NONE',  ( -9.594673741351310580E-17, 0.3917322834645669549, -0.5524741225383709153 ) ) ;
#30962=CARTESIAN_POINT ( 'NONE',  ( 0.1958661417322834775, 0.3392501089628018884, -0.7014435695538058235 ) ) ;
#30967=CARTESIAN_POINT ( 'NONE',  ( -0.3392501089628019995, 0.1958661417322832277, -2.695538057742782101 ) ) ;
#30970=CARTESIAN_POINT ( 'NONE',  ( -0.1265901696524993347, 0.4724409448818895907, -0.8707349081364830212 ) ) ;
#30978=CARTESIAN_POINT ( 'NONE',  ( 0.3458507752293908943, 0.3458507752293908943, -0.2952755905511810774 ) ) ;
#30982=CARTESIAN_POINT ( 'NONE',  ( -0.1998031496062994405, 0.3460692066303957537, -2.137139107611548905 ) ) ;
#30990=CARTESIAN_POINT ( 'NONE',  ( 0.3996062992125985480, -0.1070741851644052972, -0.6607611548556431291 ) ) ;
#30991=CARTESIAN_POINT ( 'NONE',  ( -0.3996062992125987146, 0.1070741851644051862, -0.9776902887139107268 ) ) ;
#30992=CARTESIAN_POINT ( 'NONE',  ( -0.1974969037888703871, -0.3420746716998661063, -0.2230971128608924547 ) ) ;
#30998=CARTESIAN_POINT ( 'NONE',  ( 0.2362204724409451007, -0.4091458600556402980, -2.373359580052493367 ) ) ;
#30999=CARTESIAN_POINT ( 'NONE',  ( 0.2891555358219910499, 0.2891555358219910499, -1.159448818897637956 ) ) ;
#31004=CARTESIAN_POINT ( 'NONE',  ( -0.4091458600556402980, -0.2362204724409451284, -1.784776902887138972 ) ) ;
#31005=CARTESIAN_POINT ( 'NONE',  ( -0.1998031496062991907, -0.3460692066303959757, -2.742782152230971437 ) ) ;
#31007=ORIENTED_EDGE ( 'NONE', *, *, #3924, .F. ) ;
#31020=CARTESIAN_POINT ( 'NONE',  ( -0.3917322834645671215, 0.1049643490035301469, -1.599737532808399143 ) ) ;
#31023=CARTESIAN_POINT ( 'NONE',  ( -0.2891555358219911054, 0.2891555358219909388, -1.279527559055118280 ) ) ;
#31028=CARTESIAN_POINT ( 'NONE',  ( -0.1998031496062994683, 0.3460692066303958092, -0.01312335958005250193 ) ) ;
#31035=CARTESIAN_POINT ( 'NONE',  ( -0.3392501089628017219, -0.1958661417322836718, 0.02034120734908127781 ) ) ;
#31041=CARTESIAN_POINT ( 'NONE',  ( -0.2925321140481932924, 0.2925321140481931814, -2.066929133858267154 ) ) ;
#31044=CARTESIAN_POINT ( 'NONE',  ( -0.1998031496062994405, 0.3460692066303957537, -1.507217847769029007 ) ) ;
#31048=CARTESIAN_POINT ( 'NONE',  ( 0.2362204724409449064, 0.4091458600556404646, -0.9317585301837270073 ) ) ;
#31051=CARTESIAN_POINT ( 'NONE',  ( -0.3917322834645670104, -7.196005306013484475E-17, -2.801181102362204633 ) ) ;
#31057=CARTESIAN_POINT ( 'NONE',  ( -0.1998031496062991630, -0.3460692066303959202, 0.1725721784776902690 ) ) ;
#31060=CARTESIAN_POINT ( 'NONE',  ( 0.1058382717557500852, -0.3949938075777408852, -2.209317585301837639 ) ) ;
#31071=( BOUNDED_CURVE ( )  B_SPLINE_CURVE ( 2, ( #72961, #47689, #48108, #15312, #67071, #73806, #9403, #29170, #35487, #35073, #61151, #61575, #76277 ),
 .UNSPECIFIED., .F., .F. ) 
 B_SPLINE_CURVE_WITH_KNOTS ( ( 3, 2, 2, 2, 2, 2, 3 ),
 ( 0.3875000000000000111, 0.3916666666666666630, 0.3958333333333333148, 0.4000000000000000222, 0.4041666666666667296, 0.4083333333333333814, 0.4125000000000000333 ),
 .UNSPECIFIED. ) 
 CURVE ( )  GEOMETRIC_REPRESENTATION_ITEM ( )  RATIONAL_B_SPLINE_CURVE ( ( 1.000000000000000000, 0.9659258262890683122, 1.000000000000000000, 0.9659258262890683122, 1.000000000000000000, 0.9659258262890683122, 1.000000000000000000, 0.9659258262890683122, 1.000000000000000000, 0.9659258262890683122, 1.000000000000000000, 0.9659258262890678681, 1.000000000000000444 ) ) 
 REPRESENTATION_ITEM ( '' )  );
#31082=CARTESIAN_POINT ( 'NONE',  ( -0.2925321140481932369, 0.2925321140481931259, -0.8838582677165351953 ) ) ;
#31083=CARTESIAN_POINT ( 'NONE',  ( 0.3392501089628018329, 0.1958661417322835607, -2.105643044619422533 ) ) ;
#31099=CARTESIAN_POINT ( 'NONE',  ( 0.1958661417322836440, -0.3392501089628017219, -1.908792650918635259 ) ) ;
#31106=CARTESIAN_POINT ( 'NONE',  ( 0.1998031496062992740, 0.3460692066303959757, -0.9317585301837270073 ) ) ;
#31108=CARTESIAN_POINT ( 'NONE',  ( -0.1958661417322834220, -0.3392501089628018884, -2.577427821522309426 ) ) ;
#31121=CARTESIAN_POINT ( 'NONE',  ( -0.1049643490035307020, 0.3917322834645669549, 0.1587926509186352031 ) ) ;
#31124=CARTESIAN_POINT ( 'NONE',  ( -0.1974969037888706647, 0.3420746716998658843, -0.1706036745406825095 ) ) ;
#31132=CARTESIAN_POINT ( 'NONE',  ( 0.1049643490035303967, 0.3917322834645670659, -1.722460260663728926 ) ) ;
#31134=CARTESIAN_POINT ( 'NONE',  ( -0.2867679344610365999, 0.2867679344610364889, -2.624015748031495399 ) ) ;
#31139=CARTESIAN_POINT ( 'NONE',  ( 0.3996062992125986035, 2.446882876249141962E-17, -0.9055118110236221041 ) ) ;
#31141=CARTESIAN_POINT ( 'NONE',  ( 0.1998031496062992463, 0.3460692066303959202, -0.2211286089238845010 ) ) ;
#31143=CARTESIAN_POINT ( 'NONE',  ( 0.1998031496062992740, 0.3460692066303959757, -2.191601049868766360 ) ) ;
#31145=CARTESIAN_POINT ( 'NONE',  ( -0.1958661417322836718, 0.3392501089628017219, -1.830052493438320216 ) ) ;
#31149=CARTESIAN_POINT ( 'NONE',  ( -0.4091458600556405756, 0.2362204724409446288, -1.205380577427821454 ) ) ;
#31152=CARTESIAN_POINT ( 'NONE',  ( -0.1058382717557503072, 0.3949938075777408852, -1.185695538057742748 ) ) ;
#31163=CARTESIAN_POINT ( 'NONE',  ( -0.1070741851644056997, 0.3996062992125984925, -1.815616797900262425 ) ) ;
#31180=CARTESIAN_POINT ( 'NONE',  ( 0.1958661417322834775, 0.3392501089628018884, -1.173884514435695525 ) ) ;
#31197=CARTESIAN_POINT ( 'NONE',  ( -0.4724409448818898682, -8.678599364036362592E-17, -1.218503937007874072 ) ) ;
#31201=CARTESIAN_POINT ( 'NONE',  ( -0.2867679344610364334, -0.2867679344610367109, -2.255905511811023612 ) ) ;
#31204=CARTESIAN_POINT ( 'NONE',  ( -0.4091458600556405756, 0.2362204724409446288, -0.3412073490813647969 ) ) ;
#31205=CARTESIAN_POINT ( 'NONE',  ( 0.1974969037888706369, -0.3420746716998659953, -2.926509186351706315 ) ) ;
#31208=CARTESIAN_POINT ( 'NONE',  ( 0.1049643490035303689, 0.3917322834645670104, -1.245406824146981561 ) ) ;
#31210=CARTESIAN_POINT ( 'NONE',  ( -0.4724409448818899238, 0.1265901696524986686, -2.709973753280840114 ) ) ;
#31217=CARTESIAN_POINT ( 'NONE',  ( 4.797336870675655290E-17, -0.3917322834645669549, -0.7886945949793155997 ) ) ;
#31224=CARTESIAN_POINT ( 'NONE',  ( -9.594673741351313045E-17, 0.3917322834645670659, -1.886502255414385099 ) ) ;
#31230=AXIS2_PLACEMENT_3D ( 'NONE', #45148, #69606, #70851 ) ;
#31232=CARTESIAN_POINT ( 'NONE',  ( -0.3917322834645671215, 0.1049643490035301469, -1.534776902887139194 ) ) ;
#31237=CARTESIAN_POINT ( 'NONE',  ( -9.787531504996567848E-17, 0.3996062992125986035, -1.920830620545185230E-17 ) ) ;
#31242=CARTESIAN_POINT ( 'NONE',  ( 0.2867679344610365999, 0.2867679344610365999, -2.649606299212598604 ) ) ;
#31249=CARTESIAN_POINT ( 'NONE',  ( 0.3392501089628018884, -0.1958661417322834220, -1.134514435695538115 ) ) ;
#31252=CARTESIAN_POINT ( 'NONE',  ( -0.3996062992125985480, -7.340648628747423112E-17, -2.635826771653543066 ) ) ;
#31262=CARTESIAN_POINT ( 'NONE',  ( 0.1998031496062994128, -0.3460692066303957537, -0.6410761154855643129 ) ) ;
#31264=CARTESIAN_POINT ( 'NONE',  ( -0.3917322834645669549, -0.1049643490035306603, -0.1955380577427821009 ) ) ;
#31271=EDGE_CURVE ( 'NONE', #59707, #23851, #20989, .T. ) ;
#31280=CARTESIAN_POINT ( 'NONE',  ( -0.3917322834645671770, 0.1049643490035302024, -0.8169484496401069329 ) ) ;
#31284=CARTESIAN_POINT ( 'NONE',  ( -0.4724409448818898682, -8.678599364036362592E-17, -2.478346456692913868 ) ) ;
#31303=CARTESIAN_POINT ( 'NONE',  ( -0.3460692066303958092, -0.1998031496062994683, -0.3674540682414698112 ) ) ;
#31304=CARTESIAN_POINT ( 'NONE',  ( -0.3460692066303957537, -0.1998031496062994405, -2.806430446194225770 ) ) ;
#31309=CARTESIAN_POINT ( 'NONE',  ( 0.1070741851644053527, 0.3996062992125986590, -2.355643044619422533 ) ) ;
#31310=CARTESIAN_POINT ( 'NONE',  ( 0.2891555358219910499, 0.2891555358219910499, -1.555118110236220375 ) ) ;
#31311=CARTESIAN_POINT ( 'NONE',  ( 0.2925321140481932369, -0.2925321140481932369, -2.933070866141732402 ) ) ;
#31313=CARTESIAN_POINT ( 'NONE',  ( -0.3917322834645670104, -7.196005306013484475E-17, -0.5039370078740157410 ) ) ;
#31316=CARTESIAN_POINT ( 'NONE',  ( 4.837279021331061486E-17, -0.3949938075777409963, -2.675196850393700920 ) ) ;
#31320=CARTESIAN_POINT ( 'NONE',  ( 5.785732909357575061E-17, -0.4724409448818898682, -2.755905511811023612 ) ) ;
#31321=CARTESIAN_POINT ( 'NONE',  ( -0.3996062992125987146, 0.1070741851644051862, -2.237532808398950301 ) ) ;
#31328=CARTESIAN_POINT ( 'NONE',  ( 0.2867679344610365999, 0.2867679344610365999, -0.2224409448818898127 ) ) ;
#31335=CARTESIAN_POINT ( 'NONE',  ( 0.3392501089628018329, 0.1958661417322835607, -0.3733595800524935338 ) ) ;
#31336=CARTESIAN_POINT ( 'NONE',  ( -0.3392501089628017219, -0.1958661417322836718, -1.304461942257217899 ) ) ;
#31337=CARTESIAN_POINT ( 'NONE',  ( 0.1049643490035303689, 0.3917322834645670104, -2.662729658792650778 ) ) ;
#31339=CARTESIAN_POINT ( 'NONE',  ( 0.3949938075777409963, 2.418639510665530435E-17, -2.952755905511811108 ) ) ;
#31343=CARTESIAN_POINT ( 'NONE',  ( -0.3996062992125987146, 0.1070741851644051862, -1.450131233595800317 ) ) ;
#31348=CARTESIAN_POINT ( 'NONE',  ( -9.594673741351313045E-17, 0.3917322834645670104, -0.3996062992125985480 ) ) ;
#31359=CARTESIAN_POINT ( 'NONE',  ( -0.4091458600556405756, 0.2362204724409446288, -2.230971128608923770 ) ) ;
#31366=CARTESIAN_POINT ( 'NONE',  ( -0.4091458600556402980, -0.2362204724409451284, -2.257217847769029007 ) ) ;
#31367=CARTESIAN_POINT ( 'NONE',  ( 0.4724409448818898127, -0.1265901696524988629, -2.708005249343832244 ) ) ;
#31370=CARTESIAN_POINT ( 'NONE',  ( 4.797336870675655290E-17, -0.3917322834645669549, -0.3162536500974260090 ) ) ;
#31373=CARTESIAN_POINT ( 'NONE',  ( 0.3917322834645670104, 2.398668435337828261E-17, -0.9901574803149607584 ) ) ;
#31378=CARTESIAN_POINT ( 'NONE',  ( 0.3392501089628018884, -0.1958661417322834220, -2.931758530183726563 ) ) ;
#31381=CARTESIAN_POINT ( 'NONE',  ( -0.4724409448818895907, -0.1265901696524993070, -1.382545931758530022 ) ) ;
#31394=CARTESIAN_POINT ( 'NONE',  ( -0.1998031496062994405, 0.3460692066303957537, -2.452099737532808188 ) ) ;
#31397=CARTESIAN_POINT ( 'NONE',  ( 0.1070741851644054776, -0.3996062992125984925, -1.579396325459317740 ) ) ;
#31401=DIRECTION ( 'NONE',  ( -0.000000000000000000, -1.000000000000000000, -0.000000000000000000 ) ) ;
#31403=CARTESIAN_POINT ( 'NONE',  ( -0.3460692066303957537, -0.1998031496062994405, -0.7591863517060367661 ) ) ;
#31404=CARTESIAN_POINT ( 'NONE',  ( 0.3460692066303959757, -0.1998031496062991907, -0.8923884514435694859 ) ) ;
#31406=CARTESIAN_POINT ( 'NONE',  ( -0.1058382717557497937, -0.3949938075777411628, -0.2296587926509187083 ) ) ;
#31412=CARTESIAN_POINT ( 'NONE',  ( -0.3420746716998660508, -0.1974969037888706924, -1.231627296587926468 ) ) ;
#31417=CARTESIAN_POINT ( 'NONE',  ( -0.2362204724409451284, 0.4091458600556402425, -1.587926509186351698 ) ) ;
#31432=CARTESIAN_POINT ( 'NONE',  ( 0.1958661417322834775, 0.3392501089628018884, -1.396325459317585338 ) ) ;
#31435=CARTESIAN_POINT ( 'NONE',  ( -0.1058382717557497937, -0.3949938075777411628, -1.489501312335957950 ) ) ;
#31440=CARTESIAN_POINT ( 'NONE',  ( 0.1998031496062992740, 0.3460692066303959757, -0.3018372703412073310 ) ) ;
#31447=CARTESIAN_POINT ( 'NONE',  ( -0.1958661417322836718, 0.3392501089628017219, -0.09776902887139117537 ) ) ;
#31454=CARTESIAN_POINT ( 'NONE',  ( 0.1070741851644053527, 0.3996062992125986590, -2.198162729658792447 ) ) ;
#31457=CARTESIAN_POINT ( 'NONE',  ( 0.3996062992125985480, 2.446882876249141654E-17, -1.769685039370078927 ) ) ;
#31462=CARTESIAN_POINT ( 'NONE',  ( -0.4091458600556402980, -0.2362204724409451284, -0.6824146981627295938 ) ) ;
#31464=CARTESIAN_POINT ( 'NONE',  ( 0.1958661417322836440, -0.3392501089628017219, -0.08398950131233590133 ) ) ;
#31466=CARTESIAN_POINT ( 'NONE',  ( 0.1958661417322834775, 0.3392501089628018884, -2.118766404199475151 ) ) ;
#31470=CARTESIAN_POINT ( 'NONE',  ( -0.4724409448818898682, -8.678599364036362592E-17, -2.635826771653543066 ) ) ;
#31474=CARTESIAN_POINT ( 'NONE',  ( -0.3420746716998662729, 0.1974969037888702206, -2.307742782152230721 ) ) ;
#31487=DIRECTION ( 'NONE',  ( 0.000000000000000000, 0.000000000000000000, 1.000000000000000000 ) ) ;
#31496=CARTESIAN_POINT ( 'NONE',  ( -0.3996062992125985480, -7.340648628747423112E-17, -0.7460629921259841479 ) ) ;
#31498=CARTESIAN_POINT ( 'NONE',  ( 0.3917322834645669549, 0.1049643490035304660, -2.414041994750655729 ) ) ;
#31508=CARTESIAN_POINT ( 'NONE',  ( -0.3917322834645670104, -0.1049643490035307020, -2.247394643865828545 ) ) ;
#31509=EDGE_LOOP ( 'NONE', ( #49142, #76909, #25116, #2367, #34287 ) ) ;
#31510=AXIS2_PLACEMENT_3D ( 'NONE', #64477, #59827, #7237 ) ;
#31516=CARTESIAN_POINT ( 'NONE',  ( -0.1958661417322834220, -0.3392501089628018884, -1.882545931758530244 ) ) ;
#31524=CARTESIAN_POINT ( 'NONE',  ( 0.1998031496062994405, -0.3460692066303958092, -1.509186351706036655 ) ) ;
#31527=CARTESIAN_POINT ( 'NONE',  ( 0.1049643490035303689, 0.3917322834645670104, -2.505249343832020248 ) ) ;
#31539=CARTESIAN_POINT ( 'NONE',  ( -9.594673741351313045E-17, 0.3917322834645670104, -0.3070866141732283006 ) ) ;
#31542=CARTESIAN_POINT ( 'NONE',  ( 0.1058382717557500713, -0.3949938075777409408, -0.2427821522309712154 ) ) ;
#31545=DIRECTION ( 'NONE',  ( 0.000000000000000000, 0.000000000000000000, 1.000000000000000000 ) ) ;
#31549=CARTESIAN_POINT ( 'NONE',  ( 0.2867679344610366554, -0.2867679344610365999, -1.512486507382889256 ) ) ;
#31551=CARTESIAN_POINT ( 'NONE',  ( -0.3917322834645670104, -7.196005306013484475E-17, -2.486220472440944906 ) ) ;
#31555=CARTESIAN_POINT ( 'NONE',  ( -0.1998031496062991907, -0.3460692066303959757, -0.6955380577427822120 ) ) ;
#31557=CARTESIAN_POINT ( 'NONE',  ( 0.3996062992125985480, 2.446882876249141654E-17, -0.5098425196850393526 ) ) ;
#31558=CARTESIAN_POINT ( 'NONE',  ( -0.2925321140481930149, -0.2925321140481933480, -0.1358267716535433156 ) ) ;
#31560=CARTESIAN_POINT ( 'NONE',  ( 0.3996062992125986035, 0.1070741851644054776, -2.801837270341207553 ) ) ;
#31561=CARTESIAN_POINT ( 'NONE',  ( 0.1049643490035303689, 0.3917322834645670104, -1.810367454068241511 ) ) ;
#31566=CARTESIAN_POINT ( 'NONE',  ( -0.3458507752293909498, 0.3458507752293907833, -1.513779527559054872 ) ) ;
#31570=CARTESIAN_POINT ( 'NONE',  ( 0.3949938075777408852, 0.1058382717557500435, -0.9888451443569553634 ) ) ;
#31581=CARTESIAN_POINT ( 'NONE',  ( -0.1998031496062994405, 0.3460692066303957537, -1.979658792650918597 ) ) ;
#31584=CYLINDRICAL_SURFACE ( 'NONE', #48676, 0.4724409448818898682 ) ;
#31596=CARTESIAN_POINT ( 'NONE',  ( 0.3917322834645670104, 2.398668435337828261E-17, -0.8326771653543307838 ) ) ;
#31604=LINE ( 'NONE', #464, #50150 ) ;
#31611=CARTESIAN_POINT ( 'NONE',  ( -0.3458507752293906723, -0.3458507752293910609, -0.5314960629921260393 ) ) ;
#31612=CARTESIAN_POINT ( 'NONE',  ( -0.4724409448818898682, -8.678599364036362592E-17, -2.244094488188976388 ) ) ;
#31615=CARTESIAN_POINT ( 'NONE',  ( 0.2867679344610366554, 0.2867679344610366554, -2.019685039370078261 ) ) ;
#31618=CARTESIAN_POINT ( 'NONE',  ( 0.3458507752293908943, 0.3458507752293908943, -0.1377952755905511861 ) ) ;
#31619=CARTESIAN_POINT ( 'NONE',  ( -0.1974969037888706647, 0.3420746716998658843, -2.690288713910760965 ) ) ;
#31622=CARTESIAN_POINT ( 'NONE',  ( -9.594673741351313045E-17, 0.3917322834645670104, -1.566929133858267820 ) ) ;
#31632=CARTESIAN_POINT ( 'NONE',  ( 4.797336870675655290E-17, -0.3917322834645669549, -0.6312142800186859581 ) ) ;
#31639=CARTESIAN_POINT ( 'NONE',  ( -0.1958661417322833942, -0.3392501089628018884, -2.109599368275277609 ) ) ;
#31645=EDGE_CURVE ( 'NONE', #45904, #69925, #79671, .T. ) ;
#31648=CARTESIAN_POINT ( 'NONE',  ( -0.1049643490035302024, -0.3917322834645671215, -1.259186351706037099 ) ) ;
#31654=CARTESIAN_POINT ( 'NONE',  ( -0.005815251566291224430, 0.3972027188793958996, 2.415985422253608372E-12 ) ) ;
#31658=CARTESIAN_POINT ( 'NONE',  ( -0.3917322834645669549, -0.1049643490035306603, -2.872703412073490448 ) ) ;
#31664=CARTESIAN_POINT ( 'NONE',  ( 0.4724409448818898127, -0.1265901696524988629, -0.4265091863517060378 ) ) ;
#31665=CARTESIAN_POINT ( 'NONE',  ( 0.3917322834645670104, 2.398668435337828261E-17, -1.147637795275590733 ) ) ;
#31666=CARTESIAN_POINT ( 'NONE',  ( -0.3458507752293909498, 0.3458507752293907833, -0.4114173228346455491 ) ) ;
#31669=CARTESIAN_POINT ( 'NONE',  ( 0.3420746716998660508, -0.1974969037888704149, 0.1332020997375328031 ) ) ;
#31680=CARTESIAN_POINT ( 'NONE',  ( -0.2925321140481932369, 0.2925321140481931259, -0.5688976377952755792 ) ) ;
#31682=CARTESIAN_POINT ( 'NONE',  ( 0.1049643490035303689, 0.3917322834645670104, -0.1430446194225721002 ) ) ;
#31696=CARTESIAN_POINT ( 'NONE',  ( 0.2867679344610366554, -0.2867679344610365999, -0.7250849325797394940 ) ) ;
#31701=CARTESIAN_POINT ( 'NONE',  ( 0.4724409448818898682, 2.892866454678787531E-17, -2.399606299212598604 ) ) ;
#31714=MANIFOLD_SOLID_BREP ( 'Cut-Sweep1', #11102 ) ;
#31720=CARTESIAN_POINT ( 'NONE',  ( -0.1070741851644057135, 0.3996062992125985480, -0.4790026246719158998 ) ) ;
#31721=CARTESIAN_POINT ( 'NONE',  ( 0.3996062992125984925, 0.1070741851644054637, -2.721128608923884418 ) ) ;
#31726=CARTESIAN_POINT ( 'NONE',  ( 0.3460692066303959202, 0.1998031496062993295, -2.020997375328084100 ) ) ;
#31727=CARTESIAN_POINT ( 'NONE',  ( -0.2891555358219911054, 0.2891555358219909388, -1.437007874015748143 ) ) ;
#31728=CARTESIAN_POINT ( 'NONE',  ( -0.1998031496062991907, -0.3460692066303959757, -2.742782152230971437 ) ) ;
#31730=CARTESIAN_POINT ( 'NONE',  ( -0.1049643490035307020, 0.3917322834645669549, -0.9435695538057738974 ) ) ;
#31733=CARTESIAN_POINT ( 'NONE',  ( 0.1974969037888704704, 0.3420746716998660508, -2.583333333333333481 ) ) ;
#31737=CARTESIAN_POINT ( 'NONE',  ( -1.157146581871515012E-16, 0.4724409448818898682, -2.677165354330708347 ) ) ;
#31739=CARTESIAN_POINT ( 'NONE',  ( 0.3460692066303959757, -0.1998031496062991907, -1.994750656167979086 ) ) ;
#31747=CARTESIAN_POINT ( 'NONE',  ( -0.1958661417322836718, 0.3392501089628017219, 0.05971128608923875758 ) ) ;
#31755=CARTESIAN_POINT ( 'NONE',  ( 0.3392501089628018329, 0.1958661417322835607, -0.6883202099737534274 ) ) ;
#31756=CARTESIAN_POINT ( 'NONE',  ( 0.3917322834645670104, 2.398668435337828261E-17, -1.527559055118110409 ) ) ;
#31757=CARTESIAN_POINT ( 'NONE',  ( -0.1958661417322836718, 0.3392501089628017219, -2.839895013123359568 ) ) ;
#31759=CARTESIAN_POINT ( 'NONE',  ( 0.3949938075777411073, -0.1058382717557499464, -2.946194225721785909 ) ) ;
#31764=CARTESIAN_POINT ( 'NONE',  ( 0.1070741851644053527, 0.3996062992125986590, -1.568241469816272993 ) ) ;
#31769=CARTESIAN_POINT ( 'NONE',  ( -0.3392501089628017219, -0.1958661417322836718, -0.9245406824146982228 ) ) ;
#31777=CARTESIAN_POINT ( 'NONE',  ( -0.3458507752293909498, 0.3458507752293907833, -1.909448818897637512 ) ) ;
#31778=CARTESIAN_POINT ( 'NONE',  ( -0.4091458600556405756, 0.2362204724409446288, -2.703412073490813583 ) ) ;
#31783=CARTESIAN_POINT ( 'NONE',  ( 0.4724409448818898682, 2.892866454678787531E-17, -0.6673228346456693272 ) ) ;
#31787=CARTESIAN_POINT ( 'NONE',  ( -0.1049643490035301746, -0.3917322834645670659, -0.6246526002286596491 ) ) ;
#31789=CARTESIAN_POINT ( 'NONE',  ( -0.3917322834645670104, -7.196005306013484475E-17, -0.9114173228346457156 ) ) ;
#31794=CARTESIAN_POINT ( 'NONE',  ( -9.594673741351313045E-17, 0.3917322834645670104, -2.826771653543306506 ) ) ;
#31799=CARTESIAN_POINT ( 'NONE',  ( -0.1265901696524993347, 0.4724409448818895907, -1.028215223097112663 ) ) ;
#31812=CARTESIAN_POINT ( 'NONE',  ( -0.3460692066303960313, 0.1998031496062989965, -2.307742782152230721 ) ) ;
#31816=CARTESIAN_POINT ( 'NONE',  ( 0.1998031496062994128, -0.3460692066303957537, -1.428477690288713964 ) ) ;
#31822=CARTESIAN_POINT ( 'NONE',  ( -0.1998031496062994405, 0.3460692066303957537, -0.5623359580052492701 ) ) ;
#31823=CARTESIAN_POINT ( 'NONE',  ( -0.3996062992125986035, -0.1070741851644056997, -0.8333333333333332593 ) ) ;
#31824=CARTESIAN_POINT ( 'NONE',  ( 0.1058382717557499880, 0.3949938075777411073, -0.1509186351706037210 ) ) ;
#31830=CARTESIAN_POINT ( 'NONE',  ( 0.3949938075777409408, -0.1058382717557499186, -1.133202099737532720 ) ) ;
#31836=CARTESIAN_POINT ( 'NONE',  ( -0.4724409448818899238, 0.1265901696524986686, -1.607611548556430403 ) ) ;
#31837=CARTESIAN_POINT ( 'NONE',  ( 0.3460692066303959202, 0.1998031496062993295, -2.650918635170603554 ) ) ;
#31844=CARTESIAN_POINT ( 'NONE',  ( -0.3917322834645669549, -7.196005306013483243E-17, -2.166647350884827183 ) ) ;
#31851=CARTESIAN_POINT ( 'NONE',  ( 0.1958661417322834775, 0.3392501089628018884, -1.553805774278215202 ) ) ;
#31854=CARTESIAN_POINT ( 'NONE',  ( -0.3420746716998661618, 0.1974969037888702206, -1.916010498687664043 ) ) ;
#31862=CARTESIAN_POINT ( 'NONE',  ( 4.893765752498283924E-17, -0.3996062992125986035, -0.3937007874015748254 ) ) ;
#31869=CARTESIAN_POINT ( 'NONE',  ( 0.3917322834645670104, -0.1049643490035303411, -0.3536745406824148286 ) ) ;
#31876=CARTESIAN_POINT ( 'NONE',  ( -0.2925321140481932369, 0.2925321140481931259, -2.143700787401574548 ) ) ;
#31881=CARTESIAN_POINT ( 'NONE',  ( -0.2362204724409447953, -0.4091458600556404646, -0.6955380577427822120 ) ) ;
#31883=CARTESIAN_POINT ( 'NONE',  ( 0.2867679344610365999, -0.2867679344610365444, -2.860236220472440749 ) ) ;
#31884=CARTESIAN_POINT ( 'NONE',  ( 4.797336870675656522E-17, -0.3917322834645670104, -2.210629921259842590 ) ) ;
#31888=CARTESIAN_POINT ( 'NONE',  ( -0.4724409448818898682, -8.678599364036362592E-17, -2.793307086614173151 ) ) ;
#31891=CARTESIAN_POINT ( 'NONE',  ( 0.1974969037888706092, -0.3420746716998660508, -2.373359580052493811 ) ) ;
#31898=CARTESIAN_POINT ( 'NONE',  ( 0.1049643490035303689, 0.3917322834645670104, -1.560367454068241511 ) ) ;
#31901=CARTESIAN_POINT ( 'NONE',  ( -0.4724409448818898682, -8.678599364036362592E-17, 0.04133858267716534335 ) ) ;
#31905=DIRECTION ( 'NONE',  ( 1.000000000000000000, 0.000000000000000000, 0.000000000000000000 ) ) ;
#31913=CARTESIAN_POINT ( 'NONE',  ( -0.1998031496062994405, 0.3460692066303957537, -1.349737532808398921 ) ) ;
#31914=CARTESIAN_POINT ( 'NONE',  ( 0.3917322834645670104, 2.398668435337828261E-17, -2.250000000000000000 ) ) ;
#31926=CARTESIAN_POINT ( 'NONE',  ( 0.1049643490035303967, 0.3917322834645670659, -2.037420890584989319 ) ) ;
#31932=CARTESIAN_POINT ( 'NONE',  ( -0.2867679344610365999, 0.2867679344610364889, -2.151574803149605586 ) ) ;
#31933=CARTESIAN_POINT ( 'NONE',  ( -0.1584414948821151747, 0.3588842212258044340, -1.220472440944881942 ) ) ;
#31937=CARTESIAN_POINT ( 'NONE',  ( 0.000000000000000000, 0.000000000000000000, -2.755905511811024056 ) ) ;
#31940=CARTESIAN_POINT ( 'NONE',  ( 0.1070741851644054915, -0.3996062992125986035, -1.187664041994750619 ) ) ;
#31942=CARTESIAN_POINT ( 'NONE',  ( -0.3917322834645670659, -7.196005306013484475E-17, -0.03610855462698352170 ) ) ;
#31956=CARTESIAN_POINT ( 'NONE',  ( -0.3392501089628019995, 0.1958661417322832277, -0.01837270341207344546 ) ) ;
#31959=CARTESIAN_POINT ( 'NONE',  ( -9.674558042662121740E-17, 0.3949938075777409963, -0.6299212598425196763 ) ) ;
#31966=CARTESIAN_POINT ( 'NONE',  ( 0.3917322834645670659, 2.398668435337828261E-17, -1.532171546752967739 ) ) ;
#31968=CARTESIAN_POINT ( 'NONE',  ( 4.797336870675656522E-17, -0.3917322834645670104, -2.683070866141731958 ) ) ;
#31973=CARTESIAN_POINT ( 'NONE',  ( -0.3460692066303958092, -0.1998031496062994683, -0.8398950131233595684 ) ) ;
#31975=CARTESIAN_POINT ( 'NONE',  ( 0.2925321140481932369, -0.2925321140481931814, -0.1751968503937007537 ) ) ;
#31976=CARTESIAN_POINT ( 'NONE',  ( 0.1998031496062992463, 0.3460692066303959202, -0.2211286089238845565 ) ) ;
#31978=CARTESIAN_POINT ( 'NONE',  ( -0.3996062992125987146, 0.1070741851644051862, -2.709973753280840114 ) ) ;
#31979=CARTESIAN_POINT ( 'NONE',  ( -9.594673741351313045E-17, 0.3917322834645670104, -1.659448818897637734 ) ) ;
#31985=CARTESIAN_POINT ( 'NONE',  ( 0.2362204724409451007, -0.4091458600556402980, -1.585958005249344049 ) ) ;
#31988=CARTESIAN_POINT ( 'NONE',  ( 0.3420746716998660508, 0.1974969037888705814, -0.9954068241469814504 ) ) ;
#31998=CARTESIAN_POINT ( 'NONE',  ( -0.3460692066303957537, -0.1998031496062994405, -2.019028871391076230 ) ) ;
#32000=EDGE_CURVE ( 'NONE', #81066, #78139, #35203, .T. ) ;
#32001=CARTESIAN_POINT ( 'NONE',  ( 0.1958661417322834497, 0.3392501089628018329, -1.484232652722097923 ) ) ;
#32003=CARTESIAN_POINT ( 'NONE',  ( 0.000000000000000000, 0.000000000000000000, -2.755905511811024056 ) ) ;
#32012=CARTESIAN_POINT ( 'NONE',  ( 4.893765752498283308E-17, -0.3996062992125985480, 0.001968503937007862279 ) ) ;
#32014=CARTESIAN_POINT ( 'NONE',  ( -9.594673741351313045E-17, 0.3917322834645670104, -0.8720472440944883052 ) ) ;
#32032=DIRECTION ( 'NONE',  ( 0.000000000000000000, 0.000000000000000000, 1.000000000000000000 ) ) ;
#32035=CARTESIAN_POINT ( 'NONE',  ( -0.1049643490035301885, -0.3917322834645671215, -2.583989501312335513 ) ) ;
#32038=CARTESIAN_POINT ( 'NONE',  ( -0.2362204724409451284, 0.4091458600556402425, -0.1706036745406823985 ) ) ;
#32039=CARTESIAN_POINT ( 'NONE',  ( -0.1070741851644051862, -0.3996062992125987146, 0.08530183727034119923 ) ) ;
#32042=CARTESIAN_POINT ( 'NONE',  ( 0.3392501089628018329, 0.1958661417322835607, -1.698162729658792891 ) ) ;
#32044=CARTESIAN_POINT ( 'NONE',  ( 0.3458507752293908943, 0.3458507752293908943, -2.814960629921259727 ) ) ;
#32051=CARTESIAN_POINT ( 'NONE',  ( 0.2867679344610365999, 0.2867679344610365999, -0.6902693981289222958 ) ) ;
#32058=CARTESIAN_POINT ( 'NONE',  ( 0.1958661417322834775, 0.3392501089628018884, -2.188339525755591986 ) ) ;
#32065=CARTESIAN_POINT ( 'NONE',  ( -9.594673741351313045E-17, 0.3917322834645670104, -1.187007874015748143 ) ) ;
#32081=CARTESIAN_POINT ( 'NONE',  ( -0.3917322834645670104, -7.196005306013484475E-17, -1.226377952755905776 ) ) ;
#32082=CARTESIAN_POINT ( 'NONE',  ( 0.2362204724409451007, -0.4091458600556402980, -0.1686351706036745557 ) ) ;
#32085=CARTESIAN_POINT ( 'NONE',  ( 0.3996062992125985480, 2.446882876249141654E-17, -2.872047244094488416 ) ) ;
#32090=CARTESIAN_POINT ( 'NONE',  ( 0.3949938075777409408, -0.1058382717557499186, -0.1883202099737532886 ) ) ;
#32097=CARTESIAN_POINT ( 'NONE',  ( 0.1998031496062994128, -0.3460692066303957537, -0.7985564304461942875 ) ) ;
#32099=EDGE_CURVE ( 'NONE', #64782, #39936, #83143, .T. ) ;
#32100=CARTESIAN_POINT ( 'NONE',  ( -0.2867679344610365999, 0.2867679344610364889, -0.1692913385826771144 ) ) ;
#32118=CARTESIAN_POINT ( 'NONE',  ( -0.3458507752293909498, 0.3458507752293907833, -2.458661417322834719 ) ) ;
#32135=CARTESIAN_POINT ( 'NONE',  ( 0.3996062992125986035, 2.446882876249141962E-17, -0.2755905511811024278 ) ) ;
#32136=CARTESIAN_POINT ( 'NONE',  ( -0.1998031496062994405, 0.3460692066303957537, -2.609580052493438274 ) ) ;
#32142=CARTESIAN_POINT ( 'NONE',  ( 0.3460692066303959202, 0.1998031496062993295, -2.335958005249343827 ) ) ;
#32143=CARTESIAN_POINT ( 'NONE',  ( 0.1974969037888704704, 0.3420746716998660508, -2.034120734908136718 ) ) ;
#32144=CARTESIAN_POINT ( 'NONE',  ( 0.1049643490035304938, -0.3917322834645669549, -0.5498687664041993495 ) ) ;
#32146=CARTESIAN_POINT ( 'NONE',  ( 0.1958661417322834775, 0.3392501089628018884, -0.9238845144356954142 ) ) ;
#32149=CARTESIAN_POINT ( 'NONE',  ( 0.1058382717557499880, 0.3949938075777409408, -2.747375328083990098 ) ) ;
#32155=CARTESIAN_POINT ( 'NONE',  ( 0.2925321140481932369, -0.2925321140481932369, -1.988188976377952777 ) ) ;
#32156=CARTESIAN_POINT ( 'NONE',  ( 0.3917322834645670104, 0.1049643490035304660, -0.7513316517398445082 ) ) ;
#32162=CARTESIAN_POINT ( 'NONE',  ( 0.3392501089628018329, 0.1958661417322835607, -0.05839895013123368173 ) ) ;
#32170=CARTESIAN_POINT ( 'NONE',  ( -0.1958661417322834220, -0.3392501089628018884, -0.4652230971128609727 ) ) ;
#32171=CARTESIAN_POINT ( 'NONE',  ( -0.1958661417322834220, -0.3392501089628018884, -1.317585301837270295 ) ) ;
#32172=CARTESIAN_POINT ( 'NONE',  ( 0.3917322834645670104, -0.1049643490035303411, -2.623359580052493367 ) ) ;
#32175=CARTESIAN_POINT ( 'NONE',  ( -0.3460692066303958092, -0.1998031496062994683, -0.05249343832020999384 ) ) ;
#32179=CARTESIAN_POINT ( 'NONE',  ( -0.2925321140481932924, 0.2925321140481931814, -1.594488188976378229 ) ) ;
#32184=CARTESIAN_POINT ( 'NONE',  ( -9.594673741351313045E-17, 0.3917322834645670104, -1.029527559055118280 ) ) ;
#32192=CARTESIAN_POINT ( 'NONE',  ( -0.2362204724409451284, 0.4091458600556402425, -1.902887139107611647 ) ) ;
#32194=PLANE ( 'NONE',  #53251 ) ;
#32199=VERTEX_POINT ( 'NONE', #50292 ) ;
#32204=CARTESIAN_POINT ( 'NONE',  ( -0.2867679344610366554, 0.2867679344610365444, -0.7296394768690795951 ) ) ;
#32206=CARTESIAN_POINT ( 'NONE',  ( 0.1049643490035304799, -0.3917322834645669549, -0.7998687664041994605 ) ) ;
#32211=CARTESIAN_POINT ( 'NONE',  ( 0.3917322834645670104, -0.1049643490035303411, -2.780839895013122565 ) ) ;
#32214=CARTESIAN_POINT ( 'NONE',  ( 5.785732909357575061E-17, -0.4724409448818898682, -1.257874015748031260 ) ) ;
#32228=CARTESIAN_POINT ( 'NONE',  ( 0.2925321140481932369, 0.2925321140481932369, -2.419291338582676865 ) ) ;
#32232=CARTESIAN_POINT ( 'NONE',  ( -0.3996062992125985480, -7.340648628747423112E-17, -1.218503937007874072 ) ) ;
#32238=CARTESIAN_POINT ( 'NONE',  ( 0.2925321140481931814, -0.2925321140481931259, -0.6476377952755905110 ) ) ;
#32239=CARTESIAN_POINT ( 'NONE',  ( -0.1998031496062994683, 0.3460692066303958092, -0.8005249343832020470 ) ) ;
#32240=CARTESIAN_POINT ( 'NONE',  ( 0.3949938075777409408, 0.1058382717557500574, -0.1246719160104987345 ) ) ;
#32246=CARTESIAN_POINT ( 'NONE',  ( -0.2891555358219911054, 0.2891555358219909388, -1.198818897637795589 ) ) ;
#32251=CARTESIAN_POINT ( 'NONE',  ( 0.4724409448818896462, 0.1265901696524990294, -1.541994750656167978 ) ) ;
#32259=CARTESIAN_POINT ( 'NONE',  ( 0.1049643490035304522, -0.3917322834645668994, -2.055098794454381927 ) ) ;
#32260=CARTESIAN_POINT ( 'NONE',  ( 0.1070741851644054776, -0.3996062992125984925, -2.839238845144356649 ) ) ;
#32266=CARTESIAN_POINT ( 'NONE',  ( 0.1049643490035304938, -0.3917322834645669549, -1.652230971128608505 ) ) ;
#32269=CARTESIAN_POINT ( 'NONE',  ( 0.1058382717557500713, -0.3949938075777409408, -1.975065616797900159 ) ) ;
#32274=CARTESIAN_POINT ( 'NONE',  ( 0.2925321140481932369, -0.2925321140481932369, -0.09842519685039373412 ) ) ;
#32277=( LENGTH_UNIT ( ) NAMED_UNIT ( * ) SI_UNIT ( $, .METRE. ) );
#32280=CARTESIAN_POINT ( 'NONE',  ( 0.3392501089628018884, -0.1958661417322834220, -0.5045931758530184386 ) ) ;
#32287=CARTESIAN_POINT ( 'NONE',  ( -0.3460692066303957537, -0.1998031496062994405, -1.861548556430446144 ) ) ;
#32292=CARTESIAN_POINT ( 'NONE',  ( -0.2362204724409451284, 0.4091458600556402425, -0.9580052493438320216 ) ) ;
#32294=CARTESIAN_POINT ( 'NONE',  ( -0.3917322834645671215, 0.1049643490035301469, -0.1824146981627296216 ) ) ;
#32295=CARTESIAN_POINT ( 'NONE',  ( 4.797336870675656522E-17, -0.3917322834645670104, -2.053149606299212948 ) ) ;
#32299=CARTESIAN_POINT ( 'NONE',  ( -0.4091458600556402980, -0.2362204724409451284, -2.806430446194225770 ) ) ;
#32303=CARTESIAN_POINT ( 'NONE',  ( 0.3420746716998660508, -0.1974969037888704149, -2.701443569553805713 ) ) ;
#32311=CARTESIAN_POINT ( 'NONE',  ( -0.3917322834645670104, -7.196005306013484475E-17, -1.448818897637795367 ) ) ;
#32314=CARTESIAN_POINT ( 'NONE',  ( -0.1265901696524986964, -0.4724409448818899238, 0.1660104986876640432 ) ) ;
#32328=CARTESIAN_POINT ( 'NONE',  ( -0.2925321140481932369, 0.2925321140481931259, -1.041338582677165281 ) ) ;
#32329=CARTESIAN_POINT ( 'NONE',  ( -0.2867679344610364334, -0.2867679344610367109, -2.505905511811023612 ) ) ;
#32339=CARTESIAN_POINT ( 'NONE',  ( -0.2925321140481932924, 0.2925321140481931814, 0.1377952755905511584 ) ) ;
#32340=CARTESIAN_POINT ( 'NONE',  ( 0.2867679344610366554, 0.2867679344610366554, -2.181777845965566343 ) ) ;
#32347=CARTESIAN_POINT ( 'NONE',  ( -0.3917322834645670104, -7.196005306013484475E-17, -2.171259842519685179 ) ) ;
#32351=CARTESIAN_POINT ( 'NONE',  ( -0.03757601356356682354, 0.4709442531824372113, -2.755905511811023612 ) ) ;
#32352=CARTESIAN_POINT ( 'NONE',  ( 0.2925321140481931814, -0.2925321140481931259, -2.694881889763779625 ) ) ;
#32354=CARTESIAN_POINT ( 'NONE',  ( 0.3460692066303959202, 0.1998031496062993295, -1.391076115485564424 ) ) ;
#32356=CARTESIAN_POINT ( 'NONE',  ( -0.3392501089628019995, 0.1958661417322831999, -0.02298519504693102150 ) ) ;
#32368=CARTESIAN_POINT ( 'NONE',  ( -0.3392501089628019995, 0.1958661417322832277, -0.1758530183727033402 ) ) ;
#32370=ORIENTED_EDGE ( 'NONE', *, *, #23484, .F. ) ;
#32371=CARTESIAN_POINT ( 'NONE',  ( -0.1058382717557503211, 0.3949938075777409408, -0.4790026246719162328 ) ) ;
#32378=CARTESIAN_POINT ( 'NONE',  ( 0.1049643490035304799, -0.3917322834645670104, -1.656843462763466723 ) ) ;
#32384=VECTOR ( 'NONE', #60864, 39.37007874015748143 ) ;
#32385=CARTESIAN_POINT ( 'NONE',  ( 0.1070741851644054915, -0.3996062992125986035, -1.345144356955380704 ) ) ;
#32387=CARTESIAN_POINT ( 'NONE',  ( -0.1070741851644051862, -0.3996062992125986590, -0.6213910761154856077 ) ) ;
#32388=CARTESIAN_POINT ( 'NONE',  ( -0.1070741851644056997, 0.3996062992125984925, 0.07414698162729654873 ) ) ;
#32390=CARTESIAN_POINT ( 'NONE',  ( 0.2925321140481932369, -0.2925321140481932369, -2.775590551181101429 ) ) ;
#32391=CARTESIAN_POINT ( 'NONE',  ( -0.1049643490035307020, 0.3917322834645669549, -1.666010498687664043 ) ) ;
#32397=CARTESIAN_POINT ( 'NONE',  ( 0.4724409448818896462, 0.1265901696524990294, -1.461286089238844843 ) ) ;
#32400=CARTESIAN_POINT ( 'NONE',  ( -0.3420746716998662729, 0.1974969037888702206, -1.205380577427821454 ) ) ;
#32411=CARTESIAN_POINT ( 'NONE',  ( -0.1070741851644051862, -0.3996062992125986590, -2.196194225721784576 ) ) ;
#32414=CARTESIAN_POINT ( 'NONE',  ( -0.1958661417322834497, -0.3392501089628018884, -1.720453125163043051 ) ) ;
#32422=CARTESIAN_POINT ( 'NONE',  ( 0.3458507752293908943, 0.3458507752293908943, -2.342519685039369914 ) ) ;
#32427=CARTESIAN_POINT ( 'NONE',  ( -0.1958661417322834220, -0.3392501089628018884, -1.567585301837270295 ) ) ;
#32436=CARTESIAN_POINT ( 'NONE',  ( -0.4091458600556402980, -0.2362204724409451284, -2.572178477690288734 ) ) ;
#32448=CARTESIAN_POINT ( 'NONE',  ( -0.3392501089628017219, -0.1958661417322836718, -2.406824146981627166 ) ) ;
#32451=CARTESIAN_POINT ( 'NONE',  ( 5.785732909357575061E-17, -0.4724409448818898682, -0.7086614173228346081 ) ) ;
#32452=CARTESIAN_POINT ( 'NONE',  ( 0.1070741851644054915, -0.3996062992125986035, -0.08530183727034119923 ) ) ;
#32455=CARTESIAN_POINT ( 'NONE',  ( 0.3917322834645670104, -0.1049643490035303411, -1.678477690288713964 ) ) ;
#32459=CARTESIAN_POINT ( 'NONE',  ( -0.1265901696524986964, -0.4724409448818899238, -2.749343832020996636 ) ) ;
#32466=CARTESIAN_POINT ( 'NONE',  ( -0.3392501089628018329, -0.1958661417322836440, -1.234888820701100398 ) ) ;
#32473=CARTESIAN_POINT ( 'NONE',  ( -0.3917322834645671770, 0.1049643490035302024, -2.549231914207035654 ) ) ;
#32481=CARTESIAN_POINT ( 'NONE',  ( -0.1958661417322836718, 0.3392501089628017219, -1.830052493438320216 ) ) ;
#32497=CARTESIAN_POINT ( 'NONE',  ( 0.4724409448818897572, -0.1265901696524988906, -0.3458005249343831244 ) ) ;
#32500=CARTESIAN_POINT ( 'NONE',  ( 4.893765752498283308E-17, -0.3996062992125985480, -2.832677165354331006 ) ) ;
#32506=CARTESIAN_POINT ( 'NONE',  ( 0.3949938075777409408, -0.1058382717557499186, 0.1266404199475065773 ) ) ;
#32514=CARTESIAN_POINT ( 'NONE',  ( -0.3996062992125986590, 0.1070741851644051723, -1.054461942257217899 ) ) ;
#32516=CARTESIAN_POINT ( 'NONE',  ( 0.1049643490035303689, 0.3917322834645670104, -0.7729658792650916377 ) ) ;
#32518=CARTESIAN_POINT ( 'NONE',  ( -0.4724409448818898682, -8.678599364036362592E-17, -1.141732283464566899 ) ) ;
#32531=CARTESIAN_POINT ( 'NONE',  ( -1.157146581871515012E-16, 0.4724409448818898682, -2.596456692913385655 ) ) ;
#32549=CARTESIAN_POINT ( 'NONE',  ( -0.3460692066303960868, 0.1998031496062990242, -0.4986876640419947715 ) ) ;
#32550=CARTESIAN_POINT ( 'NONE',  ( 0.2925321140481932369, -0.2925321140481931814, -2.852362204724409711 ) ) ;
#32555=CARTESIAN_POINT ( 'NONE',  ( 0.1070741851644054915, -0.3996062992125986035, -2.604986876640420057 ) ) ;
#32556=CARTESIAN_POINT ( 'NONE',  ( -0.3420746716998661618, 0.1974969037888702206, -2.073490813648294129 ) ) ;
#32557=CARTESIAN_POINT ( 'NONE',  ( 0.3392501089628018884, -0.1958661417322834220, -0.5695538057742781657 ) ) ;
#32559=CARTESIAN_POINT ( 'NONE',  ( 0.3917322834645670104, 2.398668435337828261E-17, -1.055118110236220375 ) ) ;
#32561=CARTESIAN_POINT ( 'NONE',  ( 0.3392501089628018884, -0.1958661417322834220, -1.199475065616797842 ) ) ;
#32564=CARTESIAN_POINT ( 'NONE',  ( 0.2867679344610365999, 0.2867679344610365999, 0.09713217667422754942 ) ) ;
#32569=CARTESIAN_POINT ( 'NONE',  ( -0.3458507752293906723, -0.3458507752293910609, -2.736220472440944018 ) ) ;
#32570=CARTESIAN_POINT ( 'NONE',  ( -9.787531504996567848E-17, 0.3996062992125986035, -2.519685039370078705 ) ) ;
#32571=CARTESIAN_POINT ( 'NONE',  ( 0.3917322834645670659, 2.398668435337828261E-17, -1.217210916831708012 ) ) ;
#32578=CARTESIAN_POINT ( 'NONE',  ( 0.2867679344610365999, -0.2867679344610365444, -0.02559055118110245899 ) ) ;
#32586=CARTESIAN_POINT ( 'NONE',  ( -0.1504864506472308738, -0.3622863298698439927, -1.929133858267717549 ) ) ;
#32587=CARTESIAN_POINT ( 'NONE',  ( -0.3917322834645670104, -7.196005306013484475E-17, -1.921259842519684957 ) ) ;
#32588=CARTESIAN_POINT ( 'NONE',  ( -0.2867679344610365999, 0.2867679344610364889, -2.846456692913385655 ) ) ;
#32590=CARTESIAN_POINT ( 'NONE',  ( 4.893765752498283924E-17, -0.3996062992125986035, 0.07874015748031494566 ) ) ;
#32591=ORIENTED_EDGE ( 'NONE', *, *, #13980, .T. ) ;
#32594=CARTESIAN_POINT ( 'NONE',  ( 0.1998031496062994405, -0.3460692066303958092, -1.981627296587926690 ) ) ;
#32598=CARTESIAN_POINT ( 'NONE',  ( 0.1958661417322836440, -0.3392501089628017219, -0.9639107611548557442 ) ) ;
#32608=CARTESIAN_POINT ( 'NONE',  ( -0.1265901696524993347, 0.4724409448818896462, -2.683727034120734878 ) ) ;
#32615=CARTESIAN_POINT ( 'NONE',  ( -0.1265901696524986964, -0.4724409448818899238, -2.668635170603674833 ) ) ;
#32618=CARTESIAN_POINT ( 'NONE',  ( -0.1958661417322836440, 0.3392501089628016664, -0.8805581120396831496 ) ) ;
#32621=CARTESIAN_POINT ( 'NONE',  ( -0.2867679344610366554, 0.2867679344610365444, -1.206692913385826849 ) ) ;
#32626=CARTESIAN_POINT ( 'NONE',  ( -0.1958661417322834220, -0.3392501089628018884, -2.577427821522309426 ) ) ;
#32630=CARTESIAN_POINT ( 'NONE',  ( -0.1265901696524993347, 0.4724409448818895907, -1.185695538057742526 ) ) ;
#32643=CARTESIAN_POINT ( 'NONE',  ( 0.3460692066303959202, -0.1998031496062991630, -2.386482939632545985 ) ) ;
#32647=CARTESIAN_POINT ( 'NONE',  ( 0.2925321140481932369, -0.2925321140481931814, -1.907480314960629642 ) ) ;
#32653=CARTESIAN_POINT ( 'NONE',  ( -0.3460692066303957537, -0.1998031496062994405, -1.074146981627296604 ) ) ;
#32654=CARTESIAN_POINT ( 'NONE',  ( -0.2925321140481930704, -0.2925321140481933480, -1.003937007874015741 ) ) ;
#32655=CARTESIAN_POINT ( 'NONE',  ( -0.3949938075777409963, -7.255918531996591613E-17, -0.5118110236220473341 ) ) ;
#32661=CARTESIAN_POINT ( 'NONE',  ( -0.2891555358219909388, -0.2891555358219912164, -1.395669291338582418 ) ) ;
#32666=CARTESIAN_POINT ( 'NONE',  ( -0.1265901696524993347, 0.4724409448818895907, -1.738845144356955696 ) ) ;
#32667=CARTESIAN_POINT ( 'NONE',  ( 0.1998031496062994405, -0.3460692066303958092, -2.611548556430446144 ) ) ;
#32675=CARTESIAN_POINT ( 'NONE',  ( 0.3917322834645669549, 2.398668435337827645E-17, -1.930426878443882943 ) ) ;
#32676=CARTESIAN_POINT ( 'NONE',  ( -0.3996062992125985480, -7.340648628747423112E-17, -2.793307086614173151 ) ) ;
#32682=CARTESIAN_POINT ( 'NONE',  ( 0.3917322834645670104, -0.1049643490035303411, -1.363517060367453793 ) ) ;
#32685=CARTESIAN_POINT ( 'NONE',  ( 0.3420746716998660508, -0.1974969037888703871, -1.679790026246719359 ) ) ;
#32686=ORIENTED_EDGE ( 'NONE', *, *, #32099, .T. ) ;
#32690=CARTESIAN_POINT ( 'NONE',  ( 0.3460692066303959202, 0.1998031496062993295, -0.1312335958005249603 ) ) ;
#32694=FILL_AREA_STYLE ('',( #59617 ) ) ;
#32696=CARTESIAN_POINT ( 'NONE',  ( -0.3392501089628019995, 0.1958661417322832277, 0.2040682414698161695 ) ) ;
#32699=CARTESIAN_POINT ( 'NONE',  ( -0.1049643490035307020, 0.3917322834645669549, -0.4061679790026246351 ) ) ;
#32707=CARTESIAN_POINT ( 'NONE',  ( 0.3996062992125984925, 0.1070741851644054637, -1.933727034120735100 ) ) ;
#32712=CARTESIAN_POINT ( 'NONE',  ( -0.4724409448818899238, 0.1265901696524986686, -0.6627296587926508886 ) ) ;
#32714=CARTESIAN_POINT ( 'NONE',  ( 4.797336870675656522E-17, -0.3917322834645670104, -0.2283464566929133410 ) ) ;
#32715=CARTESIAN_POINT ( 'NONE',  ( 0.3917322834645669549, 0.1049643490035304660, -1.941601049868766582 ) ) ;
#32719=CARTESIAN_POINT ( 'NONE',  ( 0.4724409448818896462, 0.1265901696524990294, -2.563648293963254776 ) ) ;
#32721=CARTESIAN_POINT ( 'NONE',  ( 0.4724409448818898682, 2.892866454678787531E-17, -1.139763779527559029 ) ) ;
#32724=CARTESIAN_POINT ( 'NONE',  ( -0.1974969037888704149, -0.3420746716998661063, -2.662073490813648746 ) ) ;
#32726=CARTESIAN_POINT ( 'NONE',  ( 4.797336870675656522E-17, -0.3917322834645670104, -0.1633858267716536417 ) ) ;
#32732=CARTESIAN_POINT ( 'NONE',  ( -0.1958661417322836718, 0.3392501089628017219, -1.580052493438320216 ) ) ;
#32735=CARTESIAN_POINT ( 'NONE',  ( 0.2362204724409449064, 0.4091458600556404646, -0.06364829396325459576 ) ) ;
#32737=CARTESIAN_POINT ( 'NONE',  ( -0.4724409448818908119, 0.1265901696524971698, -1.054461942257217899 ) ) ;
#32749=CARTESIAN_POINT ( 'NONE',  ( -0.2925321140481930149, -0.2925321140481933480, -1.080708661417322691 ) ) ;
#32750=CARTESIAN_POINT ( 'NONE',  ( -0.1049643490035307020, 0.3917322834645669549, -2.610892388451443225 ) ) ;
#32759=CARTESIAN_POINT ( 'NONE',  ( -9.787531504996567848E-17, 0.3996062992125986035, 0.1574803149606299191 ) ) ;
#32760=CARTESIAN_POINT ( 'NONE',  ( -0.2867679344610367109, 0.2867679344610365444, -2.536108554626983480 ) ) ;
#32766=CARTESIAN_POINT ( 'NONE',  ( 0.1049643490035304938, -0.3917322834645669549, -1.902230971128608727 ) ) ;
#32773=CARTESIAN_POINT ( 'NONE',  ( -0.1070741851644051862, -0.3996062992125987146, -1.332020997375328086 ) ) ;
#32775=CARTESIAN_POINT ( 'NONE',  ( -0.1958661417322834220, -0.3392501089628018884, -2.892388451443569153 ) ) ;
#32789=CARTESIAN_POINT ( 'NONE',  ( -0.1049643490035302024, -0.3917322834645671215, -0.3792650918635169233 ) ) ;
#32792=CARTESIAN_POINT ( 'NONE',  ( 0.3949938075777409408, 0.1058382717557500574, -0.7545931758530185496 ) ) ;
#32793=ORIENTED_EDGE ( 'NONE', *, *, #13910, .T. ) ;
#32804=CARTESIAN_POINT ( 'NONE',  ( 0.3917322834645670104, -0.1049643490035303411, -2.873359580052493811 ) ) ;
#32808=CARTESIAN_POINT ( 'NONE',  ( 0.1998031496062994405, -0.3460692066303958092, -1.194225721784776928 ) ) ;
#32810=CARTESIAN_POINT ( 'NONE',  ( -0.1070741851644051862, -0.3996062992125986590, -0.7788713910761155823 ) ) ;
#32811=CARTESIAN_POINT ( 'NONE',  ( -0.3996062992125986590, 0.1070741851644051723, -0.1095800524934383291 ) ) ;
#32813=CARTESIAN_POINT ( 'NONE',  ( -0.3996062992125986035, -7.340648628747425578E-17, -2.716535433070865757 ) ) ;
#32814=CARTESIAN_POINT ( 'NONE',  ( -0.1049643490035302024, -0.3917322834645671215, -2.046587926509185973 ) ) ;
#32820=CARTESIAN_POINT ( 'NONE',  ( 0.4091458600556404646, -0.2362204724409448231, -1.599081364829396223 ) ) ;
#32823=CARTESIAN_POINT ( 'NONE',  ( -0.1058382717557503072, 0.3949938075777408852, -1.500656167979002253 ) ) ;
#32833=CARTESIAN_POINT ( 'NONE',  ( -0.1998031496062991630, -0.3460692066303959202, -2.032152230971128848 ) ) ;
#32835=CARTESIAN_POINT ( 'NONE',  ( 0.1958661417322836162, -0.3392501089628018329, -1.904180159283777485 ) ) ;
#32847=CARTESIAN_POINT ( 'NONE',  ( -0.3996062992125984925, -0.1070741851644056858, 0.03477690288713909672 ) ) ;
#32849=CARTESIAN_POINT ( 'NONE',  ( 0.1958661417322834775, 0.3392501089628018884, -1.488845144356955252 ) ) ;
#32871=CARTESIAN_POINT ( 'NONE',  ( 0.2867679344610366554, 0.2867679344610366554, -2.649606299212598604 ) ) ;
#32874=CARTESIAN_POINT ( 'NONE',  ( -0.4091458600556402980, -0.2362204724409451284, -0.6824146981627295938 ) ) ;
#32875=CARTESIAN_POINT ( 'NONE',  ( 4.893765752498283924E-17, -0.3996062992125986035, -0.07874015748031498729 ) ) ;
#32878=CARTESIAN_POINT ( 'NONE',  ( 0.2867679344610365999, -0.2867679344610365444, -1.980314960629921073 ) ) ;
#32879=EDGE_LOOP ( 'NONE', ( #29562, #57097, #2280, #37741, #33457, #71924, #60757, #11681, #60029, #50591, #73924, #53904, #503, #46141 ) ) ;
#32882=CARTESIAN_POINT ( 'NONE',  ( -0.006307039255731988932, 0.3948371832379762858, -2.755905511811026720 ) ) ;
#32889=CARTESIAN_POINT ( 'NONE',  ( -0.1049643490035301746, -0.3917322834645670659, -0.9396132301499194872 ) ) ;
#32897=CARTESIAN_POINT ( 'NONE',  ( -0.1958661417322833942, -0.3392501089628018884, -2.582040313157166977 ) ) ;
#32899=VERTEX_POINT ( 'NONE', #33443 ) ;
#32906=CARTESIAN_POINT ( 'NONE',  ( 0.1049643490035303689, 0.3917322834645670104, -1.652887139107611425 ) ) ;
#32922=CARTESIAN_POINT ( 'NONE',  ( -0.3458507752293909498, 0.3458507752293907833, -0.09645669291338582196 ) ) ;
#32926=CARTESIAN_POINT ( 'NONE',  ( -0.2891555358219909388, -0.2891555358219912164, 0.02165354330708659999 ) ) ;
#32931=CARTESIAN_POINT ( 'NONE',  ( -0.2891555358219911054, 0.2891555358219909388, 0.06102362204724409017 ) ) ;
#32938=CARTESIAN_POINT ( 'NONE',  ( -0.3460692066303960313, 0.1998031496062989965, -0.7329396325459317518 ) ) ;
#32940=CARTESIAN_POINT ( 'NONE',  ( 4.797336870675656522E-17, -0.3917322834645670104, -0.7007874015748030150 ) ) ;
#32942=CARTESIAN_POINT ( 'NONE',  ( -0.4091458600556402980, -0.2362204724409451284, -0.4442257217847768724 ) ) ;
#32954=CARTESIAN_POINT ( 'NONE',  ( -0.1265901696524986964, -0.4724409448818899238, -2.668635170603674833 ) ) ;
#32970=CARTESIAN_POINT ( 'NONE',  ( -0.2925321140481932369, 0.2925321140481931814, -0.3346456692913385433 ) ) ;
#32976=CARTESIAN_POINT ( 'NONE',  ( 0.3460692066303959202, 0.1998031496062993295, -2.650918635170603554 ) ) ;
#32977=CARTESIAN_POINT ( 'NONE',  ( -0.1058382717557503211, 0.3949938075777409408, -2.053805774278215868 ) ) ;
#32978=CARTESIAN_POINT ( 'NONE',  ( 0.1958661417322834775, 0.3392501089628018884, -0.4514435695538057125 ) ) ;
#32980=CARTESIAN_POINT ( 'NONE',  ( -0.3392501089628017219, -0.1958661417322836718, -0.9895013123359579499 ) ) ;
#32982=CARTESIAN_POINT ( 'NONE',  ( 0.1049643490035304938, -0.3917322834645669549, -1.179790026246718915 ) ) ;
#32984=CARTESIAN_POINT ( 'NONE',  ( 0.3949938075777409408, -0.1058382717557499186, -2.865485564304462329 ) ) ;
#32990=CARTESIAN_POINT ( 'NONE',  ( -0.3996062992125987146, 0.1070741851644051862, -2.709973753280840114 ) ) ;
#32991=CARTESIAN_POINT ( 'NONE',  ( -0.1049643490035302301, -0.3917322834645671770, -1.171279158301524292 ) ) ;
#32996=CARTESIAN_POINT ( 'NONE',  ( -0.3392501089628017219, -0.1958661417322836718, -0.4520997375328084655 ) ) ;
#33004=CARTESIAN_POINT ( 'NONE',  ( 0.2316922116746869542, -0.3165741174733261998, -1.929133858267716439 ) ) ;
#33005=CARTESIAN_POINT ( 'NONE',  ( -0.2867679344610365999, 0.2867679344610364889, -1.744094488188976610 ) ) ;
#33007=CARTESIAN_POINT ( 'NONE',  ( 0.1070741851644054915, -0.3996062992125986035, 0.07217847769028869209 ) ) ;
#33011=CARTESIAN_POINT ( 'NONE',  ( -0.4724409448818898682, -8.678599364036362592E-17, -1.929133858267716439 ) ) ;
#33014=CARTESIAN_POINT ( 'NONE',  ( -0.1958661417322834220, -0.3392501089628018884, -0.9376640419947508409 ) ) ;
#33017=CARTESIAN_POINT ( 'NONE',  ( -0.3996062992125986035, -1.273259842764937629E-12, -1.929133858267794599 ) ) ;
#33021=EDGE_CURVE ( 'NONE', #12829, #59707, #8125, .T. ) ;
#33025=CARTESIAN_POINT ( 'NONE',  ( 0.3458507752293908943, 0.3458507752293908943, -2.657480314960630086 ) ) ;
#33026=FACE_OUTER_BOUND ( 'NONE', #64, .T. ) ;
#33036=CARTESIAN_POINT ( 'NONE',  ( -0.3917322834645669549, -7.196005306013483243E-17, -0.9068048311997882749 ) ) ;
#33039=CARTESIAN_POINT ( 'NONE',  ( 0.2867679344610366554, 0.2867679344610366554, -1.167322834645669438 ) ) ;
#33045=CARTESIAN_POINT ( 'NONE',  ( 0.1958661417322836718, -0.3392501089628017219, 0.06887832201343642435 ) ) ;
#33049=CARTESIAN_POINT ( 'NONE',  ( 0.2362204724409449064, 0.4091458600556404646, -1.323490813648294129 ) ) ;
#33059=CARTESIAN_POINT ( 'NONE',  ( 0.4724409448818898682, 2.892866454678787531E-17, -2.084645669291338432 ) ) ;
#33066=CARTESIAN_POINT ( 'NONE',  ( -0.1998031496062994405, 0.3460692066303957537, -2.609580052493438274 ) ) ;
#33071=CARTESIAN_POINT ( 'NONE',  ( 0.3460692066303958092, 0.1998031496062993018, -1.940288713910761409 ) ) ;
#33079=CARTESIAN_POINT ( 'NONE',  ( -0.2925321140481932369, 0.2925321140481930704, -1.041338582677165281 ) ) ;
#33080=CARTESIAN_POINT ( 'NONE',  ( 0.1998031496062994405, -0.3460692066303958092, -1.194225721784776928 ) ) ;
#33081=CARTESIAN_POINT ( 'NONE',  ( -0.3420746716998659953, -0.1974969037888706647, -0.6824146981627297048 ) ) ;
#33087=CARTESIAN_POINT ( 'NONE',  ( 0.1058382717557500852, -0.3949938075777408852, -1.894356955380577245 ) ) ;
#33092=CARTESIAN_POINT ( 'NONE',  ( 0.3458507752293908943, 0.3458507752293908943, -2.027559055118109743 ) ) ;
#33100=CARTESIAN_POINT ( 'NONE',  ( 0.1049643490035304522, -0.3917322834645668994, -2.370059424375641211 ) ) ;
#33106=CARTESIAN_POINT ( 'NONE',  ( 0.2867679344610365999, 0.2867679344610365999, 0.09251968503937001154 ) ) ;
#33107=SHAPE_REPRESENTATION ( 'Independent Actuating Lead Screws', ( #22098 ), #649 ) ;
#33109=CARTESIAN_POINT ( 'NONE',  ( 0.3392501089628018329, 0.1958661417322835607, -1.698162729658792891 ) ) ;
#33112=CARTESIAN_POINT ( 'NONE',  ( -0.1058382717557503211, 0.3949938075777409408, -1.738845144356955696 ) ) ;
#33114=DIRECTION ( 'NONE',  ( 1.000000000000000000, 0.000000000000000000, 0.000000000000000000 ) ) ;
#33117=CARTESIAN_POINT ( 'NONE',  ( -0.1070741851644051862, -0.3996062992125987146, -0.7020997375328084100 ) ) ;
#33125=CARTESIAN_POINT ( 'NONE',  ( 0.1958661417322834775, 0.3392501089628018884, -0.5439632545931759600 ) ) ;
#33132=CARTESIAN_POINT ( 'NONE',  ( -0.3996062992125986590, 0.1070741851644051723, -2.156824146981627166 ) ) ;
#33136=CARTESIAN_POINT ( 'NONE',  ( 0.2362204724409449064, 0.4091458600556404646, -1.404199475065616820 ) ) ;
#33138=CARTESIAN_POINT ( 'NONE',  ( 0.2867679344610365999, 0.2867679344610365999, -0.4448818897637794589 ) ) ;
#33140=CARTESIAN_POINT ( 'NONE',  ( 0.1958661417322836440, -0.3392501089628017219, -2.066272965879265122 ) ) ;
#33146=CARTESIAN_POINT ( 'NONE',  ( -0.3460692066303957537, -0.1998031496062994405, 0.02821522309711283621 ) ) ;
#33151=CARTESIAN_POINT ( 'NONE',  ( -0.3949938075777408852, -0.1058382717557502933, -2.642388451443569597 ) ) ;
#33153=CARTESIAN_POINT ( 'NONE',  ( 4.797336870675656522E-17, -0.3917322834645670104, -0.005905511811023714773 ) ) ;
#33158=CARTESIAN_POINT ( 'NONE',  ( -0.3392501089628019995, 0.1958661417322832277, -1.750656167979002698 ) ) ;
#33162=CARTESIAN_POINT ( 'NONE',  ( -0.4091458600556405756, 0.2362204724409446288, 0.05446194225721784354 ) ) ;
#33175=CARTESIAN_POINT ( 'NONE',  ( -0.1070741851644056997, 0.3996062992125984925, -1.185695538057742526 ) ) ;
#33176=CARTESIAN_POINT ( 'NONE',  ( 0.3917322834645670104, 2.398668435337828261E-17, -2.879921259842519454 ) ) ;
#33185=CARTESIAN_POINT ( 'NONE',  ( 0.1070741851644053527, 0.3996062992125986590, 0.006561679790026237087 ) ) ;
#33186=CARTESIAN_POINT ( 'NONE',  ( -0.3917322834645671770, 0.1049643490035302024, -2.549231914207035654 ) ) ;
#33192=VECTOR ( 'NONE', #54607, 39.37007874015748143 ) ;
#33194=CARTESIAN_POINT ( 'NONE',  ( -0.1958661417322834220, -0.3392501089628018884, -2.197506561679789971 ) ) ;
#33204=CARTESIAN_POINT ( 'NONE',  ( -0.3996062992125986035, -0.1070741851644056997, -1.463254593175853158 ) ) ;
#33206=CARTESIAN_POINT ( 'NONE',  ( 0.3392501089628018329, 0.1958661417322835607, -0.1279720716873509745 ) ) ;
#33217=EDGE_CURVE ( 'NONE', #18027, #2500, #22920, .T. ) ;
#33219=CARTESIAN_POINT ( 'NONE',  ( 0.2867679344610365999, 0.2867679344610365999, -0.2874015748031494843 ) ) ;
#33222=CARTESIAN_POINT ( 'NONE',  ( -0.1058382717557497937, -0.3949938075777411628, -0.5446194225721784354 ) ) ;
#33238=CARTESIAN_POINT ( 'NONE',  ( -0.1998031496062991907, -0.3460692066303959757, -1.482939632545931863 ) ) ;
#33240=CARTESIAN_POINT ( 'NONE',  ( -0.3460692066303957537, -0.1998031496062994405, -0.6017060367454067915 ) ) ;
#33241=CARTESIAN_POINT ( 'NONE',  ( 0.1070741851644053388, 0.3996062992125986035, -0.07020997375328086321 ) ) ;
#33243=CARTESIAN_POINT ( 'NONE',  ( 0.3996062992125986035, 2.446882876249141962E-17, -2.795275590551181022 ) ) ;
#33245=CARTESIAN_POINT ( 'NONE',  ( -9.594673741351313045E-17, 0.3917322834645670104, -2.289370078740157410 ) ) ;
#33251=CARTESIAN_POINT ( 'NONE',  ( 0.4724409448818896462, 0.1265901696524990294, -1.303805774278215202 ) ) ;
#33254=CARTESIAN_POINT ( 'NONE',  ( 0.1058382717557499880, 0.3949938075777409408, -1.330052493438319994 ) ) ;
#33264=CARTESIAN_POINT ( 'NONE',  ( -0.2925321140481930149, -0.2925321140481933480, -2.340551181102362488 ) ) ;
#33268=CARTESIAN_POINT ( 'NONE',  ( 0.1049643490035303689, 0.3917322834645668994, -2.120715592354644130 ) ) ;
#33280=CARTESIAN_POINT ( 'NONE',  ( 0.3460692066303958092, 0.1998031496062993018, 0.1069553805774278027 ) ) ;
#33282=CARTESIAN_POINT ( 'NONE',  ( -0.3392501089628019995, 0.1958661417322832277, -1.213254593175852936 ) ) ;
#33290=EDGE_CURVE ( 'NONE', #56483, #42415, #29197, .T. ) ;
#33293=CARTESIAN_POINT ( 'NONE',  ( -0.4724409448818898682, -8.678599364036362592E-17, -2.559055118110236560 ) ) ;
#33304=CARTESIAN_POINT ( 'NONE',  ( 0.3917322834645670104, -0.1049643490035303273, -2.465879265091862838 ) ) ;
#33307=CARTESIAN_POINT ( 'NONE',  ( -0.4091458600556402980, -0.2362204724409451284, -0.8398950131233595684 ) ) ;
#33308=CARTESIAN_POINT ( 'NONE',  ( 0.2925321140481932369, -0.2925321140481932369, -0.09842519685039373412 ) ) ;
#33311=CARTESIAN_POINT ( 'NONE',  ( 0.2867679344610365999, 0.2867679344610365999, -1.704724409448818978 ) ) ;
#33322=CARTESIAN_POINT ( 'NONE',  ( -0.2867679344610364334, -0.2867679344610368219, -1.083970185530496844 ) ) ;
#33328=CARTESIAN_POINT ( 'NONE',  ( 0.3917322834645670659, 2.398668435337828261E-17, -2.319573121556117279 ) ) ;
#33337=CARTESIAN_POINT ( 'NONE',  ( 0.3392501089628018884, -0.1958661417322834220, -1.764435695538057791 ) ) ;
#33350=CARTESIAN_POINT ( 'NONE',  ( -0.4091458600556402980, -0.2362204724409451284, -0.1292650918635170620 ) ) ;
#33353=CARTESIAN_POINT ( 'NONE',  ( 0.1058382717557500852, -0.3949938075777408852, -0.1620734908136483021 ) ) ;
#33358=CARTESIAN_POINT ( 'NONE',  ( 0.1974969037888704704, 0.3420746716998660508, -0.06364829396325460964 ) ) ;
#33365=CARTESIAN_POINT ( 'NONE',  ( 0.1070741851644054776, -0.3996062992125984925, -0.9494750656167976199 ) ) ;
#33367=CARTESIAN_POINT ( 'NONE',  ( 4.797336870675656522E-17, -0.3917322834645670104, -0.5433070866141732624 ) ) ;
#33382=CARTESIAN_POINT ( 'NONE',  ( 0.1265901696524989462, 0.4724409448818897572, -2.747375328083988766 ) ) ;
#33399=CARTESIAN_POINT ( 'NONE',  ( -0.1998031496062994683, 0.3460692066303958092, -0.8005249343832020470 ) ) ;
#33404=CARTESIAN_POINT ( 'NONE',  ( -0.2925321140481930704, -0.2925321140481933480, -2.421259842519684735 ) ) ;
#33405=CARTESIAN_POINT ( 'NONE',  ( 0.2891555358219910499, 0.2891555358219910499, -1.870078740157480324 ) ) ;
#33406=CARTESIAN_POINT ( 'NONE',  ( 4.797336870675656522E-17, -0.3917322834645670104, -0.7007874015748030150 ) ) ;
#33407=CARTESIAN_POINT ( 'NONE',  ( -0.2867679344610366554, 0.2867679344610365444, -0.9566929133858265155 ) ) ;
#33409=CARTESIAN_POINT ( 'NONE',  ( -0.1958661417322836718, 0.3392501089628017219, -0.9501312335958004285 ) ) ;
#33411=CARTESIAN_POINT ( 'NONE',  ( -0.1958661417322836440, 0.3392501089628016664, 0.06432377772409630934 ) ) ;
#33417=CARTESIAN_POINT ( 'NONE',  ( 0.1070741851644053527, 0.3996062992125986590, -2.513123359580052174 ) ) ;
#33418=CARTESIAN_POINT ( 'NONE',  ( -9.594673741351313045E-17, 0.3917322834645670659, -1.414061310532495286 ) ) ;
#33425=CARTESIAN_POINT ( 'NONE',  ( 0.3917322834645670104, -0.1049643490035303411, -0.3536745406824148286 ) ) ;
#33433=CARTESIAN_POINT ( 'NONE',  ( -0.3726288332202236653, -0.1208384647423932784, -1.929133858267952473 ) ) ;
#33434=CARTESIAN_POINT ( 'NONE',  ( 0.1958661417322836440, -0.3392501089628017219, -2.131233595800524849 ) ) ;
#33437=CARTESIAN_POINT ( 'NONE',  ( 0.3996062992125986590, -0.1070741851644053111, -0.4265091863517060933 ) ) ;
#33443=CARTESIAN_POINT ( 'NONE',  ( 0.4724409448818898682, 2.892866454678787531E-17, -2.714566929133858331 ) ) ;
#33444=CARTESIAN_POINT ( 'NONE',  ( 0.2867679344610365999, 0.2867679344610365999, -1.009842519685039353 ) ) ;
#33446=CARTESIAN_POINT ( 'NONE',  ( -0.3790285851608742318, -0.1011035889004742866, -1.929133858267716439 ) ) ;
#33449=ORIENTED_EDGE ( 'NONE', *, *, #19165, .T. ) ;
#33457=ORIENTED_EDGE ( 'NONE', *, *, #82059, .T. ) ;
#33462=CARTESIAN_POINT ( 'NONE',  ( 0.2867679344610365999, -0.2867679344610365999, -0.9658599493100242794 ) ) ;
#33465=CARTESIAN_POINT ( 'NONE',  ( -0.3392501089628019995, 0.1958661417322832277, -1.213254593175852936 ) ) ;
#33471=CARTESIAN_POINT ( 'NONE',  ( 0.2867679344610366554, -0.2867679344610365999, 0.06231664222341019160 ) ) ;
#33475=CARTESIAN_POINT ( 'NONE',  ( 0.3458507752293908943, -0.3458507752293908943, -1.435039370078740051 ) ) ;
#33491=CARTESIAN_POINT ( 'NONE',  ( -0.2891555358219911054, 0.2891555358219909388, 0.2185039370078739884 ) ) ;
#33495=CARTESIAN_POINT ( 'NONE',  ( 0.3996062992125986035, -0.1070741851644052972, -1.763123359580052174 ) ) ;
#33500=CARTESIAN_POINT ( 'NONE',  ( 0.2925321140481931814, 0.2925321140481931814, -1.001968503937007871 ) ) ;
#33501=CARTESIAN_POINT ( 'NONE',  ( 0.2925321140481932369, 0.2925321140481932369, -1.397637795275590067 ) ) ;
#33502=CARTESIAN_POINT ( 'NONE',  ( -0.3420746716998661618, 0.1974969037888702206, -0.6561679790026245795 ) ) ;
#33507=CARTESIAN_POINT ( 'NONE',  ( -0.2891555358219909388, -0.2891555358219912164, -1.553149606299212504 ) ) ;
#33512=CARTESIAN_POINT ( 'NONE',  ( -0.2362204724409447953, -0.4091458600556404646, -2.112860892388451539 ) ) ;
#33519=CARTESIAN_POINT ( 'NONE',  ( 0.2867679344610365999, -0.2867679344610365999, -2.540663098916323914 ) ) ;
#33525=CARTESIAN_POINT ( 'NONE',  ( -0.2867679344610365999, 0.2867679344610364889, 0.2106299212598424508 ) ) ;
#33527=CARTESIAN_POINT ( 'NONE',  ( 0.1958661417322836440, -0.3392501089628017219, -1.973753280839895208 ) ) ;
#33530=CARTESIAN_POINT ( 'NONE',  ( 0.3420746716998659953, 0.1974969037888705536, -1.863517060367453793 ) ) ;
#33535=CARTESIAN_POINT ( 'NONE',  ( 0.3460692066303959202, 0.1998031496062993295, -0.7611548556430446366 ) ) ;
#33543=CARTESIAN_POINT ( 'NONE',  ( -0.1958661417322834220, -0.3392501089628018884, -0.4652230971128609727 ) ) ;
#33553=CARTESIAN_POINT ( 'NONE',  ( 0.4724409448818898682, 2.892866454678787531E-17, -1.062992125984252079 ) ) ;
#33555=CARTESIAN_POINT ( 'NONE',  ( 0.2867679344610365999, 0.2867679344610365999, -0.2874015748031494843 ) ) ;
#33556=CARTESIAN_POINT ( 'NONE',  ( 0.3917322834645670104, 2.398668435337828261E-17, -2.407480314960630086 ) ) ;
#33560=CARTESIAN_POINT ( 'NONE',  ( -0.3996062992125986590, 0.1070741851644051723, -0.1095800524934383291 ) ) ;
#33565=CARTESIAN_POINT ( 'NONE',  ( -0.3420746716998662729, 0.1974969037888702206, -2.780183727034121866 ) ) ;
#33567=FACE_OUTER_BOUND ( 'NONE', #34132, .T. ) ;
#33572=CARTESIAN_POINT ( 'NONE',  ( 0.3917322834645670104, 2.398668435337828261E-17, -1.842519685039370136 ) ) ;
#33575=CARTESIAN_POINT ( 'NONE',  ( -0.4724409448818898682, -8.678599364036362592E-17, -0.1161417322834645827 ) ) ;
#33588=CARTESIAN_POINT ( 'NONE',  ( 4.893765752498283308E-17, -0.3996062992125985480, -0.9429133858267716439 ) ) ;
#33589=CARTESIAN_POINT ( 'NONE',  ( 4.797336870675656522E-17, -0.3917322834645670104, -2.840551181102362044 ) ) ;
#33598=CARTESIAN_POINT ( 'NONE',  ( 0.1998031496062992740, 0.3460692066303959757, -0.1443569553805774397 ) ) ;
#33599=CARTESIAN_POINT ( 'NONE',  ( -9.594673741351313045E-17, 0.3917322834645670659, -2.673903830217533972 ) ) ;
#33606=CARTESIAN_POINT ( 'NONE',  ( 0.3917322834645670104, 2.398668435337828261E-17, -2.564960629921259727 ) ) ;
#33614=CARTESIAN_POINT ( 'NONE',  ( -0.1070741851644056997, 0.3996062992125986035, -1.738845144356955696 ) ) ;
#33616=CARTESIAN_POINT ( 'NONE',  ( -0.1958661417322833942, -0.3392501089628018884, -0.5347962186689783071 ) ) ;
#33629=CARTESIAN_POINT ( 'NONE',  ( -0.3917322834645671215, 0.1049643490035301469, -0.6548556430446192955 ) ) ;
#33632=CARTESIAN_POINT ( 'NONE',  ( -0.3949938075777411628, 0.1058382717557497937, -0.8202099737532810853 ) ) ;
#33648=CARTESIAN_POINT ( 'NONE',  ( -0.3996062992125986035, -0.1070741851644056997, -1.148293963254592986 ) ) ;
#33650=CARTESIAN_POINT ( 'NONE',  ( -0.3996062992125984925, -0.1070741851644056858, -0.9101049868766404316 ) ) ;
#33651=CARTESIAN_POINT ( 'NONE',  ( -0.3996062992125986590, 0.1070741851644051723, -0.5820209973753280863 ) ) ;
#33653=CARTESIAN_POINT ( 'NONE',  ( -1.157146581871515012E-16, 0.4724409448818898682, -0.1574803149606299191 ) ) ;
#33654=CARTESIAN_POINT ( 'NONE',  ( -0.3917322834645670104, -7.196005306013484475E-17, -2.013779527559055094 ) ) ;
#33660=CARTESIAN_POINT ( 'NONE',  ( -0.4724409448818895907, -0.1265901696524993070, -2.012467191601049699 ) ) ;
#33663=CARTESIAN_POINT ( 'NONE',  ( -0.1974969037888704149, -0.3420746716998661063, -1.559711286089239035 ) ) ;
#33674=CARTESIAN_POINT ( 'NONE',  ( 0.2925321140481932369, -0.2925321140481931814, -2.379921259842520342 ) ) ;
#33675=CARTESIAN_POINT ( 'NONE',  ( -0.1958661417322834497, -0.3392501089628018884, -2.035413755084302778 ) ) ;
#33688=CARTESIAN_POINT ( 'NONE',  ( -0.1998031496062991630, -0.3460692066303959202, 0.01509186351706036204 ) ) ;
#33690=CARTESIAN_POINT ( 'NONE',  ( -0.1049643490035307020, 0.3917322834645669549, -1.351049868766404538 ) ) ;
#33695=CARTESIAN_POINT ( 'NONE',  ( -0.2952755905511810774, 3.616083068348483797E-17, -1.929133858267716661 ) ) ;
#33712=CARTESIAN_POINT ( 'NONE',  ( -0.3917322834645670104, -7.196005306013484475E-17, -2.393700787401574992 ) ) ;
#33713=CARTESIAN_POINT ( 'NONE',  ( -0.3808816823641234528, 0.09156050430092053938, -1.220472440944881942 ) ) ;
#33715=CARTESIAN_POINT ( 'NONE',  ( 0.1070741851644054915, -0.3996062992125986035, -0.2427821522309711877 ) ) ;
#33718=CARTESIAN_POINT ( 'NONE',  ( -0.3392501089628017219, -0.1958661417322836718, -1.776902887139107490 ) ) ;
#33730=CARTESIAN_POINT ( 'NONE',  ( -0.1958661417322836440, 0.3392501089628016664, -1.352999056921573295 ) ) ;
#33737=CARTESIAN_POINT ( 'NONE',  ( 0.1958661417322836718, -0.3392501089628017219, -2.450806717356642128 ) ) ;
#33745=CARTESIAN_POINT ( 'NONE',  ( -0.1049643490035302024, -0.3917322834645671215, -1.889107611548556109 ) ) ;
#33759=CARTESIAN_POINT ( 'NONE',  ( 0.4724409448818896462, 0.1265901696524990294, -0.5164041994750655507 ) ) ;
#33763=CARTESIAN_POINT ( 'NONE',  ( -0.1974969037888706924, 0.3420746716998658843, -0.2473753280839895707 ) ) ;
#33769=CARTESIAN_POINT ( 'NONE',  ( 0.2891555358219910499, 0.2891555358219910499, -0.05708661417322836301 ) ) ;
#33776=CARTESIAN_POINT ( 'NONE',  ( 0.1998031496062994128, -0.3460692066303957537, -0.9560367454068241511 ) ) ;
#33778=CARTESIAN_POINT ( 'NONE',  ( 0.3392501089628018884, -0.1958661417322834220, -0.5695538057742781657 ) ) ;
#33791=CARTESIAN_POINT ( 'NONE',  ( -0.3857547143408425749, 0.07128922432405607190, -1.220472440944881942 ) ) ;
#33793=CARTESIAN_POINT ( 'NONE',  ( -0.3458507752293906723, -0.3458507752293910609, -2.812992125984251857 ) ) ;
#33809=CARTESIAN_POINT ( 'NONE',  ( 0.3996062992125986035, 2.446882876249141962E-17, -0.5905511811023621549 ) ) ;
#33814=CARTESIAN_POINT ( 'NONE',  ( 0.3460692066303959757, -0.1998031496062991907, -2.624671916010498762 ) ) ;
#33815=CARTESIAN_POINT ( 'NONE',  ( 0.3949938075777409408, 0.1058382717557500574, -2.014435695538057569 ) ) ;
#33816=CARTESIAN_POINT ( 'NONE',  ( 0.2867679344610365999, 0.2867679344610365999, -0.6023622047244093780 ) ) ;
#33819=CARTESIAN_POINT ( 'NONE',  ( -0.1958661417322836718, 0.3392501089628017219, -1.107611548556430403 ) ) ;
#33821=CARTESIAN_POINT ( 'NONE',  ( -0.2867679344610364334, -0.2867679344610368219, 0.1758723341545424812 ) ) ;
#33827=CARTESIAN_POINT ( 'NONE',  ( -0.1998031496062991907, -0.3460692066303959757, -2.742782152230971437 ) ) ;
#33828=CARTESIAN_POINT ( 'NONE',  ( 0.2867679344610366554, -0.2867679344610365999, -1.040045562500999443 ) ) ;
#33833=CARTESIAN_POINT ( 'NONE',  ( 0.3392501089628018884, -0.1958661417322834220, -0.6620734908136483021 ) ) ;
#33842=CARTESIAN_POINT ( 'NONE',  ( 0.3758920641862648626, -0.1123167701215118386, -1.929133858267716883 ) ) ;
#33843=CARTESIAN_POINT ( 'NONE',  ( -0.3917322834645671215, 0.1049643490035301469, -1.757217847769028340 ) ) ;
#33845=CARTESIAN_POINT ( 'NONE',  ( -0.1070741851644051862, -0.3996062992125987146, -0.2296587926509186528 ) ) ;
#33852=CARTESIAN_POINT ( 'NONE',  ( -0.3917322834645670104, -7.196005306013484475E-17, -1.068897637795275690 ) ) ;
#33873=CARTESIAN_POINT ( 'NONE',  ( 0.1958661417322836162, -0.3392501089628018329, -1.116778584480628389 ) ) ;
#33882=CARTESIAN_POINT ( 'NONE',  ( 0.3392501089628018329, 0.1958661417322835607, 0.02950824327327895152 ) ) ;
#33885=CARTESIAN_POINT ( 'NONE',  ( -0.3458507752293906723, -0.3458507752293910609, -1.710629921259842812 ) ) ;
#33902=CARTESIAN_POINT ( 'NONE',  ( 0.2925321140481932369, -0.2925321140481931814, -2.852362204724409711 ) ) ;
#33907=CARTESIAN_POINT ( 'NONE',  ( -0.3460692066303960313, 0.1998031496062989965, -1.835301837270341352 ) ) ;
#33912=CARTESIAN_POINT ( 'NONE',  ( -0.3996062992125986035, 0.1070741851644051584, -1.054461942257217899 ) ) ;
#33913=CARTESIAN_POINT ( 'NONE',  ( 0.1070741851644054915, -0.3996062992125986035, -1.502624671916010346 ) ) ;
#33914=CARTESIAN_POINT ( 'NONE',  ( -0.2891555358219908833, -0.2891555358219912164, -0.6889763779527559029 ) ) ;
#33919=CARTESIAN_POINT ( 'NONE',  ( 0.1058382717557500852, -0.3949938075777408852, -1.579396325459317740 ) ) ;
#33925=CARTESIAN_POINT ( 'NONE',  ( -0.2362204724409451284, 0.4091458600556402425, -2.217847769028871596 ) ) ;
#33926=CARTESIAN_POINT ( 'NONE',  ( 0.2955417804206911248, -0.2579773093944459084, -2.755905511811021835 ) ) ;
#33927=EDGE_LOOP ( 'NONE', ( #62718, #32793, #34538 ) ) ;
#33932=CARTESIAN_POINT ( 'NONE',  ( -0.1049643490035301746, -0.3917322834645670659, -2.199455749834958951 ) ) ;
#33938=CARTESIAN_POINT ( 'NONE',  ( -0.3392501089628019995, 0.1958661417322832277, 0.2040682414698161695 ) ) ;
#33941=CARTESIAN_POINT ( 'NONE',  ( -0.1958661417322836718, 0.3392501089628017219, -1.895013123359580165 ) ) ;
#33944=CARTESIAN_POINT ( 'NONE',  ( -0.3420746716998661618, 0.1974969037888702206, -2.388451443569553856 ) ) ;
#33949=CARTESIAN_POINT ( 'NONE',  ( 0.3996062992125986590, -0.1070741851644053111, -0.4265091863517060933 ) ) ;
#33954=CARTESIAN_POINT ( 'NONE',  ( -0.2867679344610364334, -0.2867679344610367109, 0.1712598425196849850 ) ) ;
#33958=CARTESIAN_POINT ( 'NONE',  ( 0.2867679344610365999, -0.2867679344610365444, -0.8129921259842518566 ) ) ;
#33963=CARTESIAN_POINT ( 'NONE',  ( -0.1049643490035302024, -0.3917322834645671215, 0.09317585301837272294 ) ) ;
#33969=CARTESIAN_POINT ( 'NONE',  ( -0.4724409448818898682, -8.678599364036362592E-17, -1.299212598425196985 ) ) ;
#33971=CARTESIAN_POINT ( 'NONE',  ( -0.3917322834645671215, 0.1049643490035301469, -0.4973753280839895430 ) ) ;
#33972=CARTESIAN_POINT ( 'NONE',  ( -0.3392501089628017219, -0.1958661417322836718, -2.499343832020997080 ) ) ;
#33975=CARTESIAN_POINT ( 'NONE',  ( 0.3460692066303958092, 0.1998031496062993018, -0.05052493438320212332 ) ) ;
#33980=CARTESIAN_POINT ( 'NONE',  ( -0.3949938075777409963, -7.255918531996591613E-17, -2.478346456692914312 ) ) ;
#33982=CARTESIAN_POINT ( 'NONE',  ( 0.3392501089628018329, 0.1958661417322835607, -0.05839895013123368173 ) ) ;
#33987=CARTESIAN_POINT ( 'NONE',  ( -0.3917322834645671215, 0.1049643490035301469, -2.072178477690288734 ) ) ;
#33991=CARTESIAN_POINT ( 'NONE',  ( -0.4724409448818899238, 0.1265901696524986686, -0.2670603674540683037 ) ) ;
#34005=CARTESIAN_POINT ( 'NONE',  ( 0.1070741851644054776, -0.3996062992125984925, -1.421916010498687877 ) ) ;
#34006=CARTESIAN_POINT ( 'NONE',  ( 0.3917322834645669549, 0.1049643490035304660, -2.571522309711286258 ) ) ;
#34014=CARTESIAN_POINT ( 'NONE',  ( 0.3996062992125986035, 2.446882876249141962E-17, -0.1181102362204724671 ) ) ;
#34016=CARTESIAN_POINT ( 'NONE',  ( -0.3917322834645670659, -7.196005306013484475E-17, -2.398313279036432100 ) ) ;
#34022=CARTESIAN_POINT ( 'NONE',  ( -0.1049643490035302024, -0.3917322834645671215, -2.519028871391075786 ) ) ;
#34030=CARTESIAN_POINT ( 'NONE',  ( -0.3917322834645670104, -0.1049643490035307020, -0.3576308643382697383 ) ) ;
#34042=CARTESIAN_POINT ( 'NONE',  ( -0.3917322834645670104, -7.196005306013484475E-17, -0.5039370078740157410 ) ) ;
#34045=CARTESIAN_POINT ( 'NONE',  ( 0.3420746716998660508, -0.1974969037888703871, -1.049868766404199460 ) ) ;
#34056=CARTESIAN_POINT ( 'NONE',  ( -0.3458507752293906723, -0.3458507752293910609, -2.736220472440943574 ) ) ;
#34062=CARTESIAN_POINT ( 'NONE',  ( -0.3460692066303960868, 0.1998031496062990242, -1.286089238845144367 ) ) ;
#34064=CARTESIAN_POINT ( 'NONE',  ( 0.3996062992125986035, -0.1070741851644052972, -1.133202099737532720 ) ) ;
#34065=CARTESIAN_POINT ( 'NONE',  ( 0.3460692066303958092, 0.1998031496062993018, -0.6804461942257218343 ) ) ;
#34067=CARTESIAN_POINT ( 'NONE',  ( 0.2362204724409449064, 0.4091458600556404646, 0.01312335958005249326 ) ) ;
#34068=CARTESIAN_POINT ( 'NONE',  ( -0.2867679344610364334, -0.2867679344610367109, -2.190944881889763440 ) ) ;
#34074=CARTESIAN_POINT ( 'NONE',  ( -0.3458507752293909498, 0.3458507752293907833, -1.828740157480315265 ) ) ;
#34078=CARTESIAN_POINT ( 'NONE',  ( 0.3949938075777409963, 2.418639510665530743E-17, -1.612204724409448842 ) ) ;
#34084=CARTESIAN_POINT ( 'NONE',  ( -0.4724409448818898682, -8.678599364036362592E-17, -2.320866141732283783 ) ) ;
#34088=CARTESIAN_POINT ( 'NONE',  ( 0.3996062992125984925, 0.1070741851644054637, -2.563648293963254776 ) ) ;
#34089=CARTESIAN_POINT ( 'NONE',  ( -0.2867679344610366554, 0.2867679344610365444, -1.989481996554119059 ) ) ;
#34104=CARTESIAN_POINT ( 'NONE',  ( 0.1998031496062992463, 0.3460692066303959202, -0.3786089238845143923 ) ) ;
#34106=CARTESIAN_POINT ( 'NONE',  ( 0.2867679344610365999, 0.2867679344610365999, -1.482283464566929387 ) ) ;
#34115=CARTESIAN_POINT ( 'NONE',  ( -0.3996062992125986590, 0.1070741851644051723, -1.054461942257217899 ) ) ;
#34131=CARTESIAN_POINT ( 'NONE',  ( -0.1998031496062994683, 0.3460692066303958092, -0.4855643044619422644 ) ) ;
#34132=EDGE_LOOP ( 'NONE', ( #10929, #66782, #82492, #27526 ) ) ;
#34135=CARTESIAN_POINT ( 'NONE',  ( -0.3392501089628017219, -0.1958661417322836718, -2.091863517060367439 ) ) ;
#34146=CARTESIAN_POINT ( 'NONE',  ( 0.3917322834645668994, -0.1049643490035303134, -0.9789833088900768976 ) ) ;
#34152=CARTESIAN_POINT ( 'NONE',  ( -0.3392501089628017219, -0.1958661417322836995, -2.568916953577114359 ) ) ;
#34154=ORIENTED_EDGE ( 'NONE', *, *, #31271, .F. ) ;
#34161=CARTESIAN_POINT ( 'NONE',  ( -0.3917322834645669549, -0.1049643490035306603, -1.862860892388451761 ) ) ;
#34166=CARTESIAN_POINT ( 'NONE',  ( 0.3917322834645670104, -0.1049643490035303411, -2.938320209973753538 ) ) ;
#34170=CARTESIAN_POINT ( 'NONE',  ( -0.1070741851644056997, 0.3996062992125986035, -1.738845144356955696 ) ) ;
#34175=CARTESIAN_POINT ( 'NONE',  ( -0.3458507752293909498, 0.3458507752293907833, -0.5688976377952755792 ) ) ;
#34178=CARTESIAN_POINT ( 'NONE',  ( -0.2891555358219911054, 0.2891555358219909388, -0.2539370078740157410 ) ) ;
#34184=CARTESIAN_POINT ( 'NONE',  ( -0.1974969037888704149, -0.3420746716998661063, -0.2998687664041995715 ) ) ;
#34188=CARTESIAN_POINT ( 'NONE',  ( -0.4724409448818896462, -0.1265901696524993070, -0.1227034120734908362 ) ) ;
#34191=CARTESIAN_POINT ( 'NONE',  ( 0.1998031496062992463, 0.3460692066303959202, -1.480971128608923992 ) ) ;
#34193=CARTESIAN_POINT ( 'NONE',  ( -0.1049643490035307020, 0.3917322834645669549, -0.6286089238845143923 ) ) ;
#34208=CARTESIAN_POINT ( 'NONE',  ( -0.2362204724409447953, -0.4091458600556404646, -2.819553805774277944 ) ) ;
#34226=CARTESIAN_POINT ( 'NONE',  ( 0.3460692066303959202, 0.1998031496062993295, -0.7611548556430446366 ) ) ;
#34231=CARTESIAN_POINT ( 'NONE',  ( -0.3996062992125987146, 0.1070741851644051862, -2.709973753280840114 ) ) ;
#34232=CARTESIAN_POINT ( 'NONE',  ( -0.3420746716998661618, 0.1974969037888702206, -2.230971128608923770 ) ) ;
#34234=CARTESIAN_POINT ( 'NONE',  ( 4.797336870675656522E-17, -0.3917322834645670104, -1.015748031496062964 ) ) ;
#34238=CARTESIAN_POINT ( 'NONE',  ( 0.1049643490035303689, 0.3917322834645670104, -0.9304461942257216123 ) ) ;
#34240=CARTESIAN_POINT ( 'NONE',  ( -0.3392501089628019439, 0.1958661417322832554, 0.2086807331046737768 ) ) ;
#34246=CARTESIAN_POINT ( 'NONE',  ( 0.3460692066303959757, -0.1998031496062991907, -2.467191601049868677 ) ) ;
#34247=CARTESIAN_POINT ( 'NONE',  ( -0.2867679344610365444, -0.2867679344610367664, -1.315636113682101982 ) ) ;
#34254=CARTESIAN_POINT ( 'NONE',  ( 0.2867679344610365999, 0.2867679344610365999, -0.5374015748031496509 ) ) ;
#34262=CARTESIAN_POINT ( 'NONE',  ( -0.3021538998208400661, -0.2502216998138593884, -1.929133858267717549 ) ) ;
#34264=CARTESIAN_POINT ( 'NONE',  ( 0.1049643490035304938, -0.3917322834645669549, -1.967191601049868899 ) ) ;
#34266=CARTESIAN_POINT ( 'NONE',  ( 0.3460692066303959202, 0.1998031496062993295, -0.4461942257217847430 ) ) ;
#34273=CARTESIAN_POINT ( 'NONE',  ( -0.1049643490035302024, -0.3917322834645671215, -1.416666666666666519 ) ) ;
#34275=CARTESIAN_POINT ( 'NONE',  ( -0.3972027188793493813, -0.005815251566504483528, -1.929133858265299262 ) ) ;
#34282=CARTESIAN_POINT ( 'NONE',  ( -9.787531504996566615E-17, 0.3996062992125985480, -2.124015748031496287 ) ) ;
#34287=ORIENTED_EDGE ( 'NONE', *, *, #39222, .T. ) ;
#34294=CARTESIAN_POINT ( 'NONE',  ( 0.3392501089628018329, 0.1958661417322835052, -1.313628978181415441 ) ) ;
#34297=CARTESIAN_POINT ( 'NONE',  ( 0.3917322834645669549, 0.1049643490035304660, -1.154199475065616820 ) ) ;
#34303=CARTESIAN_POINT ( 'NONE',  ( 4.797336870675656522E-17, -0.3917322834645670659, 0.08200168159348891761 ) ) ;
#34306=CARTESIAN_POINT ( 'NONE',  ( 0.2362204724409449064, 0.4091458600556404646, -1.638451443569553634 ) ) ;
#34316=DIRECTION ( 'NONE',  ( 0.000000000000000000, 0.000000000000000000, 1.000000000000000000 ) ) ;
#34322=CARTESIAN_POINT ( 'NONE',  ( -0.1070741851644056997, 0.3996062992125984925, -2.760498687664041384 ) ) ;
#34327=CARTESIAN_POINT ( 'NONE',  ( -0.3996062992125984925, -0.1070741851644056858, -1.697506561679790194 ) ) ;
#34332=CARTESIAN_POINT ( 'NONE',  ( -0.3460692066303960313, 0.1998031496062989965, -1.047900262467191590 ) ) ;
#34334=CARTESIAN_POINT ( 'NONE',  ( -0.3460692066303960868, 0.1998031496062990242, -1.286089238845144367 ) ) ;
#34335=CARTESIAN_POINT ( 'NONE',  ( 0.2891555358219910499, 0.2891555358219910499, -0.7677165354330709457 ) ) ;
#34336=CARTESIAN_POINT ( 'NONE',  ( -0.3392501089628017219, -0.1958661417322836718, -0.2020997375328083545 ) ) ;
#34340=CARTESIAN_POINT ( 'NONE',  ( -0.3949938075777409963, -7.255918531996591613E-17, -1.848425196850393970 ) ) ;
#34344=CARTESIAN_POINT ( 'NONE',  ( -0.2362204724409447953, -0.4091458600556404646, -1.955380577427821454 ) ) ;
#34345=CARTESIAN_POINT ( 'NONE',  ( 0.3486222174624411529, -0.1789624963018366099, -2.755905511811023612 ) ) ;
#34352=CARTESIAN_POINT ( 'NONE',  ( 0.2867679344610365999, 0.2867679344610365999, -2.580033177656481325 ) ) ;
#34359=CARTESIAN_POINT ( 'NONE',  ( -0.2867679344610364334, -0.2867679344610368219, -2.658773335136795701 ) ) ;
#34361=CARTESIAN_POINT ( 'NONE',  ( 0.3917322834645669549, 0.1049643490035304660, -1.849081364829396223 ) ) ;
#34363=VERTEX_POINT ( 'NONE', #15260 ) ;
#34364=CARTESIAN_POINT ( 'NONE',  ( -0.3949938075777409408, -0.1058382717557502933, -2.408136482939633449 ) ) ;
#34370=CARTESIAN_POINT ( 'NONE',  ( 0.1998031496062994405, -0.3460692066303958092, -0.4068241469816273326 ) ) ;
#34375=CARTESIAN_POINT ( 'NONE',  ( -0.1958661417322834220, -0.3392501089628018884, 0.007217847769028785422 ) ) ;
#34386=CARTESIAN_POINT ( 'NONE',  ( -1.157146581871515012E-16, 0.4724409448818898682, -1.259842519685039353 ) ) ;
#34388=CARTESIAN_POINT ( 'NONE',  ( -0.2867679344610364334, -0.2867679344610367109, -0.6811023622047243098 ) ) ;
#34389=CARTESIAN_POINT ( 'NONE',  ( 0.1958661417322834775, 0.3392501089628018884, -2.276246719160105236 ) ) ;
#34392=CARTESIAN_POINT ( 'NONE',  ( -0.1998031496062994405, 0.3460692066303957537, 0.06758530183727032292 ) ) ;
#34397=CARTESIAN_POINT ( 'NONE',  ( -0.3917322834645669549, -7.196005306013483243E-17, 0.1955573735246212974 ) ) ;
#34399=CARTESIAN_POINT ( 'NONE',  ( -0.09156050430092219083, -0.3808816823641230087, -1.492482962822815952E-17 ) ) ;
#34404=CARTESIAN_POINT ( 'NONE',  ( -0.1958661417322834220, -0.3392501089628018884, -1.947506561679789971 ) ) ;
#34408=CARTESIAN_POINT ( 'NONE',  ( 5.785732909357575061E-17, -0.4724409448818898682, -0.4704724409448819422 ) ) ;
#34423=CARTESIAN_POINT ( 'NONE',  ( 0.1070741851644053388, 0.3996062992125986035, -1.645013123359579943 ) ) ;
#34424=( BOUNDED_CURVE ( )  B_SPLINE_CURVE ( 2, ( #29521, #34188, #21972, #2204, #28281, #48875, #53532, #53943, #66185, #16087, #47216, #41732, #9760 ),
 .UNSPECIFIED., .F., .F. ) 
 B_SPLINE_CURVE_WITH_KNOTS ( ( 3, 2, 2, 2, 2, 2, 3 ),
 ( 0.1125000000000000028, 0.1166666666666666685, 0.1208333333333333343, 0.1250000000000000000, 0.1291666666666666796, 0.1333333333333333315, 0.1375000000000000111 ),
 .UNSPECIFIED. ) 
 CURVE ( )  GEOMETRIC_REPRESENTATION_ITEM ( )  RATIONAL_B_SPLINE_CURVE ( ( 1.000000000000000000, 0.9659258262890683122, 1.000000000000000000, 0.9659258262890683122, 1.000000000000000000, 0.9659258262890683122, 1.000000000000000000, 0.9659258262890683122, 1.000000000000000000, 0.9659258262890683122, 1.000000000000000000, 0.9659258262890683122, 1.000000000000000000 ) ) 
 REPRESENTATION_ITEM ( '' )  );
#34434=CARTESIAN_POINT ( 'NONE',  ( -0.1998031496062991907, -0.3460692066303959757, -0.06561679790026248016 ) ) ;
#34435=CARTESIAN_POINT ( 'NONE',  ( 0.1958661417322836718, -0.3392501089628017219, -2.450806717356642128 ) ) ;
#34440=CARTESIAN_POINT ( 'NONE',  ( -0.1958661417322834220, -0.3392501089628018884, -2.354986876640420057 ) ) ;
#34445=CARTESIAN_POINT ( 'NONE',  ( -0.3460692066303958092, -0.1998031496062994683, -1.942257217847769057 ) ) ;
#34448=CARTESIAN_POINT ( 'NONE',  ( 4.797336870675656522E-17, -0.3917322834645670659, -0.5479195782490308142 ) ) ;
#34461=CARTESIAN_POINT ( 'NONE',  ( 0.3917322834645669549, 0.1049643490035304660, -0.5892388451443569819 ) ) ;
#34464=CARTESIAN_POINT ( 'NONE',  ( -0.1974969037888703871, -0.3420746716998661063, -1.010498687664042050 ) ) ;
#34468=AXIS2_PLACEMENT_3D ( 'NONE', #27261, #78635, #20959 ) ;
#34483=CARTESIAN_POINT ( 'NONE',  ( -0.1998031496062994683, 0.3460692066303958092, -1.587926509186351698 ) ) ;
#34485=CARTESIAN_POINT ( 'NONE',  ( 0.1070741851644054776, -0.3996062992125984925, -1.264435695538057569 ) ) ;
#34486=CARTESIAN_POINT ( 'NONE',  ( -0.3996062992125985480, -7.340648628747423112E-17, -0.4311023622047244208 ) ) ;
#34488=CARTESIAN_POINT ( 'NONE',  ( 0.1998031496062994405, -0.3460692066303958092, -2.926509186351706315 ) ) ;
#34489=CARTESIAN_POINT ( 'NONE',  ( 0.3917322834645670104, 2.398668435337828261E-17, -2.564960629921259727 ) ) ;
#34496=CARTESIAN_POINT ( 'NONE',  ( 5.785732909357575061E-17, -0.4724409448818898682, -2.045275590551181022 ) ) ;
#34499=CARTESIAN_POINT ( 'NONE',  ( -0.3420746716998660508, -0.1974969037888706924, -2.019028871391076230 ) ) ;
#34502=CARTESIAN_POINT ( 'NONE',  ( 0.000000000000000000, 0.000000000000000000, -1.929133858267716661 ) ) ;
#34505=CARTESIAN_POINT ( 'NONE',  ( 0.4724409448818880919, 0.1265901696525020825, -2.248687664041995049 ) ) ;
#34509=CARTESIAN_POINT ( 'NONE',  ( 0.3460692066303959202, -0.1998031496062991630, -2.386482939632545985 ) ) ;
#34510=CARTESIAN_POINT ( 'NONE',  ( 0.3392501089628018329, -0.1958661417322834497, -2.232264148785090274 ) ) ;
#34522=CARTESIAN_POINT ( 'NONE',  ( -0.3460692066303960313, 0.1998031496062989965, -0.2604986876640419946 ) ) ;
#34526=CARTESIAN_POINT ( 'NONE',  ( -0.1958661417322834220, -0.3392501089628018884, -2.040026246719160330 ) ) ;
#34535=CARTESIAN_POINT ( 'NONE',  ( 0.3996062992125985480, 2.446882876249141654E-17, -0.8248031496062991907 ) ) ;
#34537=CARTESIAN_POINT ( 'NONE',  ( 0.4724409448818898682, 2.892866454678787531E-17, -2.637795275590551380 ) ) ;
#34538=ORIENTED_EDGE ( 'NONE', *, *, #68721, .T. ) ;
#34550=CARTESIAN_POINT ( 'NONE',  ( -0.1998031496062994683, 0.3460692066303958092, -0.3280839895013123453 ) ) ;
#34553=CARTESIAN_POINT ( 'NONE',  ( -0.3917322834645670104, -7.196005306013484475E-17, -2.078740157480314821 ) ) ;
#34565=CARTESIAN_POINT ( 'NONE',  ( 0.1958661417322836162, -0.3392501089628018329, -1.431739214401887894 ) ) ;
#34571=CARTESIAN_POINT ( 'NONE',  ( 0.1049643490035304799, -0.3917322834645670104, -2.916685982448506298 ) ) ;
#34580=CARTESIAN_POINT ( 'NONE',  ( -0.3917322834645670104, -7.196005306013484475E-17, -2.328740157480315265 ) ) ;
#34587=CARTESIAN_POINT ( 'NONE',  ( 0.1998031496062994128, -0.3460692066303957537, -0.01115485564304462100 ) ) ;
#34590=CARTESIAN_POINT ( 'NONE',  ( 0.1070741851644053527, 0.3996062992125986590, -1.883202099737532276 ) ) ;
#34598=CARTESIAN_POINT ( 'NONE',  ( 0.2362204724409451007, -0.4091458600556402980, -0.4835958005249343938 ) ) ;
#34601=CARTESIAN_POINT ( 'NONE',  ( -0.1058382717557497660, -0.3949938075777411073, -0.3064304461942257696 ) ) ;
#34606=CARTESIAN_POINT ( 'NONE',  ( -0.3420746716998660508, -0.1974969037888706924, -0.2867454068241469534 ) ) ;
#34613=CARTESIAN_POINT ( 'NONE',  ( 0.3996062992125986035, -0.1070741851644052972, -1.133202099737532720 ) ) ;
#34615=CARTESIAN_POINT ( 'NONE',  ( -0.3392501089628019995, 0.1958661417322832277, -0.9632545931758529356 ) ) ;
#34628=CARTESIAN_POINT ( 'NONE',  ( -0.3460692066303957537, -0.1998031496062994405, 0.1856955380577427484 ) ) ;
#34645=CARTESIAN_POINT ( 'NONE',  ( 4.893765752498283924E-17, -0.3996062992125986035, -0.8661417322834645827 ) ) ;
#34650=CARTESIAN_POINT ( 'NONE',  ( 0.3996062992125986590, -0.1070741851644053111, -2.946194225721785465 ) ) ;
#34651=CARTESIAN_POINT ( 'NONE',  ( 0.3949938075777409963, 2.418639510665530435E-17, -2.165354330708661124 ) ) ;
#34652=ORIENTED_EDGE ( 'NONE', *, *, #74631, .F. ) ;
#34654=CARTESIAN_POINT ( 'NONE',  ( 0.3917322834645670104, 2.398668435337828261E-17, -1.055118110236220375 ) ) ;
#34658=CARTESIAN_POINT ( 'NONE',  ( -0.2017716535433071445, 0.2017716535433070613, 0.000000000000000000 ) ) ;
#34661=CARTESIAN_POINT ( 'NONE',  ( -0.3917322834645668994, -0.1049643490035306742, -0.1259649361866648498 ) ) ;
#34669=CARTESIAN_POINT ( 'NONE',  ( -0.2867679344610367109, 0.2867679344610365444, -1.433746349902574213 ) ) ;
#34675=CARTESIAN_POINT ( 'NONE',  ( 0.3917322834645669549, 0.1049643490035304660, -0.3667979002624672802 ) ) ;
#34684=CARTESIAN_POINT ( 'NONE',  ( -0.2867679344610364334, -0.2867679344610367109, -2.413385826771653253 ) ) ;
#34687=EDGE_LOOP ( 'NONE', ( #42336, #29382, #18610, #30385 ) ) ;
#34693=CARTESIAN_POINT ( 'NONE',  ( 0.3917322834645669549, 0.1049643490035304660, -1.154199475065616820 ) ) ;
#34694=CARTESIAN_POINT ( 'NONE',  ( -0.3996062992125984925, -0.1070741851644056858, -2.169947506561679340 ) ) ;
#34703=CARTESIAN_POINT ( 'NONE',  ( -0.3460692066303960313, 0.1998031496062989965, -1.992782152230971437 ) ) ;
#34705=CARTESIAN_POINT ( 'NONE',  ( -0.3917322834645670104, -7.196005306013484475E-17, 0.1259842519685039908 ) ) ;
#34713=CARTESIAN_POINT ( 'NONE',  ( 0.1958661417322834497, 0.3392501089628018329, -1.169272022800837973 ) ) ;
#34723=CARTESIAN_POINT ( 'NONE',  ( 0.3392501089628018884, -0.1958661417322833942, 0.05575496243338393110 ) ) ;
#34727=CARTESIAN_POINT ( 'NONE',  ( 5.785732909357575061E-17, -0.4724409448818898682, -1.572834645669291431 ) ) ;
#34743=CARTESIAN_POINT ( 'NONE',  ( 4.837279021331061486E-17, -0.3949938075777409963, 0.1594488188976377896 ) ) ;
#34748=CARTESIAN_POINT ( 'NONE',  ( 0.1998031496062992463, 0.3460692066303959202, -2.268372703412073754 ) ) ;
#34754=CARTESIAN_POINT ( 'NONE',  ( -0.3460692066303958092, -0.1998031496062994683, -1.312335958005249381 ) ) ;
#34755=CARTESIAN_POINT ( 'NONE',  ( -9.674558042662121740E-17, 0.3949938075777409963, -0.9448818897637795144 ) ) ;
#34756=CARTESIAN_POINT ( 'NONE',  ( -0.2925321140481932924, 0.2925321140481931814, -2.381889763779527325 ) ) ;
#34758=CARTESIAN_POINT ( 'NONE',  ( -0.3917322834645671215, 0.1049643490035301469, -0.3398950131233596239 ) ) ;
#34762=CARTESIAN_POINT ( 'NONE',  ( 0.3420746716998660508, 0.1974969037888705814, -2.097769028871391495 ) ) ;
#34764=EDGE_CURVE ( 'NONE', #25718, #23063, #10998, .T. ) ;
#34767=CARTESIAN_POINT ( 'NONE',  ( 0.4091458600556403535, 0.2362204724409449896, -2.020997375328084100 ) ) ;
#34768=CARTESIAN_POINT ( 'NONE',  ( 0.1906283239483269054, 0.3428707098288080735, -2.755905511811022279 ) ) ;
#34775=CARTESIAN_POINT ( 'NONE',  ( -0.3917322834645668994, -0.1049643490035306742, -2.488169660596113886 ) ) ;
#34782=CARTESIAN_POINT ( 'NONE',  ( 0.1049643490035303689, 0.3917322834645670104, 0.07939632545931750440 ) ) ;
#34784=CARTESIAN_POINT ( 'NONE',  ( 0.3917322834645670104, 2.398668435337828261E-17, -1.685039370078740051 ) ) ;
#34787=CARTESIAN_POINT ( 'NONE',  ( 0.3420746716998660508, -0.1974969037888703871, -2.467191601049868677 ) ) ;
#34791=CARTESIAN_POINT ( 'NONE',  ( -0.1998031496062991907, -0.3460692066303959757, -0.5380577427821522374 ) ) ;
#34794=CARTESIAN_POINT ( 'NONE',  ( 0.2017716535433070613, 0.2017716535433070613, -0.3937007874015748254 ) ) ;
#34796=CARTESIAN_POINT ( 'NONE',  ( -0.3392501089628017219, -0.1958661417322836718, -0.1371391076115486551 ) ) ;
#34803=CARTESIAN_POINT ( 'NONE',  ( -0.1958661417322834220, -0.3392501089628018884, -0.05774278215223092176 ) ) ;
#34804=ORIENTED_EDGE ( 'NONE', *, *, #75114, .F. ) ;
#34808=CARTESIAN_POINT ( 'NONE',  ( -0.4724409448818895907, -0.1265901696524993070, -1.463254593175853158 ) ) ;
#34810=CARTESIAN_POINT ( 'NONE',  ( -0.1049643490035302024, -0.3917322834645671215, -0.5367454068241469534 ) ) ;
#34811=CARTESIAN_POINT ( 'NONE',  ( -0.1958661417322834220, -0.3392501089628018884, -2.354986876640420057 ) ) ;
#34814=CARTESIAN_POINT ( 'NONE',  ( 0.1070741851644053388, 0.3996062992125986035, -0.07020997375328086321 ) ) ;
#34820=CARTESIAN_POINT ( 'NONE',  ( 0.3392501089628018329, -0.1958661417322834497, 0.1299405756243587895 ) ) ;
#34822=CARTESIAN_POINT ( 'NONE',  ( 0.1049643490035304799, -0.3917322834645669549, -0.3274278215223098143 ) ) ;
#34828=CARTESIAN_POINT ( 'NONE',  ( 0.1049643490035303689, 0.3917322834645670104, -2.032808398950130879 ) ) ;
#34831=CARTESIAN_POINT ( 'NONE',  ( 0.2362204724409449064, 0.4091458600556404646, -0.5360892388451443669 ) ) ;
#34841=CARTESIAN_POINT ( 'NONE',  ( -0.1070741851644051862, -0.3996062992125986590, -1.566272965879265344 ) ) ;
#34850=CARTESIAN_POINT ( 'NONE',  ( 0.1998031496062994405, -0.3460692066303958092, -0.09186351706036746667 ) ) ;
#34852=CARTESIAN_POINT ( 'NONE',  ( 0.2891555358219910499, 0.2891555358219910499, 0.01968503937007868437 ) ) ;
#34853=CARTESIAN_POINT ( 'NONE',  ( -0.07128922432405460086, -0.3857547143408426860, -1.492482962822815952E-17 ) ) ;
#34857=CARTESIAN_POINT ( 'NONE',  ( -0.2867679344610365999, 0.2867679344610364889, -2.309055118110235671 ) ) ;
#34862=CARTESIAN_POINT ( 'NONE',  ( -0.1265901696524993347, 0.4724409448818895907, -0.7939632545931758489 ) ) ;
#34867=CARTESIAN_POINT ( 'NONE',  ( -0.3917322834645670104, -0.1049643490035307020, -0.2001505493776396805 ) ) ;
#34880=CARTESIAN_POINT ( 'NONE',  ( -0.3917322834645669549, -0.1049643490035306603, -0.6679790026246719137 ) ) ;
#34883=CARTESIAN_POINT ( 'NONE',  ( 0.2891555358219910499, -0.2891555358219909944, -0.8858267716535433989 ) ) ;
#34893=CARTESIAN_POINT ( 'NONE',  ( -0.2362204724409451284, 0.4091458600556402425, -0.4048556430446194621 ) ) ;
#34899=CARTESIAN_POINT ( 'NONE',  ( -0.1070741851644056997, 0.3996062992125986035, -1.738845144356955696 ) ) ;
#34902=CARTESIAN_POINT ( 'NONE',  ( 4.893765752498283308E-17, -0.3996062992125985480, -1.100393700787401619 ) ) ;
#34903=CARTESIAN_POINT ( 'NONE',  ( 0.1998031496062992463, 0.3460692066303959202, -0.3786089238845143923 ) ) ;
#34905=CARTESIAN_POINT ( 'NONE',  ( 0.3458507752293908943, 0.3458507752293908943, -0.1377952755905511861 ) ) ;
#34906=CARTESIAN_POINT ( 'NONE',  ( 0.1958661417322836440, -0.3392501089628017219, -2.381233595800524849 ) ) ;
#34912=CARTESIAN_POINT ( 'NONE',  ( 0.2362204724409449064, 0.4091458600556404646, -1.795931758530183719 ) ) ;
#34916=CARTESIAN_POINT ( 'NONE',  ( -9.674558042662122972E-17, 0.3949938075777409963, -1.809055118110236560 ) ) ;
#34925=CARTESIAN_POINT ( 'NONE',  ( 0.1070741851644053388, 0.3996062992125986035, -2.589895013123359568 ) ) ;
#34927=CARTESIAN_POINT ( 'NONE',  ( 0.3392501089628018329, -0.1958661417322834497, -2.547224778706350445 ) ) ;
#34939=CARTESIAN_POINT ( 'NONE',  ( 0.3460692066303959202, -0.1998031496062991630, -0.4967191601049869010 ) ) ;
#34941=CARTESIAN_POINT ( 'NONE',  ( 0.1958661417322836440, -0.3392501089628017219, -1.751312335958005395 ) ) ;
#34950=CARTESIAN_POINT ( 'NONE',  ( -0.2925321140481930149, -0.2925321140481933480, -0.7657480314960628531 ) ) ;
#34956=CARTESIAN_POINT ( 'NONE',  ( 0.3917864676224471765, 0.04037479286078551194, -1.220472440943932702 ) ) ;
#34964=CARTESIAN_POINT ( 'NONE',  ( -9.787531504996567848E-17, 0.3996062992125986035, -0.6299212598425196763 ) ) ;
#34967=CARTESIAN_POINT ( 'NONE',  ( 0.1049643490035303689, 0.3917322834645670104, -2.032808398950130879 ) ) ;
#34977=CARTESIAN_POINT ( 'NONE',  ( -0.2867679344610366554, 0.2867679344610365444, -1.359560736711598938 ) ) ;
#34983=CARTESIAN_POINT ( 'NONE',  ( 0.3949938075777409408, 0.1058382717557500574, 0.03280839895013118457 ) ) ;
#34992=CARTESIAN_POINT ( 'NONE',  ( 0.3392501089628018329, 0.1958661417322835607, -2.105643044619422533 ) ) ;
#34999=CARTESIAN_POINT ( 'NONE',  ( 0.3996062992125986035, -0.1070741851644052972, -0.03083989501312336262 ) ) ;
#35001=CARTESIAN_POINT ( 'NONE',  ( 0.3460692066303959757, -0.1998031496062991907, -1.679790026246719137 ) ) ;
#35003=ADVANCED_FACE ( 'NONE', ( #33567 ), #7483, .T. ) ;
#35007=CARTESIAN_POINT ( 'NONE',  ( -0.4091458600556402980, -0.2362204724409451284, -0.6017060367454067915 ) ) ;
#35011=CARTESIAN_POINT ( 'NONE',  ( 0.3949938075777409963, 2.418639510665530743E-17, -0.5098425196850394636 ) ) ;
#35016=CARTESIAN_POINT ( 'NONE',  ( -0.1058382717557503072, 0.3949938075777408852, -0.3982939632545932640 ) ) ;
#35023=CARTESIAN_POINT ( 'NONE',  ( 0.2925321140481932369, -0.2925321140481931814, -1.277559055118110187 ) ) ;
#35025=CARTESIAN_POINT ( 'NONE',  ( -0.3917322834645671215, 0.1049643490035301469, -0.9698162729658791337 ) ) ;
#35039=CARTESIAN_POINT ( 'NONE',  ( -0.1265901696524986964, -0.4724409448818899238, -0.3064304461942256586 ) ) ;
#35052=CARTESIAN_POINT ( 'NONE',  ( -0.1070741851644057135, 0.3996062992125985480, -0.7939632545931758489 ) ) ;
#35053=FACE_BOUND ( 'NONE', #38185, .T. ) ;
#35056=CARTESIAN_POINT ( 'NONE',  ( -9.787531504996567848E-17, 0.3996062992125986035, -2.834645669291338432 ) ) ;
#35057=CARTESIAN_POINT ( 'NONE',  ( 0.3949938075777409408, 0.1058382717557500574, -2.486876640419947382 ) ) ;
#35060=CARTESIAN_POINT ( 'NONE',  ( -0.3917322834645669549, -0.1049643490035306603, -1.140419947506561282 ) ) ;
#35067=CARTESIAN_POINT ( 'NONE',  ( -0.3392501089628018329, -0.1958661417322836440, -0.4474872458979509138 ) ) ;
#35072=CARTESIAN_POINT ( 'NONE',  ( -0.4724409448818898682, -8.678599364036362592E-17, -0.03937007874015747977 ) ) ;
#35073=CARTESIAN_POINT ( 'NONE',  ( -0.3458507752293909498, 0.3458507752293908388, -1.122047244094488194 ) ) ;
#35074=CARTESIAN_POINT ( 'NONE',  ( 0.3917322834645670659, -0.1049643490035303273, -1.525609866962941430 ) ) ;
#35080=CARTESIAN_POINT ( 'NONE',  ( 0.1958661417322836440, -0.3392501089628017219, -1.121391076115485719 ) ) ;
#35089=CARTESIAN_POINT ( 'NONE',  ( 0.3392501089628018329, 0.1958661417322835607, -2.328083989501312345 ) ) ;
#35098=CARTESIAN_POINT ( 'NONE',  ( -0.3392501089628017219, -0.1958661417322836718, -1.396981627296587813 ) ) ;
#35099=CARTESIAN_POINT ( 'NONE',  ( 0.1998031496062992463, 0.3460692066303959202, -2.425853018372703396 ) ) ;
#35109=CARTESIAN_POINT ( 'NONE',  ( -0.3996062992125986035, 0.1070741851644051584, -2.156824146981627166 ) ) ;
#35118=CARTESIAN_POINT ( 'NONE',  ( -0.3917322834645668994, -0.1049643490035306742, -1.228327140911074089 ) ) ;
#35129=CARTESIAN_POINT ( 'NONE',  ( -0.1049643490035307158, 0.3917322834645670104, -0.3182607855981121059 ) ) ;
#35133=CARTESIAN_POINT ( 'NONE',  ( 0.4724409448818896462, 0.1265901696524990294, -1.776246719160104570 ) ) ;
#35151=CARTESIAN_POINT ( 'NONE',  ( -0.1070741851644051862, -0.3996062992125986590, -2.668635170603674833 ) ) ;
#35152=EDGE_CURVE ( 'NONE', #49144, #79206, #76447, .T. ) ;
#35157=CARTESIAN_POINT ( 'NONE',  ( -0.2925321140481930149, -0.2925321140481933480, -2.340551181102362488 ) ) ;
#35162=CARTESIAN_POINT ( 'NONE',  ( -0.2925321140481932924, 0.2925321140481931814, -1.909448818897637512 ) ) ;
#35163=CARTESIAN_POINT ( 'NONE',  ( -0.1058382717557503211, 0.3949938075777409408, -0.9514435695538059345 ) ) ;
#35164=CARTESIAN_POINT ( 'NONE',  ( 0.3460692066303959202, 0.1998031496062993295, -2.493438320209973469 ) ) ;
#35166=CARTESIAN_POINT ( 'NONE',  ( 0.1958661417322836440, -0.3392501089628017219, -0.08398950131233590133 ) ) ;
#35170=CARTESIAN_POINT ( 'NONE',  ( 0.1974969037888704704, 0.3420746716998660508, -1.953412073490814027 ) ) ;
#35174=CARTESIAN_POINT ( 'NONE',  ( 0.4724409448818897572, -0.1265901696524988906, -2.316272965879265122 ) ) ;
#35175=CARTESIAN_POINT ( 'NONE',  ( -0.1070741851644051862, -0.3996062992125987146, -1.804461942257217677 ) ) ;
#35176=CARTESIAN_POINT ( 'NONE',  ( -0.2017716535433071445, -0.2017716535433071445, 0.000000000000000000 ) ) ;
#35183=CARTESIAN_POINT ( 'NONE',  ( 4.797336870675655290E-17, -0.3917322834645669549, -2.835938689467505380 ) ) ;
#35190=CARTESIAN_POINT ( 'NONE',  ( 0.3392501089628018884, -0.1958661417322834220, -0.1896325459317586282 ) ) ;
#35192=CARTESIAN_POINT ( 'NONE',  ( 0.3392501089628018884, -0.1958661417322834220, -2.144356955380577467 ) ) ;
#35195=CARTESIAN_POINT ( 'NONE',  ( 0.2891555358219910499, -0.2891555358219909944, -2.303149606299212504 ) ) ;
#35199=CARTESIAN_POINT ( 'NONE',  ( 0.1998031496062994405, -0.3460692066303958092, -1.036745406824147064 ) ) ;
#35203=LINE ( 'NONE', #48235, #32384 ) ;
#35204=CARTESIAN_POINT ( 'NONE',  ( -0.1049643490035307020, 0.3917322834645669549, -0.09120734908136493568 ) ) ;
#35214=CARTESIAN_POINT ( 'NONE',  ( 0.4091458600556403535, 0.2362204724409449896, -1.863517060367454015 ) ) ;
#35217=CARTESIAN_POINT ( 'NONE',  ( -0.2867679344610365999, 0.2867679344610364889, -0.6417322834645668994 ) ) ;
#35218=CARTESIAN_POINT ( 'NONE',  ( -9.594673741351313045E-17, 0.3917322834645670104, -2.604330708661416693 ) ) ;
#35221=CARTESIAN_POINT ( 'NONE',  ( -0.3996062992125985480, -7.340648628747423112E-17, -0.5885826771653542844 ) ) ;
#35226=CARTESIAN_POINT ( 'NONE',  ( -0.2867679344610364334, -0.2867679344610368219, -0.1390882957667173292 ) ) ;
#35228=CARTESIAN_POINT ( 'NONE',  ( -0.1049643490035301885, -0.3917322834645671215, -0.3143044619422573072 ) ) ;
#35234=CARTESIAN_POINT ( 'NONE',  ( 0.2867679344610365999, 0.2867679344610365999, -2.177165354330708347 ) ) ;
#35237=CARTESIAN_POINT ( 'NONE',  ( 0.1265901696524989462, 0.4724409448818897572, -0.2276902887139107545 ) ) ;
#35247=ORIENTED_EDGE ( 'NONE', *, *, #20205, .F. ) ;
#35248=CARTESIAN_POINT ( 'NONE',  ( 0.2925321140481932369, -0.2925321140481931814, -1.750000000000000222 ) ) ;
#35257=CARTESIAN_POINT ( 'NONE',  ( 0.3996062992125985480, 2.446882876249141654E-17, -0.1948818897637795700 ) ) ;
#35258=CARTESIAN_POINT ( 'NONE',  ( 0.1998031496062992740, 0.3460692066303959757, -0.4593175853018372501 ) ) ;
#35259=CARTESIAN_POINT ( 'NONE',  ( -9.594673741351313045E-17, 0.3917322834645670659, -2.831384145178164058 ) ) ;
#35264=CARTESIAN_POINT ( 'NONE',  ( -0.3420746716998660508, -0.1974969037888706924, -0.9166666666666668517 ) ) ;
#35269=CARTESIAN_POINT ( 'NONE',  ( 0.4724409448818896462, 0.1265901696524990294, -0.9120734908136483021 ) ) ;
#35270=CARTESIAN_POINT ( 'NONE',  ( 0.3996062992125985480, 0.1070741851644054637, -2.329396325459317296 ) ) ;
#35272=EDGE_CURVE ( 'NONE', #21828, #42415, #13029, .T. ) ;
#35273=ORIENTED_EDGE ( 'NONE', *, *, #76425, .T. ) ;
#35274=CARTESIAN_POINT ( 'NONE',  ( 0.1958661417322836718, -0.3392501089628017219, -0.2460823079078234277 ) ) ;
#35288=CARTESIAN_POINT ( 'NONE',  ( -0.3392501089628017219, -0.1958661417322836718, -0.5170603674540682482 ) ) ;
#35291=CARTESIAN_POINT ( 'NONE',  ( -0.1974969037888703871, -0.3420746716998661063, -0.8530183727034120755 ) ) ;
#35307=CARTESIAN_POINT ( 'NONE',  ( -9.787531504996567848E-17, 0.3996062992125986035, -1.889763779527559251 ) ) ;
#35310=CARTESIAN_POINT ( 'NONE',  ( 0.1998031496062992463, 0.3460692066303959202, -1.008530183727034180 ) ) ;
#35311=CARTESIAN_POINT ( 'NONE',  ( -0.2925321140481932369, 0.2925321140481931259, -0.7263779527559056648 ) ) ;
#35314=CARTESIAN_POINT ( 'NONE',  ( 0.3996062992125986590, -0.1070741851644053111, -2.946194225721785465 ) ) ;
#35315=CARTESIAN_POINT ( 'NONE',  ( -0.3917322834645669549, -0.1049643490035306603, -2.650262467191601079 ) ) ;
#35321=CARTESIAN_POINT ( 'NONE',  ( -0.1265901696524986964, -0.4724409448818899238, -1.881233595800524849 ) ) ;
#35325=CARTESIAN_POINT ( 'NONE',  ( -0.2891555358219911054, 0.2891555358219909388, -1.828740157480315487 ) ) ;
#35335=CARTESIAN_POINT ( 'NONE',  ( -0.3392501089628019439, 0.1958661417322832554, -2.625964936186665266 ) ) ;
#35349=CARTESIAN_POINT ( 'NONE',  ( 0.3996062992125984925, 0.1070741851644054637, -0.3589238845144357426 ) ) ;
#35351=CARTESIAN_POINT ( 'NONE',  ( 0.3917322834645670104, -0.1049643490035303411, -1.770997375328083656 ) ) ;
#35356=LINE ( 'NONE', #42477, #65598 ) ;
#35360=CARTESIAN_POINT ( 'NONE',  ( 4.893765752498283308E-17, -0.3996062992125985480, -0.7854330708661416693 ) ) ;
#35368=CARTESIAN_POINT ( 'NONE',  ( 0.3917322834645670104, 2.398668435337828261E-17, -1.620078740157480324 ) ) ;
#35372=CARTESIAN_POINT ( 'NONE',  ( -0.1049643490035301885, -0.3917322834645671215, -2.741469816272965154 ) ) ;
#35376=CARTESIAN_POINT ( 'NONE',  ( -0.1070741851644051862, -0.3996062992125987146, -0.5446194225721783244 ) ) ;
#35379=CARTESIAN_POINT ( 'NONE',  ( 0.1049643490035303689, 0.3917322834645670104, -2.190288713910760521 ) ) ;
#35389=CARTESIAN_POINT ( 'NONE',  ( -0.3917322834645670659, 0.1049643490035301607, -1.530164411252281420 ) ) ;
#35395=CARTESIAN_POINT ( 'NONE',  ( -0.2891555358219911054, 0.2891555358219909388, 0.1377952755905511306 ) ) ;
#35404=CARTESIAN_POINT ( 'NONE',  ( 0.1958661417322834775, 0.3392501089628018884, -1.400937950952442668 ) ) ;
#35406=CARTESIAN_POINT ( 'NONE',  ( 0.1049643490035303689, 0.3917322834645670104, -2.282808398950130879 ) ) ;
#35412=CARTESIAN_POINT ( 'NONE',  ( 0.3460692066303959202, -0.1998031496062991630, -0.02427821522309711946 ) ) ;
#35414=CARTESIAN_POINT ( 'NONE',  ( 0.3996062992125986035, 2.446882876249141962E-17, -1.850393700787401619 ) ) ;
#35419=CARTESIAN_POINT ( 'NONE',  ( -0.1265901696524993347, 0.4724409448818895907, -0.7132545931758530466 ) ) ;
#35422=CARTESIAN_POINT ( 'NONE',  ( -0.1974969037888706924, 0.3420746716998658843, -0.4048556430446195176 ) ) ;
#35427=CARTESIAN_POINT ( 'NONE',  ( -0.3420746716998660508, -0.1974969037888706924, -0.6017060367454067915 ) ) ;
#35434=CARTESIAN_POINT ( 'NONE',  ( -0.3996062992125986590, 0.1070741851644051723, -1.369422572178477404 ) ) ;
#35436=CARTESIAN_POINT ( 'NONE',  ( -0.3917322834645671215, 0.1049643490035301469, -1.127296587926509108 ) ) ;
#35465=CARTESIAN_POINT ( 'NONE',  ( -0.3996062992125985480, -0.1070741851644057135, -1.148293963254592986 ) ) ;
#35469=CARTESIAN_POINT ( 'NONE',  ( -0.4091458600556402980, -0.2362204724409451284, 0.1049868766404199460 ) ) ;
#35470=CARTESIAN_POINT ( 'NONE',  ( 0.1974969037888704704, 0.3420746716998660508, -2.191601049868766360 ) ) ;
#35473=CARTESIAN_POINT ( 'NONE',  ( -0.1049643490035307020, 0.3917322834645669549, -0.9435695538057740084 ) ) ;
#35475=CARTESIAN_POINT ( 'NONE',  ( 0.4724409448818898682, 2.892866454678787531E-17, -2.480314960629921295 ) ) ;
#35481=CARTESIAN_POINT ( 'NONE',  ( -0.1049643490035306742, 0.3917322834645668994, -0.4015554873677671943 ) ) ;
#35487=CARTESIAN_POINT ( 'NONE',  ( -0.2362204724409451284, 0.4091458600556402425, -1.115485564304461885 ) ) ;
#35488=CARTESIAN_POINT ( 'NONE',  ( 0.3917322834645670659, 2.398668435337828261E-17, -1.689651861713597603 ) ) ;
#35494=CARTESIAN_POINT ( 'NONE',  ( 0.3917322834645669549, 0.1049643490035304660, -0.9967191601049870675 ) ) ;
#35504=CARTESIAN_POINT ( 'NONE',  ( -0.3917322834645669549, -0.1049643490035306603, -2.400262467191600635 ) ) ;
#35511=CARTESIAN_POINT ( 'NONE',  ( -9.594673741351313045E-17, 0.3917322834645670104, -0.8720472440944883052 ) ) ;
#35513=CARTESIAN_POINT ( 'NONE',  ( 0.3965571307776156740, 0.02707642104391132579, -1.929133858267719104 ) ) ;
#35514=CARTESIAN_POINT ( 'NONE',  ( 0.3917322834645670104, 2.398668435337828261E-17, -1.462598425196850460 ) ) ;
#35516=CARTESIAN_POINT ( 'NONE',  ( 0.3996062992125986035, -0.1070741851644052972, -2.550524934383202158 ) ) ;
#35525=CARTESIAN_POINT ( 'NONE',  ( -0.3996062992125985480, -7.340648628747423112E-17, -2.163385826771653697 ) ) ;
#35527=CARTESIAN_POINT ( 'NONE',  ( -9.594673741351313045E-17, 0.3917322834645670104, 0.007874015748031541057 ) ) ;
#35534=CARTESIAN_POINT ( 'NONE',  ( -9.594673741351310580E-17, 0.3917322834645669549, -1.024915067420260728 ) ) ;
#35543=CARTESIAN_POINT ( 'NONE',  ( -0.3917322834645671770, 0.1049643490035302024, -0.6594681346794770693 ) ) ;
#35546=CARTESIAN_POINT ( 'NONE',  ( 0.4724409448818896462, 0.1265901696524990294, -1.933727034120735100 ) ) ;
#35562=VERTEX_POINT ( 'NONE', #13694 ) ;
#35567=CARTESIAN_POINT ( 'NONE',  ( 0.1070741851644053666, 0.3996062992125986035, -0.1509186351706036655 ) ) ;
#35568=CARTESIAN_POINT ( 'NONE',  ( 0.3996062992125986035, -0.1070741851644052972, -2.235564304461942431 ) ) ;
#35573=CARTESIAN_POINT ( 'NONE',  ( 0.1998031496062994405, -0.3460692066303958092, -1.666666666666666741 ) ) ;
#35575=CARTESIAN_POINT ( 'NONE',  ( -0.3949938075777409963, -7.255918531996591613E-17, -0.9842519685039369248 ) ) ;
#35576=CARTESIAN_POINT ( 'NONE',  ( -0.3996062992125986035, -7.340648628747425578E-17, -2.559055118110236560 ) ) ;
#35578=CARTESIAN_POINT ( 'NONE',  ( -9.594673741351313045E-17, 0.3917322834645670104, -0.3070866141732283006 ) ) ;
#35582=CARTESIAN_POINT ( 'NONE',  ( 0.3949938075777408852, 0.1058382717557500435, -2.091207349081364519 ) ) ;
#35586=CARTESIAN_POINT ( 'NONE',  ( 0.4091458600556403535, 0.2362204724409449896, -2.493438320209973469 ) ) ;
#35587=CARTESIAN_POINT ( 'NONE',  ( -0.3996062992125987146, 0.1070741851644051862, -1.922572178477689908 ) ) ;
#35594=CARTESIAN_POINT ( 'NONE',  ( -0.3917322834645669549, -7.196005306013483243E-17, -2.639088295766717884 ) ) ;
#35602=CARTESIAN_POINT ( 'NONE',  ( -0.2867679344610365999, 0.2867679344610364889, -0.2618110236220473341 ) ) ;
#35604=CARTESIAN_POINT ( 'NONE',  ( -0.1958661417322836718, 0.3392501089628017219, -2.209973753280840114 ) ) ;
#35607=CARTESIAN_POINT ( 'NONE',  ( -0.1058382717557497937, -0.3949938075777411628, -2.276902887139107712 ) ) ;
#35611=CARTESIAN_POINT ( 'NONE',  ( -0.3996062992125986035, -0.1070741851644056997, -0.8333333333333332593 ) ) ;
#35615=CARTESIAN_POINT ( 'NONE',  ( 0.01218835185197312924, -0.3960428127060638404, -2.755905511811024056 ) ) ;
#35616=CARTESIAN_POINT ( 'NONE',  ( 0.3917322834645669549, 0.1049643490035304660, -0.05183727034120744204 ) ) ;
#35623=CARTESIAN_POINT ( 'NONE',  ( -0.3917322834645670104, -7.196005306013484475E-17, 0.1259842519685039908 ) ) ;
#35624=VERTEX_POINT ( 'NONE', #22495 ) ;
#35628=CARTESIAN_POINT ( 'NONE',  ( 0.4724409448818898682, 2.892866454678787531E-17, -1.535433070866141669 ) ) ;
#35631=CARTESIAN_POINT ( 'NONE',  ( -0.3392501089628019995, 0.1958661417322832277, -0.8057742782152230721 ) ) ;
#35632=CARTESIAN_POINT ( 'NONE',  ( 0.2867679344610366554, -0.2867679344610365444, -2.702755905511810663 ) ) ;
#35640=CARTESIAN_POINT ( 'NONE',  ( -0.3917322834645668994, -0.1049643490035306742, 0.03151537877396508314 ) ) ;
#35642=CARTESIAN_POINT ( 'NONE',  ( -0.3917322834645670104, -7.196005306013484475E-17, -0.5964566929133858775 ) ) ;
#35647=CARTESIAN_POINT ( 'NONE',  ( -0.1958661417322836718, 0.3392501089628017219, -2.209973753280840114 ) ) ;
#35650=CARTESIAN_POINT ( 'NONE',  ( 0.1265901696524989462, 0.4724409448818897572, -0.3851706036745406458 ) ) ;
#35660=CARTESIAN_POINT ( 'NONE',  ( 0.1070741851644053388, 0.3996062992125986035, -1.487532808398950301 ) ) ;
#35668=CARTESIAN_POINT ( 'NONE',  ( -0.3996062992125986035, 0.1070741851644051584, -0.2670603674540682482 ) ) ;
#35669=CARTESIAN_POINT ( 'NONE',  ( 0.1070741851644054915, -0.3996062992125986035, -0.7152230971128609172 ) ) ;
#35670=CARTESIAN_POINT ( 'NONE',  ( 0.1058382717557500713, -0.3949938075777409408, 0.07217847769028866434 ) ) ;
#35676=CARTESIAN_POINT ( 'NONE',  ( -0.1974969037888704149, -0.3420746716998661063, -0.9297900262467193588 ) ) ;
#35681=CARTESIAN_POINT ( 'NONE',  ( -0.2362204724409451284, 0.4091458600556402425, -1.115485564304461885 ) ) ;
#35682=CARTESIAN_POINT ( 'NONE',  ( -0.1070741851644057135, 0.3996062992125985480, -2.368766404199475151 ) ) ;
#35686=CARTESIAN_POINT ( 'NONE',  ( -0.2867679344610367109, 0.2867679344610365444, -0.6463447750994246732 ) ) ;
#35697=CARTESIAN_POINT ( 'NONE',  ( -0.3917322834645669549, -0.1049643490035306603, -0.8254593175853015552 ) ) ;
#35700=CARTESIAN_POINT ( 'NONE',  ( -0.1058382717557497937, -0.3949938075777411628, -1.174540682414698223 ) ) ;
#35716=CARTESIAN_POINT ( 'NONE',  ( 0.3460692066303959202, 0.1998031496062993295, -1.706036745406824151 ) ) ;
#35719=CARTESIAN_POINT ( 'NONE',  ( -0.1998031496062991630, -0.3460692066303959202, -1.087270341207349000 ) ) ;
#35723=CARTESIAN_POINT ( 'NONE',  ( 0.4091458600556403535, 0.2362204724409449896, -0.2887139107611548794 ) ) ;
#35724=CARTESIAN_POINT ( 'NONE',  ( 0.3917322834645670104, -0.1049643490035303411, -2.715879265091863726 ) ) ;
#35730=CARTESIAN_POINT ( 'NONE',  ( 0.2362204724409449064, 0.4091458600556404646, -2.425853018372703396 ) ) ;
#35734=CARTESIAN_POINT ( 'NONE',  ( -0.3420746716998662729, 0.1974969037888702206, -1.835301837270341130 ) ) ;
#35744=CARTESIAN_POINT ( 'NONE',  ( -0.3392501089628019439, 0.1958661417322832554, -2.468484621226035181 ) ) ;
#35760=CARTESIAN_POINT ( 'NONE',  ( 0.3996062992125985480, 2.446882876249141654E-17, -0.1948818897637795422 ) ) ;
#35762=CARTESIAN_POINT ( 'NONE',  ( 0.3917322834645669549, 0.1049643490035304660, -1.784120734908136274 ) ) ;
#35771=CARTESIAN_POINT ( 'NONE',  ( 0.3996062992125984925, 0.1070741851644054637, -0.9888451443569553634 ) ) ;
#35774=ORIENTED_EDGE ( 'NONE', *, *, #59249, .F. ) ;
#35779=CARTESIAN_POINT ( 'NONE',  ( -0.3917322834645671215, 0.1049643490035301469, -1.534776902887139194 ) ) ;
#35783=CARTESIAN_POINT ( 'NONE',  ( -0.1958661417322836718, 0.3392501089628017219, -2.682414698162729483 ) ) ;
#35785=CARTESIAN_POINT ( 'NONE',  ( -0.3996062992125986035, 0.1070741851644051584, -2.471784776902886893 ) ) ;
#35788=CARTESIAN_POINT ( 'NONE',  ( 4.893765752498283924E-17, -0.3996062992125986035, -0.3937007874015748254 ) ) ;
#35792=CARTESIAN_POINT ( 'NONE',  ( 0.1958661417322834775, 0.3392501089628018884, -2.183727034120734878 ) ) ;
#35802=CARTESIAN_POINT ( 'NONE',  ( 0.3917322834645669549, 2.398668435337827645E-17, -1.615466248522622550 ) ) ;
#35807=CARTESIAN_POINT ( 'NONE',  ( -0.2867679344610364334, -0.2867679344610367109, 0.1062992125984252439 ) ) ;
#35810=CARTESIAN_POINT ( 'NONE',  ( -0.2891555358219908833, -0.2891555358219912164, 0.09842519685039366473 ) ) ;
#35819=CARTESIAN_POINT ( 'NONE',  ( -0.1958661417322836995, 0.3392501089628017219, -1.427184670112547682 ) ) ;
#35821=CARTESIAN_POINT ( 'NONE',  ( 0.1049643490035304938, -0.3917322834645669549, -2.217191601049868677 ) ) ;
#35826=CARTESIAN_POINT ( 'NONE',  ( 0.3996062992125986035, 0.1070741851644054776, -0.4396325459317584339 ) ) ;
#35828=CARTESIAN_POINT ( 'NONE',  ( 0.3996062992125986035, -0.1070741851644052972, 0.1266404199475065218 ) ) ;
#35830=CARTESIAN_POINT ( 'NONE',  ( -0.3996062992125987146, 0.1070741851644051862, -2.237532808398950301 ) ) ;
#35835=CARTESIAN_POINT ( 'NONE',  ( -0.2362204724409451284, 0.4091458600556402425, -1.192257217847769057 ) ) ;
#35838=CARTESIAN_POINT ( 'NONE',  ( -0.1974969037888704149, -0.3420746716998661063, -0.7723097112860893843 ) ) ;
#35851=CARTESIAN_POINT ( 'NONE',  ( -0.3996062992125984925, -0.1070741851644056858, -1.225065616797899937 ) ) ;
#35854=CARTESIAN_POINT ( 'NONE',  ( -0.3917322834645669549, -0.1049643490035306603, -1.140419947506561282 ) ) ;
#35858=CARTESIAN_POINT ( 'NONE',  ( -0.3902087894128231649, -0.03611438844012619664, 1.721458645558462781E-17 ) ) ;
#35883=CARTESIAN_POINT ( 'NONE',  ( 0.2925321140481932369, -0.2925321140481931814, -1.043307086614173151 ) ) ;
#35887=CARTESIAN_POINT ( 'NONE',  ( 0.3458507752293908943, 0.3458507752293908943, 0.01968503937007874335 ) ) ;
#35888=CARTESIAN_POINT ( 'NONE',  ( -0.1058382717557497937, -0.3949938075777411628, -2.276902887139107712 ) ) ;
#35891=CARTESIAN_POINT ( 'NONE',  ( 0.1049643490035303689, 0.3917322834645670104, -0.9304461942257216123 ) ) ;
#35893=CARTESIAN_POINT ( 'NONE',  ( -1.157146581871515012E-16, 0.4724409448818898682, -2.519685039370078705 ) ) ;
#35894=CARTESIAN_POINT ( 'NONE',  ( -0.2362204724409451284, 0.4091458600556402425, -0.8772965879265091083 ) ) ;
#35900=CARTESIAN_POINT ( 'NONE',  ( -0.3917322834645670659, 0.1049643490035301607, -0.4278022065278722641 ) ) ;
#35905=( BOUNDED_CURVE ( )  B_SPLINE_CURVE ( 2, ( #48598, #36390, #68796, #35985, #11558, #29660, #54914, #11141, #62476, #61655, #24167, #49836, #3996, #4811, #62064, #75535, #4403, #30487, #37215, #62894, #18283, #43926, #69622, #35567, #22932, #25812, #46000, #26660, #24980, #77601, #57792, #58213, #38861, #18688, #38033, #57381, #579, #63708, #64542, #45160, #51472, #51896, #32135, #77175, #6465, #37622, #7301, #50654, #63298, #19506, #51060, #32970, #5636, #19090, #38447, #58638, #31303, #44739, #26233, #64131, #78020, #12375, #44331, #70865, #6879, #76356, #1006, #13215, #19935, #70022, #6048, #159, #56967, #31720, #83075, #25396, #32549, #76760, #45584, #70434, #82665, #12791, #11967, #52313, #71277, #13626, #39278, #64965, #20348, #54395, #33809, #65396, #80106, #59887, #72941, #1827, #60718, #14471, #40125, #2241, #22425, #8558, #53979, #8144, #78442, #66634, #67049, #28318, #21590, #53566, #7732, #27906, #72532, #27487, #40540, #79691, #34226, #79275, #66220, #14050, #9382, #35052, #33399, #47252, #15711, #20768, #22008, #15293, #47668, #3067, #40954, #8971, #34645, #60310, #72113, #14880, #41368, #2659, #73362, #28734, #71696, #46421, #59474, #39704, #59061, #1416, #27072, #53145, #46838, #52731, #65811, #78858, #21183, #61552, #16538, #11451, #30791, #3480, #5126, #35883, #67459, #54815, #56457, #29147, #61960, #62792, #4704, #16120, #69103, #3896, #81752, #80517, #55628, #81337, #24063, #35465, #43403, #42183, #73784, #42999, #62366, #49732, #67878, #75431, #41766, #36691, #30377 ),
 .UNSPECIFIED., .F., .F. ) 
 B_SPLINE_CURVE_WITH_KNOTS ( ( 3, 2, 2, 2, 2, 2, 2, 2, 2, 2, 2, 2, 2, 2, 2, 2, 2, 2, 2, 2, 2, 2, 2, 2, 2, 2, 2, 2, 2, 2, 2, 2, 2, 2, 2, 2, 2, 2, 2, 2, 2, 2, 2, 2, 2, 2, 2, 2, 2, 2, 2, 2, 2, 2, 2, 2, 2, 2, 2, 2, 2, 2, 2, 2, 2, 2, 2, 2, 2, 2, 2, 2, 2, 2, 2, 2, 2, 2, 2, 2, 2, 2, 2, 2, 2, 2, 2, 2, 2, 2, 2, 2, 2, 3 ),
 ( 0.05000000000000000278, 0.05416666666666666852, 0.05833333333333333426, 0.06250000000000000000, 0.06666666666666666574, 0.07083333333333333148, 0.07499999999999999722, 0.07916666666666666297, 0.08333333333333332871, 0.08749999999999999445, 0.09166666666666664631, 0.09583333333333333981, 0.1000000000000000056, 0.1041666666666666574, 0.1083333333333333370, 0.1124999999999999889, 0.1166666666666666546, 0.1208333333333333204, 0.1249999999999999861, 0.1291666666666666519, 0.1333333333333333037, 0.1375000000000000111, 0.1416666666666666630, 0.1458333333333333148, 0.1499999999999999667, 0.1541666666666666741, 0.1583333333333333259, 0.1624999999999999778, 0.1666666666666666297, 0.1708333333333333093, 0.1749999999999999611, 0.1791666666666666408, 0.1833333333333332926, 0.1875000000000000000, 0.1916666666666666519, 0.1958333333333333037, 0.2000000000000000111, 0.2041666666666666630, 0.2083333333333333148, 0.2124999999999999667, 0.2166666666666666741, 0.2208333333333333259, 0.2249999999999999778, 0.2291666666666666297, 0.2333333333333333370, 0.2374999999999999889, 0.2416666666666666408, 0.2458333333333332926, 0.2500000000000000000, 0.2541666666666666519, 0.2583333333333333592, 0.2624999999999999556, 0.2666666666666666630, 0.2708333333333333148, 0.2750000000000000222, 0.2791666666666666741, 0.2833333333333333259, 0.2874999999999999223, 0.2916666666666666297, 0.2958333333333333370, 0.2999999999999999889, 0.3041666666666665853, 0.3083333333333332926, 0.3125000000000000000, 0.3166666666666665964, 0.3208333333333333037, 0.3249999999999999556, 0.3291666666666666075, 0.3333333333333332593, 0.3374999999999999667, 0.3416666666666666741, 0.3458333333333332704, 0.3499999999999999223, 0.3541666666666666297, 0.3583333333333332815, 0.3624999999999999334, 0.3666666666666665853, 0.3708333333333332926, 0.3749999999999999445, 0.3791666666666665964, 0.3833333333333333592, 0.3874999999999999556, 0.3916666666666666075, 0.3958333333333333148, 0.3999999999999999667, 0.4041666666666666186, 0.4083333333333332149, 0.4124999999999999223, 0.4166666666666666852, 0.4208333333333332815, 0.4249999999999999334, 0.4291666666666665853, 0.4333333333333332926, 0.4374999999999999445 ),
 .UNSPECIFIED. ) 
 CURVE ( )  GEOMETRIC_REPRESENTATION_ITEM ( )  RATIONAL_B_SPLINE_CURVE ( ( 1.000000000000000000, 0.9659258262890683122, 1.000000000000000000, 0.9659258262890683122, 1.000000000000000000, 0.9659258262890683122, 1.000000000000000000, 0.9659258262890683122, 1.000000000000000000, 0.9659258262890683122, 1.000000000000000000, 0.9659258262890683122, 1.000000000000000000, 0.9659258262890683122, 1.000000000000000000, 0.9659258262890683122, 1.000000000000000000, 0.9659258262890683122, 1.000000000000000000, 0.9659258262890683122, 1.000000000000000000, 0.9659258262890683122, 1.000000000000000000, 0.9659258262890683122, 1.000000000000000000, 0.9659258262890683122, 1.000000000000000000, 0.9659258262890683122, 1.000000000000000000, 0.9659258262890683122, 1.000000000000000000, 0.9659258262890683122, 1.000000000000000000, 0.9659258262890683122, 1.000000000000000000, 0.9659258262890683122, 1.000000000000000000, 0.9659258262890683122, 1.000000000000000000, 0.9659258262890683122, 1.000000000000000000, 0.9659258262890683122, 1.000000000000000000, 0.9659258262890683122, 1.000000000000000000, 0.9659258262890683122, 1.000000000000000000, 0.9659258262890683122, 1.000000000000000000, 0.9659258262890683122, 1.000000000000000000, 0.9659258262890683122, 1.000000000000000000, 0.9659258262890683122, 1.000000000000000000, 0.9659258262890683122, 1.000000000000000000, 0.9659258262890683122, 1.000000000000000000, 0.9659258262890683122, 1.000000000000000000, 0.9659258262890683122, 1.000000000000000000, 0.9659258262890683122, 1.000000000000000000, 0.9659258262890683122, 1.000000000000000000, 0.9659258262890683122, 1.000000000000000000, 0.9659258262890683122, 1.000000000000000000, 0.9659258262890683122, 1.000000000000000000, 0.9659258262890683122, 1.000000000000000000, 0.9659258262890683122, 1.000000000000000000, 0.9659258262890683122, 1.000000000000000000, 0.9659258262890683122, 1.000000000000000000, 0.9659258262890683122, 1.000000000000000000, 0.9659258262890683122, 1.000000000000000000, 0.9659258262890683122, 1.000000000000000000, 0.9659258262890683122, 1.000000000000000000, 0.9659258262890683122, 1.000000000000000000, 0.9659258262890683122, 1.000000000000000000, 0.9659258262890683122, 1.000000000000000000, 0.9659258262890683122, 1.000000000000000000, 0.9659258262890683122, 1.000000000000000000, 0.9659258262890683122, 1.000000000000000000, 0.9659258262890683122, 1.000000000000000000, 0.9659258262890683122, 1.000000000000000000, 0.9659258262890683122, 1.000000000000000000, 0.9659258262890683122, 1.000000000000000000, 0.9659258262890683122, 1.000000000000000000, 0.9659258262890683122, 1.000000000000000000, 0.9659258262890683122, 1.000000000000000000, 0.9659258262890683122, 1.000000000000000000, 0.9659258262890683122, 1.000000000000000000, 0.9659258262890683122, 1.000000000000000000, 0.9659258262890683122, 1.000000000000000000, 0.9659258262890683122, 1.000000000000000000, 0.9659258262890683122, 1.000000000000000000, 0.9659258262890683122, 1.000000000000000000, 0.9659258262890683122, 1.000000000000000000, 0.9659258262890683122, 1.000000000000000000, 0.9659258262890683122, 1.000000000000000000, 0.9659258262890683122, 1.000000000000000000, 0.9659258262890683122, 1.000000000000000000, 0.9659258262890683122, 1.000000000000000000, 0.9659258262890683122, 1.000000000000000000, 0.9659258262890683122, 1.000000000000000000, 0.9659258262890683122, 1.000000000000000000, 0.9659258262890683122, 1.000000000000000000, 0.9659258262890683122, 1.000000000000000000, 0.9659258262890683122, 1.000000000000000000, 0.9659258262890683122, 1.000000000000000000, 0.9659258262890683122, 1.000000000000000000, 0.9659258262890683122, 1.000000000000000000, 0.9659258262890683122, 1.000000000000000000, 0.9659258262890683122, 1.000000000000000000, 0.9659258262890683122, 1.000000000000000000, 0.9659258262890683122, 1.000000000000000000, 0.9659258262890683122, 1.000000000000000000, 0.9659258262890683122, 1.000000000000000000, 0.9659258262890683122, 1.000000000000000000, 0.9659258262890683122, 1.000000000000000000, 0.9659258262890683122, 1.000000000000000000, 0.9659258262890683122, 1.000000000000000000, 0.9659258262890683122, 1.000000000000000000, 0.9659258262890683122, 1.000000000000000000, 0.9659258262890683122, 1.000000000000000000, 0.9659258262890687563, 0.9999999999999995559 ) ) 
 REPRESENTATION_ITEM ( '' )  );
#35909=CARTESIAN_POINT ( 'NONE',  ( -0.1049643490035302301, -0.3917322834645671770, -1.486239788222784020 ) ) ;
#35916=CARTESIAN_POINT ( 'NONE',  ( -0.1958661417322834220, -0.3392501089628018884, -1.095144356955380704 ) ) ;
#35925=CARTESIAN_POINT ( 'NONE',  ( -0.3917322834645670104, -7.196005306013484475E-17, -2.551181102362204633 ) ) ;
#35927=ORIENTED_EDGE ( 'NONE', *, *, #50646, .T. ) ;
#35932=CARTESIAN_POINT ( 'NONE',  ( -0.3392501089628019995, 0.1958661417322832277, -0.7408136482939633449 ) ) ;
#35934=CARTESIAN_POINT ( 'NONE',  ( 0.3969271875946612238, 0.02899565511876848675, -1.929133858267718660 ) ) ;
#35935=CARTESIAN_POINT ( 'NONE',  ( 0.1070741851644054776, -0.3996062992125984925, -2.524278215223096478 ) ) ;
#35953=CARTESIAN_POINT ( 'NONE',  ( -0.1958661417322836440, 0.3392501089628016664, -1.667959686842832356 ) ) ;
#35962=CARTESIAN_POINT ( 'NONE',  ( -0.1049643490035302301, -0.3917322834645671770, -0.3838775834983745860 ) ) ;
#35965=CARTESIAN_POINT ( 'NONE',  ( -0.1265901696524993347, 0.4724409448818895907, -1.973097112860892510 ) ) ;
#35985=CARTESIAN_POINT ( 'NONE',  ( -0.2925321140481932369, 0.2925321140481931814, -0.01968503937007875723 ) ) ;
#35986=CARTESIAN_POINT ( 'NONE',  ( -0.3460692066303957537, -0.1998031496062994405, -2.333989501312335957 ) ) ;
#35991=CARTESIAN_POINT ( 'NONE',  ( 0.1070741851644054915, -0.3996062992125986035, -1.660104986876640210 ) ) ;
#35992=CARTESIAN_POINT ( 'NONE',  ( 0.1974969037888704704, 0.3420746716998660508, -0.9317585301837268963 ) ) ;
#35993=CARTESIAN_POINT ( 'NONE',  ( 0.3996062992125986590, -0.1070741851644053111, -2.473753280839894764 ) ) ;
#35995=CARTESIAN_POINT ( 'NONE',  ( -0.3392501089628017219, -0.1958661417322836718, -0.04461942257217842850 ) ) ;
#35999=CARTESIAN_POINT ( 'NONE',  ( -0.1974969037888704149, -0.3420746716998661063, -2.032152230971128848 ) ) ;
#36003=CARTESIAN_POINT ( 'NONE',  ( -0.4724409448818895907, -0.1265901696524993070, -2.408136482939632561 ) ) ;
#36004=CARTESIAN_POINT ( 'NONE',  ( -0.3460692066303960868, 0.1998031496062990242, -1.601049868766404094 ) ) ;
#36011=CARTESIAN_POINT ( 'NONE',  ( 0.2867679344610365999, 0.2867679344610365999, 0.09251968503937001154 ) ) ;
#36017=CARTESIAN_POINT ( 'NONE',  ( -0.2867679344610365999, 0.2867679344610364889, 0.05314960629921249707 ) ) ;
#36019=CARTESIAN_POINT ( 'NONE',  ( -0.1958661417322834220, -0.3392501089628018884, -2.419947506561679784 ) ) ;
#36022=CARTESIAN_POINT ( 'NONE',  ( -0.2891555358219911054, 0.2891555358219909388, -2.854330708661418026 ) ) ;
#36026=CARTESIAN_POINT ( 'NONE',  ( -0.1070741851644051862, -0.3996062992125987146, -0.8595800524934383846 ) ) ;
#36028=CARTESIAN_POINT ( 'NONE',  ( 0.002674255378541693599, -0.3979867861068596691, -2.755905511811025388 ) ) ;
#36029=CARTESIAN_POINT ( 'NONE',  ( -9.594673741351313045E-17, 0.3917322834645670104, -0.5570866141732284671 ) ) ;
#36035=CARTESIAN_POINT ( 'NONE',  ( 0.3392501089628018884, -0.1958661417322834220, -0.2545931758530183275 ) ) ;
#36039=CYLINDRICAL_SURFACE ( 'NONE', #60866, 0.4724409448818898682 ) ;
#36041=CARTESIAN_POINT ( 'NONE',  ( 0.4724409448818897572, -0.1265901696524988906, -1.686351706036745446 ) ) ;
#36051=CARTESIAN_POINT ( 'NONE',  ( -0.3917322834645670659, 0.1049643490035301607, 0.2021190533146474677 ) ) ;
#36054=CARTESIAN_POINT ( 'NONE',  ( -0.3392501089628019995, 0.1958661417322832277, -0.4258530183727035068 ) ) ;
#36059=CARTESIAN_POINT ( 'NONE',  ( -0.3917322834645669549, -0.1049643490035306603, -2.242782152230970993 ) ) ;
#36062=CARTESIAN_POINT ( 'NONE',  ( 0.4091458600556403535, 0.2362204724409449896, -0.6804461942257218343 ) ) ;
#36070=CARTESIAN_POINT ( 'NONE',  ( 0.4091458600556403535, 0.2362204724409449896, -0.2887139107611548794 ) ) ;
#36074=CARTESIAN_POINT ( 'NONE',  ( -0.3996062992125984925, -0.1070741851644056858, -2.169947506561679340 ) ) ;
#36082=CARTESIAN_POINT ( 'NONE',  ( -0.3460692066303960313, 0.1998031496062989965, -0.4179790026246719137 ) ) ;
#36083=CARTESIAN_POINT ( 'NONE',  ( -0.3996062992125987146, 0.1070741851644051862, -0.5052493438320209140 ) ) ;
#36084=CARTESIAN_POINT ( 'NONE',  ( 0.3917322834645670659, -0.1049643490035303273, -2.942932701608610646 ) ) ;
#36090=CARTESIAN_POINT ( 'NONE',  ( -0.1058382717557503072, 0.3949938075777408852, -1.028215223097112885 ) ) ;
#36095=CARTESIAN_POINT ( 'NONE',  ( -0.4091458600556402980, -0.2362204724409451284, -1.154855643044619518 ) ) ;
#36096=CARTESIAN_POINT ( 'NONE',  ( 0.3996062992125986035, 2.446882876249141962E-17, -2.165354330708661568 ) ) ;
#36099=CARTESIAN_POINT ( 'NONE',  ( -0.1958661417322836995, 0.3392501089628017219, -0.9547437252306580913 ) ) ;
#36110=CARTESIAN_POINT ( 'NONE',  ( 0.3917322834645670104, 2.398668435337828261E-17, -0.8976377952755905110 ) ) ;
#36113=CARTESIAN_POINT ( 'NONE',  ( 0.3420746716998660508, -0.1974969037888703871, -1.522309711286089273 ) ) ;
#36123=CARTESIAN_POINT ( 'NONE',  ( 0.3458507752293908943, -0.3458507752293908943, -0.6476377952755905110 ) ) ;
#36128=CARTESIAN_POINT ( 'NONE',  ( 0.1998031496062994405, -0.3460692066303958092, -1.824146981627296604 ) ) ;
#36131=CARTESIAN_POINT ( 'NONE',  ( -0.3460692066303957537, -0.1998031496062994405, -1.704068241469816058 ) ) ;
#36135=CARTESIAN_POINT ( 'NONE',  ( -0.4091458600556402980, -0.2362204724409451284, -0.5249343832020997302 ) ) ;
#36138=CARTESIAN_POINT ( 'NONE',  ( 0.1049643490035304938, -0.3917322834645669549, -2.374671916010498762 ) ) ;
#36144=CARTESIAN_POINT ( 'NONE',  ( -0.1265901696524993347, 0.4724409448818895907, -2.445538057742782101 ) ) ;
#36146=CARTESIAN_POINT ( 'NONE',  ( -0.1974969037888706924, 0.3420746716998658843, -1.979658792650919041 ) ) ;
#36156=CARTESIAN_POINT ( 'NONE',  ( -0.2867679344610366554, 0.2867679344610365444, -2.461922941436009094 ) ) ;
#36168=CARTESIAN_POINT ( 'NONE',  ( 0.1070741851644054776, -0.3996062992125984925, -0.6345144356955381149 ) ) ;
#36170=CARTESIAN_POINT ( 'NONE',  ( -9.594673741351313045E-17, 0.3917322834645670104, -1.816929133858267820 ) ) ;
#36180=CARTESIAN_POINT ( 'NONE',  ( 0.3996062992125984925, 0.1070741851644054637, -1.461286089238845065 ) ) ;
#36182=CARTESIAN_POINT ( 'NONE',  ( -0.3458507752293909498, 0.3458507752293908388, -2.616141732283464361 ) ) ;
#36187=CARTESIAN_POINT ( 'NONE',  ( 0.1049643490035303689, 0.3917322834645670104, -1.652887139107611425 ) ) ;
#36193=CARTESIAN_POINT ( 'NONE',  ( 0.1998031496062994128, -0.3460692066303957537, -2.215879265091863726 ) ) ;
#36196=CARTESIAN_POINT ( 'NONE',  ( 0.2925321140481932369, 0.2925321140481932369, -0.9251968503937008093 ) ) ;
#36199=CARTESIAN_POINT ( 'NONE',  ( 0.3917322834645669549, 0.1049643490035304660, -2.479002624671915900 ) ) ;
#36210=CARTESIAN_POINT ( 'NONE',  ( 0.3917322834645669549, 2.398668435337827645E-17, -2.087907193404512363 ) ) ;
#36213=CARTESIAN_POINT ( 'NONE',  ( -0.2867679344610365999, 0.2867679344610364889, -2.781496062992125040 ) ) ;
#36215=ORIENTED_EDGE ( 'NONE', *, *, #53092, .F. ) ;
#36216=CARTESIAN_POINT ( 'NONE',  ( 0.1974969037888704704, 0.3420746716998660508, 0.01312335958005243601 ) ) ;
#36224=CARTESIAN_POINT ( 'NONE',  ( -0.3392501089628019995, 0.1958661417322831999, -1.125347399771340573 ) ) ;
#36226=CARTESIAN_POINT ( 'NONE',  ( 0.1958661417322834775, 0.3392501089628018884, -2.276246719160105236 ) ) ;
#36231=CARTESIAN_POINT ( 'NONE',  ( -0.2925321140481930704, -0.2925321140481933480, -0.3740157480314960092 ) ) ;
#36233=CARTESIAN_POINT ( 'NONE',  ( 0.3460692066303959202, -0.1998031496062991630, 0.1332020997375328031 ) ) ;
#36235=CARTESIAN_POINT ( 'NONE',  ( 0.3996062992125986035, 0.1070741851644054776, -2.171916010498687211 ) ) ;
#36240=CARTESIAN_POINT ( 'NONE',  ( 0.2362204724409451007, -0.4091458600556402980, -0.9560367454068241511 ) ) ;
#36244=CARTESIAN_POINT ( 'NONE',  ( -0.3949938075777409963, -7.255918531996591613E-17, -0.4311023622047245318 ) ) ;
#36258=CARTESIAN_POINT ( 'NONE',  ( 0.3996062992125984925, 0.1070741851644054637, -1.618766404199474929 ) ) ;
#36260=CARTESIAN_POINT ( 'NONE',  ( -0.1049643490035302024, -0.3917322834645671215, -1.639107611548556109 ) ) ;
#36262=CARTESIAN_POINT ( 'NONE',  ( -0.3857315817373087041, 0.06912221444360990008, -1.138966262901371687E-17 ) ) ;
#36281=CARTESIAN_POINT ( 'NONE',  ( -0.1049643490035302301, -0.3917322834645671770, -1.958680733104674276 ) ) ;
#36291=CARTESIAN_POINT ( 'NONE',  ( 4.893765752498283924E-17, -0.3996062992125986035, -2.913385826771653697 ) ) ;
#36292=CARTESIAN_POINT ( 'NONE',  ( 0.1974969037888704704, 0.3420746716998660508, -2.821522309711286258 ) ) ;
#36295=CARTESIAN_POINT ( 'NONE',  ( -0.1958661417322836718, 0.3392501089628017219, -1.422572178477690574 ) ) ;
#36297=CARTESIAN_POINT ( 'NONE',  ( -0.2362204724409447953, -0.4091458600556404646, -2.585301837270341352 ) ) ;
#36298=CARTESIAN_POINT ( 'NONE',  ( 0.4724409448818897017, 0.1265901696524990294, -0.8313648293963252778 ) ) ;
#36303=CARTESIAN_POINT ( 'NONE',  ( 0.1049643490035304522, -0.3917322834645668994, -0.4802956448480821261 ) ) ;
#36310=CARTESIAN_POINT ( 'NONE',  ( -0.1958661417322833942, -0.3392501089628018884, -1.637158423393387796 ) ) ;
#36317=CARTESIAN_POINT ( 'NONE',  ( 0.2867679344610365999, 0.2867679344610365999, -0.8523622047244096001 ) ) ;
#36328=CARTESIAN_POINT ( 'NONE',  ( 0.3917322834645670104, 2.398668435337828261E-17, -2.157480314960630086 ) ) ;
#36335=CARTESIAN_POINT ( 'NONE',  ( 0.3917322834645670104, -0.1049643490035303411, -0.6686351706036747222 ) ) ;
#36338=CARTESIAN_POINT ( 'NONE',  ( -0.3996062992125985480, -7.340648628747423112E-17, -2.478346456692913868 ) ) ;
#36356=CARTESIAN_POINT ( 'NONE',  ( 0.1049643490035303689, 0.3917322834645668994, -1.648274647472754095 ) ) ;
#36367=CARTESIAN_POINT ( 'NONE',  ( 0.3392501089628018329, 0.1958661417322835607, -0.4429327016086107571 ) ) ;
#36371=CARTESIAN_POINT ( 'NONE',  ( -0.2362204724409447953, -0.4091458600556404646, -2.189632545931758489 ) ) ;
#36386=VERTEX_POINT ( 'NONE', #50622 ) ;
#36390=CARTESIAN_POINT ( 'NONE',  ( -0.1070741851644057135, 0.3996062992125985480, -0.006561679790026264843 ) ) ;
#36391=CARTESIAN_POINT ( 'NONE',  ( -0.2925321140481932369, 0.2925321140481931259, -2.143700787401574548 ) ) ;
#36396=CARTESIAN_POINT ( 'NONE',  ( -0.3996062992125986035, -0.1070741851644056997, -1.620734908136482799 ) ) ;
#36397=CARTESIAN_POINT ( 'NONE',  ( -0.1974969037888706647, 0.3420746716998658843, -0.9580052493438320216 ) ) ;
#36398=CARTESIAN_POINT ( 'NONE',  ( 0.3996062992125986035, 2.446882876249141962E-17, -2.637795275590551380 ) ) ;
#36399=CARTESIAN_POINT ( 'NONE',  ( 0.4724409448818898682, 2.892866454678787531E-17, -0.5905511811023621549 ) ) ;
#36400=CARTESIAN_POINT ( 'NONE',  ( -0.3917322834645669549, -0.1049643490035306603, -0.5104986876640419391 ) ) ;
#36404=CARTESIAN_POINT ( 'NONE',  ( -0.2891555358219911054, 0.2891555358219909388, -2.301181102362205078 ) ) ;
#36407=CARTESIAN_POINT ( 'NONE',  ( 0.1265901696524989462, 0.4724409448818897572, -2.355643044619422533 ) ) ;
#36408=CARTESIAN_POINT ( 'NONE',  ( 0.3460692066303959202, 0.1998031496062993295, -1.706036745406824151 ) ) ;
#36417=CARTESIAN_POINT ( 'NONE',  ( -9.594673741351313045E-17, 0.3917322834645670104, 0.2303149606299211838 ) ) ;
#36418=DIRECTION ( 'NONE',  ( -0.000000000000000000, -0.000000000000000000, 1.000000000000000000 ) ) ;
#36424=CARTESIAN_POINT ( 'NONE',  ( -0.3917322834645671215, 0.1049643490035301469, 0.04002624671916000382 ) ) ;
#36426=CARTESIAN_POINT ( 'NONE',  ( -9.594673741351313045E-17, 0.3917322834645670104, -2.354330708661417138 ) ) ;
#36429=CARTESIAN_POINT ( 'NONE',  ( -0.3420746716998659953, -0.1974969037888706647, -2.572178477690288734 ) ) ;
#36433=CARTESIAN_POINT ( 'NONE',  ( 0.1070741851644054915, -0.3996062992125986035, -1.187664041994750619 ) ) ;
#36434=CYLINDRICAL_SURFACE ( 'NONE', #59930, 0.4724409448818898682 ) ;
#36438=CARTESIAN_POINT ( 'NONE',  ( -0.3917322834645670104, -7.196005306013484475E-17, -0.2814960629921260393 ) ) ;
#36444=CARTESIAN_POINT ( 'NONE',  ( -0.2867679344610365999, 0.2867679344610364889, -0.1692913385826771144 ) ) ;
#36445=ORIENTED_EDGE ( 'NONE', *, *, #67062, .T. ) ;
#36448=CARTESIAN_POINT ( 'NONE',  ( 0.4724409448818896462, 0.1265901696524990294, -1.699475065616798064 ) ) ;
#36450=CARTESIAN_POINT ( 'NONE',  ( 0.3392501089628018329, 0.1958661417322835607, -2.735564304461941987 ) ) ;
#36457=CARTESIAN_POINT ( 'NONE',  ( 0.3917322834645668994, -0.1049643490035303134, -0.1915817340869272467 ) ) ;
#36459=CARTESIAN_POINT ( 'NONE',  ( -0.3917322834645670104, -7.196005306013484475E-17, -0.2814960629921260393 ) ) ;
#36464=CARTESIAN_POINT ( 'NONE',  ( -0.3392501089628019995, 0.1958661417322832277, -2.538057742782152015 ) ) ;
#36467=CARTESIAN_POINT ( 'NONE',  ( -0.4091458600556402980, -0.2362204724409451284, -0.6017060367454067915 ) ) ;
#36479=CARTESIAN_POINT ( 'NONE',  ( -0.3996062992125985480, -7.340648628747423112E-17, -1.848425196850393526 ) ) ;
#36487=CARTESIAN_POINT ( 'NONE',  ( -0.3460692066303957537, -0.1998031496062994405, -0.4442257217847768724 ) ) ;
#36488=CARTESIAN_POINT ( 'NONE',  ( -0.1070741851644051862, -0.3996062992125987146, -0.3871391076115485719 ) ) ;
#36489=CARTESIAN_POINT ( 'NONE',  ( 0.3420746716998660508, -0.1974969037888703871, 0.05249343832020991057 ) ) ;
#36494=CARTESIAN_POINT ( 'NONE',  ( -0.3949938075777409963, -7.255918531996591613E-17, -1.061023622047243986 ) ) ;
#36500=CARTESIAN_POINT ( 'NONE',  ( -0.4724409448818895907, -0.1265901696524993070, -1.148293963254592986 ) ) ;
#36501=CARTESIAN_POINT ( 'NONE',  ( 0.3996062992125986035, 2.446882876249141962E-17, -2.480314960629921295 ) ) ;
#36504=CARTESIAN_POINT ( 'NONE',  ( -0.3392501089628019995, 0.1958661417322831999, -0.9678670848107107094 ) ) ;
#36516=CARTESIAN_POINT ( 'NONE',  ( 0.2867679344610365999, -0.2867679344610365444, -1.035433070866141447 ) ) ;
#36519=CARTESIAN_POINT ( 'NONE',  ( 0.1058382717557500713, -0.3949938075777409408, -1.502624671916010790 ) ) ;
#36530=CARTESIAN_POINT ( 'NONE',  ( -0.3392501089628019995, 0.1958661417322832277, -0.1108923884514436548 ) ) ;
#36536=CARTESIAN_POINT ( 'NONE',  ( -0.3460692066303960868, 0.1998031496062990242, -1.916010498687664043 ) ) ;
#36539=CARTESIAN_POINT ( 'NONE',  ( 0.3460692066303958092, 0.1998031496062993018, -1.625328083989501460 ) ) ;
#36543=CARTESIAN_POINT ( 'NONE',  ( 0.3458507752293908943, 0.3458507752293908943, -0.2952755905511811330 ) ) ;
#36545=CARTESIAN_POINT ( 'NONE',  ( -0.2867679344610364334, -0.2867679344610367109, -2.820866141732283339 ) ) ;
#36551=CARTESIAN_POINT ( 'NONE',  ( -0.4091458600556405756, 0.2362204724409446288, -2.465223097112860806 ) ) ;
#36553=CARTESIAN_POINT ( 'NONE',  ( -0.3949938075777411073, 0.1058382717557497660, -2.156824146981627610 ) ) ;
#36573=CARTESIAN_POINT ( 'NONE',  ( -9.787531504996566615E-17, 0.3996062992125985480, -0.7066929133858268486 ) ) ;
#36574=CARTESIAN_POINT ( 'NONE',  ( -0.1958661417322834220, -0.3392501089628018884, -2.197506561679789971 ) ) ;
#36590=CARTESIAN_POINT ( 'NONE',  ( 0.2867679344610365999, -0.2867679344610365444, -1.442913385826771755 ) ) ;
#36595=CARTESIAN_POINT ( 'NONE',  ( -0.1070741851644057135, 0.3996062992125984925, -2.445538057742782101 ) ) ;
#36597=CARTESIAN_POINT ( 'NONE',  ( -0.2925321140481930704, -0.2925321140481933480, -1.003937007874015741 ) ) ;
#36600=CARTESIAN_POINT ( 'NONE',  ( 4.797336870675656522E-17, -0.3917322834645670104, -2.590551181102362044 ) ) ;
#36610=CARTESIAN_POINT ( 'NONE',  ( 0.1958661417322836162, -0.3392501089628018329, -1.904180159283777485 ) ) ;
#36613=( BOUNDED_CURVE ( )  B_SPLINE_CURVE ( 2, ( #55112, #61443, #17264, #29454, #80416, #22728, #24367, #49626, #81649, #36182, #16432, #5024, #61025 ),
 .UNSPECIFIED., .F., .F. ) 
 B_SPLINE_CURVE_WITH_KNOTS ( ( 3, 2, 2, 2, 2, 2, 3 ),
 ( 0.8875000000000000666, 0.8916666666666668295, 0.8958333333333334814, 0.9000000000000001332, 0.9041666666666667851, 0.9083333333333334370, 0.9125000000000000888 ),
 .UNSPECIFIED. ) 
 CURVE ( )  GEOMETRIC_REPRESENTATION_ITEM ( )  RATIONAL_B_SPLINE_CURVE ( ( 0.9999999999999991118, 0.9659258262890692004, 1.000000000000000000, 0.9659258262890683122, 1.000000000000000000, 0.9659258262890683122, 1.000000000000000000, 0.9659258262890683122, 1.000000000000000000, 0.9659258262890683122, 1.000000000000000000, 0.9659258262890674240, 1.000000000000000888 ) ) 
 REPRESENTATION_ITEM ( '' )  );
#36614=CARTESIAN_POINT ( 'NONE',  ( 0.1958661417322834775, 0.3392501089628018884, -2.748687664041994605 ) ) ;
#36617=CARTESIAN_POINT ( 'NONE',  ( -0.3949938075777409408, -0.1058382717557502933, -0.04593175853018378885 ) ) ;
#36619=ORIENTED_EDGE ( 'NONE', *, *, #81291, .T. ) ;
#36626=CARTESIAN_POINT ( 'NONE',  ( 0.2867679344610366554, 0.2867679344610366554, -1.079415641241156854 ) ) ;
#36628=CARTESIAN_POINT ( 'NONE',  ( 0.1958661417322834775, 0.3392501089628018884, -2.748687664041994605 ) ) ;
#36634=CARTESIAN_POINT ( 'NONE',  ( -0.1998031496062991907, -0.3460692066303959757, -0.8530183727034120755 ) ) ;
#36636=CARTESIAN_POINT ( 'NONE',  ( 0.2925321140481932369, -0.2925321140481931814, -0.3326771653543306728 ) ) ;
#36638=CARTESIAN_POINT ( 'NONE',  ( -0.3460692066303958092, -0.1998031496062994683, -2.414698162729658648 ) ) ;
#36642=CARTESIAN_POINT ( 'NONE',  ( -0.1265901696524993347, 0.4724409448818895907, -1.028215223097112663 ) ) ;
#36645=CIRCLE ( 'NONE', #51402, 0.4724409448818898682 ) ;
#36646=CARTESIAN_POINT ( 'NONE',  ( -0.3949938075777408852, -0.1058382717557502933, -0.9101049868766403206 ) ) ;
#36648=CARTESIAN_POINT ( 'NONE',  ( 0.3458507752293908943, -0.3458507752293908943, -1.120078740157480324 ) ) ;
#36652=CYLINDRICAL_SURFACE ( 'NONE', #2327, 0.4724409448818898682 ) ;
#36658=CARTESIAN_POINT ( 'NONE',  ( 0.4724409448818898682, 0.000000000000000000, -2.755905511811024056 ) ) ;
#36659=CARTESIAN_POINT ( 'NONE',  ( 0.1070741851644054776, -0.3996062992125984925, -1.736876640419947826 ) ) ;
#36662=CARTESIAN_POINT ( 'NONE',  ( 4.797336870675656522E-17, -0.3917322834645670104, -1.330708661417322691 ) ) ;
#36676=CARTESIAN_POINT ( 'NONE',  ( 0.2362204724409451007, -0.4091458600556402980, -0.3261154855643044748 ) ) ;
#36691=CARTESIAN_POINT ( 'NONE',  ( 0.3996062992125979929, -0.1070741851644065740, -1.213910761154855411 ) ) ;
#36693=CARTESIAN_POINT ( 'NONE',  ( -0.1958661417322834220, -0.3392501089628018884, -2.104986876640420057 ) ) ;
#36696=CARTESIAN_POINT ( 'NONE',  ( -0.4091458600556402980, -0.2362204724409451284, -0.5249343832020997302 ) ) ;
#36697=CARTESIAN_POINT ( 'NONE',  ( 0.1058382717557500713, -0.3949938075777409408, -2.604986876640420501 ) ) ;
#36701=CARTESIAN_POINT ( 'NONE',  ( -9.594673741351313045E-17, 0.3917322834645670104, -1.251968503937008093 ) ) ;
#36703=CARTESIAN_POINT ( 'NONE',  ( 0.4724409448818898682, 2.892866454678787531E-17, -2.637795275590551380 ) ) ;
#36709=CARTESIAN_POINT ( 'NONE',  ( 0.3917322834645668994, 0.1049643490035304522, -0.8346263535094994301 ) ) ;
#36717=CARTESIAN_POINT ( 'NONE',  ( 0.1049643490035304799, -0.3917322834645670104, -1.971804092684726228 ) ) ;
#36723=CARTESIAN_POINT ( 'NONE',  ( -0.1049643490035302024, -0.3917322834645671215, -0.7867454068241470644 ) ) ;
#36734=CARTESIAN_POINT ( 'NONE',  ( -0.3392501089628017219, -0.1958661417322836718, -2.721784776902886893 ) ) ;
#36736=ORIENTED_EDGE ( 'NONE', *, *, #10612, .T. ) ;
#36741=CARTESIAN_POINT ( 'NONE',  ( -0.2867679344610365999, 0.2867679344610364889, -0.7342519685039372579 ) ) ;
#36742=CARTESIAN_POINT ( 'NONE',  ( -0.3458507752293909498, 0.3458507752293907833, 0.2185039370078740162 ) ) ;
#36744=CARTESIAN_POINT ( 'NONE',  ( -0.1070741851644051862, -0.3996062992125986590, -2.511154855643044748 ) ) ;
#36755=CARTESIAN_POINT ( 'NONE',  ( 0.1998031496062994128, -0.3460692066303957537, -0.3261154855643044748 ) ) ;
#36757=CARTESIAN_POINT ( 'NONE',  ( 0.3917322834645669549, 0.1049643490035304660, -0.2742782152230970327 ) ) ;
#36764=CARTESIAN_POINT ( 'NONE',  ( -0.3392501089628019439, 0.1958661417322832554, -1.838563361383515504 ) ) ;
#36774=CARTESIAN_POINT ( 'NONE',  ( -9.594673741351313045E-17, 0.3917322834645670659, -0.3116991058080859078 ) ) ;
#36778=CARTESIAN_POINT ( 'NONE',  ( 0.4724409448818897572, -0.1265901696524988906, -2.235564304461942431 ) ) ;
#36801=CARTESIAN_POINT ( 'NONE',  ( -0.3996062992125985480, -7.340648628747423112E-17, -2.635826771653543066 ) ) ;
#36806=CARTESIAN_POINT ( 'NONE',  ( 0.3460692066303959757, -0.1998031496062991907, -1.994750656167979086 ) ) ;
#36807=CARTESIAN_POINT ( 'NONE',  ( -0.1058382717557497937, -0.3949938075777411628, -1.332020997375328086 ) ) ;
#36811=CARTESIAN_POINT ( 'NONE',  ( -0.1049643490035307020, 0.3917322834645669549, -0.7860892388451442558 ) ) ;
#36815=CARTESIAN_POINT ( 'NONE',  ( -0.3949938075777408852, -0.1058382717557502933, -2.484908136482939955 ) ) ;
#36820=CARTESIAN_POINT ( 'NONE',  ( 0.1265901696524989462, 0.4724409448818897572, -2.513123359580052174 ) ) ;
#36821=CARTESIAN_POINT ( 'NONE',  ( -0.2925321140481930704, -0.2925321140481933480, -2.263779527559055094 ) ) ;
#36830=CARTESIAN_POINT ( 'NONE',  ( -0.3392501089628018329, -0.1958661417322836440, -2.652211655346770502 ) ) ;
#36837=CARTESIAN_POINT ( 'NONE',  ( -0.3392501089628017219, -0.1958661417322836718, 0.02034120734908127781 ) ) ;
#36838=CARTESIAN_POINT ( 'NONE',  ( 0.1049643490035303689, 0.3917322834645670104, -1.717847769028871596 ) ) ;
#36839=CARTESIAN_POINT ( 'NONE',  ( -0.3917322834645671215, 0.1049643490035301469, -2.387139107611548905 ) ) ;
#36843=CARTESIAN_POINT ( 'NONE',  ( -0.1058382717557503211, 0.3949938075777409408, -2.841207349081365408 ) ) ;
#36847=CARTESIAN_POINT ( 'NONE',  ( -0.3996062992125986035, -0.1070741851644056997, -1.148293963254592986 ) ) ;
#36849=CARTESIAN_POINT ( 'NONE',  ( -0.4724409448818898682, -8.678599364036362592E-17, -0.7460629921259841479 ) ) ;
#36852=CARTESIAN_POINT ( 'NONE',  ( -0.3917322834645671215, 0.1049643490035301469, -0.5898950131233595684 ) ) ;
#36857=CARTESIAN_POINT ( 'NONE',  ( 0.3917322834645669549, 0.1049643490035304660, -0.2742782152230970327 ) ) ;
#36862=CARTESIAN_POINT ( 'NONE',  ( 0.1265901696524990294, -0.4724409448818896462, -1.817585301837270517 ) ) ;
#36864=CARTESIAN_POINT ( 'NONE',  ( 0.1958661417322834775, 0.3392501089628018884, -2.748687664041994605 ) ) ;
#36871=CARTESIAN_POINT ( 'NONE',  ( 0.3392501089628018329, 0.1958661417322835052, -0.5262274033782657900 ) ) ;
#36873=CARTESIAN_POINT ( 'NONE',  ( 0.1049643490035303689, 0.3917322834645670104, -1.022965879265091749 ) ) ;
#36879=CARTESIAN_POINT ( 'NONE',  ( 0.1958661417322834775, 0.3392501089628018884, -2.183727034120734878 ) ) ;
#36882=CARTESIAN_POINT ( 'NONE',  ( -0.4091458600556402980, -0.2362204724409451284, -0.7591863517060367661 ) ) ;
#36887=AXIS2_PLACEMENT_3D ( 'NONE', #31937, #57598, #7949 ) ;
#36895=CARTESIAN_POINT ( 'NONE',  ( 0.1998031496062994128, -0.3460692066303957537, -1.900918635170603554 ) ) ;
#36903=CARTESIAN_POINT ( 'NONE',  ( -0.1998031496062991630, -0.3460692066303959202, -0.2998687664041995160 ) ) ;
#36904=CARTESIAN_POINT ( 'NONE',  ( -0.3460692066303958092, -0.1998031496062994683, -0.3674540682414698112 ) ) ;
#36905=CARTESIAN_POINT ( 'NONE',  ( 0.2891555358219910499, -0.2891555358219909944, -0.2559055118110237226 ) ) ;
#36911=CARTESIAN_POINT ( 'NONE',  ( 0.3949938075777409963, 2.418639510665530743E-17, -0.9822834645669292764 ) ) ;
#36916=CARTESIAN_POINT ( 'NONE',  ( -0.4091458600556402980, -0.2362204724409451284, -0.9973753280839895430 ) ) ;
#36917=CARTESIAN_POINT ( 'NONE',  ( -0.1070741851644057135, 0.3996062992125985480, -2.526246719160104792 ) ) ;
#36920=CARTESIAN_POINT ( 'NONE',  ( 0.2867679344610366554, -0.2867679344610365999, -0.8825652475403695796 ) ) ;
#36931=CARTESIAN_POINT ( 'NONE',  ( 0.3917322834645670104, -0.1049643490035303411, -1.048556430446194287 ) ) ;
#36933=ORIENTED_EDGE ( 'NONE', *, *, #49705, .F. ) ;
#36934=CARTESIAN_POINT ( 'NONE',  ( 0.3949938075777409963, 2.418639510665530435E-17, -1.377952755905511584 ) ) ;
#36939=CARTESIAN_POINT ( 'NONE',  ( 0.3460692066303959757, -0.1998031496062991907, 0.05249343832020996609 ) ) ;
#36947=CARTESIAN_POINT ( 'NONE',  ( -0.3917322834645671215, 0.1049643490035301469, 0.04002624671916000382 ) ) ;
#36953=CARTESIAN_POINT ( 'NONE',  ( 0.3460692066303959202, 0.1998031496062993295, -2.178477690288713742 ) ) ;
#36956=CARTESIAN_POINT ( 'NONE',  ( 4.893765752498283308E-17, -0.3996062992125985480, -1.730314960629921517 ) ) ;
#36960=CARTESIAN_POINT ( 'NONE',  ( -0.4724409448818898682, -8.678599364036362592E-17, -0.3543307086614173040 ) ) ;
#36962=CARTESIAN_POINT ( 'NONE',  ( -0.1958661417322834220, -0.3392501089628018884, -0.05774278215223092176 ) ) ;
#36968=CARTESIAN_POINT ( 'NONE',  ( 0.1265901696524990294, -0.4724409448818896462, -2.209317585301837195 ) ) ;
#36970=CARTESIAN_POINT ( 'NONE',  ( -0.3949938075777409963, -7.255918531996591613E-17, -2.320866141732283339 ) ) ;
#36992=CARTESIAN_POINT ( 'NONE',  ( -0.2925321140481932369, 0.2925321140481931259, -0.5688976377952755792 ) ) ;
#36993=CARTESIAN_POINT ( 'NONE',  ( -0.1049643490035302024, -0.3917322834645671215, -2.204068241469816503 ) ) ;
#37010=CARTESIAN_POINT ( 'NONE',  ( -0.1958661417322834220, -0.3392501089628018884, -1.567585301837270295 ) ) ;
#37011=CARTESIAN_POINT ( 'NONE',  ( 0.1504864506494466569, 0.3622863298689281142, -1.220472440944881054 ) ) ;
#37015=CARTESIAN_POINT ( 'NONE',  ( -0.2925321140481932369, 0.2925321140481930704, -2.458661417322834719 ) ) ;
#37017=CARTESIAN_POINT ( 'NONE',  ( 0.2925321140481932369, -0.2925321140481932369, -1.043307086614173151 ) ) ;
#37020=CARTESIAN_POINT ( 'NONE',  ( -0.3917322834645669549, -0.1049643490035306603, -2.715223097112861250 ) ) ;
#37032=CARTESIAN_POINT ( 'NONE',  ( 0.1049643490035303689, 0.3917322834645670104, -2.755249343832020248 ) ) ;
#37035=CARTESIAN_POINT ( 'NONE',  ( -0.2891555358219911054, 0.2891555358219909388, -0.3346456692913387099 ) ) ;
#37037=VERTEX_POINT ( 'NONE', #64602 ) ;
#37039=CARTESIAN_POINT ( 'NONE',  ( 0.3458507752293908943, 0.3458507752293908943, -0.1377952755905511861 ) ) ;
#37043=CARTESIAN_POINT ( 'NONE',  ( -0.1958661417322833942, -0.3392501089628018884, -1.322197793472127625 ) ) ;
#37045=CARTESIAN_POINT ( 'NONE',  ( 0.3392501089628018884, -0.1958661417322834220, -2.551837270341207109 ) ) ;
#37050=CARTESIAN_POINT ( 'NONE',  ( 0.1998031496062992740, 0.3460692066303959757, -0.9317585301837270073 ) ) ;
#37052=CARTESIAN_POINT ( 'NONE',  ( -0.3460692066303957537, -0.1998031496062994405, -0.4442257217847768724 ) ) ;
#37054=CARTESIAN_POINT ( 'NONE',  ( -0.3460692066303958092, -0.1998031496062994683, -2.257217847769029007 ) ) ;
#37055=CARTESIAN_POINT ( 'NONE',  ( -0.2867679344610364334, -0.2867679344610367109, -1.718503937007874072 ) ) ;
#37059=CARTESIAN_POINT ( 'NONE',  ( -0.4091458600556402980, -0.2362204724409451284, -1.231627296587926468 ) ) ;
#37062=CARTESIAN_POINT ( 'NONE',  ( 0.1974969037888706092, -0.3420746716998660508, -0.9560367454068241511 ) ) ;
#37074=CARTESIAN_POINT ( 'NONE',  ( -0.2925321140481932369, 0.2925321140481931259, -1.828740157480315265 ) ) ;
#37076=ADVANCED_FACE ( 'NONE', ( #6525 ), #1060, .T. ) ;
#37078=FACE_OUTER_BOUND ( 'NONE', #70170, .T. ) ;
#37090=CARTESIAN_POINT ( 'NONE',  ( -0.3917322834645671215, 0.1049643490035301469, -0.9048556430446195176 ) ) ;
#37105=( BOUNDED_CURVE ( )  B_SPLINE_CURVE ( 2, ( #80188, #27146, #27982, #79769, #53642, #79350, #52810, #21669, #3148, #15370, #8220, #15793, #67541 ),
 .UNSPECIFIED., .F., .F. ) 
 B_SPLINE_CURVE_WITH_KNOTS ( ( 3, 2, 2, 2, 2, 2, 3 ),
 ( 0.1125000000000000028, 0.1166666666666666685, 0.1208333333333333343, 0.1250000000000000000, 0.1291666666666666796, 0.1333333333333333315, 0.1375000000000000111 ),
 .UNSPECIFIED. ) 
 CURVE ( )  GEOMETRIC_REPRESENTATION_ITEM ( )  RATIONAL_B_SPLINE_CURVE ( ( 1.000000000000000000, 0.9659258262890683122, 1.000000000000000000, 0.9659258262890683122, 1.000000000000000000, 0.9659258262890683122, 1.000000000000000000, 0.9659258262890683122, 1.000000000000000000, 0.9659258262890683122, 1.000000000000000000, 0.9659258262890683122, 1.000000000000000000 ) ) 
 REPRESENTATION_ITEM ( '' )  );
#37110=CARTESIAN_POINT ( 'NONE',  ( -0.3598931997249494308, -0.1601112597069882237, -1.931802261947322519 ) ) ;
#37114=CARTESIAN_POINT ( 'NONE',  ( 0.4091458600556404646, -0.2362204724409448231, -0.4199475065616797842 ) ) ;
#37115=CARTESIAN_POINT ( 'NONE',  ( 0.3949938075777411073, -0.1058382717557499464, -2.631233595800525293 ) ) ;
#37118=CARTESIAN_POINT ( 'NONE',  ( 0.1049643490035304938, -0.3917322834645669549, -1.179790026246718915 ) ) ;
#37120=CARTESIAN_POINT ( 'NONE',  ( -0.1265901696524993347, 0.4724409448818895907, -2.526246719160104792 ) ) ;
#37126=CARTESIAN_POINT ( 'NONE',  ( 0.2867679344610365999, -0.2867679344610365999, -0.8083796343493945269 ) ) ;
#37134=CARTESIAN_POINT ( 'NONE',  ( -0.1049643490035302301, -0.3917322834645671770, -1.958680733104674276 ) ) ;
#37140=CARTESIAN_POINT ( 'NONE',  ( -0.1049643490035307020, 0.3917322834645669549, -1.193569553805774452 ) ) ;
#37150=CARTESIAN_POINT ( 'NONE',  ( 0.1958661417322836440, -0.3392501089628017219, -2.918635170603674389 ) ) ;
#37160=CARTESIAN_POINT ( 'NONE',  ( -0.3917322834645670104, -7.196005306013484475E-17, -1.068897637795275690 ) ) ;
#37161=CARTESIAN_POINT ( 'NONE',  ( -1.157146581871515012E-16, 0.4724409448818898682, 0.08070866141732283006 ) ) ;
#37163=CARTESIAN_POINT ( 'NONE',  ( 0.1998031496062994128, -0.3460692066303957537, -2.845800524934383624 ) ) ;
#37172=CARTESIAN_POINT ( 'NONE',  ( -0.1070741851644051862, -0.3996062992125986590, -0.4639107611548556331 ) ) ;
#37174=CARTESIAN_POINT ( 'NONE',  ( -0.1958661417322834220, -0.3392501089628018884, -0.3727034120734908362 ) ) ;
#37176=AXIS2_PLACEMENT_3D ( 'NONE', #71528, #52979, #13875 ) ;
#37190=CARTESIAN_POINT ( 'NONE',  ( -0.2867679344610367109, 0.2867679344610365444, -0.9613054050206844003 ) ) ;
#37194=CARTESIAN_POINT ( 'NONE',  ( 0.3458507752293908943, 0.3458507752293908943, -1.946850393700787274 ) ) ;
#37215=CARTESIAN_POINT ( 'NONE',  ( 0.3996062992125986035, 2.446882876249141962E-17, -0.1181102362204724671 ) ) ;
#37216=CARTESIAN_POINT ( 'NONE',  ( 0.3460692066303958092, 0.1998031496062993018, -2.727690288713910949 ) ) ;
#37223=CARTESIAN_POINT ( 'NONE',  ( 0.2925321140481932369, 0.2925321140481932369, -2.185039370078739829 ) ) ;
#37224=CARTESIAN_POINT ( 'NONE',  ( 4.837279021331060870E-17, -0.3949938075777409963, -1.496062992125984037 ) ) ;
#37225=CARTESIAN_POINT ( 'NONE',  ( -0.1998031496062994683, 0.3460692066303958092, -2.847769028871391050 ) ) ;
#37226=CARTESIAN_POINT ( 'NONE',  ( -0.4091458600556405756, 0.2362204724409446288, -2.545931758530183497 ) ) ;
#37227=CARTESIAN_POINT ( 'NONE',  ( 0.3917322834645670104, -0.1049643490035303273, -0.5761154855643044748 ) ) ;
#37231=CARTESIAN_POINT ( 'NONE',  ( 0.1058382717557499880, 0.3949938075777409408, -2.589895013123359124 ) ) ;
#37237=CARTESIAN_POINT ( 'NONE',  ( 0.3460692066303959757, -0.1998031496062991907, -2.309711286089239035 ) ) ;
#37246=CARTESIAN_POINT ( 'NONE',  ( 0.3917322834645670104, -0.1049643490035303411, -0.03871391076115493490 ) ) ;
#37253=CARTESIAN_POINT ( 'NONE',  ( -0.3392501089628017219, -0.1958661417322836718, -0.4520997375328084655 ) ) ;
#37254=CARTESIAN_POINT ( 'NONE',  ( 0.1049643490035304938, -0.3917322834645669549, -1.494750656167978642 ) ) ;
#37255=CARTESIAN_POINT ( 'NONE',  ( 0.3392501089628018884, -0.1958661417322834220, -2.774278215223096922 ) ) ;
#37258=CARTESIAN_POINT ( 'NONE',  ( 4.837279021331060870E-17, -0.3949938075777409963, -2.913385826771653253 ) ) ;
#37262=CARTESIAN_POINT ( 'NONE',  ( -0.3996062992125986035, -0.1070741851644056997, -1.463254593175853158 ) ) ;
#37267=CARTESIAN_POINT ( 'NONE',  ( -0.3917322834645669549, -0.1049643490035306603, -0.4455380577427821565 ) ) ;
#37277=CARTESIAN_POINT ( 'NONE',  ( 0.4724409448818896462, 0.1265901696524990294, -2.014435695538057569 ) ) ;
#37280=AXIS2_PLACEMENT_3D ( 'NONE', #26518, #70717, #38723 ) ;
#37288=CARTESIAN_POINT ( 'NONE',  ( 0.3917322834645668994, -0.1049643490035303134, -0.3490620490475572768 ) ) ;
#37290=CARTESIAN_POINT ( 'NONE',  ( 0.3917322834645669549, 0.1049643490035304660, -0.8392388451443569819 ) ) ;
#37295=CARTESIAN_POINT ( 'NONE',  ( -0.1049643490035302024, -0.3917322834645671215, -2.741469816272964710 ) ) ;
#37297=ADVANCED_FACE ( 'NONE', ( #33026 ), #32194, .F. ) ;
#37299=CARTESIAN_POINT ( 'NONE',  ( 5.785732909357575061E-17, -0.4724409448818898682, -0.6279527559055118058 ) ) ;
#37311=CARTESIAN_POINT ( 'NONE',  ( -0.3996062992125984925, -0.1070741851644056858, -1.854986876640420057 ) ) ;
#37321=CARTESIAN_POINT ( 'NONE',  ( 0.3460692066303959202, -0.1998031496062991630, -0.6541994750656167090 ) ) ;
#37322=CARTESIAN_POINT ( 'NONE',  ( -9.787531504996567848E-17, 0.3996062992125986035, -1.102362204724409489 ) ) ;
#37323=CARTESIAN_POINT ( 'NONE',  ( -0.1058382717557497937, -0.3949938075777411628, -0.07217847769028878924 ) ) ;
#37328=CARTESIAN_POINT ( 'NONE',  ( 0.2891555358219910499, 0.2891555358219910499, -1.474409448818897683 ) ) ;
#37333=CARTESIAN_POINT ( 'NONE',  ( 0.4724409448818896462, 0.1265901696524990294, -1.384514435695537671 ) ) ;
#37348=CARTESIAN_POINT ( 'NONE',  ( 0.3392501089628018329, 0.1958661417322835607, -1.068241469816272771 ) ) ;
#37351=CARTESIAN_POINT ( 'NONE',  ( -0.1974969037888703871, -0.3420746716998661063, -1.640419947506561948 ) ) ;
#37356=CARTESIAN_POINT ( 'NONE',  ( -0.1070741851644051862, -0.3996062992125987146, -0.3871391076115485719 ) ) ;
#37364=CARTESIAN_POINT ( 'NONE',  ( -0.1958661417322834220, -0.3392501089628018884, 0.1646981627296586759 ) ) ;
#37370=VERTEX_POINT ( 'NONE', #29209 ) ;
#37371=CARTESIAN_POINT ( 'NONE',  ( -0.3996062992125986035, -0.1070741851644056997, -2.250656167979002920 ) ) ;
#37374=CARTESIAN_POINT ( 'NONE',  ( 0.1070741851644053388, 0.3996062992125986035, -1.487532808398950301 ) ) ;
#37378=CARTESIAN_POINT ( 'NONE',  ( 0.2362204724409449064, 0.4091458600556404646, -0.4593175853018372501 ) ) ;
#37380=CARTESIAN_POINT ( 'NONE',  ( -0.1049643490035302024, -0.3917322834645671215, -0.06430446194225715451 ) ) ;
#37386=CARTESIAN_POINT ( 'NONE',  ( 0.2362204724409449064, 0.4091458600556404646, -2.268372703412073310 ) ) ;
#37388=CARTESIAN_POINT ( 'NONE',  ( 0.3420746716998660508, 0.1974969037888705814, -2.255249343832021136 ) ) ;
#37410=CARTESIAN_POINT ( 'NONE',  ( 0.1998031496062992463, 0.3460692066303959202, -0.6935695538057742304 ) ) ;
#37411=CARTESIAN_POINT ( 'NONE',  ( -0.1958661417322836718, 0.3392501089628017219, -2.459973753280839670 ) ) ;
#37420=CARTESIAN_POINT ( 'NONE',  ( -0.4724409448818904789, -0.1265901696524977804, -0.6758530183727032847 ) ) ;
#37426=CARTESIAN_POINT ( 'NONE',  ( -9.594673741351313045E-17, 0.3917322834645670104, -2.131889763779527769 ) ) ;
#37431=CARTESIAN_POINT ( 'NONE',  ( -9.787531504996566615E-17, 0.3996062992125985480, -2.281496062992125928 ) ) ;
#37433=CARTESIAN_POINT ( 'NONE',  ( -9.787531504996567848E-17, 0.3996062992125986035, -1.102362204724409489 ) ) ;
#37435=CARTESIAN_POINT ( 'NONE',  ( -0.2867679344610365999, 0.2867679344610364889, -2.688976377952755570 ) ) ;
#37447=CARTESIAN_POINT ( 'NONE',  ( 0.1958661417322836440, -0.3392501089628017219, -2.853674540682414662 ) ) ;
#37450=CARTESIAN_POINT ( 'NONE',  ( 0.1058382717557499880, 0.3949938075777411073, -0.3083989501312336956 ) ) ;
#37451=ORIENTED_EDGE ( 'NONE', *, *, #60460, .T. ) ;
#37453=CARTESIAN_POINT ( 'NONE',  ( 0.1265901696524989184, 0.4724409448818898127, -0.1509186351706036655 ) ) ;
#37458=CARTESIAN_POINT ( 'NONE',  ( 0.2867679344610366554, 0.2867679344610366554, -1.709336901083676086 ) ) ;
#37460=CARTESIAN_POINT ( 'NONE',  ( -9.594673741351313045E-17, 0.3917322834645670104, -2.761811023622046779 ) ) ;
#37465=CARTESIAN_POINT ( 'NONE',  ( 0.1998031496062994405, -0.3460692066303958092, -1.036745406824147064 ) ) ;
#37467=CARTESIAN_POINT ( 'NONE',  ( 0.3996062992125984925, 0.1070741851644054637, -0.2014435695538057958 ) ) ;
#37469=CARTESIAN_POINT ( 'NONE',  ( 0.3460692066303959757, -0.1998031496062991907, -2.467191601049868677 ) ) ;
#37470=CARTESIAN_POINT ( 'NONE',  ( -0.3917322834645671215, 0.1049643490035301469, -1.692257217847769057 ) ) ;
#37474=CARTESIAN_POINT ( 'NONE',  ( -1.157146581871515012E-16, 0.4724409448818898682, -1.179133858267716661 ) ) ;
#37478=CARTESIAN_POINT ( 'NONE',  ( 0.3420746716998660508, 0.1974969037888705814, -1.152887139107611425 ) ) ;
#37482=CARTESIAN_POINT ( 'NONE',  ( 0.000000000000000000, 0.000000000000000000, -2.755905511811024056 ) ) ;
#37488=CARTESIAN_POINT ( 'NONE',  ( -0.3460692066303957537, -0.1998031496062994405, -1.861548556430446366 ) ) ;
#37502=CARTESIAN_POINT ( 'NONE',  ( -0.3917322834645670104, -7.196005306013484475E-17, -1.068897637795275690 ) ) ;
#37510=DIRECTION ( 'NONE',  ( 0.000000000000000000, 0.000000000000000000, 1.000000000000000000 ) ) ;
#37521=CARTESIAN_POINT ( 'NONE',  ( -0.3392501089628019995, 0.1958661417322832277, -2.223097112860892288 ) ) ;
#37524=CARTESIAN_POINT ( 'NONE',  ( -0.4091458600556402980, -0.2362204724409451284, -0.2099737532808398921 ) ) ;
#37525=CARTESIAN_POINT ( 'NONE',  ( 0.2891555358219910499, 0.2891555358219910499, -2.657480314960630530 ) ) ;
#37528=CARTESIAN_POINT ( 'NONE',  ( -0.1958661417322834220, -0.3392501089628018884, -1.317585301837270295 ) ) ;
#37530=CARTESIAN_POINT ( 'NONE',  ( 5.785732909357575061E-17, -0.4724409448818898682, -2.913385826771653697 ) ) ;
#37537=CARTESIAN_POINT ( 'NONE',  ( 0.3917322834645668994, 0.1049643490035304522, -0.5196657235882398140 ) ) ;
#37545=CARTESIAN_POINT ( 'NONE',  ( -0.3392501089628019995, 0.1958661417322831999, -1.912748974574490113 ) ) ;
#37553=CARTESIAN_POINT ( 'NONE',  ( -0.1958661417322836718, 0.3392501089628017219, -1.200131233595800540 ) ) ;
#37560=CARTESIAN_POINT ( 'NONE',  ( -0.1208384647389192101, 0.3726288332213502641, 1.112018681666451222E-17 ) ) ;
#37562=CARTESIAN_POINT ( 'NONE',  ( -0.3392501089628017219, -0.1958661417322836718, -2.564304461942256808 ) ) ;
#37569=CARTESIAN_POINT ( 'NONE',  ( 0.1049643490035304938, -0.3917322834645669549, -1.272309711286089273 ) ) ;
#37570=CARTESIAN_POINT ( 'NONE',  ( -0.3458507752293909498, 0.3458507752293907833, 0.06102362204724409017 ) ) ;
#37573=CARTESIAN_POINT ( 'NONE',  ( -0.1070741851644051862, -0.3996062992125986590, -2.826115485564304475 ) ) ;
#37582=CARTESIAN_POINT ( 'NONE',  ( -0.3996062992125985480, -7.340648628747423112E-17, -0.4311023622047244208 ) ) ;
#37584=CARTESIAN_POINT ( 'NONE',  ( 0.2867679344610365999, 0.2867679344610365999, -0.1299212598425196485 ) ) ;
#37598=CARTESIAN_POINT ( 'NONE',  ( 0.1049643490035304799, -0.3917322834645670104, -0.7119615729996870979 ) ) ;
#37600=( BOUNDED_CURVE ( )  B_SPLINE_CURVE ( 2, ( #38920, #78075, #51119, #33025, #76814, #45639, #19562, #32608, #71334, #1059, #31778, #45221, #46057 ),
 .UNSPECIFIED., .F., .F. ) 
 B_SPLINE_CURVE_WITH_KNOTS ( ( 3, 2, 2, 2, 2, 2, 3 ),
 ( 0.8875000000000000666, 0.8916666666666668295, 0.8958333333333334814, 0.9000000000000001332, 0.9041666666666667851, 0.9083333333333334370, 0.9125000000000000888 ),
 .UNSPECIFIED. ) 
 CURVE ( )  GEOMETRIC_REPRESENTATION_ITEM ( )  RATIONAL_B_SPLINE_CURVE ( ( 0.9999999999999991118, 0.9659258262890692004, 1.000000000000000000, 0.9659258262890683122, 1.000000000000000000, 0.9659258262890683122, 1.000000000000000000, 0.9659258262890683122, 1.000000000000000000, 0.9659258262890683122, 1.000000000000000000, 0.9659258262890674240, 1.000000000000000888 ) ) 
 REPRESENTATION_ITEM ( '' )  );
#37603=CARTESIAN_POINT ( 'NONE',  ( 0.4724409448818897572, -0.1265901696524988906, -2.393044619422572072 ) ) ;
#37622=CARTESIAN_POINT ( 'NONE',  ( 0.2925321140481932369, 0.2925321140481932369, -0.2952755905511811330 ) ) ;
#37623=CARTESIAN_POINT ( 'NONE',  ( -0.3996062992125985480, -7.340648628747423112E-17, -2.793307086614173151 ) ) ;
#37628=CARTESIAN_POINT ( 'NONE',  ( 4.893765752498283924E-17, -0.3996062992125986035, -2.283464566929133799 ) ) ;
#37629=CARTESIAN_POINT ( 'NONE',  ( 0.2891555358219910499, 0.2891555358219910499, -1.397637795275590733 ) ) ;
#37632=CARTESIAN_POINT ( 'NONE',  ( 0.2867679344610366554, -0.2867679344610365444, -0.5629921259842519676 ) ) ;
#37635=CARTESIAN_POINT ( 'NONE',  ( 0.3420746716998660508, -0.1974969037888704149, -2.543963254593176071 ) ) ;
#37639=CARTESIAN_POINT ( 'NONE',  ( 0.1265901696524989462, 0.4724409448818897572, -2.670603674540682260 ) ) ;
#37640=CARTESIAN_POINT ( 'NONE',  ( -9.787531504996567848E-17, 0.3996062992125986035, -2.362204724409448620 ) ) ;
#37646=CARTESIAN_POINT ( 'NONE',  ( 0.1958661417322836440, -0.3392501089628017219, -0.3339895013123360679 ) ) ;
#37653=CARTESIAN_POINT ( 'NONE',  ( 0.3917322834645669549, 0.1049643490035304660, -0.5242782152230972548 ) ) ;
#37654=CARTESIAN_POINT ( 'NONE',  ( 0.1958661417322836440, -0.3392501089628017219, -1.658792650918635259 ) ) ;
#37655=CARTESIAN_POINT ( 'NONE',  ( -0.2867679344610365999, 0.2867679344610364889, -2.688976377952755570 ) ) ;
#37658=CARTESIAN_POINT ( 'NONE',  ( 0.3996062992125986590, -0.1070741851644053111, -0.1115485564304461857 ) ) ;
#37659=ORIENTED_EDGE ( 'NONE', *, *, #59375, .F. ) ;
#37662=CARTESIAN_POINT ( 'NONE',  ( 0.3996062992125986035, 0.1070741851644054776, -1.541994750656167978 ) ) ;
#37667=CARTESIAN_POINT ( 'NONE',  ( -0.1958661417322834220, -0.3392501089628018884, -0.6227034120734910028 ) ) ;
#37679=CARTESIAN_POINT ( 'NONE',  ( -0.3458507752293909498, 0.3458507752293907833, -2.224409448818897239 ) ) ;
#37682=EDGE_CURVE ( 'NONE', #2500, #57445, #59731, .T. ) ;
#37690=CARTESIAN_POINT ( 'NONE',  ( 0.1958661417322834497, 0.3392501089628018329, -0.2243901330370585701 ) ) ;
#37692=CARTESIAN_POINT ( 'NONE',  ( 0.3392501089628018884, -0.1958661417322834220, -0.9770341207349081403 ) ) ;
#37697=CARTESIAN_POINT ( 'NONE',  ( 4.797336870675656522E-17, -0.3917322834645670104, -2.905511811023621771 ) ) ;
#37702=CARTESIAN_POINT ( 'NONE',  ( -0.4724409448818898682, -8.678599364036362592E-17, -1.375984251968503713 ) ) ;
#37709=DIRECTION ( 'NONE',  ( 1.000000000000000000, 0.000000000000000000, 0.000000000000000000 ) ) ;
#37714=CARTESIAN_POINT ( 'NONE',  ( 0.2925321140481932369, -0.2925321140481931814, -2.064960629921259283 ) ) ;
#37717=CARTESIAN_POINT ( 'NONE',  ( -0.1070741851644056997, 0.3996062992125984925, -1.343175853018372834 ) ) ;
#37721=LINE ( 'NONE', #63395, #41193 ) ;
#37723=CARTESIAN_POINT ( 'NONE',  ( 0.1998031496062994128, -0.3460692066303957537, -0.4835958005249343938 ) ) ;
#37724=CARTESIAN_POINT ( 'NONE',  ( 0.1998031496062992740, 0.3460692066303959757, -0.9317585301837270073 ) ) ;
#37725=CARTESIAN_POINT ( 'NONE',  ( 0.3420746716998660508, -0.1974969037888703871, -0.4199475065616798952 ) ) ;
#37732=CARTESIAN_POINT ( 'NONE',  ( 0.3949938075777409408, -0.1058382717557499186, -1.448162729658792669 ) ) ;
#37737=CARTESIAN_POINT ( 'NONE',  ( -1.157146581871515012E-16, 0.4724409448818898682, -1.417322834645669216 ) ) ;
#37738=CARTESIAN_POINT ( 'NONE',  ( -0.3460692066303960868, 0.1998031496062990242, -2.545931758530183497 ) ) ;
#37741=ORIENTED_EDGE ( 'NONE', *, *, #47486, .T. ) ;
#37752=CARTESIAN_POINT ( 'NONE',  ( -0.1049643490035307020, 0.3917322834645669549, -1.416010498687664043 ) ) ;
#37755=CARTESIAN_POINT ( 'NONE',  ( -9.674558042662121740E-17, 0.3949938075777409963, -1.574803149606299302 ) ) ;
#37760=CARTESIAN_POINT ( 'NONE',  ( -0.1998031496062991907, -0.3460692066303959757, -0.2230971128608923715 ) ) ;
#37767=CARTESIAN_POINT ( 'NONE',  ( -0.2867679344610364334, -0.2867679344610367109, 0.01377952755905502598 ) ) ;
#37772=ORIENTED_EDGE ( 'NONE', *, *, #19166, .T. ) ;
#37773=CARTESIAN_POINT ( 'NONE',  ( -0.3996062992125986035, -7.340648628747425578E-17, -2.086614173228346303 ) ) ;
#37776=CARTESIAN_POINT ( 'NONE',  ( 0.3996062992125984925, 0.1070741851644054637, -1.618766404199474929 ) ) ;
#37781=CARTESIAN_POINT ( 'NONE',  ( -0.4724409448818899238, 0.1265901696524986686, -0.8202099737532806412 ) ) ;
#37783=CARTESIAN_POINT ( 'NONE',  ( -0.3917322834645671215, 0.1049643490035301469, -0.02493438320209968861 ) ) ;
#37789=CARTESIAN_POINT ( 'NONE',  ( -0.1265901696524993347, 0.4724409448818895907, -2.603018372703412631 ) ) ;
#37791=CARTESIAN_POINT ( 'NONE',  ( 0.3949938075777409408, -0.1058382717557499186, -2.078083989501312345 ) ) ;
#37803=CARTESIAN_POINT ( 'NONE',  ( 0.2017716535433070613, 0.2017716535433070613, -0.3937007874015748254 ) ) ;
#37814=CARTESIAN_POINT ( 'NONE',  ( 0.3460692066303959202, -0.1998031496062991630, -0.8116797900262466836 ) ) ;
#37815=CARTESIAN_POINT ( 'NONE',  ( -0.3917322834645669549, -0.1049643490035306603, -2.177821522309711266 ) ) ;
#37826=CARTESIAN_POINT ( 'NONE',  ( -0.3392501089628019995, 0.1958661417322831999, -1.912748974574490113 ) ) ;
#37833=CARTESIAN_POINT ( 'NONE',  ( -0.3917322834645669549, -0.1049643490035306603, -2.020341207349081181 ) ) ;
#37837=CARTESIAN_POINT ( 'NONE',  ( -1.157146581871515012E-16, 0.4724409448818898682, -0.4724409448818898127 ) ) ;
#37840=CARTESIAN_POINT ( 'NONE',  ( 0.1070741851644053527, 0.3996062992125986590, -0.7808398950131233418 ) ) ;
#37842=CARTESIAN_POINT ( 'NONE',  ( -0.3392501089628017219, -0.1958661417322836718, -2.721784776902886893 ) ) ;
#37856=CARTESIAN_POINT ( 'NONE',  ( 0.1958661417322836440, -0.3392501089628017219, -0.08398950131233590133 ) ) ;
#37859=CARTESIAN_POINT ( 'NONE',  ( -0.3949938075777409963, -7.255918531996591613E-17, -0.03937007874015754222 ) ) ;
#37867=CARTESIAN_POINT ( 'NONE',  ( 0.1958661417322834775, 0.3392501089628018884, -1.873378895834332258 ) ) ;
#37869=CARTESIAN_POINT ( 'NONE',  ( 0.1958661417322836440, -0.3392501089628017219, -2.696194225721784576 ) ) ;
#37874=CARTESIAN_POINT ( 'NONE',  ( -0.3996062992125987146, 0.1070741851644051862, -0.6627296587926508886 ) ) ;
#37876=CARTESIAN_POINT ( 'NONE',  ( -0.2925321140481930149, -0.2925321140481933480, -0.2933070866141732069 ) ) ;
#37877=CARTESIAN_POINT ( 'NONE',  ( -0.1998031496062991630, -0.3460692066303959202, 0.01509186351706034469 ) ) ;
#37879=CARTESIAN_POINT ( 'NONE',  ( -0.3460692066303958092, -0.1998031496062994683, -2.887139107611548461 ) ) ;
#37880=CARTESIAN_POINT ( 'NONE',  ( -0.1958661417322836718, 0.3392501089628017219, -1.515091863517060489 ) ) ;
#37885=CARTESIAN_POINT ( 'NONE',  ( -0.4091458600556402980, -0.2362204724409451284, -1.704068241469816058 ) ) ;
#37888=CARTESIAN_POINT ( 'NONE',  ( 0.1058382717557499880, 0.3949938075777409408, -0.8576115485564304031 ) ) ;
#37897=CARTESIAN_POINT ( 'NONE',  ( 0.2925321140481932369, -0.2925321140481931814, -1.907480314960629642 ) ) ;
#37912=CARTESIAN_POINT ( 'NONE',  ( 0.2867679344610365999, 0.2867679344610365999, -1.009842519685039353 ) ) ;
#37932=CARTESIAN_POINT ( 'NONE',  ( 0.3917322834645670104, -0.1049643490035303273, -1.993438320209973913 ) ) ;
#37935=CARTESIAN_POINT ( 'NONE',  ( -0.4091458600556405756, 0.2362204724409446288, -0.1837270341207349056 ) ) ;
#37936=CARTESIAN_POINT ( 'NONE',  ( 0.1974969037888706369, -0.3420746716998659953, -2.769028871391075786 ) ) ;
#37937=ORIENTED_EDGE ( 'NONE', *, *, #45564, .F. ) ;
#37939=CARTESIAN_POINT ( 'NONE',  ( 0.2867679344610365999, 0.2867679344610365999, -1.547244094488189115 ) ) ;
#37941=CARTESIAN_POINT ( 'NONE',  ( -0.4724409448818895907, -0.1265901696524993070, -2.723097112860892288 ) ) ;
#37948=CARTESIAN_POINT ( 'NONE',  ( 0.1049643490035303689, 0.3917322834645668994, -0.5459124427483446063 ) ) ;
#37955=CARTESIAN_POINT ( 'NONE',  ( -0.3392501089628019995, 0.1958661417322831999, -2.070229289535120198 ) ) ;
#37961=AXIS2_PLACEMENT_3D ( 'NONE', #52472, #78180, #16698 ) ;
#37963=CARTESIAN_POINT ( 'NONE',  ( -0.3917322834645671215, 0.1049643490035301469, -1.377296587926508664 ) ) ;
#37968=CARTESIAN_POINT ( 'NONE',  ( 0.4724409448818898682, 2.892866454678787531E-17, -0.03740157480314962313 ) ) ;
#37973=CARTESIAN_POINT ( 'NONE',  ( -0.1958661417322834220, -0.3392501089628018884, -2.734908136482939511 ) ) ;
#37975=ORIENTED_EDGE ( 'NONE', *, *, #40988, .T. ) ;
#37980=CARTESIAN_POINT ( 'NONE',  ( -0.1958661417322836718, 0.3392501089628017219, -1.042650918635170676 ) ) ;
#37981=CARTESIAN_POINT ( 'NONE',  ( 0.1265901696524990294, -0.4724409448818896462, -0.3195538057742782212 ) ) ;
#37984=CARTESIAN_POINT ( 'NONE',  ( 0.3460692066303959202, -0.1998031496062991630, -2.858923884514435798 ) ) ;
#37993=CARTESIAN_POINT ( 'NONE',  ( 4.893765752498283308E-17, -0.3996062992125985480, -0.4704724409448819422 ) ) ;
#37995=CARTESIAN_POINT ( 'NONE',  ( 0.1958661417322836440, -0.3392501089628017219, -0.08398950131233591521 ) ) ;
#38009=CARTESIAN_POINT ( 'NONE',  ( 0.2867679344610366554, 0.2867679344610366554, -0.9219353262805269900 ) ) ;
#38015=CARTESIAN_POINT ( 'NONE',  ( 0.4091458600556404646, -0.2362204724409448231, -2.386482939632545985 ) ) ;
#38033=CARTESIAN_POINT ( 'NONE',  ( -0.1998031496062991907, -0.3460692066303959757, -0.2230971128608923992 ) ) ;
#38034=CARTESIAN_POINT ( 'NONE',  ( -0.3460692066303960313, 0.1998031496062989965, -2.465223097112860806 ) ) ;
#38039=CARTESIAN_POINT ( 'NONE',  ( 0.3996062992125986035, 2.446882876249141962E-17, -2.165354330708661568 ) ) ;
#38040=CARTESIAN_POINT ( 'NONE',  ( -0.3949938075777409963, -7.255918531996591613E-17, -1.456692913385826627 ) ) ;
#38041=CARTESIAN_POINT ( 'NONE',  ( -0.1070741851644056997, 0.3996062992125986035, -2.683727034120735322 ) ) ;
#38042=CARTESIAN_POINT ( 'NONE',  ( -0.4724409448818899238, 0.1265901696524986964, -2.552493438320209140 ) ) ;
#38043=CARTESIAN_POINT ( 'NONE',  ( 0.2867679344610366554, 0.2867679344610366554, -0.4448818897637794589 ) ) ;
#38046=CARTESIAN_POINT ( 'NONE',  ( 0.2891555358219910499, 0.2891555358219910499, -2.576771653543307838 ) ) ;
#38051=CARTESIAN_POINT ( 'NONE',  ( 0.3460692066303959202, 0.1998031496062993295, -2.335958005249343827 ) ) ;
#38057=CARTESIAN_POINT ( 'NONE',  ( -9.594673741351313045E-17, 0.3917322834645670104, -0.2421259842519686289 ) ) ;
#38066=CARTESIAN_POINT ( 'NONE',  ( -0.2867679344610364334, -0.2867679344610367109, -0.4586614173228347746 ) ) ;
#38067=CARTESIAN_POINT ( 'NONE',  ( 0.1049643490035303689, 0.3917322834645670104, -1.560367454068241511 ) ) ;
#38068=CARTESIAN_POINT ( 'NONE',  ( 0.3917322834645669549, 0.1049643490035304660, -2.793963254593175183 ) ) ;
#38070=CARTESIAN_POINT ( 'NONE',  ( 0.2891555358219910499, -0.2891555358219909944, -2.933070866141733291 ) ) ;
#38074=CARTESIAN_POINT ( 'NONE',  ( -0.1998031496062994683, 0.3460692066303958092, -1.430446194225721834 ) ) ;
#38079=CARTESIAN_POINT ( 'NONE',  ( -0.1958661417322836718, 0.3392501089628017219, -0.7276902887139108378 ) ) ;
#38089=CARTESIAN_POINT ( 'NONE',  ( -0.4724409448818898682, -8.678599364036362592E-17, -2.086614173228346303 ) ) ;
#38092=( BOUNDED_CURVE ( )  B_SPLINE_CURVE ( 2, ( #47915, #3315, #21431, #80356, #67711, #48743, #66891, #16788, #42425, #36123, #29394, #22669, #9632 ),
 .UNSPECIFIED., .F., .F. ) 
 B_SPLINE_CURVE_WITH_KNOTS ( ( 3, 2, 2, 2, 2, 2, 3 ),
 ( 0.2624999999999999556, 0.2666666666666666075, 0.2708333333333333148, 0.2750000000000000222, 0.2791666666666666741, 0.2833333333333333814, 0.2875000000000000333 ),
 .UNSPECIFIED. ) 
 CURVE ( )  GEOMETRIC_REPRESENTATION_ITEM ( )  RATIONAL_B_SPLINE_CURVE ( ( 1.000000000000000444, 0.9659258262890678681, 1.000000000000000000, 0.9659258262890683122, 1.000000000000000000, 0.9659258262890683122, 1.000000000000000000, 0.9659258262890683122, 1.000000000000000000, 0.9659258262890683122, 1.000000000000000000, 0.9659258262890678681, 1.000000000000000444 ) ) 
 REPRESENTATION_ITEM ( '' )  );
#38096=CARTESIAN_POINT ( 'NONE',  ( -0.4724409448818898682, -8.678599364036362592E-17, -2.244094488188976388 ) ) ;
#38100=CARTESIAN_POINT ( 'NONE',  ( 0.3392501089628018329, 0.1958661417322835052, -0.9986683482601557138 ) ) ;
#38102=CARTESIAN_POINT ( 'NONE',  ( 0.3917322834645670104, 2.398668435337828261E-17, -0.8326771653543307838 ) ) ;
#38107=CARTESIAN_POINT ( 'NONE',  ( -0.2867679344610364334, -0.2867679344610367109, -2.570866141732283339 ) ) ;
#38112=CARTESIAN_POINT ( 'NONE',  ( -0.4724409448818895907, -0.1265901696524993070, -1.067585301837270517 ) ) ;
#38125=CARTESIAN_POINT ( 'NONE',  ( 0.2925321140481932369, -0.2925321140481931814, -2.222440944881889813 ) ) ;
#38129=CARTESIAN_POINT ( 'NONE',  ( -9.787531504996566615E-17, 0.3996062992125985480, -1.179133858267716661 ) ) ;
#38135=CARTESIAN_POINT ( 'NONE',  ( 0.3996062992125984925, 0.1070741851644054499, -0.8313648293963252778 ) ) ;
#38136=CARTESIAN_POINT ( 'NONE',  ( 0.2925321140481932369, -0.2925321140481932369, -0.8858267716535430658 ) ) ;
#38138=CARTESIAN_POINT ( 'NONE',  ( 0.1974969037888704704, 0.3420746716998660508, -0.1443569553805774675 ) ) ;
#38144=CARTESIAN_POINT ( 'NONE',  ( -0.1265901696524986964, -0.4724409448818899238, -2.353674540682414662 ) ) ;
#38145=CARTESIAN_POINT ( 'NONE',  ( 4.837279021331061486E-17, -0.3949938075777409963, -1.257874015748031260 ) ) ;
#38150=CARTESIAN_POINT ( 'NONE',  ( -0.1265901696524993347, 0.4724409448818895907, -1.423884514435695525 ) ) ;
#38158=CARTESIAN_POINT ( 'NONE',  ( 0.1958661417322834497, 0.3392501089628018329, -2.114153912564617599 ) ) ;
#38164=CARTESIAN_POINT ( 'NONE',  ( -0.3917322834645669549, -0.1049643490035306603, -1.297900262467191590 ) ) ;
#38167=CARTESIAN_POINT ( 'NONE',  ( -9.674558042662121740E-17, 0.3949938075777409963, -1.889763779527559029 ) ) ;
#38172=CARTESIAN_POINT ( 'NONE',  ( -0.3996062992125986035, -7.340648628747425578E-17, -0.03937007874015749365 ) ) ;
#38179=CARTESIAN_POINT ( 'NONE',  ( -0.2867679344610364334, -0.2867679344610367109, 0.1712598425196849850 ) ) ;
#38185=EDGE_LOOP ( 'NONE', ( #38686, #11781 ) ) ;
#38186=CARTESIAN_POINT ( 'NONE',  ( -9.787531504996566615E-17, 0.3996062992125985480, -2.124015748031495843 ) ) ;
#38191=CARTESIAN_POINT ( 'NONE',  ( -1.157146581871515012E-16, 0.4724409448818898682, -0.7874015748031496509 ) ) ;
#38193=CARTESIAN_POINT ( 'NONE',  ( 0.3392501089628018884, -0.1958661417322834220, -0.09711286089238840846 ) ) ;
#38194=CARTESIAN_POINT ( 'NONE',  ( -0.3392501089628019995, 0.1958661417322832277, -2.158136482939632561 ) ) ;
#38198=CARTESIAN_POINT ( 'NONE',  ( -0.2362204724409451284, 0.4091458600556402425, -2.609580052493438274 ) ) ;
#38202=CARTESIAN_POINT ( 'NONE',  ( 0.1058382717557500852, -0.3949938075777408852, -2.366797900262467280 ) ) ;
#38209=CARTESIAN_POINT ( 'NONE',  ( -0.2867679344610365999, 0.2867679344610364889, -1.429133858267716661 ) ) ;
#38212=CARTESIAN_POINT ( 'NONE',  ( -0.4724409448818895907, -0.1265901696524993070, 0.1922572178477690297 ) ) ;
#38224=CARTESIAN_POINT ( 'NONE',  ( 0.1070741851644053388, 0.3996062992125986035, -1.330052493438320216 ) ) ;
#38225=CARTESIAN_POINT ( 'NONE',  ( -0.1049643490035307020, 0.3917322834645669549, -2.295931758530183497 ) ) ;
#38235=CARTESIAN_POINT ( 'NONE',  ( 4.797336870675656522E-17, -0.3917322834645670659, -2.280203042815959869 ) ) ;
#38239=EDGE_CURVE ( 'NONE', #23562, #64782, #30721, .T. ) ;
#38243=CARTESIAN_POINT ( 'NONE',  ( 0.3392501089628018329, 0.1958661417322835607, -2.105643044619422533 ) ) ;
#38244=CARTESIAN_POINT ( 'NONE',  ( -0.3692639355350240127, 0.1324727617108177880, -1.220472440944881720 ) ) ;
#38248=CARTESIAN_POINT ( 'NONE',  ( -0.3460692066303960313, 0.1998031496062989965, -2.622703412073490892 ) ) ;
#38250=CARTESIAN_POINT ( 'NONE',  ( 0.1070741851644053527, 0.3996062992125986590, -1.253280839895013044 ) ) ;
#38253=CARTESIAN_POINT ( 'NONE',  ( -0.1958661417322836995, 0.3392501089628017219, -0.009861835466878533449 ) ) ;
#38254=EDGE_LOOP ( 'NONE', ( #52773, #63387, #26894, #72579, #28356, #61710, #28142 ) ) ;
#38266=CARTESIAN_POINT ( 'NONE',  ( 0.1958661417322834775, 0.3392501089628018884, -0.1364829396325459021 ) ) ;
#38269=CARTESIAN_POINT ( 'NONE',  ( 0.3949938075777409408, 0.1058382717557500574, -0.5971128608923886860 ) ) ;
#38272=CARTESIAN_POINT ( 'NONE',  ( -0.2362204724409451284, 0.4091458600556402425, -0.1706036745406823985 ) ) ;
#38275=EDGE_CURVE ( 'NONE', #82700, #62471, #57913, .T. ) ;
#38277=CARTESIAN_POINT ( 'NONE',  ( 0.2867679344610366554, 0.2867679344610366554, -1.866817216044307060 ) ) ;
#38279=PRODUCT_DEFINITION ( 'UNKNOWN', '', #53084, #77355 ) ;
#38280=CARTESIAN_POINT ( 'NONE',  ( 0.2867679344610365999, 0.2867679344610365999, -2.742125984251967630 ) ) ;
#38284=CARTESIAN_POINT ( 'NONE',  ( 0.3460692066303959757, -0.1998031496062991907, -0.8923884514435694859 ) ) ;
#38286=CARTESIAN_POINT ( 'NONE',  ( -0.1070741851644056997, 0.3996062992125984925, -0.2408136482939632061 ) ) ;
#38287=CARTESIAN_POINT ( 'NONE',  ( -0.2925321140481932369, 0.2925321140481931259, 0.06102362204724406242 ) ) ;
#38289=CARTESIAN_POINT ( 'NONE',  ( 0.1998031496062992740, 0.3460692066303959757, -2.821522309711286258 ) ) ;
#38290=CARTESIAN_POINT ( 'NONE',  ( -0.2867679344610364334, -0.2867679344610367109, -1.875984251968503935 ) ) ;
#38295=CARTESIAN_POINT ( 'NONE',  ( 0.4724409448818898682, 2.892866454678787531E-17, -1.297244094488188670 ) ) ;
#38299=CARTESIAN_POINT ( 'NONE',  ( 0.1058382717557500852, -0.3949938075777408852, -0.9494750656167980640 ) ) ;
#38310=CARTESIAN_POINT ( 'NONE',  ( 0.3460692066303959202, -0.1998031496062991630, -2.229002624671916344 ) ) ;
#38312=CARTESIAN_POINT ( 'NONE',  ( 0.3392501089628018329, 0.1958661417322835052, -1.628589608102675390 ) ) ;
#38327=CARTESIAN_POINT ( 'NONE',  ( 4.797336870675656522E-17, -0.3917322834645670104, -0.7933070866141732624 ) ) ;
#38336=CARTESIAN_POINT ( 'NONE',  ( 0.3458507752293908943, -0.3458507752293908943, -2.618110236220472675 ) ) ;
#38348=CARTESIAN_POINT ( 'NONE',  ( 0.3917322834645670104, 2.398668435337828261E-17, -2.157480314960630086 ) ) ;
#38351=CARTESIAN_POINT ( 'NONE',  ( 0.4091458600556403535, 0.2362204724409449896, -0.4461942257217847430 ) ) ;
#38352=CARTESIAN_POINT ( 'NONE',  ( 0.3460692066303959757, -0.1998031496062991907, -0.2624671916010499206 ) ) ;
#38355=CARTESIAN_POINT ( 'NONE',  ( -0.3917322834645669549, -0.1049643490035306603, -1.927821522309711044 ) ) ;
#38357=CARTESIAN_POINT ( 'NONE',  ( 0.3458507752293908943, -0.3458507752293908943, -2.933070866141732402 ) ) ;
#38364=CARTESIAN_POINT ( 'NONE',  ( -0.3392501089628019439, 0.1958661417322832554, -0.5787208416984759296 ) ) ;
#38371=CARTESIAN_POINT ( 'NONE',  ( -0.2867679344610367109, 0.2867679344610365444, -2.063667609745093667 ) ) ;
#38379=CARTESIAN_POINT ( 'NONE',  ( 4.797336870675656522E-17, -0.3917322834645670104, -1.265748031496062964 ) ) ;
#38383=CARTESIAN_POINT ( 'NONE',  ( -0.01987007963502784164, 0.3948464311378730440, -1.229201863956146261E-17 ) ) ;
#38387=CARTESIAN_POINT ( 'NONE',  ( 4.797336870675656522E-17, -0.3917322834645670104, -2.748031496062991685 ) ) ;
#38394=CARTESIAN_POINT ( 'NONE',  ( 0.1958661417322834775, 0.3392501089628018884, -1.331364829396325611 ) ) ;
#38395=CARTESIAN_POINT ( 'NONE',  ( 0.1265901696524989462, 0.4724409448818897572, -0.07020997375328083545 ) ) ;
#38399=CARTESIAN_POINT ( 'NONE',  ( -0.2925321140481930149, -0.2925321140481933480, -2.812992125984251857 ) ) ;
#38404=CARTESIAN_POINT ( 'NONE',  ( -0.2891555358219909388, -0.2891555358219912164, -0.1358267716535433156 ) ) ;
#38410=CARTESIAN_POINT ( 'NONE',  ( 0.1998031496062992463, 0.3460692066303959202, -1.008530183727034180 ) ) ;
#38412=CARTESIAN_POINT ( 'NONE',  ( 0.2867679344610365999, -0.2867679344610365444, -0.2480314960629920740 ) ) ;
#38426=CARTESIAN_POINT ( 'NONE',  ( -0.3392501089628019995, 0.1958661417322831999, -0.8103867698500807348 ) ) ;
#38430=CARTESIAN_POINT ( 'NONE',  ( -0.3458507752293909498, 0.3458507752293907833, -2.301181102362204633 ) ) ;
#38434=CYLINDRICAL_SURFACE ( 'NONE', #31230, 0.4724409448818898682 ) ;
#38447=CARTESIAN_POINT ( 'NONE',  ( -0.3996062992125986035, -7.340648628747425578E-17, -0.3543307086614173040 ) ) ;
#38448=CARTESIAN_POINT ( 'NONE',  ( 0.3996062992125986035, -0.1070741851644052972, -2.708005249343832688 ) ) ;
#38453=CARTESIAN_POINT ( 'NONE',  ( -0.3996062992125987146, 0.1070741851644051862, -2.237532808398950301 ) ) ;
#38454=CARTESIAN_POINT ( 'NONE',  ( -0.1974969037888703871, -0.3420746716998661063, -1.325459317585301777 ) ) ;
#38455=CARTESIAN_POINT ( 'NONE',  ( -0.2925321140481930704, -0.2925321140481933480, -2.893700787401574992 ) ) ;
#38457=CARTESIAN_POINT ( 'NONE',  ( -0.3917322834645671215, 0.1049643490035301469, -0.9698162729658791337 ) ) ;
#38460=CARTESIAN_POINT ( 'NONE',  ( 0.2891555358219910499, -0.2891555358219909944, -2.694881889763779625 ) ) ;
#38466=CARTESIAN_POINT ( 'NONE',  ( -0.1070741851644051862, -0.3996062992125987146, -1.961942257217847763 ) ) ;
#38467=CARTESIAN_POINT ( 'NONE',  ( 0.1049643490035304799, -0.3917322834645670104, -0.8694418879603171835 ) ) ;
#38470=VECTOR ( 'NONE', #76874, 39.37007874015748143 ) ;
#38475=CARTESIAN_POINT ( 'NONE',  ( -0.1958661417322836718, 0.3392501089628017219, -0.2552493438320210806 ) ) ;
#38483=CARTESIAN_POINT ( 'NONE',  ( -0.3392501089628019995, 0.1958661417322832277, -0.7408136482939633449 ) ) ;
#38484=CARTESIAN_POINT ( 'NONE',  ( -0.3917322834645669549, -0.1049643490035306603, -1.455380577427821676 ) ) ;
#38485=CARTESIAN_POINT ( 'NONE',  ( 0.1049643490035304938, -0.3917322834645669549, -2.754593175853017328 ) ) ;
#38487=CARTESIAN_POINT ( 'NONE',  ( 0.3996062992125986035, 0.1070741851644054776, 0.03280839895013121232 ) ) ;
#38492=CARTESIAN_POINT ( 'NONE',  ( 0.1998031496062992740, 0.3460692066303959757, -1.561679790026246684 ) ) ;
#38497=CARTESIAN_POINT ( 'NONE',  ( 0.3917322834645669549, 0.1049643490035304660, -0.6817585301837268963 ) ) ;
#38507=CARTESIAN_POINT ( 'NONE',  ( -0.4091458600556402980, -0.2362204724409451284, -1.942257217847769057 ) ) ;
#38517=CARTESIAN_POINT ( 'NONE',  ( -0.3917322834645670659, 0.1049643490035301607, -0.7427628364491322133 ) ) ;
#38519=CARTESIAN_POINT ( 'NONE',  ( -0.3392501089628019995, 0.1958661417322832277, -0.7408136482939633449 ) ) ;
#38524=CARTESIAN_POINT ( 'NONE',  ( 0.1049643490035303689, 0.3917322834645670104, -2.820209973753280419 ) ) ;
#38529=CARTESIAN_POINT ( 'NONE',  ( 0.2362204724409449064, 0.4091458600556404646, -1.166010498687663821 ) ) ;
#38542=CARTESIAN_POINT ( 'NONE',  ( 0.3460692066303959202, -0.1998031496062991630, -2.543963254593176071 ) ) ;
#38546=CARTESIAN_POINT ( 'NONE',  ( 0.3996062992125984925, 0.1070741851644054637, -1.303805774278215202 ) ) ;
#38552=CARTESIAN_POINT ( 'NONE',  ( -0.1070741851644057135, 0.3996062992125984925, -0.5557742782152230721 ) ) ;
#38553=CARTESIAN_POINT ( 'NONE',  ( 0.2925321140481932369, -0.2925321140481932369, -1.043307086614173151 ) ) ;
#38554=CARTESIAN_POINT ( 'NONE',  ( 0.3949938075777411073, -0.1058382717557499464, -0.1115485564304462551 ) ) ;
#38560=CARTESIAN_POINT ( 'NONE',  ( -0.3949938075777411073, 0.1058382717557497660, -1.526902887139107934 ) ) ;
#38565=CARTESIAN_POINT ( 'NONE',  ( 0.3458507752293908943, -0.3458507752293908943, -1.673228346456692828 ) ) ;
#38566=CARTESIAN_POINT ( 'NONE',  ( -0.3460692066303958092, -0.1998031496062994683, -2.729658792650918375 ) ) ;
#38573=CARTESIAN_POINT ( 'NONE',  ( -0.3917322834645670659, 0.1049643490035301607, -2.160085671094801540 ) ) ;
#38581=CARTESIAN_POINT ( 'NONE',  ( -0.3392501089628019995, 0.1958661417322832277, -1.435695538057742970 ) ) ;
#38584=CARTESIAN_POINT ( 'NONE',  ( 0.1974969037888706369, -0.3420746716998659953, -1.824146981627296382 ) ) ;
#38590=CARTESIAN_POINT ( 'NONE',  ( -9.787531504996567848E-17, 0.3996062992125986035, -8.919671568592925241E-18 ) ) ;
#38596=CARTESIAN_POINT ( 'NONE',  ( 0.3917322834645669549, 0.1049643490035304660, -0.5242782152230972548 ) ) ;
#38603=CARTESIAN_POINT ( 'NONE',  ( -0.3996062992125984925, -0.1070741851644056858, -2.012467191601049699 ) ) ;
#38608=CARTESIAN_POINT ( 'NONE',  ( 0.1265901696524990294, -0.4724409448818896462, -1.030183727034120533 ) ) ;
#38610=CARTESIAN_POINT ( 'NONE',  ( -0.2867679344610364334, -0.2867679344610367109, -0.2086614173228345248 ) ) ;
#38611=CARTESIAN_POINT ( 'NONE',  ( -0.4724409448818898682, 5.785732909357575061E-17, -2.755905511811024056 ) ) ;
#38615=CARTESIAN_POINT ( 'NONE',  ( 0.4724409448818898682, 2.892866454678787531E-17, -2.872047244094488416 ) ) ;
#38619=CARTESIAN_POINT ( 'NONE',  ( -0.1058382717557503072, 0.3949938075777408852, -2.603018372703412187 ) ) ;
#38627=CARTESIAN_POINT ( 'NONE',  ( -0.2867679344610364334, -0.2867679344610367109, -1.311023622047244430 ) ) ;
#38630=CARTESIAN_POINT ( 'NONE',  ( -0.2362204724409447953, -0.4091458600556404646, -0.1423884514435695414 ) ) ;
#38642=CARTESIAN_POINT ( 'NONE',  ( 0.3460692066303958092, 0.1998031496062993018, -0.9954068241469815614 ) ) ;
#38643=CARTESIAN_POINT ( 'NONE',  ( -0.3917322834645671215, 0.1049643490035301469, -2.479658792650918375 ) ) ;
#38655=CARTESIAN_POINT ( 'NONE',  ( -0.2867679344610365444, -0.2867679344610367664, -2.103037688485251522 ) ) ;
#38661=CARTESIAN_POINT ( 'NONE',  ( -0.3917322834645669549, -0.1049643490035306603, -2.177821522309711266 ) ) ;
#38668=CARTESIAN_POINT ( 'NONE',  ( 0.1998031496062994405, -0.3460692066303958092, -1.351706036745406792 ) ) ;
#38670=CARTESIAN_POINT ( 'NONE',  ( -0.3392501089628017219, -0.1958661417322836995, 0.1082484007535938902 ) ) ;
#38684=CARTESIAN_POINT ( 'NONE',  ( 0.1049643490035303689, 0.3917322834645670104, 0.01443569553805778768 ) ) ;
#38686=ORIENTED_EDGE ( 'NONE', *, *, #74544, .T. ) ;
#38687=CARTESIAN_POINT ( 'NONE',  ( -0.2891555358219911054, 0.2891555358219909388, -0.4921259842519685179 ) ) ;
#38690=FACE_OUTER_BOUND ( 'NONE', #30930, .T. ) ;
#38694=CARTESIAN_POINT ( 'NONE',  ( 0.3392501089628018884, -0.1958661417322833942, -1.834008817094174848 ) ) ;
#38700=CARTESIAN_POINT ( 'NONE',  ( 0.1070741851644053527, 0.3996062992125986590, -1.253280839895013044 ) ) ;
#38702=CARTESIAN_POINT ( 'NONE',  ( 0.1070741851644054776, -0.3996062992125984925, -0.6345144356955381149 ) ) ;
#38703=CARTESIAN_POINT ( 'NONE',  ( -0.3996062992125985480, -7.340648628747423112E-17, -0.1161417322834645965 ) ) ;
#38705=CARTESIAN_POINT ( 'NONE',  ( -0.2925321140481930704, -0.2925321140481933480, -2.736220472440944018 ) ) ;
#38706=CARTESIAN_POINT ( 'NONE',  ( -9.594673741351313045E-17, 0.3917322834645670104, -1.501968503937008093 ) ) ;
#38713=CARTESIAN_POINT ( 'NONE',  ( 0.2362204724409449064, 0.4091458600556404646, -1.480971128608923548 ) ) ;
#38716=CARTESIAN_POINT ( 'NONE',  ( 0.3949938075777408852, 0.1058382717557500435, -1.461286089238844843 ) ) ;
#38723=DIRECTION ( 'NONE',  ( 1.000000000000000000, 0.000000000000000000, 0.000000000000000000 ) ) ;
#38727=CARTESIAN_POINT ( 'NONE',  ( 0.3460692066303958092, 0.1998031496062993018, -2.255249343832021136 ) ) ;
#38729=EDGE_CURVE ( 'NONE', #39936, #57846, #5197, .T. ) ;
#38730=CARTESIAN_POINT ( 'NONE',  ( -0.3917322834645668994, -0.1049643490035306742, -1.858248400753593987 ) ) ;
#38738=CARTESIAN_POINT ( 'NONE',  ( 0.4091458600556403535, 0.2362204724409449896, -2.335958005249343827 ) ) ;
#38742=CARTESIAN_POINT ( 'NONE',  ( 0.3460692066303959202, -0.1998031496062991630, 0.1332020997375328031 ) ) ;
#38744=CARTESIAN_POINT ( 'NONE',  ( 0.3917322834645670104, -0.1049643490035303411, -1.141076115485564202 ) ) ;
#38763=CARTESIAN_POINT ( 'NONE',  ( 0.1958661417322834775, 0.3392501089628018884, -2.498687664041994605 ) ) ;
#38766=CARTESIAN_POINT ( 'NONE',  ( 0.1265901696524989462, 0.4724409448818897572, -0.7808398950131233418 ) ) ;
#38767=CARTESIAN_POINT ( 'NONE',  ( 0.1998031496062992740, 0.3460692066303959757, -0.1443569553805774397 ) ) ;
#38770=CARTESIAN_POINT ( 'NONE',  ( 0.3917322834645669549, 0.1049643490035304660, -1.691601049868766360 ) ) ;
#38774=CARTESIAN_POINT ( 'NONE',  ( -0.2362204724409451284, 0.4091458600556402425, -2.847769028871391050 ) ) ;
#38781=CARTESIAN_POINT ( 'NONE',  ( 0.2867679344610365999, 0.2867679344610365999, -1.005230028050182245 ) ) ;
#38788=CARTESIAN_POINT ( 'NONE',  ( -0.2867679344610365444, -0.2867679344610367664, -2.260518003445880719 ) ) ;
#38792=EDGE_CURVE ( 'NONE', #400, #25602, #16661, .T. ) ;
#38797=CARTESIAN_POINT ( 'NONE',  ( -0.2867679344610364334, -0.2867679344610367109, -1.718503937007874072 ) ) ;
#38813=CARTESIAN_POINT ( 'NONE',  ( -0.1265901696524993347, 0.4724409448818895907, -0.08333333333333335646 ) ) ;
#38815=CARTESIAN_POINT ( 'NONE',  ( 0.3996062992125984925, 0.1070741851644054637, -2.721128608923884418 ) ) ;
#38820=CARTESIAN_POINT ( 'NONE',  ( -0.3420746716998660508, -0.1974969037888706924, 0.02821522309711286050 ) ) ;
#38827=CARTESIAN_POINT ( 'NONE',  ( -0.1998031496062994405, 0.3460692066303957537, -0.7198162729658792447 ) ) ;
#38830=CARTESIAN_POINT ( 'NONE',  ( -0.1049643490035302024, -0.3917322834645671215, -0.6942257217847765949 ) ) ;
#38845=CARTESIAN_POINT ( 'NONE',  ( -0.4091458600556402980, -0.2362204724409451284, -2.648950131233595684 ) ) ;
#38861=CARTESIAN_POINT ( 'NONE',  ( -0.3460692066303958092, -0.1998031496062994683, -0.2099737532808399199 ) ) ;
#38869=CARTESIAN_POINT ( 'NONE',  ( 4.893765752498283924E-17, -0.3996062992125986035, -2.755905511811023612 ) ) ;
#38870=CARTESIAN_POINT ( 'NONE',  ( -0.2891555358219908833, -0.2891555358219912164, -1.791338582677165725 ) ) ;
#38871=CARTESIAN_POINT ( 'NONE',  ( 0.1958661417322836440, -0.3392501089628017219, -0.3989501312335957950 ) ) ;
#38873=CARTESIAN_POINT ( 'NONE',  ( -0.3392501089628019995, 0.1958661417322832277, -1.120734908136482799 ) ) ;
#38876=CARTESIAN_POINT ( 'NONE',  ( -0.3917322834645669549, -0.1049643490035306603, -1.140419947506561282 ) ) ;
#38878=CARTESIAN_POINT ( 'NONE',  ( -0.2867679344610366554, 0.2867679344610365444, 0.2152424128947000026 ) ) ;
#38882=CARTESIAN_POINT ( 'NONE',  ( -0.4091458600556402980, -0.2362204724409451284, -2.729658792650918375 ) ) ;
#38883=CARTESIAN_POINT ( 'NONE',  ( 0.2925321140481932369, -0.2925321140481932369, -2.618110236220472675 ) ) ;
#38884=CARTESIAN_POINT ( 'NONE',  ( -0.2867679344610367109, 0.2867679344610365444, -1.276266034941944127 ) ) ;
#38890=CARTESIAN_POINT ( 'NONE',  ( 0.1958661417322836440, -0.3392501089628017219, -0.01902887139107619849 ) ) ;
#38898=CARTESIAN_POINT ( 'NONE',  ( -0.2867679344610364334, -0.2867679344610367109, -0.6161417322834646937 ) ) ;
#38899=CARTESIAN_POINT ( 'NONE',  ( -0.3392501089628017219, -0.1958661417322836718, -2.091863517060367439 ) ) ;
#38900=CARTESIAN_POINT ( 'NONE',  ( -0.1049643490035307020, 0.3917322834645669549, -2.518372703412073754 ) ) ;
#38902=CARTESIAN_POINT ( 'NONE',  ( 0.1070741851644053527, 0.3996062992125986590, 0.006561679790026227546 ) ) ;
#38906=CARTESIAN_POINT ( 'NONE',  ( -0.1998031496062991907, -0.3460692066303959757, -1.640419947506561726 ) ) ;
#38910=CARTESIAN_POINT ( 'NONE',  ( 0.4091458600556404646, -0.2362204724409448231, -1.207349081364829324 ) ) ;
#38911=CARTESIAN_POINT ( 'NONE',  ( 0.3917322834645669549, 0.1049643490035304660, -0.8392388451443569819 ) ) ;
#38920=CARTESIAN_POINT ( 'NONE',  ( 0.4724409448818898682, 2.892866454678787531E-17, -2.637795275590551380 ) ) ;
#38930=CARTESIAN_POINT ( 'NONE',  ( 0.3917322834645668994, 0.1049643490035304522, -0.8346263535094994301 ) ) ;
#38938=CARTESIAN_POINT ( 'NONE',  ( -0.1049643490035307020, 0.3917322834645669549, -2.833333333333333037 ) ) ;
#38941=CARTESIAN_POINT ( 'NONE',  ( -0.4091458600556405756, 0.2362204724409446288, -1.047900262467191590 ) ) ;
#38953=CARTESIAN_POINT ( 'NONE',  ( -0.2925321140481930149, -0.2925321140481933480, -2.498031496062992574 ) ) ;
#38957=CARTESIAN_POINT ( 'NONE',  ( 0.3996062992125985480, 2.446882876249141654E-17, -1.297244094488189115 ) ) ;
#38963=CARTESIAN_POINT ( 'NONE',  ( 0.1070741851644054637, -0.3996062992125984925, -0.4770341207349080848 ) ) ;
#38965=CARTESIAN_POINT ( 'NONE',  ( -0.1998031496062994683, 0.3460692066303958092, -0.9580052493438320216 ) ) ;
#38966=CARTESIAN_POINT ( 'NONE',  ( -0.2891555358219908833, -0.2891555358219912164, -0.8464566929133858775 ) ) ;
#38972=CARTESIAN_POINT ( 'NONE',  ( 0.1974969037888704704, 0.3420746716998660508, -1.323490813648294129 ) ) ;
#38977=CARTESIAN_POINT ( 'NONE',  ( -0.3458507752293909498, 0.3458507752293907833, -1.594488188976378229 ) ) ;
#38978=CARTESIAN_POINT ( 'NONE',  ( 0.3996062992125986035, -0.1070741851644053111, -2.631233595800524405 ) ) ;
#38985=CARTESIAN_POINT ( 'NONE',  ( -0.1958661417322834497, -0.3392501089628018884, -2.035413755084302778 ) ) ;
#38986=CARTESIAN_POINT ( 'NONE',  ( 0.2925321140481932369, 0.2925321140481932369, -2.734251968503936148 ) ) ;
#38992=CARTESIAN_POINT ( 'NONE',  ( 0.1049643490035304938, -0.3917322834645669549, -1.337270341207349000 ) ) ;
#38995=CARTESIAN_POINT ( 'NONE',  ( -0.1974969037888703871, -0.3420746716998661063, -1.797900262467191590 ) ) ;
#39000=CARTESIAN_POINT ( 'NONE',  ( -0.3996062992125986035, -7.340648628747425578E-17, -0.3543307086614173040 ) ) ;
#39006=CARTESIAN_POINT ( 'NONE',  ( 0.4724409448818898682, 2.892866454678787531E-17, -0.9055118110236221041 ) ) ;
#39007=CARTESIAN_POINT ( 'NONE',  ( 0.3917322834645670104, 2.398668435337828261E-17, -0.2027559055118111353 ) ) ;
#39014=CARTESIAN_POINT ( 'NONE',  ( -0.1998031496062991630, -0.3460692066303959202, -2.189632545931758489 ) ) ;
#39019=CARTESIAN_POINT ( 'NONE',  ( -0.3458507752293906723, -0.3458507752293910609, -0.6889763779527556808 ) ) ;
#39021=CARTESIAN_POINT ( 'NONE',  ( 0.3392501089628018329, 0.1958661417322835607, -0.2808398950131232863 ) ) ;
#39022=CARTESIAN_POINT ( 'NONE',  ( -0.1958661417322834220, -0.3392501089628018884, -2.197506561679789971 ) ) ;
#39026=CARTESIAN_POINT ( 'NONE',  ( -0.4091458600556405756, 0.2362204724409446288, -2.780183727034120977 ) ) ;
#39031=CARTESIAN_POINT ( 'NONE',  ( -0.3420746716998662729, 0.1974969037888702206, -2.622703412073491336 ) ) ;
#39039=CARTESIAN_POINT ( 'NONE',  ( 0.2867679344610365999, -0.2867679344610365444, -1.507874015748031260 ) ) ;
#39043=CARTESIAN_POINT ( 'NONE',  ( -0.2362204724409447953, -0.4091458600556404646, 0.1725721784776902690 ) ) ;
#39056=CARTESIAN_POINT ( 'NONE',  ( 0.1998031496062992463, 0.3460692066303959202, -1.166010498687663821 ) ) ;
#39058=CARTESIAN_POINT ( 'NONE',  ( 4.797336870675656522E-17, -0.3917322834645670104, -2.525590551181102317 ) ) ;
#39067=CARTESIAN_POINT ( 'NONE',  ( 0.2362204724409451007, -0.4091458600556402980, -0.7217847769028871152 ) ) ;
#39069=CARTESIAN_POINT ( 'NONE',  ( 0.2867679344610366554, 0.2867679344610366554, -2.496738475886826070 ) ) ;
#39076=CARTESIAN_POINT ( 'NONE',  ( -0.1049643490035307020, 0.3917322834645669549, -1.980971128608924214 ) ) ;
#39083=CARTESIAN_POINT ( 'NONE',  ( 0.3460692066303959757, -0.1998031496062991907, -1.364829396325459188 ) ) ;
#39085=CARTESIAN_POINT ( 'NONE',  ( -0.1958661417322836995, 0.3392501089628017219, 0.1476184794937513700 ) ) ;
#39098=CARTESIAN_POINT ( 'NONE',  ( -0.3392501089628017219, -0.1958661417322836718, -0.3595800524934382736 ) ) ;
#39101=CARTESIAN_POINT ( 'NONE',  ( 0.3420746716998660508, -0.1974969037888703871, -0.5774278215223097588 ) ) ;
#39108=CARTESIAN_POINT ( 'NONE',  ( -0.3392501089628019995, 0.1958661417322831999, -1.597788344653229720 ) ) ;
#39115=CARTESIAN_POINT ( 'NONE',  ( -0.1998031496062991907, -0.3460692066303959757, -1.167979002624671914 ) ) ;
#39117=CARTESIAN_POINT ( 'NONE',  ( 4.893765752498283308E-17, -0.3996062992125985480, -0.6279527559055118058 ) ) ;
#39118=CARTESIAN_POINT ( 'NONE',  ( -0.2925321140481932369, 0.2925321140481931259, -0.2539370078740156855 ) ) ;
#39120=CARTESIAN_POINT ( 'NONE',  ( -0.2925321140481930704, -0.2925321140481933480, -2.578740157480315265 ) ) ;
#39121=CARTESIAN_POINT ( 'NONE',  ( 0.3392501089628018884, -0.1958661417322834220, -1.921916010498687877 ) ) ;
#39127=CARTESIAN_POINT ( 'NONE',  ( 0.1265901696524990294, -0.4724409448818896462, -1.579396325459317296 ) ) ;
#39130=CARTESIAN_POINT ( 'NONE',  ( 0.1058382717557499880, 0.3949938075777409408, -1.487532808398950523 ) ) ;
#39134=CARTESIAN_POINT ( 'NONE',  ( -0.4724409448818898682, 5.785732909357575061E-17, -2.755905511811024056 ) ) ;
#39140=CARTESIAN_POINT ( 'NONE',  ( -0.3460692066303960313, 0.1998031496062989965, -2.307742782152231165 ) ) ;
#39142=CARTESIAN_POINT ( 'NONE',  ( 0.3917322834645668994, 0.1049643490035304522, -2.251949188155168979 ) ) ;
#39153=CARTESIAN_POINT ( 'NONE',  ( 0.1070741851644053388, 0.3996062992125986035, 0.08727034120734905587 ) ) ;
#39155=CARTESIAN_POINT ( 'NONE',  ( -0.3917322834645671215, 0.1049643490035301469, -1.377296587926508664 ) ) ;
#39177=CARTESIAN_POINT ( 'NONE',  ( 0.3917322834645670104, 2.398668435337828261E-17, -2.472440944881889813 ) ) ;
#39180=CARTESIAN_POINT ( 'NONE',  ( -0.3458507752293909498, 0.3458507752293907833, -0.9645669291338579976 ) ) ;
#39181=CARTESIAN_POINT ( 'NONE',  ( -0.3460692066303960868, 0.1998031496062990242, -0.1837270341207349333 ) ) ;
#39182=ORIENTED_EDGE ( 'NONE', *, *, #33290, .F. ) ;
#39184=CARTESIAN_POINT ( 'NONE',  ( -0.1049643490035302024, -0.3917322834645671215, -1.954068241469816503 ) ) ;
#39196=CARTESIAN_POINT ( 'NONE',  ( 0.3392501089628018329, 0.1958661417322835052, -1.156148663220785799 ) ) ;
#39203=CARTESIAN_POINT ( 'NONE',  ( 0.1049643490035303967, 0.3917322834645670659, -2.352381520506248602 ) ) ;
#39211=CARTESIAN_POINT ( 'NONE',  ( -0.2867679344610365999, 0.2867679344610364889, -1.679133858267716661 ) ) ;
#39222=EDGE_CURVE ( 'NONE', #32899, #53885, #53822, .T. ) ;
#39228=CARTESIAN_POINT ( 'NONE',  ( -0.4724409448818895907, -0.1265901696524993070, -0.4376640419947506744 ) ) ;
#39231=CARTESIAN_POINT ( 'NONE',  ( 4.837279021331061486E-17, -0.3949938075777409963, -0.1555118110236220486 ) ) ;
#39236=CARTESIAN_POINT ( 'NONE',  ( 0.1058382717557499880, 0.3949938075777409408, -0.07020997375328083545 ) ) ;
#39245=CARTESIAN_POINT ( 'NONE',  ( -0.3996062992125986590, 0.1070741851644051723, -0.7395013123359580609 ) ) ;
#39247=CARTESIAN_POINT ( 'NONE',  ( 0.2867679344610365999, 0.2867679344610365999, -0.6023622047244093780 ) ) ;
#39262=CARTESIAN_POINT ( 'NONE',  ( 0.2362204724409449064, 0.4091458600556404646, -2.268372703412073310 ) ) ;
#39278=CARTESIAN_POINT ( 'NONE',  ( 0.1998031496062994405, -0.3460692066303958092, -0.5643044619422572516 ) ) ;
#39279=CARTESIAN_POINT ( 'NONE',  ( -0.2362204724409451284, 0.4091458600556402425, -1.192257217847769057 ) ) ;
#39283=CARTESIAN_POINT ( 'NONE',  ( -0.2925321140481932924, 0.2925321140481931814, -2.539370078740157410 ) ) ;
#39284=CARTESIAN_POINT ( 'NONE',  ( -0.1974969037888706647, 0.3420746716998658843, -1.745406824146981339 ) ) ;
#39285=CARTESIAN_POINT ( 'NONE',  ( 0.3917322834645670104, -0.1049643490035303411, -0.5761154855643042527 ) ) ;
#39287=CARTESIAN_POINT ( 'NONE',  ( 0.1958661417322836440, -0.3392501089628017219, -1.186351706036745446 ) ) ;
#39290=CARTESIAN_POINT ( 'NONE',  ( -0.3917322834645670104, -7.196005306013484475E-17, -0.9763779527559053317 ) ) ;
#39293=CARTESIAN_POINT ( 'NONE',  ( 0.3917322834645668994, -0.1049643490035303134, 0.1233788958343325359 ) ) ;
#39298=CARTESIAN_POINT ( 'NONE',  ( -0.4091458600556405756, 0.2362204724409446288, -0.1030183727034120617 ) ) ;
#39299=CARTESIAN_POINT ( 'NONE',  ( -0.2925321140481932924, 0.2925321140481931814, -2.381889763779527325 ) ) ;
#39300=CARTESIAN_POINT ( 'NONE',  ( 0.3392501089628018329, 0.1958661417322835607, -1.387814591372390272 ) ) ;
#39305=CARTESIAN_POINT ( 'NONE',  ( -0.3917322834645669549, -0.1049643490035306603, -0.6030183727034120755 ) ) ;
#39313=CARTESIAN_POINT ( 'NONE',  ( 0.1778467755342286460, -0.3496712940250776835, -1.929133858267715329 ) ) ;
#39314=CARTESIAN_POINT ( 'NONE',  ( 0.3917322834645670104, -0.1049643490035303411, -1.993438320209974135 ) ) ;
#39318=CARTESIAN_POINT ( 'NONE',  ( -0.3460692066303960868, 0.1998031496062990242, -0.02624671916010500733 ) ) ;
#39325=CARTESIAN_POINT ( 'NONE',  ( -0.1958661417322834220, -0.3392501089628018884, -0.7801837270341208663 ) ) ;
#39328=CARTESIAN_POINT ( 'NONE',  ( -0.3900885325446892815, -0.05060072268104446463, -1.929133858267718216 ) ) ;
#39345=CARTESIAN_POINT ( 'NONE',  ( -0.2867679344610364334, -0.2867679344610368219, -0.7690095556092370055 ) ) ;
#39349=CARTESIAN_POINT ( 'NONE',  ( -0.4091458600556405756, 0.2362204724409446288, -0.8136482939632546652 ) ) ;
#39356=CARTESIAN_POINT ( 'NONE',  ( 0.1958661417322836718, -0.3392501089628017219, -0.08860199294719349472 ) ) ;
#39359=CARTESIAN_POINT ( 'NONE',  ( -0.2362204724409447953, -0.4091458600556404646, -1.244750656167979086 ) ) ;
#39368=LINE ( 'NONE', #60396, #23294 ) ;
#39375=CARTESIAN_POINT ( 'NONE',  ( 0.1998031496062992463, 0.3460692066303959202, -2.268372703412073310 ) ) ;
#39379=CARTESIAN_POINT ( 'NONE',  ( 0.2925321140481932369, -0.2925321140481931814, -1.750000000000000222 ) ) ;
#39385=CARTESIAN_POINT ( 'NONE',  ( -0.1070741851644051862, -0.3996062992125986035, -1.093832020997375309 ) ) ;
#39386=CARTESIAN_POINT ( 'NONE',  ( -0.2925321140481932924, 0.2925321140481931814, -1.437007874015747921 ) ) ;
#39387=ADVANCED_FACE ( 'NONE', ( #18303 ), #69642, .T. ) ;
#39388=CARTESIAN_POINT ( 'NONE',  ( -0.1974969037888706647, 0.3420746716998658843, -0.6430446194225721834 ) ) ;
#39389=AXIS2_PLACEMENT_3D ( 'NONE', #25480, #63794, #18769 ) ;
#39395=CARTESIAN_POINT ( 'NONE',  ( -0.1058382717557497660, -0.3949938075777411073, -1.723753280839894986 ) ) ;
#39401=CARTESIAN_POINT ( 'NONE',  ( -0.4724409448818898682, -8.678599364036362592E-17, -2.086614173228346303 ) ) ;
#39409=CARTESIAN_POINT ( 'NONE',  ( -0.2867679344610364334, -0.2867679344610368219, -2.343812705215535974 ) ) ;
#39415=CARTESIAN_POINT ( 'NONE',  ( -0.3392501089628017219, -0.1958661417322836718, 0.1778215223097112108 ) ) ;
#39417=CARTESIAN_POINT ( 'NONE',  ( 0.1958661417322836440, -0.3392501089628017219, -1.816272965879265122 ) ) ;
#39420=CARTESIAN_POINT ( 'NONE',  ( -0.1058382717557497937, -0.3949938075777411628, -1.961942257217847763 ) ) ;
#39425=CARTESIAN_POINT ( 'NONE',  ( 0.3460692066303959202, 0.1998031496062993295, -0.6036745406824146620 ) ) ;
#39432=CARTESIAN_POINT ( 'NONE',  ( -0.1049643490035307020, 0.3917322834645669549, -0.2486876640419948270 ) ) ;
#39439=CARTESIAN_POINT ( 'NONE',  ( -0.1070741851644056997, 0.3996062992125984925, -2.130577427821522374 ) ) ;
#39444=CARTESIAN_POINT ( 'NONE',  ( 0.3458507752293908943, -0.3458507752293908943, -0.8858267716535430658 ) ) ;
#39446=CARTESIAN_POINT ( 'NONE',  ( -0.2867679344610365999, 0.2867679344610364889, -0.3267716535433070613 ) ) ;
#39447=CARTESIAN_POINT ( 'NONE',  ( -0.1958661417322834220, -0.3392501089628018884, -2.040026246719160330 ) ) ;
#39451=CARTESIAN_POINT ( 'NONE',  ( -0.3460692066303960313, 0.1998031496062989965, -0.2604986876640419946 ) ) ;
#39453=CARTESIAN_POINT ( 'NONE',  ( -0.1265901696524986964, -0.4724409448818899238, -1.093832020997375309 ) ) ;
#39457=CARTESIAN_POINT ( 'NONE',  ( 0.2891555358219910499, -0.2891555358219909944, -2.694881889763779625 ) ) ;
#39459=CARTESIAN_POINT ( 'NONE',  ( 0.3392501089628018884, -0.1958661417322834220, -0.1896325459317586282 ) ) ;
#39466=CARTESIAN_POINT ( 'NONE',  ( -9.594673741351313045E-17, 0.3917322834645670104, -1.881889763779527769 ) ) ;
#39469=CARTESIAN_POINT ( 'NONE',  ( 0.1265901696524990294, -0.4724409448818896462, -0.004593175853018378711 ) ) ;
#39483=CARTESIAN_POINT ( 'NONE',  ( 0.2925321140481932369, -0.2925321140481931814, -1.120078740157480324 ) ) ;
#39484=CARTESIAN_POINT ( 'NONE',  ( -0.1958661417322834220, -0.3392501089628018884, -2.669947506561679784 ) ) ;
#39493=CARTESIAN_POINT ( 'NONE',  ( 0.3996062992125986035, 0.1070741851644054776, 0.03280839895013121926 ) ) ;
#39494=CARTESIAN_POINT ( 'NONE',  ( 0.2867679344610366554, -0.2867679344610365999, -2.614848712107298745 ) ) ;
#39496=CARTESIAN_POINT ( 'NONE',  ( 0.02190130575838795945, -0.3959418824714272533, -2.713666019654406154E-16 ) ) ;
#39500=CARTESIAN_POINT ( 'NONE',  ( -0.3917322834645670104, -7.196005306013484475E-17, -2.328740157480315265 ) ) ;
#39505=CARTESIAN_POINT ( 'NONE',  ( -0.3996062992125985480, -0.1070741851644057135, -2.093175853018372834 ) ) ;
#39507=CARTESIAN_POINT ( 'NONE',  ( -0.2925321140481932924, 0.2925321140481931814, -1.437007874015747921 ) ) ;
#39509=CARTESIAN_POINT ( 'NONE',  ( 0.1958661417322836440, -0.3392501089628017219, -2.918635170603674389 ) ) ;
#39521=CARTESIAN_POINT ( 'NONE',  ( 4.797336870675656522E-17, -0.3917322834645670104, -0.07086614173228342195 ) ) ;
#39524=CARTESIAN_POINT ( 'NONE',  ( 0.1974969037888706369, -0.3420746716998659953, -0.4068241469816273326 ) ) ;
#39540=CARTESIAN_POINT ( 'NONE',  ( -0.3996062992125986035, -0.1070741851644056997, -1.463254593175853158 ) ) ;
#39542=CARTESIAN_POINT ( 'NONE',  ( 0.1070741851644053388, 0.3996062992125986035, -0.5426509186351704539 ) ) ;
#39543=CARTESIAN_POINT ( 'NONE',  ( 0.1998031496062994128, -0.3460692066303957537, -0.01115485564304463835 ) ) ;
#39545=CARTESIAN_POINT ( 'NONE',  ( 0.1070741851644054915, -0.3996062992125986035, -2.604986876640420057 ) ) ;
#39546=CARTESIAN_POINT ( 'NONE',  ( 4.797336870675656522E-17, -0.3917322834645670104, -2.210629921259842590 ) ) ;
#39552=CARTESIAN_POINT ( 'NONE',  ( -0.4091458600556405756, 0.2362204724409446288, -1.362860892388451539 ) ) ;
#39556=CARTESIAN_POINT ( 'NONE',  ( 0.3949938075777409408, -0.1058382717557499186, -1.290682414698162583 ) ) ;
#39559=LINE ( 'NONE', #39134, #47403 ) ;
#39566=CARTESIAN_POINT ( 'NONE',  ( -0.3996062992125984925, -0.1070741851644056858, -2.012467191601049699 ) ) ;
#39568=CARTESIAN_POINT ( 'NONE',  ( -0.1958661417322836440, 0.3392501089628016664, -2.140400631724722835 ) ) ;
#39581=CARTESIAN_POINT ( 'NONE',  ( -0.1998031496062994405, 0.3460692066303957537, 0.06758530183727033680 ) ) ;
#39583=CARTESIAN_POINT ( 'NONE',  ( -9.594673741351313045E-17, 0.3917322834645670104, -1.344488188976378007 ) ) ;
#39605=CARTESIAN_POINT ( 'NONE',  ( -9.594673741351313045E-17, 0.3917322834645670104, -2.354330708661417138 ) ) ;
#39609=CARTESIAN_POINT ( 'NONE',  ( -1.157146581871515012E-16, 0.4724409448818898682, -0.6299212598425196763 ) ) ;
#39610=CARTESIAN_POINT ( 'NONE',  ( -0.2925321140481932924, 0.2925321140481931814, -0.01968503937007875723 ) ) ;
#39613=CARTESIAN_POINT ( 'NONE',  ( 0.3392501089628018884, -0.1958661417322834220, -1.986876640419947604 ) ) ;
#39624=CARTESIAN_POINT ( 'NONE',  ( -0.1049643490035306742, 0.3917322834645668994, -1.031476747210287037 ) ) ;
#39630=CARTESIAN_POINT ( 'NONE',  ( 0.2867679344610366554, 0.2867679344610366554, -2.339258160926195984 ) ) ;
#39638=CARTESIAN_POINT ( 'NONE',  ( 0.2867679344610365999, 0.2867679344610365999, -1.797244094488188892 ) ) ;
#39654=CARTESIAN_POINT ( 'NONE',  ( 0.4091458600556403535, 0.2362204724409449896, -0.05052493438320210251 ) ) ;
#39658=CARTESIAN_POINT ( 'NONE',  ( -0.3420746716998662729, 0.1974969037888702206, -0.1030183727034120894 ) ) ;
#39663=CARTESIAN_POINT ( 'NONE',  ( -0.1974969037888706924, 0.3420746716998658843, 0.06758530183727033680 ) ) ;
#39670=CARTESIAN_POINT ( 'NONE',  ( -0.2925321140481932369, 0.2925321140481931259, -0.7263779527559056648 ) ) ;
#39672=CARTESIAN_POINT ( 'NONE',  ( 0.1958661417322834775, 0.3392501089628018884, -0.6089238845144356871 ) ) ;
#39674=CARTESIAN_POINT ( 'NONE',  ( 0.4091458600556404646, -0.2362204724409448231, -0.4967191601049869010 ) ) ;
#39687=CARTESIAN_POINT ( 'NONE',  ( 0.1998031496062992463, 0.3460692066303959202, 0.09383202099737530943 ) ) ;
#39691=( BOUNDED_CURVE ( )  B_SPLINE_CURVE ( 2, ( #53608, #22472, #27532, #16169, #53189, #48131, #21223 ),
 .UNSPECIFIED., .F., .F. ) 
 B_SPLINE_CURVE_WITH_KNOTS ( ( 3, 2, 2, 3 ),
 ( 0.07563788552403438725, 0.07916666666666666297, 0.08333333333333334259, 0.08750000000000000833 ),
 .UNSPECIFIED. ) 
 CURVE ( )  GEOMETRIC_REPRESENTATION_ITEM ( )  RATIONAL_B_SPLINE_CURVE ( ( 0.9911642120908014109, 0.9711423276059411025, 1.000000000000000000, 0.9659258262890683122, 1.000000000000000000, 0.9659258262890682012, 1.000000000000000222 ) ) 
 REPRESENTATION_ITEM ( '' )  );
#39695=CARTESIAN_POINT ( 'NONE',  ( -0.3458507752293909498, 0.3458507752293908388, -2.066929133858267598 ) ) ;
#39704=CARTESIAN_POINT ( 'NONE',  ( 0.1070741851644053666, 0.3996062992125986035, -0.9383202099737532054 ) ) ;
#39705=CARTESIAN_POINT ( 'NONE',  ( -0.4091458600556405756, 0.2362204724409446288, -1.205380577427821454 ) ) ;
#39710=CARTESIAN_POINT ( 'NONE',  ( 0.3460692066303959757, -0.1998031496062991907, -2.782152230971128848 ) ) ;
#39711=CARTESIAN_POINT ( 'NONE',  ( 0.1058382717557500713, -0.3949938075777409408, -2.132545931758530244 ) ) ;
#39712=CARTESIAN_POINT ( 'NONE',  ( -0.2867679344610364334, -0.2867679344610367109, -0.5236220472440944462 ) ) ;
#39713=CARTESIAN_POINT ( 'NONE',  ( 0.1958661417322836440, -0.3392501089628017219, -0.8713910761154854967 ) ) ;
#39715=CARTESIAN_POINT ( 'NONE',  ( -0.2867679344610365999, 0.2867679344610364889, -1.271653543307086798 ) ) ;
#39717=CARTESIAN_POINT ( 'NONE',  ( -0.1958661417322834497, -0.3392501089628018884, 0.01183033940388633805 ) ) ;
#39723=CARTESIAN_POINT ( 'NONE',  ( -0.3996062992125986035, -0.1070741851644056997, -2.408136482939632561 ) ) ;
#39724=CARTESIAN_POINT ( 'NONE',  ( -0.2867679344610367109, 0.2867679344610365444, -1.118785719981314264 ) ) ;
#39730=CARTESIAN_POINT ( 'NONE',  ( 0.3917322834645670104, 2.398668435337828261E-17, -0.3602362204724410266 ) ) ;
#39738=CARTESIAN_POINT ( 'NONE',  ( -0.4724409448818898682, -8.678599364036362592E-17, -0.5885826771653542844 ) ) ;
#39739=CARTESIAN_POINT ( 'NONE',  ( 4.797336870675656522E-17, -0.3917322834645670104, -2.118110236220472675 ) ) ;
#39741=CARTESIAN_POINT ( 'NONE',  ( 0.3996062992125986590, -0.1070741851644053111, -0.2690288713910760632 ) ) ;
#39748=CARTESIAN_POINT ( 'NONE',  ( -0.1049643490035302024, -0.3917322834645671215, -0.7867454068241470644 ) ) ;
#39768=CARTESIAN_POINT ( 'NONE',  ( -0.1049643490035301746, -0.3917322834645670659, -0.9396132301499194872 ) ) ;
#39771=CARTESIAN_POINT ( 'NONE',  ( -0.3392501089628017219, -0.1958661417322836718, -1.082020997375328086 ) ) ;
#39778=CARTESIAN_POINT ( 'NONE',  ( -0.3392501089628017219, -0.1958661417322836995, -0.2067122291676659340 ) ) ;
#39782=CARTESIAN_POINT ( 'NONE',  ( 0.1265901696524989462, 0.4724409448818897572, -1.645013123359579943 ) ) ;
#39797=CARTESIAN_POINT ( 'NONE',  ( 4.893765752498283308E-17, -0.3996062992125985480, -2.517716535433071279 ) ) ;
#39803=CARTESIAN_POINT ( 'NONE',  ( -9.787531504996566615E-17, 0.3996062992125985480, -1.966535433070866201 ) ) ;
#39811=CARTESIAN_POINT ( 'NONE',  ( -0.3460692066303960313, 0.1998031496062989965, -1.205380577427821454 ) ) ;
#39812=CARTESIAN_POINT ( 'NONE',  ( 0.2925321140481932369, -0.2925321140481932369, -1.515748031496062742 ) ) ;
#39813=CARTESIAN_POINT ( 'NONE',  ( 0.2891555358219910499, -0.2891555358219909944, -0.5708661417322835607 ) ) ;
#39819=CARTESIAN_POINT ( 'NONE',  ( 0.3949938075777409963, 2.418639510665530743E-17, -1.612204724409448842 ) ) ;
#39825=CARTESIAN_POINT ( 'NONE',  ( 5.785732909357575061E-17, -0.4724409448818898682, -2.125984251968504157 ) ) ;
#39828=ORIENTED_EDGE ( 'NONE', *, *, #62908, .T. ) ;
#39833=CARTESIAN_POINT ( 'NONE',  ( 0.3392501089628018329, -0.1958661417322834497, -2.547224778706350445 ) ) ;
#39839=CARTESIAN_POINT ( 'NONE',  ( -0.1049643490035306742, 0.3917322834645668994, -2.763760211777216202 ) ) ;
#39841=CARTESIAN_POINT ( 'NONE',  ( -0.3917322834645670104, -7.196005306013484475E-17, -1.763779527559055094 ) ) ;
#39844=CARTESIAN_POINT ( 'NONE',  ( -0.1058382717557503211, 0.3949938075777409408, -2.053805774278215868 ) ) ;
#39849=CARTESIAN_POINT ( 'NONE',  ( -0.1998031496062994683, 0.3460692066303958092, -0.6430446194225721834 ) ) ;
#39853=CARTESIAN_POINT ( 'NONE',  ( 0.03757601356357168076, -0.4709442531824368783, -4.620136098463503353E-16 ) ) ;
#39857=CARTESIAN_POINT ( 'NONE',  ( -0.2867679344610365999, 0.2867679344610364889, -0.4192913385826772532 ) ) ;
#39868=CARTESIAN_POINT ( 'NONE',  ( -0.4724409448818895907, -0.1265901696524993070, -1.305774278215223072 ) ) ;
#39871=CARTESIAN_POINT ( 'NONE',  ( 0.3917322834645669549, 0.1049643490035304660, -0.2742782152230970327 ) ) ;
#39872=CARTESIAN_POINT ( 'NONE',  ( 0.3917322834645670104, -0.1049643490035303273, -2.400918635170603110 ) ) ;
#39878=CARTESIAN_POINT ( 'NONE',  ( 0.1998031496062994128, -0.3460692066303957537, -0.01115485564304463835 ) ) ;
#39883=CARTESIAN_POINT ( 'NONE',  ( -0.3420746716998660508, -0.1974969037888706924, -2.806430446194226214 ) ) ;
#39890=CARTESIAN_POINT ( 'NONE',  ( -0.1049643490035307020, 0.3917322834645669549, -1.888451443569553412 ) ) ;
#39893=CARTESIAN_POINT ( 'NONE',  ( -0.4724409448818899238, 0.1265901696524986686, -0.1095800524934383152 ) ) ;
#39906=CARTESIAN_POINT ( 'NONE',  ( 0.2925321140481932369, 0.2925321140481932369, -1.316929133858267598 ) ) ;
#39908=CARTESIAN_POINT ( 'NONE',  ( -0.3917322834645671215, 0.1049643490035301469, -2.637139107611548461 ) ) ;
#39917=CARTESIAN_POINT ( 'NONE',  ( -0.1070741851644056997, 0.3996062992125986035, -0.1640419947506561726 ) ) ;
#39918=CARTESIAN_POINT ( 'NONE',  ( 0.1049643490035304799, -0.3917322834645670104, -2.444245037566615597 ) ) ;
#39925=CARTESIAN_POINT ( 'NONE',  ( -0.1958661417322834220, -0.3392501089628018884, -2.512467191601049699 ) ) ;
#39931=AXIS2_PLACEMENT_3D ( 'NONE', #6068, #82281, #45181 ) ;
#39935=CARTESIAN_POINT ( 'NONE',  ( 0.1070741851644054915, -0.3996062992125986035, -1.502624671916010346 ) ) ;
#39936=VERTEX_POINT ( 'NONE', #60970 ) ;
#39937=CARTESIAN_POINT ( 'NONE',  ( 0.1049643490035304799, -0.3917322834645670104, 0.07544000180346267792 ) ) ;
#39950=CARTESIAN_POINT ( 'NONE',  ( -9.594673741351313045E-17, 0.3917322834645670104, -0.6220472440944880832 ) ) ;
#39953=CARTESIAN_POINT ( 'NONE',  ( -0.1974969037888706647, 0.3420746716998658843, -0.8005249343832020470 ) ) ;
#39968=CARTESIAN_POINT ( 'NONE',  ( -0.1070741851644056997, 0.3996062992125986035, -1.108923884514435798 ) ) ;
#39970=CARTESIAN_POINT ( 'NONE',  ( -0.3996062992125984925, -0.1070741851644056858, -0.5951443569553805935 ) ) ;
#39971=CARTESIAN_POINT ( 'NONE',  ( -0.2925321140481930149, -0.2925321140481933480, -0.4507874015748031815 ) ) ;
#39973=CARTESIAN_POINT ( 'NONE',  ( -0.3458507752293909498, 0.3458507752293907833, -0.01968503937007874335 ) ) ;
#39974=CARTESIAN_POINT ( 'NONE',  ( -0.1049643490035302024, -0.3917322834645671215, -2.204068241469816503 ) ) ;
#39980=CARTESIAN_POINT ( 'NONE',  ( -0.4724409448818898682, -8.678599364036362592E-17, -2.005905511811023612 ) ) ;
#39983=CARTESIAN_POINT ( 'NONE',  ( 0.2891555358219910499, 0.2891555358219910499, -1.474409448818897683 ) ) ;
#39993=CARTESIAN_POINT ( 'NONE',  ( 0.3460692066303959202, -0.1998031496062991630, -2.071522309711286258 ) ) ;
#39996=CARTESIAN_POINT ( 'NONE',  ( 0.1049643490035303689, 0.3917322834645668994, -2.278195907315273327 ) ) ;
#40008=CARTESIAN_POINT ( 'NONE',  ( 0.3996062992125985480, 2.446882876249141654E-17, 0.1200787401574803098 ) ) ;
#40010=CARTESIAN_POINT ( 'NONE',  ( 0.3392501089628018884, -0.1958661417322834220, -1.606955380577427928 ) ) ;
#40031=CARTESIAN_POINT ( 'NONE',  ( 0.3392501089628018884, -0.1958661417322834220, -2.459317585301837195 ) ) ;
#40035=CARTESIAN_POINT ( 'NONE',  ( -0.3996062992125987146, 0.1070741851644051862, -0.03280839895013124702 ) ) ;
#40038=CARTESIAN_POINT ( 'NONE',  ( -0.3917322834645669549, -0.1049643490035306603, -1.612860892388451539 ) ) ;
#40045=DIRECTION ( 'NONE',  ( 0.000000000000000000, 0.000000000000000000, 1.000000000000000000 ) ) ;
#40049=CARTESIAN_POINT ( 'NONE',  ( 0.3917322834645669549, 2.398668435337827645E-17, -1.143025303640733181 ) ) ;
#40054=CARTESIAN_POINT ( 'NONE',  ( 0.3917322834645670659, -0.1049643490035303273, -2.313011441766091192 ) ) ;
#40062=CARTESIAN_POINT ( 'NONE',  ( 0.1958661417322834775, 0.3392501089628018884, -1.803805774278215202 ) ) ;
#40075=CARTESIAN_POINT ( 'NONE',  ( 5.785732909357575061E-17, -0.4724409448818898682, -0.6279527559055118058 ) ) ;
#40079=CARTESIAN_POINT ( 'NONE',  ( -0.1974969037888706924, 0.3420746716998658843, -0.08989501312335958227 ) ) ;
#40084=CARTESIAN_POINT ( 'NONE',  ( 0.2891555358219910499, -0.2891555358219909944, -0.01771653543307087977 ) ) ;
#40091=CARTESIAN_POINT ( 'NONE',  ( -0.2925321140481932369, 0.2925321140481931259, -1.041338582677165281 ) ) ;
#40093=CARTESIAN_POINT ( 'NONE',  ( -0.1958661417322834220, -0.3392501089628018884, -0.5301837270341206443 ) ) ;
#40107=CARTESIAN_POINT ( 'NONE',  ( -0.1265901696524986964, -0.4724409448818899238, -2.826115485564304475 ) ) ;
#40125=CARTESIAN_POINT ( 'NONE',  ( -0.1998031496062994683, 0.3460692066303958092, -0.6430446194225721834 ) ) ;
#40130=CARTESIAN_POINT ( 'NONE',  ( -0.3996062992125987146, 0.1070741851644051862, -2.552493438320210029 ) ) ;
#40131=CARTESIAN_POINT ( 'NONE',  ( -0.3949938075777409408, -0.1058382717557502933, -1.935695538057742748 ) ) ;
#40132=CARTESIAN_POINT ( 'NONE',  ( 0.1958661417322836440, -0.3392501089628017219, -0.5564304461942257696 ) ) ;
#40134=CARTESIAN_POINT ( 'NONE',  ( -0.3917322834645671215, 0.1049643490035301469, -1.127296587926509108 ) ) ;
#40136=CARTESIAN_POINT ( 'NONE',  ( -0.1049643490035307020, 0.3917322834645669549, -0.9435695538057740084 ) ) ;
#40138=CARTESIAN_POINT ( 'NONE',  ( 0.1958661417322834497, 0.3392501089628018329, -0.06690981807642862322 ) ) ;
#40144=CARTESIAN_POINT ( 'NONE',  ( -0.1070741851644051862, -0.3996062992125987146, -2.434383202099737353 ) ) ;
#40145=CARTESIAN_POINT ( 'NONE',  ( 0.1958661417322836718, -0.3392501089628017219, -1.348444512632232861 ) ) ;
#40151=CARTESIAN_POINT ( 'NONE',  ( 0.3392501089628018329, 0.1958661417322835607, -0.6883202099737534274 ) ) ;
#40159=CARTESIAN_POINT ( 'NONE',  ( 0.2643935821223346028, -0.2898214735613004467, -1.929133858267716439 ) ) ;
#40160=CARTESIAN_POINT ( 'NONE',  ( -0.3392501089628019995, 0.1958661417322832277, -1.908136482939632561 ) ) ;
#40162=CARTESIAN_POINT ( 'NONE',  ( 0.1998031496062992740, 0.3460692066303959757, -0.6167979002624671692 ) ) ;
#40168=CARTESIAN_POINT ( 'NONE',  ( 0.3458507752293908943, -0.3458507752293908943, -1.200787401574802793 ) ) ;
#40169=CARTESIAN_POINT ( 'NONE',  ( -0.3917322834645670104, -7.196005306013484475E-17, -1.226377952755905776 ) ) ;
#40183=VERTEX_POINT ( 'NONE', #55059 ) ;
#40184=CARTESIAN_POINT ( 'NONE',  ( 0.1265901696524990572, -0.4724409448818897017, -2.524278215223096478 ) ) ;
#40189=CARTESIAN_POINT ( 'NONE',  ( 4.797336870675655290E-17, -0.3917322834645669549, -1.103655224900575993 ) ) ;
#40199=CARTESIAN_POINT ( 'NONE',  ( -0.1958661417322833942, -0.3392501089628018884, 0.09512504117354141087 ) ) ;
#40202=CARTESIAN_POINT ( 'NONE',  ( 0.1265901696524990294, -0.4724409448818896462, -1.421916010498687877 ) ) ;
#40215=LINE ( 'NONE', #73033, #56875 ) ;
#40218=CARTESIAN_POINT ( 'NONE',  ( -0.3996062992125986590, 0.1070741851644051723, -2.629265091863517423 ) ) ;
#40223=CARTESIAN_POINT ( 'NONE',  ( 0.2925321140481932369, -0.2925321140481931814, -1.592519685039370358 ) ) ;
#40228=CARTESIAN_POINT ( 'NONE',  ( -0.1998031496062994405, 0.3460692066303957537, -0.8772965879265091083 ) ) ;
#40229=CARTESIAN_POINT ( 'NONE',  ( 0.1070741851644053527, 0.3996062992125986590, -1.410761154855643129 ) ) ;
#40230=CARTESIAN_POINT ( 'NONE',  ( -0.3949938075777409963, -7.255918531996591613E-17, -0.6692913385826770867 ) ) ;
#40235=CARTESIAN_POINT ( 'NONE',  ( -9.674558042662122972E-17, 0.3949938075777409963, -1.651574803149606474 ) ) ;
#40240=CARTESIAN_POINT ( 'NONE',  ( 0.4724409448818896462, 0.1265901696524990294, -2.171916010498687211 ) ) ;
#40242=EDGE_LOOP ( 'NONE', ( #64605, #66277, #36445, #16995 ) ) ;
#40247=CARTESIAN_POINT ( 'NONE',  ( 0.3917322834645669549, 2.398668435337827645E-17, -2.560348138286403064 ) ) ;
#40254=CARTESIAN_POINT ( 'NONE',  ( 0.3392501089628018884, -0.1958661417322834220, 0.1253280839895012100 ) ) ;
#40256=CARTESIAN_POINT ( 'NONE',  ( -0.3917322834645669549, -0.1049643490035306603, -1.927821522309711044 ) ) ;
#40259=CARTESIAN_POINT ( 'NONE',  ( -0.3949938075777409963, -7.255918531996591613E-17, -2.244094488188976388 ) ) ;
#40264=CARTESIAN_POINT ( 'NONE',  ( -0.1998031496062991907, -0.3460692066303959757, -0.6955380577427822120 ) ) ;
#40271=CARTESIAN_POINT ( 'NONE',  ( 0.2867679344610365999, 0.2867679344610365999, -0.6948818897637795144 ) ) ;
#40276=CARTESIAN_POINT ( 'NONE',  ( -9.594673741351313045E-17, 0.3917322834645670104, 0.1653543307086614844 ) ) ;
#40283=CARTESIAN_POINT ( 'NONE',  ( 0.4091458600556403535, 0.2362204724409449896, -1.233595800524934338 ) ) ;
#40286=CARTESIAN_POINT ( 'NONE',  ( 0.1049643490035303689, 0.3917322834645670104, -0.4580052493438320216 ) ) ;
#40287=CARTESIAN_POINT ( 'NONE',  ( -0.2867679344610366554, 0.2867679344610365444, -2.466535433070866201 ) ) ;
#40290=CARTESIAN_POINT ( 'NONE',  ( 0.1070741851644053388, 0.3996062992125986035, 0.08727034120734902811 ) ) ;
#40295=CARTESIAN_POINT ( 'NONE',  ( -0.2891555358219911054, 0.2891555358219909388, -2.458661417322835163 ) ) ;
#40303=CARTESIAN_POINT ( 'NONE',  ( -0.1049643490035307020, 0.3917322834645669549, -2.045931758530183497 ) ) ;
#40307=CARTESIAN_POINT ( 'NONE',  ( 0.4091458600556404646, -0.2362204724409448231, -0.3392388451443569819 ) ) ;
#40321=CARTESIAN_POINT ( 'NONE',  ( -0.3996062992125985480, -7.340648628747423112E-17, -1.533464566929133799 ) ) ;
#40322=( BOUNDED_CURVE ( )  B_SPLINE_CURVE ( 2, ( #47382, #8685, #2376, #2788, #48218, #74324, #28448, #54944, #16254, #73501, #15849, #3199, #28863 ),
 .UNSPECIFIED., .F., .F. ) 
 B_SPLINE_CURVE_WITH_KNOTS ( ( 3, 2, 2, 2, 2, 2, 3 ),
 ( 0.8125000000000000000, 0.8166666666666666519, 0.8208333333333333037, 0.8249999999999999556, 0.8291666666666667185, 0.8333333333333333703, 0.8375000000000000222 ),
 .UNSPECIFIED. ) 
 CURVE ( )  GEOMETRIC_REPRESENTATION_ITEM ( )  RATIONAL_B_SPLINE_CURVE ( ( 1.000000000000000000, 0.9659258262890683122, 1.000000000000000000, 0.9659258262890683122, 1.000000000000000000, 0.9659258262890683122, 1.000000000000000000, 0.9659258262890683122, 1.000000000000000000, 0.9659258262890683122, 1.000000000000000000, 0.9659258262890683122, 1.000000000000000000 ) ) 
 REPRESENTATION_ITEM ( '' )  );
#40323=CARTESIAN_POINT ( 'NONE',  ( -0.3392501089628017219, -0.1958661417322836718, -2.814304461942257252 ) ) ;
#40331=CARTESIAN_POINT ( 'NONE',  ( 0.1998031496062994405, -0.3460692066303958092, 0.06561679790026245240 ) ) ;
#40332=CARTESIAN_POINT ( 'NONE',  ( -0.1958661417322836995, 0.3392501089628017219, -2.687027189797587035 ) ) ;
#40338=CARTESIAN_POINT ( 'NONE',  ( 0.3917322834645669549, 0.1049643490035304660, -2.256561679790026531 ) ) ;
#40343=CARTESIAN_POINT ( 'NONE',  ( -0.2925321140481930704, -0.2925321140481933480, -2.106299212598425008 ) ) ;
#40345=CARTESIAN_POINT ( 'NONE',  ( 0.1998031496062992740, 0.3460692066303959757, -1.876640419947506411 ) ) ;
#40347=CARTESIAN_POINT ( 'NONE',  ( -0.1049643490035307158, 0.3917322834645670104, -0.3182607855981121059 ) ) ;
#40359=CARTESIAN_POINT ( 'NONE',  ( -0.3917322834645669549, -0.1049643490035306603, -0.5104986876640419391 ) ) ;
#40362=CARTESIAN_POINT ( 'NONE',  ( 0.3420746716998660508, -0.1974969037888703871, -1.207349081364829324 ) ) ;
#40376=CARTESIAN_POINT ( 'NONE',  ( -9.787531504996567848E-17, 0.3996062992125986035, -1.102362204724409489 ) ) ;
#40378=CARTESIAN_POINT ( 'NONE',  ( -0.3460692066303957537, -0.1998031496062994405, -0.7591863517060367661 ) ) ;
#40379=CARTESIAN_POINT ( 'NONE',  ( -0.3996062992125985480, -7.340648628747423112E-17, -0.5885826771653542844 ) ) ;
#40381=CARTESIAN_POINT ( 'NONE',  ( -0.2362204724409447953, -0.4091458600556404646, -0.06561679790026246628 ) ) ;
#40382=CARTESIAN_POINT ( 'NONE',  ( -0.2867679344610365999, 0.2867679344610364889, -1.994094488188976610 ) ) ;
#40388=CARTESIAN_POINT ( 'NONE',  ( -0.3458507752293906723, -0.3458507752293910609, -2.025590551181101873 ) ) ;
#40391=CARTESIAN_POINT ( 'NONE',  ( 0.3420746716998660508, -0.1974969037888704149, -1.599081364829396223 ) ) ;
#40403=CARTESIAN_POINT ( 'NONE',  ( 0.3996062992125986035, -0.1070741851644052972, -2.550524934383202158 ) ) ;
#40404=CARTESIAN_POINT ( 'NONE',  ( 4.797336870675655290E-17, -0.3917322834645669549, -2.048537114664355396 ) ) ;
#40417=CARTESIAN_POINT ( 'NONE',  ( 0.2925321140481932369, -0.2925321140481931814, 0.1397637795275590289 ) ) ;
#40419=CARTESIAN_POINT ( 'NONE',  ( 0.2867679344610365999, -0.2867679344610365444, -1.442913385826771755 ) ) ;
#40428=CARTESIAN_POINT ( 'NONE',  ( 0.3460692066303959202, -0.1998031496062991630, -0.9691601049868766582 ) ) ;
#40442=CARTESIAN_POINT ( 'NONE',  ( 0.1958661417322836440, -0.3392501089628017219, -2.446194225721784576 ) ) ;
#40445=CARTESIAN_POINT ( 'NONE',  ( 0.3996062992125986590, -0.1070741851644053111, -0.5839895013123358458 ) ) ;
#40446=ORIENTED_EDGE ( 'NONE', *, *, #21401, .F. ) ;
#40449=CARTESIAN_POINT ( 'NONE',  ( -0.3917322834645671215, 0.1049643490035301469, -2.387139107611548905 ) ) ;
#40461=CARTESIAN_POINT ( 'NONE',  ( 0.2867679344610365999, 0.2867679344610365999, -1.162710343010812108 ) ) ;
#40467=ORIENTED_EDGE ( 'NONE', *, *, #17226, .T. ) ;
#40468=CARTESIAN_POINT ( 'NONE',  ( -0.1049643490035307158, 0.3917322834645670104, -2.522985195046931306 ) ) ;
#40477=CARTESIAN_POINT ( 'NONE',  ( 0.1958661417322836440, -0.3392501089628017219, -1.751312335958005395 ) ) ;
#40484=LINE ( 'NONE', #66162, #70869 ) ;
#40486=CARTESIAN_POINT ( 'NONE',  ( 0.2925321140481932369, 0.2925321140481932369, -2.027559055118109743 ) ) ;
#40491=CARTESIAN_POINT ( 'NONE',  ( -0.2362204724409451284, 0.4091458600556402425, -0.7198162729658792447 ) ) ;
#40494=CARTESIAN_POINT ( 'NONE',  ( -0.1058382717557503072, 0.3949938075777408852, -0.08333333333333334259 ) ) ;
#40499=CARTESIAN_POINT ( 'NONE',  ( 0.1058382717557500852, -0.3949938075777408852, -0.6345144356955381149 ) ) ;
#40506=CARTESIAN_POINT ( 'NONE',  ( -0.1998031496062994405, 0.3460692066303957537, -1.192257217847769057 ) ) ;
#40508=CARTESIAN_POINT ( 'NONE',  ( -0.3917322834645670104, -7.196005306013484475E-17, -0.5039370078740157410 ) ) ;
#40524=CARTESIAN_POINT ( 'NONE',  ( -0.3996062992125985480, -7.340648628747423112E-17, 0.1988188976377952277 ) ) ;
#40540=CARTESIAN_POINT ( 'NONE',  ( 0.3996062992125986035, 2.446882876249141962E-17, -0.7480314960629921295 ) ) ;
#40544=CARTESIAN_POINT ( 'NONE',  ( -0.3460692066303960868, 0.1998031496062990242, -2.703412073490813583 ) ) ;
#40545=CARTESIAN_POINT ( 'NONE',  ( -0.2891555358219911054, 0.2891555358219909388, -2.224409448818897683 ) ) ;
#40546=CARTESIAN_POINT ( 'NONE',  ( -0.3917322834645670104, -7.196005306013484475E-17, -0.3464566929133857665 ) ) ;
#40549=CARTESIAN_POINT ( 'NONE',  ( -0.3392501089628017219, -0.1958661417322836718, -0.9895013123359579499 ) ) ;
#40551=CARTESIAN_POINT ( 'NONE',  ( 0.2891555358219910499, -0.2891555358219909944, -2.852362204724409267 ) ) ;
#40557=CARTESIAN_POINT ( 'NONE',  ( -0.2925321140481930704, -0.2925321140481933480, -2.578740157480315265 ) ) ;
#40558=CARTESIAN_POINT ( 'NONE',  ( 4.797336870675656522E-17, -0.3917322834645670659, -1.335321153052180243 ) ) ;
#40563=CARTESIAN_POINT ( 'NONE',  ( -0.3917322834645669549, -0.1049643490035306603, -0.4455380577427821565 ) ) ;
#40572=CARTESIAN_POINT ( 'NONE',  ( 0.2867679344610365999, -0.2867679344610365444, -1.822834645669291653 ) ) ;
#40574=CARTESIAN_POINT ( 'NONE',  ( -9.787531504996567848E-17, 0.3996062992125986035, -0.6299212598425196763 ) ) ;
#40580=CARTESIAN_POINT ( 'NONE',  ( 0.3974833285012838724, 0.03087045868620753170, -1.929133858267772617 ) ) ;
#40581=CARTESIAN_POINT ( 'NONE',  ( -0.3917322834645669549, -0.1049643490035306603, -1.075459317585301777 ) ) ;
#40591=CARTESIAN_POINT ( 'NONE',  ( -0.2925321140481932369, 0.2925321140481930704, -1.986220472440944906 ) ) ;
#40601=CARTESIAN_POINT ( 'NONE',  ( 0.3917322834645669549, 2.398668435337827645E-17, -1.143025303640733181 ) ) ;
#40604=CARTESIAN_POINT ( 'NONE',  ( -0.3917322834645671215, 0.1049643490035301469, -1.062335958005249381 ) ) ;
#40610=CARTESIAN_POINT ( 'NONE',  ( -0.2867679344610367109, 0.2867679344610365444, 0.1410567997037251442 ) ) ;
#40613=CARTESIAN_POINT ( 'NONE',  ( 0.4091458600556403535, 0.2362204724409449896, -1.467847769028871596 ) ) ;
#40628=VECTOR ( 'NONE', #42594, 39.37007874015748143 ) ;
#40630=CARTESIAN_POINT ( 'NONE',  ( -0.1998031496062994405, 0.3460692066303957537, -2.767060367454068359 ) ) ;
#40635=CARTESIAN_POINT ( 'NONE',  ( 0.3996062992125986035, -0.1070741851644052972, -1.605643044619422977 ) ) ;
#40640=CARTESIAN_POINT ( 'NONE',  ( 0.3460692066303958092, 0.1998031496062993018, -1.152887139107611425 ) ) ;
#40641=CARTESIAN_POINT ( 'NONE',  ( 4.893765752498283924E-17, -0.3996062992125986035, -1.496062992125984259 ) ) ;
#40642=CARTESIAN_POINT ( 'NONE',  ( 0.3949938075777409408, 0.1058382717557500574, -0.5971128608923886860 ) ) ;
#40643=CARTESIAN_POINT ( 'NONE',  ( 0.3392501089628018884, -0.1958661417322834220, -0.09711286089238840846 ) ) ;
#40647=CARTESIAN_POINT ( 'NONE',  ( 0.3420746716998660508, 0.1974969037888705814, -1.940288713910761187 ) ) ;
#40651=CARTESIAN_POINT ( 'NONE',  ( 0.1265901696524989462, 0.4724409448818897572, -2.198162729658792447 ) ) ;
#40652=CARTESIAN_POINT ( 'NONE',  ( 0.2432155562301146490, 0.3078094465263132573, -2.755905511811025388 ) ) ;
#40659=CARTESIAN_POINT ( 'NONE',  ( 0.1958661417322836162, -0.3392501089628018329, -2.534101419126297827 ) ) ;
#40666=CARTESIAN_POINT ( 'NONE',  ( 4.797336870675655290E-17, -0.3917322834645669549, -2.835938689467505380 ) ) ;
#40668=CARTESIAN_POINT ( 'NONE',  ( 0.1958661417322834775, 0.3392501089628018884, -1.868766404199474929 ) ) ;
#40671=CARTESIAN_POINT ( 'NONE',  ( 0.3420746716998659953, 0.1974969037888705536, -2.335958005249343827 ) ) ;
#40676=CARTESIAN_POINT ( 'NONE',  ( -0.2925321140481932924, 0.2925321140481931814, -0.8070866141732284671 ) ) ;
#40681=CARTESIAN_POINT ( 'NONE',  ( -0.3917322834645671215, 0.1049643490035301469, -0.1174540682414699083 ) ) ;
#40691=CARTESIAN_POINT ( 'NONE',  ( 0.4724409448818898682, 2.892866454678787531E-17, -1.139763779527559029 ) ) ;
#40692=CARTESIAN_POINT ( 'NONE',  ( 0.4724409448818896462, 0.1265901696524990294, -1.227034120734908029 ) ) ;
#40695=CARTESIAN_POINT ( 'NONE',  ( 4.797336870675656522E-17, -0.3917322834645670104, -0.8582677165354329896 ) ) ;
#40696=CARTESIAN_POINT ( 'NONE',  ( -0.1049643490035301885, -0.3917322834645671215, -2.361548556430446144 ) ) ;
#40699=CARTESIAN_POINT ( 'NONE',  ( -0.3996062992125985480, -7.340648628747423112E-17, 0.04133858267716532947 ) ) ;
#40704=CARTESIAN_POINT ( 'NONE',  ( -0.2867679344610366554, 0.2867679344610365444, 0.2152424128947000026 ) ) ;
#40711=CARTESIAN_POINT ( 'NONE',  ( 0.3917322834645670104, -0.1049643490035303411, -1.835958005249343827 ) ) ;
#40715=CARTESIAN_POINT ( 'NONE',  ( -0.1265901696524986964, -0.4724409448818899238, -0.4639107611548556331 ) ) ;
#40725=DIRECTION ( 'NONE',  ( 1.000000000000000000, 0.000000000000000000, 0.000000000000000000 ) ) ;
#40730=CARTESIAN_POINT ( 'NONE',  ( 0.1998031496062992463, 0.3460692066303959202, -1.480971128608923548 ) ) ;
#40737=CARTESIAN_POINT ( 'NONE',  ( 0.3996062992125985480, -0.1070741851644052972, -0.03083989501312337997 ) ) ;
#40739=CARTESIAN_POINT ( 'NONE',  ( 0.3460692066303959757, -0.1998031496062991907, -0.2624671916010498651 ) ) ;
#40741=CARTESIAN_POINT ( 'NONE',  ( -0.3917322834645670104, -0.1049643490035307020, -2.719835588747718802 ) ) ;
#40746=CARTESIAN_POINT ( 'NONE',  ( -0.3392501089628019995, 0.1958661417322832277, -2.473097112860892288 ) ) ;
#40751=CARTESIAN_POINT ( 'NONE',  ( -0.3996062992122574320, -0.1070741851649966020, -1.935695538057784493 ) ) ;
#40754=CARTESIAN_POINT ( 'NONE',  ( -0.1049643490035307158, 0.3917322834645670104, -0.4757411005587420805 ) ) ;
#40767=CARTESIAN_POINT ( 'NONE',  ( -0.3917322834645671215, 0.1049643490035301469, -0.8123359580052491591 ) ) ;
#40770=CARTESIAN_POINT ( 'NONE',  ( -9.674558042662121740E-17, 0.3949938075777409963, -0.9448818897637795144 ) ) ;
#40786=ORIENTED_EDGE ( 'NONE', *, *, #32000, .F. ) ;
#40787=CARTESIAN_POINT ( 'NONE',  ( 0.3460692066303959757, -0.1998031496062991907, -1.837270341207349000 ) ) ;
#40789=CARTESIAN_POINT ( 'NONE',  ( 0.3996062992125985480, 2.446882876249141654E-17, -0.9822834645669291653 ) ) ;
#40790=CARTESIAN_POINT ( 'NONE',  ( -9.787531504996566615E-17, 0.3996062992125985480, -0.5492125984251968740 ) ) ;
#40792=CARTESIAN_POINT ( 'NONE',  ( 0.2362204724409449064, 0.4091458600556404646, -0.1443569553805774397 ) ) ;
#40793=CARTESIAN_POINT ( 'NONE',  ( -0.3392501089628019995, 0.1958661417322832277, -2.315616797900262647 ) ) ;
#40799=CARTESIAN_POINT ( 'NONE',  ( 0.1265901696524989462, 0.4724409448818897572, -2.117454068241469756 ) ) ;
#40803=CARTESIAN_POINT ( 'NONE',  ( -0.3949938075777409963, -7.255918531996591613E-17, -2.005905511811023612 ) ) ;
#40813=CARTESIAN_POINT ( 'NONE',  ( 0.1070741851644053388, 0.3996062992125986035, -2.432414698162729039 ) ) ;
#40815=CARTESIAN_POINT ( 'NONE',  ( -0.1049643490035301746, -0.3917322834645670659, -2.041975434874328865 ) ) ;
#40824=CARTESIAN_POINT ( 'NONE',  ( 0.4724409448818898682, 2.892866454678787531E-17, -0.9055118110236221041 ) ) ;
#40828=CARTESIAN_POINT ( 'NONE',  ( 0.3460692066303958092, 0.1998031496062993018, -0.2080052493438320216 ) ) ;
#40831=CARTESIAN_POINT ( 'NONE',  ( 0.3917322834645670104, 2.398668435337828261E-17, -1.462598425196850460 ) ) ;
#40840=CARTESIAN_POINT ( 'NONE',  ( 0.2925321140481932369, 0.2925321140481932369, -1.159448818897637734 ) ) ;
#40846=CARTESIAN_POINT ( 'NONE',  ( 0.3972027188793966213, 0.005815251566292155977, -1.220472440942466319 ) ) ;
#40857=CARTESIAN_POINT ( 'NONE',  ( -9.787531504996567848E-17, 0.3996062992125986035, -0.4724409448818898127 ) ) ;
#40861=CARTESIAN_POINT ( 'NONE',  ( 0.1958661417322834775, 0.3392501089628018884, -2.341207349081364963 ) ) ;
#40869=CARTESIAN_POINT ( 'NONE',  ( 0.1265901696524990572, -0.4724409448818897017, -2.051837270341206665 ) ) ;
#40873=CARTESIAN_POINT ( 'NONE',  ( -0.3917322834645670659, 0.1049643490035301607, -1.372684096291651556 ) ) ;
#40879=CARTESIAN_POINT ( 'NONE',  ( -0.3917322834645670659, -7.196005306013484475E-17, -2.870754223918321912 ) ) ;
#40888=CARTESIAN_POINT ( 'NONE',  ( 0.3392501089628018884, -0.1958661417322834220, -2.236876640419947826 ) ) ;
#40896=CARTESIAN_POINT ( 'NONE',  ( -0.1070741851644056997, 0.3996062992125984925, 0.07414698162729659037 ) ) ;
#40898=CARTESIAN_POINT ( 'NONE',  ( 0.2925321140481932369, 0.2925321140481932369, -1.712598425196850460 ) ) ;
#40904=CARTESIAN_POINT ( 'NONE',  ( 0.4724409448818898682, 2.892866454678787531E-17, -0.8248031496062991907 ) ) ;
#40907=CARTESIAN_POINT ( 'NONE',  ( -0.3420746716998660508, -0.1974969037888706924, -0.2867454068241469534 ) ) ;
#40913=CARTESIAN_POINT ( 'NONE',  ( 4.837279021331061486E-17, -0.3949938075777409963, -0.3129921259842520231 ) ) ;
#40921=CARTESIAN_POINT ( 'NONE',  ( -0.3996062992125985480, -7.340648628747423112E-17, -1.218503937007874072 ) ) ;
#40923=CARTESIAN_POINT ( 'NONE',  ( -0.2867679344610365999, 0.2867679344610364889, -0.9566929133858265155 ) ) ;
#40925=CARTESIAN_POINT ( 'NONE',  ( -0.4724409448818898682, -8.678599364036362592E-17, -0.4311023622047244208 ) ) ;
#40937=CARTESIAN_POINT ( 'NONE',  ( -0.3460692066303960313, 0.1998031496062989965, 0.2119422572178477349 ) ) ;
#40954=CARTESIAN_POINT ( 'NONE',  ( -0.1998031496062991907, -0.3460692066303959757, -0.8530183727034120755 ) ) ;
#40958=CARTESIAN_POINT ( 'NONE',  ( -0.3996062992125986035, -7.340648628747425578E-17, -2.874015748031495843 ) ) ;
#40959=CARTESIAN_POINT ( 'NONE',  ( 0.3420746716998659953, 0.1974969037888705536, -2.335958005249343827 ) ) ;
#40962=CARTESIAN_POINT ( 'NONE',  ( -0.2867679344610364334, -0.2867679344610367109, -1.153543307086613900 ) ) ;
#40969=CARTESIAN_POINT ( 'NONE',  ( 0.3917322834645669549, 2.398668435337827645E-17, -0.1981434138769535558 ) ) ;
#40975=CARTESIAN_POINT ( 'NONE',  ( 4.893765752498283924E-17, -0.3996062992125986035, -2.913385826771653697 ) ) ;
#40976=CARTESIAN_POINT ( 'NONE',  ( 0.2867679344610366554, -0.2867679344610365999, -1.827447137304149205 ) ) ;
#40984=CARTESIAN_POINT ( 'NONE',  ( -0.1958661417322836718, 0.3392501089628017219, -0.4127296587926510552 ) ) ;
#40988=EDGE_CURVE ( 'NONE', #62471, #71224, #1727, .T. ) ;
#40994=CARTESIAN_POINT ( 'NONE',  ( 0.1958661417322836440, -0.3392501089628017219, -2.288713910761154935 ) ) ;
#40996=CARTESIAN_POINT ( 'NONE',  ( -0.3996062992125987146, 0.1070741851644051862, -0.5052493438320209140 ) ) ;
#41002=CARTESIAN_POINT ( 'NONE',  ( -0.1049643490035307020, 0.3917322834645669549, -1.351049868766404538 ) ) ;
#41003=CARTESIAN_POINT ( 'NONE',  ( 0.3460692066303958092, 0.1998031496062993018, -1.940288713910761187 ) ) ;
#41009=SHAPE_DEFINITION_REPRESENTATION ( #58020, #33107 ) ;
#41013=CARTESIAN_POINT ( 'NONE',  ( 0.3917322834645670104, 2.398668435337828261E-17, 0.04724409448818902429 ) ) ;
#41020=CARTESIAN_POINT ( 'NONE',  ( 0.2867679344610365999, 0.2867679344610365999, -1.320190657971441528 ) ) ;
#41029=CARTESIAN_POINT ( 'NONE',  ( -0.3917322834645670659, -7.196005306013484475E-17, -0.03610855462698352170 ) ) ;
#41032=CARTESIAN_POINT ( 'NONE',  ( -1.157146581871515012E-16, 0.4724409448818898682, -1.651574803149606474 ) ) ;
#41048=CARTESIAN_POINT ( 'NONE',  ( -0.3420746716998660508, -0.1974969037888706924, 0.1856955380577428039 ) ) ;
#41053=CARTESIAN_POINT ( 'NONE',  ( 0.2925321140481932369, -0.2925321140481931814, -2.222440944881889813 ) ) ;
#41058=CARTESIAN_POINT ( 'NONE',  ( -0.3996062992125985480, -7.340648628747423112E-17, -1.061023622047243986 ) ) ;
#41059=CARTESIAN_POINT ( 'NONE',  ( -0.1070741851644051862, -0.3996062992125987146, -1.332020997375328086 ) ) ;
#41060=CARTESIAN_POINT ( 'NONE',  ( -9.674558042662121740E-17, 0.3949938075777409963, -1.102362204724409711 ) ) ;
#41061=CARTESIAN_POINT ( 'NONE',  ( 0.1998031496062992740, 0.3460692066303959757, -2.506561679790026087 ) ) ;
#41063=CARTESIAN_POINT ( 'NONE',  ( -0.1958661417322836718, 0.3392501089628017219, -0.3202099737532808077 ) ) ;
#41067=CARTESIAN_POINT ( 'NONE',  ( 0.3949938075777409963, 2.418639510665530743E-17, -1.769685039370078927 ) ) ;
#41071=CARTESIAN_POINT ( 'NONE',  ( 0.4724409448818896462, 0.1265901696524990294, -2.014435695538057569 ) ) ;
#41080=CARTESIAN_POINT ( 'NONE',  ( 4.797336870675655290E-17, -0.3917322834645669549, -2.520978059546244765 ) ) ;
#41087=CARTESIAN_POINT ( 'NONE',  ( 0.3917322834645669549, 2.398668435337827645E-17, -2.875308768207662347 ) ) ;
#41089=CARTESIAN_POINT ( 'NONE',  ( 0.1049643490035303689, 0.3917322834645670104, -1.717847769028871596 ) ) ;
#41092=CARTESIAN_POINT ( 'NONE',  ( 0.3949938075777411073, -0.1058382717557499464, -2.158792650918635481 ) ) ;
#41098=CARTESIAN_POINT ( 'NONE',  ( 0.1070741851644053527, 0.3996062992125986590, -0.6233595800524933672 ) ) ;
#41102=CARTESIAN_POINT ( 'NONE',  ( 0.05060072268092381115, -0.3900885325447104868, -2.755905511811024056 ) ) ;
#41103=CARTESIAN_POINT ( 'NONE',  ( 4.797336870675656522E-17, -0.3917322834645670104, -0.1633858267716536417 ) ) ;
#41109=CARTESIAN_POINT ( 'NONE',  ( 0.1958661417322836440, -0.3392501089628017219, 0.07349081364829400387 ) ) ;
#41113=CARTESIAN_POINT ( 'NONE',  ( -0.4091458600556405756, 0.2362204724409446288, -1.443569553805774230 ) ) ;
#41115=CARTESIAN_POINT ( 'NONE',  ( -0.1958661417322834220, -0.3392501089628018884, -0.6876640419947506189 ) ) ;
#41116=CARTESIAN_POINT ( 'NONE',  ( -0.2867679344610364334, -0.2867679344610367109, -2.505905511811023612 ) ) ;
#41119=CARTESIAN_POINT ( 'NONE',  ( -0.3996062992125984925, -0.1070741851644056858, 0.03477690288713908284 ) ) ;
#41124=CARTESIAN_POINT ( 'NONE',  ( 0.1049643490035303689, 0.3917322834645668994, -0.07347149786645487679 ) ) ;
#41126=CARTESIAN_POINT ( 'NONE',  ( 0.1958661417322834775, 0.3392501089628018884, -0.07152230971128617498 ) ) ;
#41131=CARTESIAN_POINT ( 'NONE',  ( 0.1049643490035304938, -0.3917322834645669549, -2.124671916010498762 ) ) ;
#41136=CARTESIAN_POINT ( 'NONE',  ( 0.2362204724409451007, -0.4091458600556402980, -0.4835958005249343938 ) ) ;
#41139=CARTESIAN_POINT ( 'NONE',  ( 0.2017716535433070613, -0.2017716535433070890, -0.3937007874015748254 ) ) ;
#41147=CARTESIAN_POINT ( 'NONE',  ( -0.1998031496062991630, -0.3460692066303959202, -1.717191601049868677 ) ) ;
#41157=CARTESIAN_POINT ( 'NONE',  ( 0.1998031496062994405, -0.3460692066303958092, -0.2493438320209973857 ) ) ;
#41158=CARTESIAN_POINT ( 'NONE',  ( -0.1058382717557503211, 0.3949938075777409408, -0.006561679790026304741 ) ) ;
#41159=CARTESIAN_POINT ( 'NONE',  ( -0.09156050430092219083, -0.3808816823641230087, -1.492482962822815952E-17 ) ) ;
#41163=CARTESIAN_POINT ( 'NONE',  ( 0.3917322834645670104, 2.398668435337828261E-17, -2.250000000000000000 ) ) ;
#41165=EDGE_CURVE ( 'NONE', #11079, #2570, #62432, .T. ) ;
#41169=CARTESIAN_POINT ( 'NONE',  ( 0.4724409448818898682, 2.892866454678787531E-17, -0.9055118110236221041 ) ) ;
#41172=ORIENTED_EDGE ( 'NONE', *, *, #14046, .T. ) ;
#41173=CARTESIAN_POINT ( 'NONE',  ( -0.2867679344610367109, 0.2867679344610365444, -0.3313841451781647240 ) ) ;
#41187=CARTESIAN_POINT ( 'NONE',  ( 0.1049643490035304938, -0.3917322834645669549, -0.7073490813648293241 ) ) ;
#41190=CARTESIAN_POINT ( 'NONE',  ( 0.3420746716998659953, 0.1974969037888705536, -1.233595800524934338 ) ) ;
#41193=VECTOR ( 'NONE', #31401, 39.37007874015748143 ) ;
#41207=ORIENTED_EDGE ( 'NONE', *, *, #6822, .F. ) ;
#41208=CARTESIAN_POINT ( 'NONE',  ( 0.1998031496062994405, -0.3460692066303958092, -1.509186351706036655 ) ) ;
#41211=CARTESIAN_POINT ( 'NONE',  ( 0.3460692066303958092, 0.1998031496062993018, -1.310367454068241511 ) ) ;
#41212=CARTESIAN_POINT ( 'NONE',  ( 0.3460692066303959202, -0.1998031496062991630, -0.4967191601049869010 ) ) ;
#41214=CARTESIAN_POINT ( 'NONE',  ( 5.785732909357575061E-17, -0.4724409448818898682, -0.07874015748031495954 ) ) ;
#41215=CARTESIAN_POINT ( 'NONE',  ( -0.1958661417322836718, 0.3392501089628017219, -2.617454068241469756 ) ) ;
#41222=CARTESIAN_POINT ( 'NONE',  ( -0.2362204724409447953, -0.4091458600556404646, -2.032152230971128848 ) ) ;
#41225=CARTESIAN_POINT ( 'NONE',  ( 0.2891555358219910499, -0.2891555358219909944, -1.750000000000000000 ) ) ;
#41234=CARTESIAN_POINT ( 'NONE',  ( -0.1998031496062994405, 0.3460692066303957537, -2.609580052493438274 ) ) ;
#41235=CARTESIAN_POINT ( 'NONE',  ( 0.2867679344610365999, -0.2867679344610365999, -2.540663098916323914 ) ) ;
#41248=CARTESIAN_POINT ( 'NONE',  ( -0.3460692066303957537, -0.1998031496062994405, -0.2867454068241469534 ) ) ;
#41251=CARTESIAN_POINT ( 'NONE',  ( -0.2867679344610365999, 0.2867679344610364889, -1.679133858267716661 ) ) ;
#41261=CARTESIAN_POINT ( 'NONE',  ( -0.1998031496062994405, 0.3460692066303957537, -0.8772965879265091083 ) ) ;
#41275=CARTESIAN_POINT ( 'NONE',  ( -0.3996062992125986035, -7.340648628747425578E-17, -0.6692913385826770867 ) ) ;
#41278=CARTESIAN_POINT ( 'NONE',  ( -0.3917322834645669549, -0.1049643490035306603, -2.400262467191600635 ) ) ;
#41289=CARTESIAN_POINT ( 'NONE',  ( 0.3392501089628018329, -0.1958661417322834497, -1.444862573981940512 ) ) ;
#41295=CARTESIAN_POINT ( 'NONE',  ( -0.1974969037888703871, -0.3420746716998661063, 0.09186351706036739728 ) ) ;
#41304=CARTESIAN_POINT ( 'NONE',  ( -0.1049643490035307020, 0.3917322834645669549, -2.138451443569553412 ) ) ;
#41316=CARTESIAN_POINT ( 'NONE',  ( 0.3996062992125986035, 0.1070741851644054776, -1.856955380577427928 ) ) ;
#41323=CARTESIAN_POINT ( 'NONE',  ( -0.4724409448818899238, 0.1265901696524986686, -0.5820209973753280863 ) ) ;
#41326=CARTESIAN_POINT ( 'NONE',  ( -0.3420746716998662729, 0.1974969037888702206, -0.4179790026246719137 ) ) ;
#41332=CARTESIAN_POINT ( 'NONE',  ( 0.3420746716998660508, 0.1974969037888705814, -0.3654855643044619407 ) ) ;
#41339=CARTESIAN_POINT ( 'NONE',  ( -0.1998031496062991630, -0.3460692066303959202, -1.402230971128609172 ) ) ;
#41342=CARTESIAN_POINT ( 'NONE',  ( -9.594673741351313045E-17, 0.3917322834645670104, -1.094488188976378007 ) ) ;
#41351=CARTESIAN_POINT ( 'NONE',  ( 0.2017716535433070613, -0.2017716535433070890, 0.000000000000000000 ) ) ;
#41368=CARTESIAN_POINT ( 'NONE',  ( 0.3460692066303959757, -0.1998031496062991907, -0.8923884514435694859 ) ) ;
#41372=CARTESIAN_POINT ( 'NONE',  ( -0.2925321140481932924, 0.2925321140481931814, -2.854330708661417138 ) ) ;
#41373=CARTESIAN_POINT ( 'NONE',  ( 0.1974969037888706369, -0.3420746716998659953, -2.454068241469816503 ) ) ;
#41376=CARTESIAN_POINT ( 'NONE',  ( -0.2867679344610365999, 0.2867679344610364889, -1.114173228346456712 ) ) ;
#41382=CARTESIAN_POINT ( 'NONE',  ( 0.3917322834645669549, 2.398668435337827645E-17, -0.5131040437982135050 ) ) ;
#41388=CARTESIAN_POINT ( 'NONE',  ( -0.2362204724409451284, 0.4091458600556402425, -0.01312335958005249326 ) ) ;
#41390=CARTESIAN_POINT ( 'NONE',  ( -0.1958661417322836995, 0.3392501089628017219, -1.584664985073177546 ) ) ;
#41396=CARTESIAN_POINT ( 'NONE',  ( -0.1049643490035307020, 0.3917322834645669549, -0.8786089238845143923 ) ) ;
#41405=CARTESIAN_POINT ( 'NONE',  ( -0.3917322834645671215, 0.1049643490035301469, -2.387139107611548905 ) ) ;
#41414=CARTESIAN_POINT ( 'NONE',  ( 0.3917322834645670104, -0.1049643490035303411, -1.141076115485564202 ) ) ;
#41415=CARTESIAN_POINT ( 'NONE',  ( 0.1070741851644053388, 0.3996062992125986035, -2.274934383202099397 ) ) ;
#41433=CARTESIAN_POINT ( 'NONE',  ( 0.3392501089628018329, 0.1958661417322835052, -1.156148663220785799 ) ) ;
#41442=CARTESIAN_POINT ( 'NONE',  ( 0.1958661417322834775, 0.3392501089628018884, -0.2985757462280333452 ) ) ;
#41445=CARTESIAN_POINT ( 'NONE',  ( 0.4724409448818897572, -0.1265901696524988906, -1.763123359580051952 ) ) ;
#41463=CARTESIAN_POINT ( 'NONE',  ( 0.3996062992125984925, 0.1070741851644054637, -2.721128608923884418 ) ) ;
#41468=CARTESIAN_POINT ( 'NONE',  ( -0.3996062992125985480, -7.340648628747423112E-17, -2.320866141732283783 ) ) ;
#41474=CARTESIAN_POINT ( 'NONE',  ( -0.3460692066303958092, -0.1998031496062994683, -1.627296587926509330 ) ) ;
#41475=CARTESIAN_POINT ( 'NONE',  ( 0.3949938075777409963, 2.418639510665530435E-17, -1.220472440944881942 ) ) ;
#41476=CARTESIAN_POINT ( 'NONE',  ( -0.1070741851644056997, 0.3996062992125986035, -2.368766404199475151 ) ) ;
#41478=CARTESIAN_POINT ( 'NONE',  ( -0.3917322834645670104, -7.196005306013484475E-17, -0.1889763779527558474 ) ) ;
#41482=CARTESIAN_POINT ( 'NONE',  ( 0.1058382717557500852, -0.3949938075777408852, -2.209317585301837639 ) ) ;
#41486=CARTESIAN_POINT ( 'NONE',  ( 0.1265901696524990294, -0.4724409448818896462, -2.604986876640420057 ) ) ;
#41495=CARTESIAN_POINT ( 'NONE',  ( -0.2867679344610364334, -0.2867679344610367109, 0.1712598425196849850 ) ) ;
#41502=CARTESIAN_POINT ( 'NONE',  ( 4.797336870675656522E-17, -0.3917322834645670104, -0.005905511811023714773 ) ) ;
#41504=CARTESIAN_POINT ( 'NONE',  ( -0.2867679344610365999, 0.2867679344610364889, -2.374015748031496287 ) ) ;
#41507=CARTESIAN_POINT ( 'NONE',  ( -0.3420746716998659953, -0.1974969037888706647, -2.257217847769029007 ) ) ;
#41511=CARTESIAN_POINT ( 'NONE',  ( -0.3996062992125987146, 0.1070741851644051862, -0.9776902887139107268 ) ) ;
#41516=CARTESIAN_POINT ( 'NONE',  ( -9.594673741351313045E-17, 0.3917322834645670104, -0.08464566929133868212 ) ) ;
#41526=CARTESIAN_POINT ( 'NONE',  ( -0.3458507752293906723, -0.3458507752293910609, -1.476377952755905554 ) ) ;
#41528=CARTESIAN_POINT ( 'NONE',  ( -0.3917322834645669549, -0.1049643490035306603, -0.6679790026246719137 ) ) ;
#41529=CARTESIAN_POINT ( 'NONE',  ( -0.2867679344610366554, 0.2867679344610365444, -2.309055118110236116 ) ) ;
#41532=CARTESIAN_POINT ( 'NONE',  ( 0.3996062992125986035, -0.1070741851644052972, -0.5032808398950130435 ) ) ;
#41537=CARTESIAN_POINT ( 'NONE',  ( 0.3392501089628018329, 0.1958661417322835052, -0.05378645849637612303 ) ) ;
#41539=CARTESIAN_POINT ( 'NONE',  ( 0.1049643490035303689, 0.3917322834645670104, -0.2355643044619423199 ) ) ;
#41544=CARTESIAN_POINT ( 'NONE',  ( -0.1049643490035302024, -0.3917322834645671215, -2.269028871391075786 ) ) ;
#41547=CARTESIAN_POINT ( 'NONE',  ( -0.3458507752293909498, 0.3458507752293907833, -0.5688976377952755792 ) ) ;
#41551=DIRECTION ( 'NONE',  ( 0.000000000000000000, 1.000000000000000000, 0.000000000000000000 ) ) ;
#41558=CARTESIAN_POINT ( 'NONE',  ( -0.3460692066303957537, -0.1998031496062994405, -1.546587926509186639 ) ) ;
#41566=CARTESIAN_POINT ( 'NONE',  ( 0.3460692066303958092, 0.1998031496062993018, -0.3654855643044619407 ) ) ;
#41567=CARTESIAN_POINT ( 'NONE',  ( -0.3996062992125986035, -0.1070741851644056997, -0.5183727034120735322 ) ) ;
#41568=CARTESIAN_POINT ( 'NONE',  ( -0.2867679344610365444, -0.2867679344610367664, -2.732958948327771420 ) ) ;
#41573=CARTESIAN_POINT ( 'NONE',  ( -0.3420746716998662729, 0.1974969037888702206, -0.7329396325459319739 ) ) ;
#41578=CARTESIAN_POINT ( 'NONE',  ( 0.2362204724409451007, -0.4091458600556402980, -0.8792650918635170898 ) ) ;
#41579=CARTESIAN_POINT ( 'NONE',  ( -0.1998031496062994683, 0.3460692066303958092, -2.375328083989501238 ) ) ;
#41582=CARTESIAN_POINT ( 'NONE',  ( 4.797336870675656522E-17, -0.3917322834645670659, -0.3904392632884007841 ) ) ;
#41583=ORIENTED_EDGE ( 'NONE', *, *, #46355, .F. ) ;
#41594=CARTESIAN_POINT ( 'NONE',  ( 0.2867679344610365999, -0.2867679344610365444, -0.5629921259842519676 ) ) ;
#41597=CARTESIAN_POINT ( 'NONE',  ( -0.2891555358219911054, 0.2891555358219909388, -0.9645669291338583307 ) ) ;
#41598=ORIENTED_EDGE ( 'NONE', *, *, #54320, .T. ) ;
#41608=CARTESIAN_POINT ( 'NONE',  ( -0.4724409448818898682, -8.678599364036362592E-17, -0.9842519685039369248 ) ) ;
#41614=CARTESIAN_POINT ( 'NONE',  ( 0.2925321140481932369, 0.2925321140481932369, -1.712598425196850460 ) ) ;
#41617=CARTESIAN_POINT ( 'NONE',  ( -0.3996062992125986590, 0.1070741851644051723, -1.369422572178477404 ) ) ;
#41618=CARTESIAN_POINT ( 'NONE',  ( 0.1070741851644053388, 0.3996062992125986035, -0.7001312335958002064 ) ) ;
#41621=CARTESIAN_POINT ( 'NONE',  ( -0.4724409448818899238, 0.1265901696524986686, 0.1246719160104986929 ) ) ;
#41622=CARTESIAN_POINT ( 'NONE',  ( -0.2867679344610364334, -0.2867679344610367109, -2.348425196850393970 ) ) ;
#41628=CARTESIAN_POINT ( 'NONE',  ( -0.4091458600556402980, -0.2362204724409451284, -1.861548556430446144 ) ) ;
#41631=CARTESIAN_POINT ( 'NONE',  ( 0.2891555358219910499, -0.2891555358219909944, -1.907480314960629419 ) ) ;
#41634=DIRECTION ( 'NONE',  ( -0.000000000000000000, -0.000000000000000000, 1.000000000000000000 ) ) ;
#41637=CARTESIAN_POINT ( 'NONE',  ( 0.4091458600556403535, 0.2362204724409449896, -2.255249343832020692 ) ) ;
#41640=CARTESIAN_POINT ( 'NONE',  ( 0.1070741851644054776, -0.3996062992125984925, -2.681758530183727895 ) ) ;
#41642=CARTESIAN_POINT ( 'NONE',  ( -0.2867679344610366554, 0.2867679344610365444, -2.619403256396638735 ) ) ;
#41654=CARTESIAN_POINT ( 'NONE',  ( 0.3460692066303959202, -0.1998031496062991630, -0.1817585301837270351 ) ) ;
#41656=CARTESIAN_POINT ( 'NONE',  ( -0.3392501089628019995, 0.1958661417322832277, -1.843175853018372834 ) ) ;
#41665=CARTESIAN_POINT ( 'NONE',  ( -0.2925321140481932369, 0.2925321140481931259, -1.041338582677165281 ) ) ;
#41673=CARTESIAN_POINT ( 'NONE',  ( 0.3726288332213487653, 0.1208384647389236927, -1.220472440944882164 ) ) ;
#41678=CARTESIAN_POINT ( 'NONE',  ( -0.2925321140481932924, 0.2925321140481931814, -0.4921259842519684624 ) ) ;
#41681=CARTESIAN_POINT ( 'NONE',  ( -0.2867679344610365999, 0.2867679344610364889, -2.374015748031496287 ) ) ;
#41691=CARTESIAN_POINT ( 'NONE',  ( -9.594673741351310580E-17, 0.3917322834645669549, -1.497356012302150763 ) ) ;
#41697=CARTESIAN_POINT ( 'NONE',  ( 0.3917322834645670659, -0.1049643490035303273, -2.942932701608610646 ) ) ;
#41706=CARTESIAN_POINT ( 'NONE',  ( -0.2867679344610365444, -0.2867679344610367664, -1.315636113682101982 ) ) ;
#41708=CARTESIAN_POINT ( 'NONE',  ( -0.1049643490035302024, -0.3917322834645671215, -2.204068241469816503 ) ) ;
#41714=CARTESIAN_POINT ( 'NONE',  ( -0.2925321140481930149, -0.2925321140481933480, 0.02165354330708659653 ) ) ;
#41716=CARTESIAN_POINT ( 'NONE',  ( -0.3996062992125987146, 0.1070741851644051862, -1.765091863517059823 ) ) ;
#41720=CARTESIAN_POINT ( 'NONE',  ( 0.3458507752293908943, 0.3458507752293908943, -0.6870078740157479213 ) ) ;
#41723=CARTESIAN_POINT ( 'NONE',  ( 0.2891555358219910499, -0.2891555358219909944, -0.4901574803149606474 ) ) ;
#41728=CARTESIAN_POINT ( 'NONE',  ( 0.1058382717557500852, -0.3949938075777408852, -0.3195538057742782212 ) ) ;
#41732=CARTESIAN_POINT ( 'NONE',  ( 0.4724409448818898127, -0.1265901696524988629, -0.1883202099737532331 ) ) ;
#41735=CARTESIAN_POINT ( 'NONE',  ( -0.2925321140481932369, 0.2925321140481931259, -1.356299212598425452 ) ) ;
#41737=CARTESIAN_POINT ( 'NONE',  ( 0.2867679344610365999, -0.2867679344610365444, -1.035433070866141447 ) ) ;
#41751=CYLINDRICAL_SURFACE ( 'NONE', #1064, 0.4724409448818898682 ) ;
#41765=LINE ( 'NONE', #16537, #40628 ) ;
#41766=CARTESIAN_POINT ( 'NONE',  ( 0.3460692066303959757, -0.1998031496062991907, -1.207349081364829324 ) ) ;
#41770=CARTESIAN_POINT ( 'NONE',  ( -0.4724409448818898682, -8.678599364036362592E-17, -0.03937007874015747977 ) ) ;
#41771=CARTESIAN_POINT ( 'NONE',  ( 0.1974969037888704704, 0.3420746716998660508, -2.506561679790026087 ) ) ;
#41774=CARTESIAN_POINT ( 'NONE',  ( -0.1958661417322834220, -0.3392501089628018884, -1.002624671916010568 ) ) ;
#41782=CARTESIAN_POINT ( 'NONE',  ( 4.797336870675655290E-17, -0.3917322834645669549, -0.3162536500974260090 ) ) ;
#41791=CARTESIAN_POINT ( 'NONE',  ( -0.3917322834645670104, -0.1049643490035307020, -1.774953698983938954 ) ) ;
#41797=CARTESIAN_POINT ( 'NONE',  ( 0.3917322834645670104, 2.398668435337828261E-17, -0.8326771653543307838 ) ) ;
#41806=CARTESIAN_POINT ( 'NONE',  ( 0.2867679344610365999, 0.2867679344610365999, -2.334645669291338432 ) ) ;
#41813=CARTESIAN_POINT ( 'NONE',  ( 0.2867679344610365999, 0.2867679344610365999, -0.8523622047244096001 ) ) ;
#41816=CARTESIAN_POINT ( 'NONE',  ( -0.3917322834645671215, 0.1049643490035301469, -1.377296587926508664 ) ) ;
#41817=CARTESIAN_POINT ( 'NONE',  ( -0.3996062992125986590, 0.1070741851644051723, -2.471784776902887337 ) ) ;
#41830=CARTESIAN_POINT ( 'NONE',  ( -0.3917322834645669549, -0.1049643490035306603, 0.1194225721784776956 ) ) ;
#41837=CARTESIAN_POINT ( 'NONE',  ( 0.1958661417322836162, -0.3392501089628018329, -1.431739214401887894 ) ) ;
#41847=CARTESIAN_POINT ( 'NONE',  ( -0.2867679344610367109, 0.2867679344610365444, -0.6463447750994246732 ) ) ;
#41850=CARTESIAN_POINT ( 'NONE',  ( -0.2362204724409447953, -0.4091458600556404646, -2.032152230971128848 ) ) ;
#41871=CARTESIAN_POINT ( 'NONE',  ( -0.3996062992125984925, -0.1070741851644056858, -2.169947506561679340 ) ) ;
#41876=CARTESIAN_POINT ( 'NONE',  ( 0.2925321140481932369, -0.2925321140481932369, -1.673228346456692828 ) ) ;
#41877=CARTESIAN_POINT ( 'NONE',  ( 0.3420746716998659953, 0.1974969037888705536, -0.9186351706036742781 ) ) ;
#41878=CARTESIAN_POINT ( 'NONE',  ( 0.3996062992125986035, 0.1070741851644054776, -2.486876640419947382 ) ) ;
#41880=CARTESIAN_POINT ( 'NONE',  ( -0.3917322834645669549, -0.1049643490035306603, -0.03805774278215218187 ) ) ;
#41885=CARTESIAN_POINT ( 'NONE',  ( -0.3949938075777409963, -7.255918531996591613E-17, -2.320866141732283339 ) ) ;
#41889=CARTESIAN_POINT ( 'NONE',  ( 0.4724409448818896462, 0.1265901696524990294, -2.329396325459317296 ) ) ;
#41890=CARTESIAN_POINT ( 'NONE',  ( 0.3460692066303959757, -0.1998031496062991907, -1.679790026246719137 ) ) ;
#41898=CARTESIAN_POINT ( 'NONE',  ( -0.1958661417322836718, 0.3392501089628017219, 0.2171916010498686767 ) ) ;
#41905=CARTESIAN_POINT ( 'NONE',  ( -0.3392501089628019995, 0.1958661417322832277, -0.1108923884514436548 ) ) ;
#41907=CARTESIAN_POINT ( 'NONE',  ( -0.2867679344610365999, 0.2867679344610364889, -2.216535433070866201 ) ) ;
#41910=CARTESIAN_POINT ( 'NONE',  ( 0.2891555358219910499, -0.2891555358219909944, -2.145669291338582862 ) ) ;
#41911=ORIENTED_EDGE ( 'NONE', *, *, #74772, .F. ) ;
#41914=CARTESIAN_POINT ( 'NONE',  ( -0.3996062992125987146, 0.1070741851644051862, -1.135170603674540590 ) ) ;
#41918=CARTESIAN_POINT ( 'NONE',  ( 0.001150535885519430191, -0.3985446848723403490, -2.755905511811024500 ) ) ;
#41920=CARTESIAN_POINT ( 'NONE',  ( 0.2867679344610365999, 0.2867679344610365999, 0.09251968503937001154 ) ) ;
#41927=CARTESIAN_POINT ( 'NONE',  ( 0.3392501089628018884, -0.1958661417322834220, 0.06036745406824151755 ) ) ;
#41931=CARTESIAN_POINT ( 'NONE',  ( 5.785732909357575061E-17, -0.4724409448818898682, -1.496062992125984259 ) ) ;
#41933=CARTESIAN_POINT ( 'NONE',  ( 0.3917322834645669549, 0.1049643490035304660, -0.7467191601049868455 ) ) ;
#41934=CARTESIAN_POINT ( 'NONE',  ( -0.3392501089628017219, -0.1958661417322836718, -2.656824146981627166 ) ) ;
#41938=CARTESIAN_POINT ( 'NONE',  ( -0.4724409448818898682, -8.678599364036362592E-17, -0.1968503937007874127 ) ) ;
#41941=CARTESIAN_POINT ( 'NONE',  ( -0.3917322834645669549, -7.196005306013483243E-17, -0.1194032563966385962 ) ) ;
#41943=CARTESIAN_POINT ( 'NONE',  ( -0.3917322834645669549, -0.1049643490035306603, -0.4455380577427822120 ) ) ;
#41949=CARTESIAN_POINT ( 'NONE',  ( 0.1049643490035303689, 0.3917322834645670104, -2.347769028871391050 ) ) ;
#41953=CARTESIAN_POINT ( 'NONE',  ( 0.4724409448818898682, 2.892866454678787531E-17, -0.1948818897637795422 ) ) ;
#41964=CARTESIAN_POINT ( 'NONE',  ( -0.1998031496062994405, 0.3460692066303957537, -1.507217847769029007 ) ) ;
#41965=ADVANCED_FACE ( 'NONE', ( #11829 ), #36652, .T. ) ;
#41973=CARTESIAN_POINT ( 'NONE',  ( 4.893765752498283308E-17, -0.3996062992125985480, -0.1555118110236220763 ) ) ;
#41974=CARTESIAN_POINT ( 'NONE',  ( 0.1070741851644054915, -0.3996062992125986035, -0.5577427821522309426 ) ) ;
#41975=CARTESIAN_POINT ( 'NONE',  ( -0.3949938075777409408, -0.1058382717557502933, 0.1115485564304461441 ) ) ;
#41981=CARTESIAN_POINT ( 'NONE',  ( -0.3420746716998662729, 0.1974969037888702206, -1.047900262467191590 ) ) ;
#41986=CARTESIAN_POINT ( 'NONE',  ( 0.2362204724409451007, -0.4091458600556402980, -1.194225721784776928 ) ) ;
#41987=CARTESIAN_POINT ( 'NONE',  ( 0.3996062992125986035, -0.1070741851644053111, -2.158792650918635037 ) ) ;
#41990=CARTESIAN_POINT ( 'NONE',  ( -9.594673741351313045E-17, 0.3917322834645670659, -0.3116991058080859078 ) ) ;
#42003=CARTESIAN_POINT ( 'NONE',  ( -0.1049643490035307020, 0.3917322834645669549, -1.101049868766403872 ) ) ;
#42006=CARTESIAN_POINT ( 'NONE',  ( -0.2891555358219908833, -0.2891555358219912164, -1.161417322834645827 ) ) ;
#42007=EDGE_LOOP ( 'NONE', ( #75211, #20066, #68588, #17411 ) ) ;
#42023=CARTESIAN_POINT ( 'NONE',  ( 0.1998031496062992740, 0.3460692066303959757, -1.719160104986876769 ) ) ;
#42026=CARTESIAN_POINT ( 'NONE',  ( -0.3460692066303960313, 0.1998031496062989965, -1.047900262467191590 ) ) ;
#42030=CARTESIAN_POINT ( 'NONE',  ( 0.4724409448818898682, 2.892866454678787531E-17, -0.2755905511811023723 ) ) ;
#42032=CARTESIAN_POINT ( 'NONE',  ( 0.3392501089628018884, -0.1958661417322834220, -2.551837270341207109 ) ) ;
#42038=CARTESIAN_POINT ( 'NONE',  ( -1.157146581871515012E-16, 0.4724409448818898682, -2.281496062992125928 ) ) ;
#42041=CARTESIAN_POINT ( 'NONE',  ( 0.3949938075777409408, -0.1058382717557499186, -1.920603674540682260 ) ) ;
#42047=CARTESIAN_POINT ( 'NONE',  ( -0.1265901696524993347, 0.4724409448818896462, -2.288057742782152015 ) ) ;
#42051=CARTESIAN_POINT ( 'NONE',  ( 4.797336870675655290E-17, -0.3917322834645669549, -2.520978059546244765 ) ) ;
#42065=CARTESIAN_POINT ( 'NONE',  ( -0.1998031496062994405, 0.3460692066303957537, -0.2473753280839895152 ) ) ;
#42067=CARTESIAN_POINT ( 'NONE',  ( -9.594673741351313045E-17, 0.3917322834645670104, -1.659448818897637734 ) ) ;
#42076=CARTESIAN_POINT ( 'NONE',  ( 0.1070741851644054776, -0.3996062992125984925, -1.106955380577427706 ) ) ;
#42084=CARTESIAN_POINT ( 'NONE',  ( -0.3392501089628019995, 0.1958661417322832277, -1.528215223097112885 ) ) ;
#42085=CARTESIAN_POINT ( 'NONE',  ( 0.3594585737333455544, 0.1614515132151695398, -1.220472440944881720 ) ) ;
#42089=CARTESIAN_POINT ( 'NONE',  ( -0.1070741851644057135, 0.3996062992125984925, -2.603018372703412187 ) ) ;
#42091=CARTESIAN_POINT ( 'NONE',  ( -0.3996062992125986035, -0.1070741851644056997, -0.5183727034120735322 ) ) ;
#42094=CARTESIAN_POINT ( 'NONE',  ( -0.3917322834645669549, -0.1049643490035306603, -2.242782152230970993 ) ) ;
#42104=CARTESIAN_POINT ( 'NONE',  ( -0.3392501089628018329, -0.1958661417322836440, -1.392369135661730262 ) ) ;
#42108=CARTESIAN_POINT ( 'NONE',  ( -0.2867679344610365999, 0.2867679344610364889, 0.1456692913385827237 ) ) ;
#42111=CARTESIAN_POINT ( 'NONE',  ( 0.2867679344610366554, -0.2867679344610365999, -2.929809342028559360 ) ) ;
#42113=ORIENTED_EDGE ( 'NONE', *, *, #52589, .F. ) ;
#42118=ADVANCED_FACE ( 'NONE', ( #10991 ), #17330, .T. ) ;
#42121=CARTESIAN_POINT ( 'NONE',  ( -0.1049643490035307158, 0.3917322834645670104, -1.263142675361891731 ) ) ;
#42123=CARTESIAN_POINT ( 'NONE',  ( 0.2867679344610365999, 0.2867679344610365999, -2.427165354330708347 ) ) ;
#42127=CARTESIAN_POINT ( 'NONE',  ( 0.3392501089628018884, -0.1958661417322834220, -2.931758530183726563 ) ) ;
#42129=CARTESIAN_POINT ( 'NONE',  ( -0.2925321140481930149, -0.2925321140481933480, 0.1791338582677165503 ) ) ;
#42131=CARTESIAN_POINT ( 'NONE',  ( -0.3460692066303960868, 0.1998031496062990242, -2.230971128608923770 ) ) ;
#42136=CARTESIAN_POINT ( 'NONE',  ( -0.4724409448818895907, -0.1265901696524993070, -1.225065616797899937 ) ) ;
#42139=CARTESIAN_POINT ( 'NONE',  ( 0.1974969037888706092, -0.3420746716998660508, -0.4835958005249345049 ) ) ;
#42144=CARTESIAN_POINT ( 'NONE',  ( 0.2891555358219910499, 0.2891555358219910499, -0.5295275590551180578 ) ) ;
#42152=CARTESIAN_POINT ( 'NONE',  ( 0.3460692066303959202, -0.1998031496062991630, -1.284120734908136496 ) ) ;
#42154=CARTESIAN_POINT ( 'NONE',  ( 0.3392501089628018329, 0.1958661417322835607, -1.068241469816272771 ) ) ;
#42156=CARTESIAN_POINT ( 'NONE',  ( -0.3698506310978935119, 0.1308238996069450155, -1.587495037872345741E-17 ) ) ;
#42166=CARTESIAN_POINT ( 'NONE',  ( 0.4724409448818898682, 2.892866454678787531E-17, -0.1948818897637795422 ) ) ;
#42183=CARTESIAN_POINT ( 'NONE',  ( -0.2925321140481930704, -0.2925321140481933480, -1.161417322834645605 ) ) ;
#42187=CARTESIAN_POINT ( 'NONE',  ( 0.4724409448818898682, 2.892866454678787531E-17, -0.1181102362204724532 ) ) ;
#42188=CARTESIAN_POINT ( 'NONE',  ( -0.1058382717557503211, 0.3949938075777409408, -2.526246719160105236 ) ) ;
#42191=CARTESIAN_POINT ( 'NONE',  ( -0.1049643490035307020, 0.3917322834645669549, -0.7860892388451442558 ) ) ;
#42193=CARTESIAN_POINT ( 'NONE',  ( 0.3458507752293908943, -0.3458507752293908943, -2.303149606299212060 ) ) ;
#42199=CARTESIAN_POINT ( 'NONE',  ( -0.1958661417322834497, -0.3392501089628018884, -0.1456499755567436105 ) ) ;
#42207=CARTESIAN_POINT ( 'NONE',  ( 0.1049643490035303967, 0.3917322834645670659, -1.564979945703099062 ) ) ;
#42213=CARTESIAN_POINT ( 'NONE',  ( 0.3917322834645669549, 0.1049643490035304660, -0.8392388451443569819 ) ) ;
#42222=CARTESIAN_POINT ( 'NONE',  ( -0.1049643490035307020, 0.3917322834645669549, -2.360892388451444113 ) ) ;
#42229=CARTESIAN_POINT ( 'NONE',  ( 0.3392501089628018329, 0.1958661417322835607, -0.6883202099737534274 ) ) ;
#42232=CARTESIAN_POINT ( 'NONE',  ( -0.3460692066303960313, 0.1998031496062989965, -2.622703412073490892 ) ) ;
#42242=CARTESIAN_POINT ( 'NONE',  ( -0.1958661417322836718, 0.3392501089628017219, -0.005249343832020952200 ) ) ;
#42249=CARTESIAN_POINT ( 'NONE',  ( -0.3917322834645669549, -7.196005306013483243E-17, -1.536726091042307951 ) ) ;
#42257=CARTESIAN_POINT ( 'NONE',  ( 0.1958661417322834775, 0.3392501089628018884, -0.4560560611886632087 ) ) ;
#42261=CARTESIAN_POINT ( 'NONE',  ( 0.2362204724409449064, 0.4091458600556404646, -2.110892388451443225 ) ) ;
#42281=CARTESIAN_POINT ( 'NONE',  ( -0.1070741851644056997, 0.3996062992125984925, -2.288057742782152459 ) ) ;
#42286=CARTESIAN_POINT ( 'NONE',  ( -0.3460692066303960868, 0.1998031496062990242, -1.758530183727034180 ) ) ;
#42288=CARTESIAN_POINT ( 'NONE',  ( -0.2891555358219911054, 0.2891555358219909388, -1.279527559055118280 ) ) ;
#42289=CARTESIAN_POINT ( 'NONE',  ( 4.893765752498283924E-17, -0.3996062992125986035, -2.283464566929133799 ) ) ;
#42290=CARTESIAN_POINT ( 'NONE',  ( -1.157146581871515012E-16, 0.4724409448818898682, -0.6299212598425196763 ) ) ;
#42291=CARTESIAN_POINT ( 'NONE',  ( 4.797336870675656522E-17, -0.3917322834645670104, -0.2283464566929133410 ) ) ;
#42295=CARTESIAN_POINT ( 'NONE',  ( -0.3949938075777411073, 0.1058382717557497660, -2.314304461942256808 ) ) ;
#42299=CARTESIAN_POINT ( 'NONE',  ( -0.4724409448818895907, -0.1265901696524993070, -2.250656167979002920 ) ) ;
#42300=CARTESIAN_POINT ( 'NONE',  ( -0.3996062992125986035, -0.1070741851644056997, -1.778215223097112663 ) ) ;
#42307=CARTESIAN_POINT ( 'NONE',  ( 0.3917322834645669549, 0.1049643490035304660, 0.1056430446194224632 ) ) ;
#42314=CARTESIAN_POINT ( 'NONE',  ( -0.1049643490035302024, -0.3917322834645671215, 0.0006561679790025351077 ) ) ;
#42316=CARTESIAN_POINT ( 'NONE',  ( 0.1958661417322834775, 0.3392501089628018884, -2.341207349081364963 ) ) ;
#42319=CARTESIAN_POINT ( 'NONE',  ( 0.2891555358219910499, -0.2891555358219909944, -2.775590551181102317 ) ) ;
#42323=CARTESIAN_POINT ( 'NONE',  ( 0.2925321140481932369, -0.2925321140481932369, -0.8858267716535430658 ) ) ;
#42328=CARTESIAN_POINT ( 'NONE',  ( -0.2867679344610365999, 0.2867679344610364889, -0.1043307086614174151 ) ) ;
#42331=CARTESIAN_POINT ( 'NONE',  ( -0.3917322834645671215, 0.1049643490035301469, -2.794619422572177658 ) ) ;
#42335=CARTESIAN_POINT ( 'NONE',  ( 0.1049643490035304938, -0.3917322834645669549, -0.2349081364829396223 ) ) ;
#42336=ORIENTED_EDGE ( 'NONE', *, *, #71870, .T. ) ;
#42340=CARTESIAN_POINT ( 'NONE',  ( 0.1265901696524990294, -0.4724409448818896462, -1.502624671916010346 ) ) ;
#42343=CARTESIAN_POINT ( 'NONE',  ( 0.3458507752293908943, 0.3458507752293908943, -0.9251968503937008093 ) ) ;
#42350=CARTESIAN_POINT ( 'NONE',  ( -0.3392501089628018329, -0.1958661417322836440, 0.02495369898393883651 ) ) ;
#42352=CARTESIAN_POINT ( 'NONE',  ( -0.1958661417322836718, 0.3392501089628017219, -0.4127296587926510552 ) ) ;
#42357=CARTESIAN_POINT ( 'NONE',  ( 0.1958661417322834775, 0.3392501089628018884, -2.498687664041994605 ) ) ;
#42361=CARTESIAN_POINT ( 'NONE',  ( 0.4724409448818896462, 0.1265901696524990294, -0.8313648293963252778 ) ) ;
#42373=CARTESIAN_POINT ( 'NONE',  ( -9.787531504996566615E-17, 0.3996062992125985480, -1.966535433070865979 ) ) ;
#42381=CARTESIAN_POINT ( 'NONE',  ( -0.2925321140481932369, 0.2925321140481930704, -0.4114173228346456046 ) ) ;
#42382=CARTESIAN_POINT ( 'NONE',  ( -0.1998031496062991907, -0.3460692066303959757, -0.5380577427821522374 ) ) ;
#42383=CARTESIAN_POINT ( 'NONE',  ( 0.1049643490035303967, 0.3917322834645670659, -2.824822465388138415 ) ) ;
#42389=CARTESIAN_POINT ( 'NONE',  ( 4.837279021331061486E-17, -0.3949938075777409963, -0.7854330708661416693 ) ) ;
#42394=CARTESIAN_POINT ( 'NONE',  ( 0.4724409448818898682, 2.892866454678787531E-17, -1.062992125984252079 ) ) ;
#42395=CARTESIAN_POINT ( 'NONE',  ( -0.1998031496062991907, -0.3460692066303959757, -2.427821522309711266 ) ) ;
#42399=CARTESIAN_POINT ( 'NONE',  ( 0.2867679344610366554, 0.2867679344610366554, -0.9219353262805269900 ) ) ;
#42411=CARTESIAN_POINT ( 'NONE',  ( -0.2867679344610365999, 0.2867679344610364889, -1.114173228346456712 ) ) ;
#42414=CARTESIAN_POINT ( 'NONE',  ( 0.1974969037888704704, 0.3420746716998660508, -1.246719160104986734 ) ) ;
#42415=VERTEX_POINT ( 'NONE', #77873 ) ;
#42418=CARTESIAN_POINT ( 'NONE',  ( -0.2925321140481932924, 0.2925321140481931814, 0.1377952755905511584 ) ) ;
#42424=CARTESIAN_POINT ( 'NONE',  ( 5.785732909357575061E-17, -0.4724409448818898682, -1.023622047244094446 ) ) ;
#42425=CARTESIAN_POINT ( 'NONE',  ( 0.2362204724409451007, -0.4091458600556402980, -0.6410761154855643129 ) ) ;
#42430=CARTESIAN_POINT ( 'NONE',  ( -0.1070741851644051862, -0.3996062992125987146, -1.646981627296587591 ) ) ;
#42433=CARTESIAN_POINT ( 'NONE',  ( -0.1070741851644056997, 0.3996062992125984925, -1.185695538057742526 ) ) ;
#42437=CARTESIAN_POINT ( 'NONE',  ( -0.1265901696524993347, 0.4724409448818895907, -0.4790026246719158998 ) ) ;
#42439=CARTESIAN_POINT ( 'NONE',  ( 0.3917322834645669549, 0.1049643490035304660, -2.571522309711286258 ) ) ;
#42446=CARTESIAN_POINT ( 'NONE',  ( 0.4724409448818898682, 2.892866454678787531E-17, -2.242125984251968518 ) ) ;
#42448=CARTESIAN_POINT ( 'NONE',  ( -0.3420746716998662729, 0.1974969037888702206, -1.677821522309711710 ) ) ;
#42458=CARTESIAN_POINT ( 'NONE',  ( 0.2867679344610365999, 0.2867679344610365999, -2.580033177656481325 ) ) ;
#42471=CARTESIAN_POINT ( 'NONE',  ( -0.3996062992125984925, -0.1070741851644056858, -0.7526246719160103460 ) ) ;
#42472=CARTESIAN_POINT ( 'NONE',  ( 0.2867679344610365999, 0.2867679344610365999, -1.639763779527558807 ) ) ;
#42477=CARTESIAN_POINT ( 'NONE',  ( 0.4724409448818898682, 0.000000000000000000, -2.755905511811024056 ) ) ;
#42482=CARTESIAN_POINT ( 'NONE',  ( 0.1998031496062992463, 0.3460692066303959202, -1.480971128608923992 ) ) ;
#42484=CARTESIAN_POINT ( 'NONE',  ( -0.3458507752293909498, 0.3458507752293908388, -2.224409448818897683 ) ) ;
#42485=ORIENTED_EDGE ( 'NONE', *, *, #33290, .T. ) ;
#42490=CARTESIAN_POINT ( 'NONE',  ( -9.594673741351313045E-17, 0.3917322834645670104, -1.659448818897637734 ) ) ;
#42498=CARTESIAN_POINT ( 'NONE',  ( -0.3460692066303960313, 0.1998031496062989965, -2.465223097112860806 ) ) ;
#42500=CARTESIAN_POINT ( 'NONE',  ( -0.2925321140481930704, -0.2925321140481933480, -0.8464566929133857665 ) ) ;
#42503=CARTESIAN_POINT ( 'NONE',  ( 0.3917322834645670104, 2.398668435337828261E-17, -2.629921259842519898 ) ) ;
#42513=CARTESIAN_POINT ( 'NONE',  ( -0.1049643490035306742, 0.3917322834645668994, -1.661398007052806269 ) ) ;
#42518=CARTESIAN_POINT ( 'NONE',  ( -0.1958661417322834220, -0.3392501089628018884, -2.827427821522309426 ) ) ;
#42521=CARTESIAN_POINT ( 'NONE',  ( -0.1049643490035302301, -0.3917322834645671770, -2.746082307907824038 ) ) ;
#42530=CARTESIAN_POINT ( 'NONE',  ( 0.3917322834645670104, 0.1049643490035304660, -1.381252911582363962 ) ) ;
#42532=CARTESIAN_POINT ( 'NONE',  ( 0.1049643490035303689, 0.3917322834645670104, -2.125328083989501682 ) ) ;
#42537=CARTESIAN_POINT ( 'NONE',  ( -0.2925321140481932924, 0.2925321140481931814, -0.4921259842519684624 ) ) ;
#42539=CARTESIAN_POINT ( 'NONE',  ( -0.2925321140481932369, 0.2925321140481931259, 0.2185039370078740162 ) ) ;
#42541=CARTESIAN_POINT ( 'NONE',  ( 0.3996062992125986035, 2.446882876249141962E-17, -2.322834645669291209 ) ) ;
#42546=CARTESIAN_POINT ( 'NONE',  ( 5.785732909357575061E-17, -0.4724409448818898682, -1.100393700787401619 ) ) ;
#42549=CARTESIAN_POINT ( 'NONE',  ( -0.1058382717557503072, 0.3949938075777408852, -0.7132545931758530466 ) ) ;
#42561=CARTESIAN_POINT ( 'NONE',  ( 0.1998031496062992463, 0.3460692066303959202, -1.953412073490813805 ) ) ;
#42564=CARTESIAN_POINT ( 'NONE',  ( 0.1049643490035303689, 0.3917322834645670104, -1.245406824146981561 ) ) ;
#42589=CARTESIAN_POINT ( 'NONE',  ( 0.2867679344610366554, -0.2867679344610365999, -1.984927452264778847 ) ) ;
#42594=DIRECTION ( 'NONE',  ( 0.000000000000000000, 0.000000000000000000, 1.000000000000000000 ) ) ;
#42598=CARTESIAN_POINT ( 'NONE',  ( 0.3460692066303959757, -0.1998031496062991907, -2.939632545931758489 ) ) ;
#42599=CARTESIAN_POINT ( 'NONE',  ( 0.1974969037888704704, 0.3420746716998660508, -2.664041994750656173 ) ) ;
#42602=CARTESIAN_POINT ( 'NONE',  ( 0.3917322834645669549, 0.1049643490035304660, -0.9041994750656167090 ) ) ;
#42604=CARTESIAN_POINT ( 'NONE',  ( 0.4724409448818897572, -0.1265901696524988906, -2.473753280839894764 ) ) ;
#42611=CARTESIAN_POINT ( 'NONE',  ( 0.2867679344610365999, 0.2867679344610365999, -0.3753087682076623466 ) ) ;
#42619=CARTESIAN_POINT ( 'NONE',  ( -0.2867679344610365444, -0.2867679344610367664, -1.788077058563991795 ) ) ;
#42627=CARTESIAN_POINT ( 'NONE',  ( 0.3917322834645670104, -0.1049643490035303411, -0.9835958005249345604 ) ) ;
#42636=CARTESIAN_POINT ( 'NONE',  ( -0.3917322834645670104, -7.196005306013484475E-17, -2.236220472440944906 ) ) ;
#42642=FACE_OUTER_BOUND ( 'NONE', #65624, .T. ) ;
#42643=CARTESIAN_POINT ( 'NONE',  ( -0.1049643490035302024, -0.3917322834645671215, -0.6292650918635172008 ) ) ;
#42646=CARTESIAN_POINT ( 'NONE',  ( -0.1998031496062991630, -0.3460692066303959202, -2.347112860892388575 ) ) ;
#42657=CARTESIAN_POINT ( 'NONE',  ( 0.1049643490035304938, -0.3917322834645669549, 0.08005249343832024356 ) ) ;
#42664=CARTESIAN_POINT ( 'NONE',  ( -0.2867679344610364334, -0.2867679344610368219, -1.556411130412386656 ) ) ;
#42673=CARTESIAN_POINT ( 'NONE',  ( -0.1958661417322833942, -0.3392501089628018884, -0.3773159037083483325 ) ) ;
#42677=CARTESIAN_POINT ( 'NONE',  ( -0.4724409448818899238, 0.1265901696524986686, -1.841863517060367439 ) ) ;
#42698=CARTESIAN_POINT ( 'NONE',  ( 0.1070741851644054776, -0.3996062992125984925, -2.366797900262467280 ) ) ;
#42703=CARTESIAN_POINT ( 'NONE',  ( -0.1998031496062994683, 0.3460692066303958092, -1.587926509186351698 ) ) ;
#42704=CARTESIAN_POINT ( 'NONE',  ( 0.3420746716998660508, -0.1974969037888703871, -1.049868766404199460 ) ) ;
#42705=CARTESIAN_POINT ( 'NONE',  ( 0.2925321140481932369, 0.2925321140481932369, -2.500000000000000444 ) ) ;
#42707=CARTESIAN_POINT ( 'NONE',  ( 0.2867679344610366554, 0.2867679344610366554, -0.7598425196850391306 ) ) ;
#42711=CARTESIAN_POINT ( 'NONE',  ( 4.837279021331061486E-17, -0.3949938075777409963, -2.360236220472441193 ) ) ;
#42714=CARTESIAN_POINT ( 'NONE',  ( -0.1265901696524993347, 0.4724409448818895907, -2.526246719160104792 ) ) ;
#42715=CARTESIAN_POINT ( 'NONE',  ( -0.3460692066303960868, 0.1998031496062990242, -1.758530183727034180 ) ) ;
#42721=CARTESIAN_POINT ( 'NONE',  ( -0.3917322834645670659, 0.1049643490035301607, -2.632526615976691353 ) ) ;
#42722=LINE ( 'NONE', #10758, #4735 ) ;
#42728=CARTESIAN_POINT ( 'NONE',  ( -9.594673741351313045E-17, 0.3917322834645670104, -0.08464566929133868212 ) ) ;
#42730=CARTESIAN_POINT ( 'NONE',  ( 0.3917322834645670104, -0.1049643490035303411, -2.465879265091863282 ) ) ;
#42733=CARTESIAN_POINT ( 'NONE',  ( 0.3949938075777409408, 0.1058382717557500574, -2.644356955380577912 ) ) ;
#42737=CARTESIAN_POINT ( 'NONE',  ( -0.1070741851644051862, -0.3996062992125987146, -1.174540682414698001 ) ) ;
#42740=FACE_OUTER_BOUND ( 'NONE', #10941, .T. ) ;
#42742=CARTESIAN_POINT ( 'NONE',  ( 4.797336870675656522E-17, -0.3917322834645670104, -0.6358267716535433989 ) ) ;
#42744=EDGE_CURVE ( 'NONE', #48835, #10673, #39559, .T. ) ;
#42749=CARTESIAN_POINT ( 'NONE',  ( 0.3917322834645670104, -0.1049643490035303411, -0.2611548556430445256 ) ) ;
#42754=CARTESIAN_POINT ( 'NONE',  ( -0.1265901696524986964, -0.4724409448818899238, -1.804461942257217677 ) ) ;
#42763=CARTESIAN_POINT ( 'NONE',  ( 0.1958661417322834497, 0.3392501089628018329, -0.3818704479976884336 ) ) ;
#42765=CARTESIAN_POINT ( 'NONE',  ( -0.3917322834645671215, 0.1049643490035301469, -0.2749343832020998413 ) ) ;
#42770=CARTESIAN_POINT ( 'NONE',  ( 0.3917322834645670104, -0.1049643490035303411, -2.150918635170603554 ) ) ;
#42773=CARTESIAN_POINT ( 'NONE',  ( -0.4724409448818895907, -0.1265901696524993070, -0.7526246719160103460 ) ) ;
#42785=CARTESIAN_POINT ( 'NONE',  ( -9.787531504996566615E-17, 0.3996062992125985480, -2.124015748031495843 ) ) ;
#42793=CARTESIAN_POINT ( 'NONE',  ( 4.893765752498283308E-17, -0.3996062992125985480, -0.3129921259842520231 ) ) ;
#42794=CARTESIAN_POINT ( 'NONE',  ( -0.3996062992125987146, 0.1070741851644051862, -0.6627296587926508886 ) ) ;
#42795=CARTESIAN_POINT ( 'NONE',  ( -0.3420746716998659953, -0.1974969037888706647, 0.1049868766404198905 ) ) ;
#42801=CARTESIAN_POINT ( 'NONE',  ( -0.2891555358219909388, -0.2891555358219912164, -1.080708661417322913 ) ) ;
#42806=CARTESIAN_POINT ( 'NONE',  ( -0.4724409448818898682, -8.678599364036362592E-17, -0.9842519685039369248 ) ) ;
#42807=CARTESIAN_POINT ( 'NONE',  ( 4.893765752498283924E-17, -0.3996062992125986035, -2.440944881889763884 ) ) ;
#42810=CARTESIAN_POINT ( 'NONE',  ( 0.3917322834645670659, -0.1049643490035303273, -0.8956886071204221977 ) ) ;
#42822=CARTESIAN_POINT ( 'NONE',  ( 0.1958661417322834775, 0.3392501089628018884, -0.9238845144356954142 ) ) ;
#42825=CARTESIAN_POINT ( 'NONE',  ( -0.1974969037888706647, 0.3420746716998658843, -1.272965879265091749 ) ) ;
#42836=CARTESIAN_POINT ( 'NONE',  ( 0.3917322834645669549, 0.1049643490035304660, -0.05183727034120744204 ) ) ;
#42842=CARTESIAN_POINT ( 'NONE',  ( -0.1998031496062994683, 0.3460692066303958092, -2.060367454068241511 ) ) ;
#42845=CARTESIAN_POINT ( 'NONE',  ( -0.2925321140481932369, 0.2925321140481931259, -1.513779527559054872 ) ) ;
#42849=CARTESIAN_POINT ( 'NONE',  ( 0.4724409448818896462, 0.1265901696524990294, -0.4396325459317584339 ) ) ;
#42851=CARTESIAN_POINT ( 'NONE',  ( 0.1958661417322834775, 0.3392501089628018884, -2.433727034120734878 ) ) ;
#42857=CARTESIAN_POINT ( 'NONE',  ( -0.3458507752293906723, -0.3458507752293910609, -2.183070866141731958 ) ) ;
#42859=CARTESIAN_POINT ( 'NONE',  ( -0.1974969037888704149, -0.3420746716998661063, -2.347112860892388575 ) ) ;
#42880=CARTESIAN_POINT ( 'NONE',  ( -9.787531504996566615E-17, 0.3996062992125985480, -0.8641732283464567121 ) ) ;
#42881=CARTESIAN_POINT ( 'NONE',  ( -0.3917322834645670104, -7.196005306013484475E-17, -2.171259842519685179 ) ) ;
#42891=CARTESIAN_POINT ( 'NONE',  ( 4.893765752498283308E-17, -0.3996062992125985480, -1.572834645669291431 ) ) ;
#42898=CARTESIAN_POINT ( 'NONE',  ( 0.2867679344610365999, 0.2867679344610365999, -1.482283464566929387 ) ) ;
#42903=CARTESIAN_POINT ( 'NONE',  ( -0.2925321140481932369, 0.2925321140481930704, -2.301181102362204633 ) ) ;
#42905=CARTESIAN_POINT ( 'NONE',  ( 0.3996062992125986590, -0.1070741851644053111, -0.8989501312335956840 ) ) ;
#42908=CARTESIAN_POINT ( 'NONE',  ( 0.3917322834645670104, -0.1049643490035303411, -2.465879265091863282 ) ) ;
#42918=CARTESIAN_POINT ( 'NONE',  ( 0.3392501089628018329, 0.1958661417322835052, -1.786069923063305032 ) ) ;
#42921=CARTESIAN_POINT ( 'NONE',  ( 0.2867679344610365999, -0.2867679344610365444, 0.06692913385826775030 ) ) ;
#42924=CARTESIAN_POINT ( 'NONE',  ( 0.3949938075777409408, 0.1058382717557500574, -0.2821522309711286813 ) ) ;
#42932=CARTESIAN_POINT ( 'NONE',  ( -0.3917322834645670659, -7.196005306013484475E-17, -1.138470759351392969 ) ) ;
#42935=CARTESIAN_POINT ( 'NONE',  ( 0.3392501089628018884, -0.1958661417322834220, -2.709317585301837195 ) ) ;
#42940=CARTESIAN_POINT ( 'NONE',  ( 0.3996062992125986590, -0.1070741851644053111, -1.056430446194225992 ) ) ;
#42942=CARTESIAN_POINT ( 'NONE',  ( -0.3996062992125984925, -0.1070741851644056858, -0.4376640419947506744 ) ) ;
#42944=CARTESIAN_POINT ( 'NONE',  ( -0.1070741851644056997, 0.3996062992125986035, -2.211286089238845065 ) ) ;
#42949=CARTESIAN_POINT ( 'NONE',  ( 0.1265901696524990294, -0.4724409448818896462, -1.264435695538057569 ) ) ;
#42951=ADVANCED_FACE ( 'NONE', ( #14742 ), #2932, .T. ) ;
#42953=CARTESIAN_POINT ( 'NONE',  ( -9.674558042662122972E-17, 0.3949938075777409963, -0.5492125984251968740 ) ) ;
#42967=CARTESIAN_POINT ( 'NONE',  ( -0.3996062992125984925, -0.1070741851644056858, -1.697506561679790194 ) ) ;
#42969=CARTESIAN_POINT ( 'NONE',  ( -0.1049643490035302024, -0.3917322834645671215, -1.324146981627296826 ) ) ;
#42970=CARTESIAN_POINT ( 'NONE',  ( -0.2749078412854699671, -0.2798680777847345480, 3.457013956890523347E-17 ) ) ;
#42983=CARTESIAN_POINT ( 'NONE',  ( -0.4724409448818898682, -8.678599364036362592E-17, -0.2736220472440945017 ) ) ;
#42999=CARTESIAN_POINT ( 'NONE',  ( -0.1070741851644051862, -0.3996062992125986590, -1.174540682414698445 ) ) ;
#43000=CARTESIAN_POINT ( 'NONE',  ( -0.3917322834645670104, -7.196005306013484475E-17, -2.236220472440944906 ) ) ;
#43003=CARTESIAN_POINT ( 'NONE',  ( -0.3458507752293909498, 0.3458507752293907833, -0.3346456692913385988 ) ) ;
#43004=CARTESIAN_POINT ( 'NONE',  ( -0.3420746716998661618, 0.1974969037888702206, -2.860892388451444113 ) ) ;
#43007=CARTESIAN_POINT ( 'NONE',  ( -0.1049643490035307020, 0.3917322834645669549, -1.573490813648293907 ) ) ;
#43009=CARTESIAN_POINT ( 'NONE',  ( -0.1265901696524986964, -0.4724409448818899238, -2.591863517060367439 ) ) ;
#43016=CARTESIAN_POINT ( 'NONE',  ( -0.2867679344610366554, 0.2867679344610365444, -0.7296394768690795951 ) ) ;
#43021=CYLINDRICAL_SURFACE ( 'NONE', #73066, 0.4724409448818898682 ) ;
#43023=CARTESIAN_POINT ( 'NONE',  ( -0.3392501089628019995, 0.1958661417322831999, -2.227709604495750284 ) ) ;
#43029=CARTESIAN_POINT ( 'NONE',  ( -0.3917322834645670104, -7.196005306013484475E-17, -0.9114173228346457156 ) ) ;
#43039=CARTESIAN_POINT ( 'NONE',  ( 0.1049643490035304938, -0.3917322834645669549, -2.597112860892388131 ) ) ;
#43040=ORIENTED_EDGE ( 'NONE', *, *, #31271, .T. ) ;
#43046=CARTESIAN_POINT ( 'NONE',  ( 0.3917322834645669549, 0.1049643490035304660, -0.9967191601049870675 ) ) ;
#43049=CARTESIAN_POINT ( 'NONE',  ( -0.3996062992125984925, -0.1070741851644056858, -2.484908136482939955 ) ) ;
#43058=CARTESIAN_POINT ( 'NONE',  ( 0.2925321140481932369, 0.2925321140481932369, -0.3720472440944882497 ) ) ;
#43060=CARTESIAN_POINT ( 'NONE',  ( 0.3917322834645670104, 2.398668435337828261E-17, -0.1102362204724409156 ) ) ;
#43067=CARTESIAN_POINT ( 'NONE',  ( -0.1958661417322836440, 0.3392501089628016664, -1.825440001803462886 ) ) ;
#43076=CARTESIAN_POINT ( 'NONE',  ( -0.1049643490035307158, 0.3917322834645670104, -0.4757411005587420805 ) ) ;
#43080=CARTESIAN_POINT ( 'NONE',  ( 0.4091458600556404646, -0.2362204724409448231, -1.914041994750656395 ) ) ;
#43101=CARTESIAN_POINT ( 'NONE',  ( -0.1070741851644051862, -0.3996062992125986590, -2.826115485564304475 ) ) ;
#43106=CARTESIAN_POINT ( 'NONE',  ( -0.1998031496062994683, 0.3460692066303958092, -1.902887139107611647 ) ) ;
#43107=CARTESIAN_POINT ( 'NONE',  ( -0.3420746716998659953, -0.1974969037888706647, -1.312335958005249159 ) ) ;
#43108=CARTESIAN_POINT ( 'NONE',  ( -0.1070741851644051862, -0.3996062992125987146, -2.906824146981627610 ) ) ;
#43110=CARTESIAN_POINT ( 'NONE',  ( -0.1049643490035307020, 0.3917322834645669549, -0.4711286089238844732 ) ) ;
#43114=CARTESIAN_POINT ( 'NONE',  ( -0.1058382717557497660, -0.3949938075777411073, -2.196194225721785021 ) ) ;
#43118=CARTESIAN_POINT ( 'NONE',  ( -0.4724409448818895907, -0.1265901696524993070, -2.565616797900262647 ) ) ;
#43119=CARTESIAN_POINT ( 'NONE',  ( -0.1998031496062994683, 0.3460692066303958092, -2.217847769028871596 ) ) ;
#43120=CARTESIAN_POINT ( 'NONE',  ( -0.01881781417526427053, 0.4724409448818898682, -2.754912411187758980 ) ) ;
#43126=CARTESIAN_POINT ( 'NONE',  ( 0.1049643490035304522, -0.3917322834645668994, -2.685020054296901382 ) ) ;
#43134=CARTESIAN_POINT ( 'NONE',  ( -0.3917322834645669549, -0.1049643490035306603, -0.2880577427821523484 ) ) ;
#43135=CARTESIAN_POINT ( 'NONE',  ( 0.3392501089628018329, 0.1958661417322835607, -1.698162729658792891 ) ) ;
#43136=CARTESIAN_POINT ( 'NONE',  ( -0.1958661417322834220, -0.3392501089628018884, -2.262467191601049699 ) ) ;
#43139=CARTESIAN_POINT ( 'NONE',  ( -0.3949938075777409963, -7.255918531996591613E-17, -2.716535433070866201 ) ) ;
#43143=CARTESIAN_POINT ( 'NONE',  ( 0.3996062992125986035, 0.1070741851644054776, -1.227034120734908029 ) ) ;
#43148=CARTESIAN_POINT ( 'NONE',  ( 0.1958661417322834775, 0.3392501089628018884, -0.2290026246719160941 ) ) ;
#43154=CARTESIAN_POINT ( 'NONE',  ( -0.1958661417322834220, -0.3392501089628018884, -0.2152230971128608339 ) ) ;
#43158=CARTESIAN_POINT ( 'NONE',  ( 0.3458507752293908943, -0.3458507752293908943, -1.673228346456692828 ) ) ;
#43160=CARTESIAN_POINT ( 'NONE',  ( 0.1958661417322836440, -0.3392501089628017219, -2.696194225721784576 ) ) ;
#43164=CARTESIAN_POINT ( 'NONE',  ( -0.2362204724409447953, -0.4091458600556404646, -1.955380577427821454 ) ) ;
#43167=CARTESIAN_POINT ( 'NONE',  ( 0.2867679344610365999, 0.2867679344610365999, -0.3753087682076623466 ) ) ;
#43169=CARTESIAN_POINT ( 'NONE',  ( 0.3392501089628018329, 0.1958661417322835607, -1.003280839895013266 ) ) ;
#43174=CARTESIAN_POINT ( 'NONE',  ( 0.3917322834645670104, 2.398668435337828261E-17, -2.157480314960630086 ) ) ;
#43177=CARTESIAN_POINT ( 'NONE',  ( 0.4091458600556404646, -0.2362204724409448231, -0.8116797900262466836 ) ) ;
#43189=CARTESIAN_POINT ( 'NONE',  ( -0.1998031496062991630, -0.3460692066303959202, -2.032152230971128848 ) ) ;
#43198=CARTESIAN_POINT ( 'NONE',  ( 0.3460692066303958092, 0.1998031496062993018, -0.05052493438320212332 ) ) ;
#43199=CARTESIAN_POINT ( 'NONE',  ( 4.893765752498283924E-17, -0.3996062992125986035, -0.3937007874015748254 ) ) ;
#43200=CARTESIAN_POINT ( 'NONE',  ( -0.3420746716998661618, 0.1974969037888702206, -0.3412073490813648524 ) ) ;
#43205=CARTESIAN_POINT ( 'NONE',  ( 0.1974969037888704704, 0.3420746716998660508, -0.8510498687664042050 ) ) ;
#43210=CARTESIAN_POINT ( 'NONE',  ( 0.4091458600556404646, -0.2362204724409448231, -1.364829396325459188 ) ) ;
#43211=CARTESIAN_POINT ( 'NONE',  ( 0.2925321140481932369, 0.2925321140481932369, -2.500000000000000000 ) ) ;
#43214=CARTESIAN_POINT ( 'NONE',  ( 0.1958661417322836718, -0.3392501089628017219, -0.8760035677503431595 ) ) ;
#43226=CARTESIAN_POINT ( 'NONE',  ( 0.3392501089628018329, 0.1958661417322835607, -1.225721784776902634 ) ) ;
#43229=CARTESIAN_POINT ( 'NONE',  ( 0.3949938075777409408, 0.1058382717557500574, -1.384514435695538337 ) ) ;
#43234=CARTESIAN_POINT ( 'NONE',  ( 0.1998031496062994405, -0.3460692066303958092, 0.06561679790026245240 ) ) ;
#43246=CARTESIAN_POINT ( 'NONE',  ( 0.2925321140481932369, 0.2925321140481932369, -2.027559055118109743 ) ) ;
#43249=CARTESIAN_POINT ( 'NONE',  ( -9.787531504996566615E-17, 0.3996062992125985480, -1.494094488188976388 ) ) ;
#43254=CARTESIAN_POINT ( 'NONE',  ( -1.157146581871515012E-16, 0.4724409448818898682, -0.3149606299212598381 ) ) ;
#43256=CARTESIAN_POINT ( 'NONE',  ( -0.2867679344610364334, -0.2867679344610367109, 0.1062992125984252439 ) ) ;
#43262=CARTESIAN_POINT ( 'NONE',  ( -0.4724409448818895907, -0.1265901696524993070, -2.327427821522309426 ) ) ;
#43264=CARTESIAN_POINT ( 'NONE',  ( 0.1974969037888704704, 0.3420746716998660508, -2.110892388451443225 ) ) ;
#43276=CARTESIAN_POINT ( 'NONE',  ( 0.4091458600556403535, 0.2362204724409449896, -0.9954068241469815614 ) ) ;
#43287=CARTESIAN_POINT ( 'NONE',  ( -0.3460692066303957537, -0.1998031496062994405, -0.9166666666666666297 ) ) ;
#43288=CARTESIAN_POINT ( 'NONE',  ( -0.2867679344610364334, -0.2867679344610367109, -2.348425196850393970 ) ) ;
#43297=CARTESIAN_POINT ( 'NONE',  ( -0.2362204724409451284, 0.4091458600556402425, -2.217847769028871596 ) ) ;
#43303=CARTESIAN_POINT ( 'NONE',  ( 0.3392501089628018884, -0.1958661417322834220, -1.449475065616798064 ) ) ;
#43308=CARTESIAN_POINT ( 'NONE',  ( 0.3996062992125984925, 0.1070741851644054499, -2.248687664041995049 ) ) ;
#43310=CARTESIAN_POINT ( 'NONE',  ( 4.893765752498283924E-17, -0.3996062992125986035, -1.023622047244094446 ) ) ;
#43313=CARTESIAN_POINT ( 'NONE',  ( -0.1049643490035302024, -0.3917322834645671215, -2.583989501312335513 ) ) ;
#43324=CARTESIAN_POINT ( 'NONE',  ( 0.3392501089628018884, -0.1958661417322834220, -2.709317585301837195 ) ) ;
#43327=CARTESIAN_POINT ( 'NONE',  ( -0.1974969037888706647, 0.3420746716998658843, -0.01312335958005255224 ) ) ;
#43335=CARTESIAN_POINT ( 'NONE',  ( -0.3917322834645671770, 0.1049643490035302024, -1.131909079561366882 ) ) ;
#43337=CARTESIAN_POINT ( 'NONE',  ( -0.3392501089628019995, 0.1958661417322832277, -2.788057742782152459 ) ) ;
#43342=CARTESIAN_POINT ( 'NONE',  ( 0.3996062992125986590, -0.1070741851644053111, -0.8989501312335956840 ) ) ;
#43344=CARTESIAN_POINT ( 'NONE',  ( 0.1998031496062992463, 0.3460692066303959202, -0.3786089238845143923 ) ) ;
#43346=CARTESIAN_POINT ( 'NONE',  ( -0.3996062992125986035, -7.340648628747425578E-17, -2.401574803149606474 ) ) ;
#43347=CARTESIAN_POINT ( 'NONE',  ( -0.3392501089628017219, -0.1958661417322836718, -1.554461942257217899 ) ) ;
#43351=CARTESIAN_POINT ( 'NONE',  ( 0.1265901696524989462, 0.4724409448818897572, -1.172572178477690352 ) ) ;
#43353=( BOUNDED_CURVE ( )  B_SPLINE_CURVE ( 2, ( #67890, #36298, #61972, #29567, #10227, #81765, #24075, #50560, #35894, #50154, #4311, #49744, #30804 ),
 .UNSPECIFIED., .F., .T. ) 
 B_SPLINE_CURVE_WITH_KNOTS ( ( 3, 2, 2, 2, 2, 2, 3 ),
 ( 0.3375000000000000222, 0.3416666666666666741, 0.3458333333333333259, 0.3499999999999999778, 0.3541666666666666852, 0.3583333333333333370, 0.3624999999999999889 ),
 .UNSPECIFIED. ) 
 CURVE ( )  GEOMETRIC_REPRESENTATION_ITEM ( )  RATIONAL_B_SPLINE_CURVE ( ( 1.000000000000000000, 0.9659258262890683122, 1.000000000000000000, 0.9659258262890683122, 1.000000000000000000, 0.9659258262890683122, 1.000000000000000000, 0.9659258262890683122, 1.000000000000000000, 0.9659258262890683122, 1.000000000000000000, 0.9659258262890683122, 1.000000000000000000 ) ) 
 REPRESENTATION_ITEM ( '' )  );
#43356=CARTESIAN_POINT ( 'NONE',  ( 0.1974969037888706092, -0.3420746716998660508, -0.7985564304461942875 ) ) ;
#43369=CARTESIAN_POINT ( 'NONE',  ( 4.893765752498283308E-17, -0.3996062992125985480, -1.730314960629921517 ) ) ;
#43372=CARTESIAN_POINT ( 'NONE',  ( -0.3917322834645671215, 0.1049643490035301469, -1.442257217847769057 ) ) ;
#43386=CARTESIAN_POINT ( 'NONE',  ( -0.1049643490035307020, 0.3917322834645669549, -0.8786089238845143923 ) ) ;
#43397=VECTOR ( 'NONE', #30478, 39.37007874015748143 ) ;
#43403=CARTESIAN_POINT ( 'NONE',  ( -0.3460692066303958092, -0.1998031496062994683, -1.154855643044619518 ) ) ;
#43405=CARTESIAN_POINT ( 'NONE',  ( -0.3392501089628017219, -0.1958661417322836718, -2.249343832020997525 ) ) ;
#43409=CARTESIAN_POINT ( 'NONE',  ( -1.157146581871515012E-16, 0.4724409448818898682, -0.1574803149606299191 ) ) ;
#43410=CARTESIAN_POINT ( 'NONE',  ( 0.2891555358219910499, 0.2891555358219910499, -2.814960629921259727 ) ) ;
#43414=CARTESIAN_POINT ( 'NONE',  ( -0.1958661417322834220, -0.3392501089628018884, -1.475065616797900381 ) ) ;
#43416=CARTESIAN_POINT ( 'NONE',  ( 0.4724409448818898682, 2.892866454678787531E-17, -2.322834645669291209 ) ) ;
#43418=ADVANCED_FACE ( 'NONE', ( #18268 ), #38434, .T. ) ;
#43423=CARTESIAN_POINT ( 'NONE',  ( 0.1958661417322836162, -0.3392501089628018329, -0.8018179545593683288 ) ) ;
#43431=CARTESIAN_POINT ( 'NONE',  ( -0.3917322834645670659, -7.196005306013484475E-17, -2.083352649115172373 ) ) ;
#43437=CARTESIAN_POINT ( 'NONE',  ( -0.3392501089628019995, 0.1958661417322832277, -1.213254593175852936 ) ) ;
#43448=CARTESIAN_POINT ( 'NONE',  ( 0.1049643490035304938, -0.3917322834645669549, -2.912073490813647858 ) ) ;
#43449=ORIENTED_EDGE ( 'NONE', *, *, #47486, .F. ) ;
#43455=CARTESIAN_POINT ( 'NONE',  ( 0.2867679344610365999, -0.2867679344610365444, -1.285433070866141669 ) ) ;
#43458=CARTESIAN_POINT ( 'NONE',  ( 0.2925321140481932369, -0.2925321140481931814, -2.694881889763780070 ) ) ;
#43468=CARTESIAN_POINT ( 'NONE',  ( 0.1070741851644054776, -0.3996062992125984925, -0.4770341207349080848 ) ) ;
#43471=CARTESIAN_POINT ( 'NONE',  ( -0.1049643490035302024, -0.3917322834645671215, -0.06430446194225715451 ) ) ;
#43486=CARTESIAN_POINT ( 'NONE',  ( 0.1958661417322836718, -0.3392501089628017219, -0.7185232527897132959 ) ) ;
#43488=( BOUNDED_CURVE ( )  B_SPLINE_CURVE ( 2, ( #31197, #50545, #76249 ),
 .UNSPECIFIED., .F., .F. ) 
 B_SPLINE_CURVE_WITH_KNOTS ( ( 3, 3 ),
 ( 0.4625000000000001332, 0.4631378855240345094 ),
 .UNSPECIFIED. ) 
 CURVE ( )  GEOMETRIC_REPRESENTATION_ITEM ( )  RATIONAL_B_SPLINE_CURVE ( ( 0.9999999999999991118, 0.9947834986831257664, 0.9911642120907997455 ) ) 
 REPRESENTATION_ITEM ( '' )  );
#43491=CARTESIAN_POINT ( 'NONE',  ( 0.4724409448818897572, -0.1265901696524988906, -1.920603674540682038 ) ) ;
#43510=CARTESIAN_POINT ( 'NONE',  ( 0.3460692066303958092, 0.1998031496062993018, -2.570209973753280863 ) ) ;
#43516=CARTESIAN_POINT ( 'NONE',  ( -0.2925321140481930704, -0.2925321140481933480, -2.106299212598425452 ) ) ;
#43517=CARTESIAN_POINT ( 'NONE',  ( -0.3949938075777409963, -7.255918531996591613E-17, -1.614173228346456934 ) ) ;
#43518=CARTESIAN_POINT ( 'NONE',  ( 0.1998031496062992740, 0.3460692066303959757, -2.821522309711286258 ) ) ;
#43521=CARTESIAN_POINT ( 'NONE',  ( -0.3917322834645671215, 0.1049643490035301469, -0.8123359580052490481 ) ) ;
#43526=CARTESIAN_POINT ( 'NONE',  ( -0.3949938075777409963, -7.255918531996591613E-17, -2.635826771653543954 ) ) ;
#43530=CARTESIAN_POINT ( 'NONE',  ( 0.4724409448818898682, 2.892866454678787531E-17, -2.795275590551181022 ) ) ;
#43531=CARTESIAN_POINT ( 'NONE',  ( 0.2925321140481932369, 0.2925321140481932369, -2.027559055118109743 ) ) ;
#43539=CARTESIAN_POINT ( 'NONE',  ( 0.3917322834645670104, 2.398668435337828261E-17, -0.2027559055118111353 ) ) ;
#43546=CARTESIAN_POINT ( 'NONE',  ( -0.1049643490035307020, 0.3917322834645669549, -0.4061679790026246351 ) ) ;
#43547=CARTESIAN_POINT ( 'NONE',  ( 0.3917322834645670104, -0.1049643490035303411, -1.363517060367453793 ) ) ;
#43548=CARTESIAN_POINT ( 'NONE',  ( 0.1958661417322834775, 0.3392501089628018884, -2.813648293963254776 ) ) ;
#43551=CARTESIAN_POINT ( 'NONE',  ( -0.3949938075777409408, -0.1058382717557502933, -2.880577427821522374 ) ) ;
#43555=CARTESIAN_POINT ( 'NONE',  ( 0.1070741851644053527, 0.3996062992125986590, -1.253280839895013044 ) ) ;
#43556=CARTESIAN_POINT ( 'NONE',  ( 0.000000000000000000, 0.000000000000000000, -2.755905511811024056 ) ) ;
#43560=CARTESIAN_POINT ( 'NONE',  ( 0.2867679344610365999, 0.2867679344610365999, -0.5374015748031496509 ) ) ;
#43569=CARTESIAN_POINT ( 'NONE',  ( 0.4724409448818896462, 0.1265901696524990294, -2.171916010498687211 ) ) ;
#43579=CARTESIAN_POINT ( 'NONE',  ( -0.3392501089628018329, -0.1958661417322836440, -0.2900069309373210502 ) ) ;
#43581=CARTESIAN_POINT ( 'NONE',  ( -0.1049643490035301885, -0.3917322834645671215, -0.7867454068241470644 ) ) ;
#43587=CARTESIAN_POINT ( 'NONE',  ( 4.797336870675656522E-17, -0.3917322834645670104, -2.590551181102362044 ) ) ;
#43590=CARTESIAN_POINT ( 'NONE',  ( 0.1265901696524990294, -0.4724409448818896462, -0.9494750656167976199 ) ) ;
#43602=CARTESIAN_POINT ( 'NONE',  ( 0.3460692066303958092, 0.1998031496062993018, -2.097769028871391050 ) ) ;
#43610=CARTESIAN_POINT ( 'NONE',  ( 0.2925321140481931814, 0.2925321140481931814, -0.5295275590551181688 ) ) ;
#43612=CARTESIAN_POINT ( 'NONE',  ( -0.1070741851644056997, 0.3996062992125986035, -0.9514435695538056015 ) ) ;
#43613=CARTESIAN_POINT ( 'NONE',  ( 0.1058382717557500713, -0.3949938075777409408, -0.4002624671916010235 ) ) ;
#43619=CARTESIAN_POINT ( 'NONE',  ( 0.3949938075777408852, 0.1058382717557500435, -1.461286089238844843 ) ) ;
#43624=CARTESIAN_POINT ( 'NONE',  ( 0.3458507752293908943, -0.3458507752293908943, -1.043307086614173151 ) ) ;
#43637=CARTESIAN_POINT ( 'NONE',  ( -0.3392501089628017219, -0.1958661417322836718, -0.9895013123359579499 ) ) ;
#43640=CARTESIAN_POINT ( 'NONE',  ( -0.3949938075777409963, -7.255918531996591613E-17, -1.299212598425196985 ) ) ;
#43645=CARTESIAN_POINT ( 'NONE',  ( 0.1998031496062994405, -0.3460692066303958092, -0.2493438320209973857 ) ) ;
#43653=CARTESIAN_POINT ( 'NONE',  ( -0.1049643490035302024, -0.3917322834645671215, -0.1568241469816273603 ) ) ;
#43658=ORIENTED_EDGE ( 'NONE', *, *, #67228, .F. ) ;
#43659=CARTESIAN_POINT ( 'NONE',  ( -0.1070741851644056997, 0.3996062992125986035, -2.211286089238845065 ) ) ;
#43662=CARTESIAN_POINT ( 'NONE',  ( 0.3996062992125986035, -0.1070741851644052972, -1.763123359580051952 ) ) ;
#43666=CARTESIAN_POINT ( 'NONE',  ( 0.1265901696524990294, -0.4724409448818896462, -0.4002624671916010235 ) ) ;
#43668=CARTESIAN_POINT ( 'NONE',  ( -0.1958661417322836718, 0.3392501089628017219, -0.005249343832020950465 ) ) ;
#43674=CARTESIAN_POINT ( 'NONE',  ( -0.3458507752293909498, 0.3458507752293907833, -2.143700787401574548 ) ) ;
#43676=CARTESIAN_POINT ( 'NONE',  ( 4.837279021331061486E-17, -0.3949938075777409963, -2.360236220472441193 ) ) ;
#43687=CARTESIAN_POINT ( 'NONE',  ( -0.2362204724409451284, 0.4091458600556402425, -1.034776902887139194 ) ) ;
#43697=CARTESIAN_POINT ( 'NONE',  ( -0.2925321140481930149, -0.2925321140481933480, -0.6082677165354329896 ) ) ;
#43699=CARTESIAN_POINT ( 'NONE',  ( 0.1049643490035303689, 0.3917322834645670104, -2.282808398950130879 ) ) ;
#43716=CARTESIAN_POINT ( 'NONE',  ( 0.3917322834645670104, -0.1049643490035303411, -1.456036745406824151 ) ) ;
#43717=CARTESIAN_POINT ( 'NONE',  ( 0.06912221444360695799, 0.3857315817373091482, -1.220472440944881498 ) ) ;
#43721=CARTESIAN_POINT ( 'NONE',  ( 0.2925321140481931814, 0.2925321140481931814, -2.576771653543307394 ) ) ;
#43723=CARTESIAN_POINT ( 'NONE',  ( 0.3460692066303959202, 0.1998031496062993295, -1.076115485564304475 ) ) ;
#43725=CARTESIAN_POINT ( 'NONE',  ( 0.1958661417322836440, -0.3392501089628017219, -2.446194225721784576 ) ) ;
#43737=CARTESIAN_POINT ( 'NONE',  ( -0.3392501089628017219, -0.1958661417322836718, -2.814304461942257252 ) ) ;
#43740=CARTESIAN_POINT ( 'NONE',  ( -0.2891555358219908833, -0.2891555358219912164, -0.2165354330708662567 ) ) ;
#43747=CARTESIAN_POINT ( 'NONE',  ( -0.3917322834645670659, -7.196005306013484475E-17, -1.610911704233282560 ) ) ;
#43749=CARTESIAN_POINT ( 'NONE',  ( -0.3392501089628017219, -0.1958661417322836718, -2.656824146981627166 ) ) ;
#43754=CARTESIAN_POINT ( 'NONE',  ( 0.3996062992125986590, -0.1070741851644053111, -0.7414698162729659314 ) ) ;
#43756=CARTESIAN_POINT ( 'NONE',  ( 0.1998031496062994128, -0.3460692066303957537, -0.4835958005249343938 ) ) ;
#43758=CARTESIAN_POINT ( 'NONE',  ( 0.1998031496062994405, -0.3460692066303958092, -2.139107611548556331 ) ) ;
#43759=CARTESIAN_POINT ( 'NONE',  ( -0.2867679344610364334, -0.2867679344610367109, -1.561023622047243986 ) ) ;
#43764=CARTESIAN_POINT ( 'NONE',  ( -0.2362204724409451284, 0.4091458600556402425, -1.034776902887139194 ) ) ;
#43767=CARTESIAN_POINT ( 'NONE',  ( 0.2891555358219910499, -0.2891555358219909944, -1.120078740157480324 ) ) ;
#43773=DIRECTION ( 'NONE',  ( 0.000000000000000000, 0.000000000000000000, 1.000000000000000000 ) ) ;
#43780=CARTESIAN_POINT ( 'NONE',  ( 0.2925321140481932369, 0.2925321140481932369, -1.631889763779527325 ) ) ;
#43795=CARTESIAN_POINT ( 'NONE',  ( -0.3917322834645669549, -0.1049643490035306603, -1.075459317585301777 ) ) ;
#43814=CARTESIAN_POINT ( 'NONE',  ( -0.1958661417322836718, 0.3392501089628017219, -2.209973753280840114 ) ) ;
#43818=CARTESIAN_POINT ( 'NONE',  ( 5.785732909357575061E-17, -0.4724409448818898682, -0.5511811023622047445 ) ) ;
#43819=CARTESIAN_POINT ( 'NONE',  ( -0.3949938075777409963, -7.255918531996591613E-17, -2.874015748031495843 ) ) ;
#43822=CARTESIAN_POINT ( 'NONE',  ( -0.1049643490035307020, 0.3917322834645669549, -1.416010498687664043 ) ) ;
#43824=CARTESIAN_POINT ( 'NONE',  ( 0.3458507752293908943, 0.3458507752293908943, -2.342519685039369914 ) ) ;
#43832=ADVANCED_FACE ( 'NONE', ( #739, #26814 ), #77759, .T. ) ;
#43833=CARTESIAN_POINT ( 'NONE',  ( -0.1049643490035306742, 0.3917322834645668994, -0.8739964322496570626 ) ) ;
#43841=CARTESIAN_POINT ( 'NONE',  ( 0.1049643490035303967, 0.3917322834645670659, -2.194901205545618961 ) ) ;
#43848=CARTESIAN_POINT ( 'NONE',  ( 0.1049643490035304938, -0.3917322834645669549, -1.587270341207349222 ) ) ;
#43857=CARTESIAN_POINT ( 'NONE',  ( -0.1958661417322836718, 0.3392501089628017219, -2.682414698162729483 ) ) ;
#43868=CARTESIAN_POINT ( 'NONE',  ( -9.594673741351313045E-17, 0.3917322834645670104, -1.344488188976378007 ) ) ;
#43871=CARTESIAN_POINT ( 'NONE',  ( -0.3996062992125984925, -0.1070741851644056858, -2.642388451443570041 ) ) ;
#43882=CARTESIAN_POINT ( 'NONE',  ( 4.893765752498283308E-17, -0.3996062992125985480, -0.3129921259842520231 ) ) ;
#43884=CARTESIAN_POINT ( 'NONE',  ( 0.2867679344610365999, -0.2867679344610365444, -0.09055118110236216877 ) ) ;
#43888=DIRECTION ( 'NONE',  ( 0.000000000000000000, 0.000000000000000000, 1.000000000000000000 ) ) ;
#43900=CARTESIAN_POINT ( 'NONE',  ( -0.1049643490035307158, 0.3917322834645670104, -0.9481820454406320042 ) ) ;
#43904=CARTESIAN_POINT ( 'NONE',  ( 0.2362204724409451007, -0.4091458600556402980, -2.530839895013123453 ) ) ;
#43919=ORIENTED_EDGE ( 'NONE', *, *, #65648, .T. ) ;
#43926=CARTESIAN_POINT ( 'NONE',  ( 0.2925321140481932369, 0.2925321140481932369, -0.1377952755905512139 ) ) ;
#43927=CARTESIAN_POINT ( 'NONE',  ( 0.3460692066303959202, -0.1998031496062991630, -2.701443569553806157 ) ) ;
#43934=CARTESIAN_POINT ( 'NONE',  ( -0.1998031496062991907, -0.3460692066303959757, -2.112860892388451539 ) ) ;
#43935=CARTESIAN_POINT ( 'NONE',  ( -0.3420746716998659953, -0.1974969037888706647, -1.469816272965879245 ) ) ;
#43938=CARTESIAN_POINT ( 'NONE',  ( 0.1049643490035304799, -0.3917322834645669549, -0.7073490813648293241 ) ) ;
#43941=CARTESIAN_POINT ( 'NONE',  ( 4.837279021331061486E-17, -0.3949938075777409963, -2.517716535433071279 ) ) ;
#43945=CARTESIAN_POINT ( 'NONE',  ( 0.3458507752293908943, -0.3458507752293908943, -2.775590551181101429 ) ) ;
#43946=CARTESIAN_POINT ( 'NONE',  ( 0.2925321140481932369, 0.2925321140481932369, -2.342519685039369914 ) ) ;
#43952=CARTESIAN_POINT ( 'NONE',  ( -9.594673741351313045E-17, 0.3917322834645670104, -0.08464566929133868212 ) ) ;
#43959=CARTESIAN_POINT ( 'NONE',  ( -0.3392501089628017219, -0.1958661417322836718, -0.6095800524934383846 ) ) ;
#43960=CARTESIAN_POINT ( 'NONE',  ( 4.797336870675656522E-17, -0.3917322834645670104, -1.645669291338582640 ) ) ;
#43961=CARTESIAN_POINT ( 'NONE',  ( 4.797336870675656522E-17, -0.3917322834645670104, -2.905511811023621771 ) ) ;
#43964=CARTESIAN_POINT ( 'NONE',  ( 0.3949938075777409963, 2.418639510665530435E-17, -2.637795275590551380 ) ) ;
#43968=CARTESIAN_POINT ( 'NONE',  ( -0.1070741851644051862, -0.3996062992125987146, -1.489501312335957950 ) ) ;
#43973=CARTESIAN_POINT ( 'NONE',  ( -0.2867679344610364334, -0.2867679344610367109, -0.6161417322834646937 ) ) ;
#43983=CARTESIAN_POINT ( 'NONE',  ( -0.2362204724409451284, 0.4091458600556402425, -2.217847769028871596 ) ) ;
#43992=CARTESIAN_POINT ( 'NONE',  ( -0.4091458600556402980, -0.2362204724409451284, -2.648950131233595684 ) ) ;
#43996=CARTESIAN_POINT ( 'NONE',  ( -0.1049643490035306742, 0.3917322834645668994, -0.2440751724071372475 ) ) ;
#43998=CARTESIAN_POINT ( 'NONE',  ( -0.1958661417322836718, 0.3392501089628017219, -0.8851706036745407014 ) ) ;
#44004=CARTESIAN_POINT ( 'NONE',  ( -0.2867679344610364334, -0.2867679344610367109, -2.885826771653543066 ) ) ;
#44007=CARTESIAN_POINT ( 'NONE',  ( 0.4724409448818896462, 0.1265901696524990294, -0.9888451443569553634 ) ) ;
#44015=CARTESIAN_POINT ( 'NONE',  ( 0.2362204724409449064, 0.4091458600556404646, -0.3018372703412073310 ) ) ;
#44019=EDGE_CURVE ( 'NONE', #78139, #25753, #36645, .T. ) ;
#44020=CARTESIAN_POINT ( 'NONE',  ( -0.2925321140481932369, 0.2925321140481931259, -2.143700787401574548 ) ) ;
#44026=CARTESIAN_POINT ( 'NONE',  ( 0.3458507752293908943, -0.3458507752293908943, -0.09842519685039370636 ) ) ;
#44028=CARTESIAN_POINT ( 'NONE',  ( 0.2925321140481931814, 0.2925321140481931814, -0.8444881889763780070 ) ) ;
#44029=CARTESIAN_POINT ( 'NONE',  ( -0.1998031496062994683, 0.3460692066303958092, -1.115485564304461885 ) ) ;
#44031=CARTESIAN_POINT ( 'NONE',  ( -0.2891555358219908833, -0.2891555358219912164, -0.3740157480314962313 ) ) ;
#44036=CARTESIAN_POINT ( 'NONE',  ( 0.3458507752293908943, -0.3458507752293908943, -2.379921259842519898 ) ) ;
#44037=CARTESIAN_POINT ( 'NONE',  ( 0.1974969037888706092, -0.3420746716998660508, -1.113517060367454015 ) ) ;
#44042=CARTESIAN_POINT ( 'NONE',  ( -0.3458507752293909498, 0.3458507752293907833, -1.437007874015747921 ) ) ;
#44056=CARTESIAN_POINT ( 'NONE',  ( -0.3392501089628017219, -0.1958661417322836718, -1.304461942257217899 ) ) ;
#44058=ORIENTED_EDGE ( 'NONE', *, *, #67062, .F. ) ;
#44059=CARTESIAN_POINT ( 'NONE',  ( -0.3949938075777409408, -0.1058382717557502933, -1.305774278215223072 ) ) ;
#44064=CARTESIAN_POINT ( 'NONE',  ( -0.1070741851644051862, -0.3996062992125987146, -0.07217847769028871985 ) ) ;
#44072=CARTESIAN_POINT ( 'NONE',  ( 0.3392501089628018329, 0.1958661417322835607, -0.05839895013123368173 ) ) ;
#44078=CARTESIAN_POINT ( 'NONE',  ( 0.2925321140481932369, -0.2925321140481932369, -2.145669291338581974 ) ) ;
#44081=CARTESIAN_POINT ( 'NONE',  ( 0.1070741851644054776, -0.3996062992125984925, -1.579396325459317296 ) ) ;
#44085=CARTESIAN_POINT ( 'NONE',  ( -0.3458507752293906723, -0.3458507752293910609, -1.003937007874015741 ) ) ;
#44087=CARTESIAN_POINT ( 'NONE',  ( 0.1958661417322834775, 0.3392501089628018884, -2.748687664041994605 ) ) ;
#44089=CARTESIAN_POINT ( 'NONE',  ( 0.2867679344610366554, 0.2867679344610366554, -2.112204724409449064 ) ) ;
#44093=CARTESIAN_POINT ( 'NONE',  ( -0.4091458600556405756, 0.2362204724409446288, -2.622703412073490892 ) ) ;
#44095=ADVANCED_FACE ( 'NONE', ( #74354 ), #36039, .T. ) ;
#44096=CARTESIAN_POINT ( 'NONE',  ( 0.2891555358219910499, -0.2891555358219909944, -2.064960629921260171 ) ) ;
#44101=CARTESIAN_POINT ( 'NONE',  ( -0.1265901696524986964, -0.4724409448818899238, -2.196194225721784576 ) ) ;
#44117=CARTESIAN_POINT ( 'NONE',  ( -0.1070741851644056997, 0.3996062992125984925, -0.5557742782152230721 ) ) ;
#44118=CARTESIAN_POINT ( 'NONE',  ( -0.1958661417322836718, 0.3392501089628017219, -2.302493438320210029 ) ) ;
#44128=CARTESIAN_POINT ( 'NONE',  ( 0.3392501089628018329, 0.1958661417322835607, -2.175216166175539811 ) ) ;
#44134=CARTESIAN_POINT ( 'NONE',  ( -0.1958661417322834220, -0.3392501089628018884, -2.040026246719160330 ) ) ;
#44141=CARTESIAN_POINT ( 'NONE',  ( -0.1070741851644051862, -0.3996062992125987146, -0.8595800524934383846 ) ) ;
#44142=EDGE_LOOP ( 'NONE', ( #12435, #8466, #60350, #43658, #34154, #13273 ) ) ;
#44143=CARTESIAN_POINT ( 'NONE',  ( -9.594673741351313045E-17, 0.3917322834645670104, -2.826771653543306506 ) ) ;
#44155=CARTESIAN_POINT ( 'NONE',  ( 0.1049643490035303689, 0.3917322834645670104, -0.3005249343832020470 ) ) ;
#44158=CARTESIAN_POINT ( 'NONE',  ( 4.837279021331060870E-17, -0.3949938075777409963, -0.3937007874015748810 ) ) ;
#44165=CARTESIAN_POINT ( 'NONE',  ( 0.3917322834645670659, -0.1049643490035303273, -1.840570496884201379 ) ) ;
#44167=CARTESIAN_POINT ( 'NONE',  ( 4.797336870675656522E-17, -0.3917322834645670104, -2.840551181102362044 ) ) ;
#44172=CARTESIAN_POINT ( 'NONE',  ( -0.1070741851644056997, 0.3996062992125986035, -0.9514435695538056015 ) ) ;
#44174=CARTESIAN_POINT ( 'NONE',  ( -0.1070741851644056997, 0.3996062992125984925, -0.3982939632545932085 ) ) ;
#44175=CARTESIAN_POINT ( 'NONE',  ( 0.1998031496062992463, 0.3460692066303959202, -0.06364829396325462352 ) ) ;
#44177=CARTESIAN_POINT ( 'NONE',  ( -0.1998031496062994683, 0.3460692066303958092, -2.847769028871391050 ) ) ;
#44179=CARTESIAN_POINT ( 'NONE',  ( 0.1049643490035304938, -0.3917322834645669549, -1.587270341207349222 ) ) ;
#44183=CARTESIAN_POINT ( 'NONE',  ( -0.2362204724409451284, 0.4091458600556402425, -1.349737532808398921 ) ) ;
#44187=CARTESIAN_POINT ( 'NONE',  ( -0.2891555358219909388, -0.2891555358219912164, -1.080708661417322913 ) ) ;
#44189=CARTESIAN_POINT ( 'NONE',  ( -0.4091458600556402980, -0.2362204724409451284, -1.074146981627296604 ) ) ;
#44197=CARTESIAN_POINT ( 'NONE',  ( 4.893765752498283308E-17, -0.3996062992125985480, -1.887795275590551158 ) ) ;
#44211=CARTESIAN_POINT ( 'NONE',  ( -0.3917322834645671215, 0.1049643490035301469, -1.062335958005249603 ) ) ;
#44230=CARTESIAN_POINT ( 'NONE',  ( -9.594673741351313045E-17, 0.3917322834645670104, -2.196850393700787496 ) ) ;
#44234=CARTESIAN_POINT ( 'NONE',  ( -0.4724409448818899238, 0.1265901696524986686, -0.5052493438320209140 ) ) ;
#44235=CARTESIAN_POINT ( 'NONE',  ( -0.3949938075777409408, -0.1058382717557502933, -2.723097112860892732 ) ) ;
#44238=CARTESIAN_POINT ( 'NONE',  ( -0.3392501089628017219, -0.1958661417322836718, -1.461942257217847763 ) ) ;
#44240=CARTESIAN_POINT ( 'NONE',  ( -0.3458507752293909498, 0.3458507752293907833, -2.854330708661417138 ) ) ;
#44247=CARTESIAN_POINT ( 'NONE',  ( 0.3917322834645668994, 0.1049643490035304522, -0.6771460385488696776 ) ) ;
#44254=CARTESIAN_POINT ( 'NONE',  ( -0.3392501089628017219, -0.1958661417322836995, -2.253956323655855076 ) ) ;
#44261=CARTESIAN_POINT ( 'NONE',  ( -0.1049643490035307020, 0.3917322834645669549, -1.508530183727033736 ) ) ;
#44270=CARTESIAN_POINT ( 'NONE',  ( -0.3392501089628017219, -0.1958661417322836718, -2.879265091863516979 ) ) ;
#44277=CARTESIAN_POINT ( 'NONE',  ( -0.4091458600556402980, -0.2362204724409451284, -0.3674540682414698112 ) ) ;
#44278=CARTESIAN_POINT ( 'NONE',  ( 0.3917322834645669549, 0.1049643490035304660, -1.154199475065616820 ) ) ;
#44279=CARTESIAN_POINT ( 'NONE',  ( -0.2362204724409447953, -0.4091458600556404646, 0.01509186351706036204 ) ) ;
#44282=CARTESIAN_POINT ( 'NONE',  ( -0.1998031496062991630, -0.3460692066303959202, -2.819553805774277944 ) ) ;
#44291=CARTESIAN_POINT ( 'NONE',  ( 0.3996062992125984925, 0.1070741851644054637, -0.6738845144356955252 ) ) ;
#44293=CARTESIAN_POINT ( 'NONE',  ( 4.797336870675656522E-17, -0.3917322834645670104, -0.2283464566929133410 ) ) ;
#44308=CARTESIAN_POINT ( 'NONE',  ( 4.797336870675656522E-17, -0.3917322834645670659, -0.8628802081702905413 ) ) ;
#44312=CARTESIAN_POINT ( 'NONE',  ( -0.4091458600556405756, 0.2362204724409446288, -2.465223097112860806 ) ) ;
#44331=CARTESIAN_POINT ( 'NONE',  ( 0.1998031496062994405, -0.3460692066303958092, -0.4068241469816273326 ) ) ;
#44332=CARTESIAN_POINT ( 'NONE',  ( 0.1998031496062992463, 0.3460692066303959202, -2.583333333333333481 ) ) ;
#44337=CARTESIAN_POINT ( 'NONE',  ( -0.3460692066303960868, 0.1998031496062990242, -2.073490813648294129 ) ) ;
#44338=CARTESIAN_POINT ( 'NONE',  ( 0.3420746716998659953, 0.1974969037888705536, -1.391076115485564424 ) ) ;
#44339=CARTESIAN_POINT ( 'NONE',  ( 0.1070741851644054915, -0.3996062992125986035, -2.762467191601049255 ) ) ;
#44341=CARTESIAN_POINT ( 'NONE',  ( 0.1958661417322836440, -0.3392501089628017219, -0.7139107611548556331 ) ) ;
#44344=CARTESIAN_POINT ( 'NONE',  ( 0.2891555358219910499, -0.2891555358219909944, -2.379921259842519898 ) ) ;
#44348=CARTESIAN_POINT ( 'NONE',  ( 0.4724409448818898682, 2.892866454678787531E-17, -0.03740157480314962313 ) ) ;
#44349=CARTESIAN_POINT ( 'NONE',  ( 0.1070741851644054915, -0.3996062992125986035, -2.132545931758530244 ) ) ;
#44355=CARTESIAN_POINT ( 'NONE',  ( 0.3917322834645670104, -0.1049643490035303411, -0.1961942257217848817 ) ) ;
#44362=CARTESIAN_POINT ( 'NONE',  ( 0.1958661417322836440, -0.3392501089628017219, -0.4914698162729659869 ) ) ;
#44363=CARTESIAN_POINT ( 'NONE',  ( 0.2867679344610365999, -0.2867679344610365444, -1.350393700787401619 ) ) ;
#44364=CARTESIAN_POINT ( 'NONE',  ( 0.3917322834645670104, 2.398668435337828261E-17, -2.787401574803149096 ) ) ;
#44366=CARTESIAN_POINT ( 'NONE',  ( -0.1070741851644051862, -0.3996062992125987146, 0.08530183727034119923 ) ) ;
#44370=CARTESIAN_POINT ( 'NONE',  ( 0.2925321140481932369, 0.2925321140481932369, -1.555118110236220597 ) ) ;
#44375=CARTESIAN_POINT ( 'NONE',  ( -0.3917322834645671215, 0.1049643490035301469, -0.7473753280839893209 ) ) ;
#44383=CARTESIAN_POINT ( 'NONE',  ( -0.3458507752293906723, -0.3458507752293910609, -2.106299212598425452 ) ) ;
#44391=CARTESIAN_POINT ( 'NONE',  ( -0.4724409448818898682, -8.678599364036362592E-17, -2.635826771653543066 ) ) ;
#44395=CARTESIAN_POINT ( 'NONE',  ( 0.3392501089628018329, -0.1958661417322834497, -0.4999806842181608868 ) ) ;
#44397=CARTESIAN_POINT ( 'NONE',  ( -9.594673741351313045E-17, 0.3917322834645670104, -0.8720472440944883052 ) ) ;
#44402=CARTESIAN_POINT ( 'NONE',  ( -0.1049643490035307158, 0.3917322834645670104, 0.1541801592837776513 ) ) ;
#44405=CARTESIAN_POINT ( 'NONE',  ( -0.4724409448818898682, -8.678599364036362592E-17, -1.061023622047243986 ) ) ;
#44412=DIRECTION ( 'NONE',  ( 1.000000000000000000, 0.000000000000000000, 0.000000000000000000 ) ) ;
#44417=CARTESIAN_POINT ( 'NONE',  ( 0.3996062992125985480, 2.446882876249141654E-17, -2.242125984251968518 ) ) ;
#44421=CARTESIAN_POINT ( 'NONE',  ( -0.1070741851644051862, -0.3996062992125986590, -1.251312335958005395 ) ) ;
#44428=CARTESIAN_POINT ( 'NONE',  ( 0.3996062992125985480, -0.1070741851644052972, -0.5032808398950130435 ) ) ;
#44429=CARTESIAN_POINT ( 'NONE',  ( -0.3996062992125986035, -0.1070741851644056997, -1.148293963254592986 ) ) ;
#44430=CARTESIAN_POINT ( 'NONE',  ( 0.2891555358219910499, 0.2891555358219910499, -0.1377952755905512694 ) ) ;
#44431=CARTESIAN_POINT ( 'NONE',  ( 0.3726288332213487653, 0.1208384647389236927, -1.220472440944882164 ) ) ;
#44437=CARTESIAN_POINT ( 'NONE',  ( -0.2891555358219911054, 0.2891555358219909388, -1.513779527559055094 ) ) ;
#44442=CARTESIAN_POINT ( 'NONE',  ( -0.4091458600556405756, 0.2362204724409446288, -1.601049868766404094 ) ) ;
#44443=CARTESIAN_POINT ( 'NONE',  ( -0.2925321140481930704, -0.2925321140481933480, -2.736220472440943574 ) ) ;
#44451=CARTESIAN_POINT ( 'NONE',  ( 4.797336870675655290E-17, -0.3917322834645669549, -2.048537114664355396 ) ) ;
#44459=CARTESIAN_POINT ( 'NONE',  ( -9.594673741351313045E-17, 0.3917322834645670104, -1.409448818897637734 ) ) ;
#44462=CARTESIAN_POINT ( 'NONE',  ( 0.2891555358219910499, 0.2891555358219910499, -1.870078740157480324 ) ) ;
#44467=CARTESIAN_POINT ( 'NONE',  ( -9.787531504996567848E-17, 0.3996062992125986035, -0.3149606299212598381 ) ) ;
#44474=CARTESIAN_POINT ( 'NONE',  ( -0.2867679344610365999, 0.2867679344610364889, 0.05314960629921249707 ) ) ;
#44481=CARTESIAN_POINT ( 'NONE',  ( 0.3460692066303959202, -0.1998031496062991630, -1.599081364829396223 ) ) ;
#44486=CARTESIAN_POINT ( 'NONE',  ( 0.2362204724409449064, 0.4091458600556404646, -0.7742782152230971437 ) ) ;
#44489=CARTESIAN_POINT ( 'NONE',  ( 0.2867679344610365999, 0.2867679344610365999, 0.02755905511811028441 ) ) ;
#44495=CARTESIAN_POINT ( 'NONE',  ( 0.1265901696524989462, 0.4724409448818897572, -2.747375328083988766 ) ) ;
#44499=CARTESIAN_POINT ( 'NONE',  ( 0.3420746716998660508, -0.1974969037888704149, -2.071522309711286258 ) ) ;
#44510=CARTESIAN_POINT ( 'NONE',  ( -0.2362204724409451284, 0.4091458600556402425, 0.2250656167979002698 ) ) ;
#44522=CARTESIAN_POINT ( 'NONE',  ( 0.3996062992125986035, -0.1070741851644052972, -1.133202099737532720 ) ) ;
#44523=CARTESIAN_POINT ( 'NONE',  ( 0.3917322834645670104, -0.1049643490035303411, -2.243438320209974357 ) ) ;
#44533=CARTESIAN_POINT ( 'NONE',  ( 0.1958661417322836718, -0.3392501089628017219, -2.293326402396012487 ) ) ;
#44539=CARTESIAN_POINT ( 'NONE',  ( 0.3392501089628018884, -0.1958661417322834220, -1.921916010498687877 ) ) ;
#44547=CARTESIAN_POINT ( 'NONE',  ( -0.3996062992125987146, 0.1070741851644051862, -1.135170603674540590 ) ) ;
#44549=CARTESIAN_POINT ( 'NONE',  ( 0.2867679344610366554, 0.2867679344610366554, 0.02294656348325270490 ) ) ;
#44562=CARTESIAN_POINT ( 'NONE',  ( 0.3392501089628018329, 0.1958661417322835607, -0.1233595800524933811 ) ) ;
#44565=CARTESIAN_POINT ( 'NONE',  ( 0.2891555358219910499, -0.2891555358219909944, -0.09842519685039378963 ) ) ;
#44572=CARTESIAN_POINT ( 'NONE',  ( -0.1049643490035302301, -0.3917322834645671770, -1.486239788222784020 ) ) ;
#44574=CARTESIAN_POINT ( 'NONE',  ( -0.3917322834645670104, -7.196005306013484475E-17, -2.801181102362204633 ) ) ;
#44578=CARTESIAN_POINT ( 'NONE',  ( -9.787531504996567848E-17, 0.3996062992125986035, -0.9448818897637796255 ) ) ;
#44580=CARTESIAN_POINT ( 'NONE',  ( 0.1070741851644053388, 0.3996062992125986035, -0.2276902887139107545 ) ) ;
#44581=CARTESIAN_POINT ( 'NONE',  ( 0.3460692066303958092, 0.1998031496062993018, -0.2080052493438320771 ) ) ;
#44583=CARTESIAN_POINT ( 'NONE',  ( -0.3996062992125987146, 0.1070741851644051862, -2.552493438320210029 ) ) ;
#44584=CARTESIAN_POINT ( 'NONE',  ( 0.3917322834645669549, 0.1049643490035304660, -1.626640419947506411 ) ) ;
#44589=CARTESIAN_POINT ( 'NONE',  ( -0.4724409448818899238, 0.1265901696524986686, -1.526902887139107490 ) ) ;
#44592=CARTESIAN_POINT ( 'NONE',  ( -0.3949938075777411073, 0.1058382717557497660, -1.054461942257217899 ) ) ;
#44601=CARTESIAN_POINT ( 'NONE',  ( 0.3996062992125985480, 2.446882876249141654E-17, -2.084645669291338876 ) ) ;
#44603=CARTESIAN_POINT ( 'NONE',  ( -0.3917322834645670659, 0.1049643490035301607, -1.687644726212911506 ) ) ;
#44617=CARTESIAN_POINT ( 'NONE',  ( 4.797336870675656522E-17, -0.3917322834645670104, -1.108267716535433101 ) ) ;
#44636=CARTESIAN_POINT ( 'NONE',  ( 0.1049643490035304799, -0.3917322834645669549, -2.124671916010498762 ) ) ;
#44640=CARTESIAN_POINT ( 'NONE',  ( 0.1265901696524990294, -0.4724409448818896462, -0.4002624671916010235 ) ) ;
#44642=CARTESIAN_POINT ( 'NONE',  ( 0.2925321140481932369, -0.2925321140481932369, -0.2559055118110236116 ) ) ;
#44645=CARTESIAN_POINT ( 'NONE',  ( 4.797336870675656522E-17, -0.3917322834645670104, -1.960629921259842368 ) ) ;
#44647=CARTESIAN_POINT ( 'NONE',  ( -0.4091458600556405756, 0.2362204724409446288, -2.703412073490813583 ) ) ;
#44654=CARTESIAN_POINT ( 'NONE',  ( 0.3917322834645669549, 2.398668435337827645E-17, -0.8280646737194732321 ) ) ;
#44661=CARTESIAN_POINT ( 'NONE',  ( -0.3917322834645671770, 0.1049643490035302024, -2.076790969325146730 ) ) ;
#44669=CARTESIAN_POINT ( 'NONE',  ( -0.3917322834645669549, -0.1049643490035306603, -1.232939632545931863 ) ) ;
#44683=CARTESIAN_POINT ( 'NONE',  ( -0.4724409448818898682, -8.678599364036362592E-17, -0.3543307086614173040 ) ) ;
#44684=CARTESIAN_POINT ( 'NONE',  ( 0.3917322834645670104, -0.1049643490035303411, -1.298556430446194510 ) ) ;
#44685=CARTESIAN_POINT ( 'NONE',  ( -1.157146581871515012E-16, 0.4724409448818898682, -0.3917322834645669549 ) ) ;
#44688=CARTESIAN_POINT ( 'NONE',  ( -0.1974969037888704149, -0.3420746716998661063, 0.1725721784776902690 ) ) ;
#44693=CARTESIAN_POINT ( 'NONE',  ( 0.3949938075777408852, 0.1058382717557500435, -0.2014435695538058235 ) ) ;
#44697=CARTESIAN_POINT ( 'NONE',  ( -0.1265901696524993347, 0.4724409448818896462, -0.9514435695538056015 ) ) ;
#44700=CARTESIAN_POINT ( 'NONE',  ( 0.1998031496062994128, -0.3460692066303957537, -1.113517060367454015 ) ) ;
#44702=( BOUNDED_CURVE ( )  B_SPLINE_CURVE ( 2, ( #33293, #893, #32436, #6764, #82552, #26550, #52203, #24870, #50538, #38336, #45, #77062, #34537 ),
 .UNSPECIFIED., .F., .F. ) 
 B_SPLINE_CURVE_WITH_KNOTS ( ( 3, 2, 2, 2, 2, 2, 3 ),
 ( 0.8625000000000000444, 0.8666666666666666963, 0.8708333333333333481, 0.8750000000000001110, 0.8791666666666667629, 0.8833333333333334147, 0.8875000000000000666 ),
 .UNSPECIFIED. ) 
 CURVE ( )  GEOMETRIC_REPRESENTATION_ITEM ( )  RATIONAL_B_SPLINE_CURVE ( ( 1.000000000000000000, 0.9659258262890683122, 1.000000000000000000, 0.9659258262890683122, 1.000000000000000000, 0.9659258262890683122, 1.000000000000000000, 0.9659258262890683122, 1.000000000000000000, 0.9659258262890683122, 1.000000000000000000, 0.9659258262890674240, 1.000000000000000888 ) ) 
 REPRESENTATION_ITEM ( '' )  );
#44703=CARTESIAN_POINT ( 'NONE',  ( -0.3917322834645670104, -7.196005306013484475E-17, -0.1889763779527558474 ) ) ;
#44705=CYLINDRICAL_SURFACE ( 'NONE', #82878, 0.4724409448818898682 ) ;
#44716=CARTESIAN_POINT ( 'NONE',  ( -0.1958661417322833942, -0.3392501089628018884, -0.8497568485902381452 ) ) ;
#44720=CARTESIAN_POINT ( 'NONE',  ( -0.4091458600556405756, 0.2362204724409446288, -2.622703412073490892 ) ) ;
#44739=CARTESIAN_POINT ( 'NONE',  ( -0.2925321140481930704, -0.2925321140481933480, -0.3740157480314960092 ) ) ;
#44740=CARTESIAN_POINT ( 'NONE',  ( -0.2925321140481932369, 0.2925321140481931259, -2.773622047244094002 ) ) ;
#44745=CARTESIAN_POINT ( 'NONE',  ( -0.1070741851644051862, -0.3996062992125987146, -2.119422572178477626 ) ) ;
#44746=CARTESIAN_POINT ( 'NONE',  ( -0.3420746716998659953, -0.1974969037888706647, -1.627296587926509330 ) ) ;
#44747=CARTESIAN_POINT ( 'NONE',  ( -0.3996062992125987146, 0.1070741851644051862, -2.709973753280840114 ) ) ;
#44749=CARTESIAN_POINT ( 'NONE',  ( -0.3917322834645669549, -0.1049643490035306603, -1.140419947506561504 ) ) ;
#44752=CARTESIAN_POINT ( 'NONE',  ( -0.1974969037888704149, -0.3420746716998661063, -2.504593175853018661 ) ) ;
#44756=CARTESIAN_POINT ( 'NONE',  ( 0.4724409448818897572, -0.1265901696524988906, -2.946194225721785465 ) ) ;
#44757=CARTESIAN_POINT ( 'NONE',  ( 0.3996062992125986590, -0.1070741851644053111, -2.158792650918635037 ) ) ;
#44758=CARTESIAN_POINT ( 'NONE',  ( 0.2867679344610366554, -0.2867679344610365999, -0.7250849325797394940 ) ) ;
#44764=CARTESIAN_POINT ( 'NONE',  ( 0.1049643490035303689, 0.3917322834645670104, -0.2355643044619422921 ) ) ;
#44772=CARTESIAN_POINT ( 'NONE',  ( 0.3917322834645669549, 0.1049643490035304660, -0.6817585301837268963 ) ) ;
#44773=CARTESIAN_POINT ( 'NONE',  ( -0.1958661417322834220, -0.3392501089628018884, -1.475065616797900381 ) ) ;
#44774=CARTESIAN_POINT ( 'NONE',  ( 0.1958661417322836440, -0.3392501089628017219, -2.761154855643044304 ) ) ;
#44776=CARTESIAN_POINT ( 'NONE',  ( 0.1998031496062994405, -0.3460692066303958092, -0.09186351706036746667 ) ) ;
#44780=CARTESIAN_POINT ( 'NONE',  ( -0.1070741851644056997, 0.3996062992125986035, -1.423884514435695525 ) ) ;
#44784=CARTESIAN_POINT ( 'NONE',  ( 0.3928700489057012635, -0.01966910102760525275, -1.929133858267715329 ) ) ;
#44785=CARTESIAN_POINT ( 'NONE',  ( -0.3917322834645669549, -0.1049643490035306603, -0.9179790026246721357 ) ) ;
#44795=CARTESIAN_POINT ( 'NONE',  ( 0.4724409448818897572, -0.1265901696524988906, -2.158792650918635037 ) ) ;
#44802=CARTESIAN_POINT ( 'NONE',  ( 5.785732909357575061E-17, -0.4724409448818898682, -2.517716535433071279 ) ) ;
#44803=CARTESIAN_POINT ( 'NONE',  ( 0.1265901696524990572, -0.4724409448818897017, -2.681758530183727451 ) ) ;
#44806=CARTESIAN_POINT ( 'NONE',  ( 0.3917322834645669549, 2.398668435337827645E-17, -0.6705843587588433685 ) ) ;
#44808=CARTESIAN_POINT ( 'NONE',  ( 0.3392501089628018884, -0.1958661417322834220, -0.8195538057742782767 ) ) ;
#44813=CARTESIAN_POINT ( 'NONE',  ( -0.3917322834645670104, -7.196005306013484475E-17, -2.708661417322834275 ) ) ;
#44816=CARTESIAN_POINT ( 'NONE',  ( -1.157146581871515012E-16, 0.4724409448818898682, -1.179133858267716661 ) ) ;
#44829=CARTESIAN_POINT ( 'NONE',  ( -9.787531504996566615E-17, 0.3996062992125985480, -2.438976377952756014 ) ) ;
#44833=CARTESIAN_POINT ( 'NONE',  ( 0.1070741851644053388, 0.3996062992125986035, -1.172572178477690352 ) ) ;
#44839=CARTESIAN_POINT ( 'NONE',  ( -9.787531504996566615E-17, 0.3996062992125985480, -0.7066929133858268486 ) ) ;
#44840=CARTESIAN_POINT ( 'NONE',  ( -0.3996062992125986035, -0.1070741851644056997, -0.9908136482939633449 ) ) ;
#44842=CARTESIAN_POINT ( 'NONE',  ( -0.3949938075777411628, 0.1058382717557497937, -0.3477690288713912170 ) ) ;
#44848=CARTESIAN_POINT ( 'NONE',  ( 0.2891555358219910499, -0.2891555358219909944, -1.120078740157480324 ) ) ;
#44853=CARTESIAN_POINT ( 'NONE',  ( 5.785732909357575061E-17, -0.4724409448818898682, -1.653543307086614123 ) ) ;
#44861=CARTESIAN_POINT ( 'NONE',  ( -0.2867679344610366554, 0.2867679344610365444, -2.146962311514748478 ) ) ;
#44869=CARTESIAN_POINT ( 'NONE',  ( -9.594673741351313045E-17, 0.3917322834645670104, -1.566929133858267820 ) ) ;
#44872=CARTESIAN_POINT ( 'NONE',  ( 0.1974969037888704704, 0.3420746716998660508, -1.719160104986876769 ) ) ;
#44877=CARTESIAN_POINT ( 'NONE',  ( -0.3996062992125987146, 0.1070741851644051862, -0.3477690288713909950 ) ) ;
#44881=DIRECTION ( 'NONE',  ( 0.000000000000000000, 0.000000000000000000, 1.000000000000000000 ) ) ;
#44884=CARTESIAN_POINT ( 'NONE',  ( -0.1958661417322836718, 0.3392501089628017219, -0.4127296587926510552 ) ) ;
#44892=CARTESIAN_POINT ( 'NONE',  ( -0.1070741851644056997, 0.3996062992125984925, -1.815616797900262425 ) ) ;
#44897=CARTESIAN_POINT ( 'NONE',  ( 5.785732909357575061E-17, -0.4724409448818898682, -1.023622047244094446 ) ) ;
#44900=CARTESIAN_POINT ( 'NONE',  ( -0.3917322834645669549, -0.1049643490035306603, -0.03805774278215218187 ) ) ;
#44905=CARTESIAN_POINT ( 'NONE',  ( 5.785732909357575061E-17, -0.4724409448818898682, -2.675196850393700920 ) ) ;
#44909=VECTOR ( 'NONE', #26716, 39.37007874015748143 ) ;
#44910=CARTESIAN_POINT ( 'NONE',  ( 4.837279021331061486E-17, -0.3949938075777409963, -2.517716535433071279 ) ) ;
#44918=CARTESIAN_POINT ( 'NONE',  ( 0.2867679344610365999, -0.2867679344610365444, -1.665354330708661124 ) ) ;
#44921=CARTESIAN_POINT ( 'NONE',  ( -0.4724409448818899238, 0.1265901696524986686, 0.04790026246719158304 ) ) ;
#44933=CARTESIAN_POINT ( 'NONE',  ( -0.3996062992125986590, 0.1070741851644051723, -1.211942257217847541 ) ) ;
#44934=CARTESIAN_POINT ( 'NONE',  ( -0.1049643490035302024, -0.3917322834645671215, -2.676509186351705871 ) ) ;
#44945=CARTESIAN_POINT ( 'NONE',  ( -0.3458507752293906723, -0.3458507752293910609, -0.6889763779527556808 ) ) ;
#44946=CARTESIAN_POINT ( 'NONE',  ( -0.3392501089628019995, 0.1958661417322831999, -2.070229289535120198 ) ) ;
#44954=CARTESIAN_POINT ( 'NONE',  ( 0.1049643490035304938, -0.3917322834645669549, -2.059711286089238591 ) ) ;
#44959=CARTESIAN_POINT ( 'NONE',  ( 0.1998031496062992463, 0.3460692066303959202, -2.740813648293963567 ) ) ;
#44961=CARTESIAN_POINT ( 'NONE',  ( -0.3996062992125986035, -0.1070741851644056997, -1.148293963254592986 ) ) ;
#44964=CARTESIAN_POINT ( 'NONE',  ( -0.2867679344610367109, 0.2867679344610365444, -0.01642351525690478181 ) ) ;
#44979=CARTESIAN_POINT ( 'NONE',  ( -0.2867679344610365999, 0.2867679344610364889, -0.3267716535433070613 ) ) ;
#44982=CARTESIAN_POINT ( 'NONE',  ( -0.1058382717557497937, -0.3949938075777411628, -0.7020997375328085210 ) ) ;
#44989=CARTESIAN_POINT ( 'NONE',  ( 4.797336870675656522E-17, -0.3917322834645670659, -1.807762097934070278 ) ) ;
#44995=CARTESIAN_POINT ( 'NONE',  ( 0.3460692066303959757, -0.1998031496062991907, -1.207349081364829324 ) ) ;
#44997=CARTESIAN_POINT ( 'NONE',  ( 0.1070741851644054776, -0.3996062992125984925, -0.7919947506561679784 ) ) ;
#44998=CARTESIAN_POINT ( 'NONE',  ( -0.3460692066303960313, 0.1998031496062989965, -0.2604986876640419946 ) ) ;
#45000=CARTESIAN_POINT ( 'NONE',  ( 0.3996062992125986590, -0.1070741851644053111, -2.631233595800525293 ) ) ;
#45001=CARTESIAN_POINT ( 'NONE',  ( -0.1049643490035307020, 0.3917322834645669549, -1.508530183727033736 ) ) ;
#45007=CARTESIAN_POINT ( 'NONE',  ( 0.1265901696524990294, -0.4724409448818896462, -1.421916010498687877 ) ) ;
#45010=CARTESIAN_POINT ( 'NONE',  ( 0.1974969037888704704, 0.3420746716998660508, -1.166010498687664265 ) ) ;
#45020=CARTESIAN_POINT ( 'NONE',  ( 4.893765752498283308E-17, -0.3996062992125985480, -2.045275590551181466 ) ) ;
#45022=CARTESIAN_POINT ( 'NONE',  ( 0.1049643490035303689, 0.3917322834645668994, -1.490794332512124010 ) ) ;
#45036=CARTESIAN_POINT ( 'NONE',  ( 0.1070741851644053388, 0.3996062992125986035, -0.07020997375328083545 ) ) ;
#45038=CARTESIAN_POINT ( 'NONE',  ( -0.3392501089628017219, -0.1958661417322836718, -1.082020997375328086 ) ) ;
#45058=CARTESIAN_POINT ( 'NONE',  ( 0.3917322834645670104, -0.1049643490035303273, -2.308398950131233640 ) ) ;
#45061=CARTESIAN_POINT ( 'NONE',  ( 0.1265901696524989462, 0.4724409448818897572, -0.6233595800524933672 ) ) ;
#45062=CARTESIAN_POINT ( 'NONE',  ( 4.893765752498283924E-17, -0.3996062992125986035, 0.07874015748031494566 ) ) ;
#45065=CARTESIAN_POINT ( 'NONE',  ( 0.1049643490035304938, -0.3917322834645669549, -1.652230971128608505 ) ) ;
#45069=CARTESIAN_POINT ( 'NONE',  ( 0.3458507752293908943, -0.3458507752293908943, -2.775590551181101429 ) ) ;
#45076=CARTESIAN_POINT ( 'NONE',  ( -0.3392501089628018329, -0.1958661417322836440, -1.077408505740470535 ) ) ;
#45082=CARTESIAN_POINT ( 'NONE',  ( -9.594673741351313045E-17, 0.3917322834645670659, -2.516423515256904331 ) ) ;
#45090=CARTESIAN_POINT ( 'NONE',  ( 0.1958661417322834775, 0.3392501089628018884, -1.488845144356955252 ) ) ;
#45105=CARTESIAN_POINT ( 'NONE',  ( -0.1265901696524986964, -0.4724409448818899238, -0.3871391076115485719 ) ) ;
#45106=CARTESIAN_POINT ( 'NONE',  ( -0.3917322834645671215, 0.1049643490035301469, -1.062335958005249603 ) ) ;
#45107=CARTESIAN_POINT ( 'NONE',  ( -0.4724409448818899238, 0.1265901696524986686, -0.1095800524934383152 ) ) ;
#45110=CARTESIAN_POINT ( 'NONE',  ( 0.3996062992125985480, 2.446882876249141654E-17, -2.714566929133858331 ) ) ;
#45115=CARTESIAN_POINT ( 'NONE',  ( 4.837279021331061486E-17, -0.3949938075777409963, 0.001968503937007861845 ) ) ;
#45122=CARTESIAN_POINT ( 'NONE',  ( -0.3996062992125985480, -7.340648628747423112E-17, -0.7460629921259841479 ) ) ;
#45124=CARTESIAN_POINT ( 'NONE',  ( -0.1958661417322836718, 0.3392501089628017219, -0.6351706036745405903 ) ) ;
#45143=CARTESIAN_POINT ( 'NONE',  ( 0.4724409448818897572, -0.1265901696524988906, -2.550524934383202158 ) ) ;
#45148=CARTESIAN_POINT ( 'NONE',  ( 0.000000000000000000, 0.000000000000000000, -2.755905511811024056 ) ) ;
#45160=CARTESIAN_POINT ( 'NONE',  ( 0.2925321140481932369, -0.2925321140481931814, -0.2559055118110236116 ) ) ;
#45161=CARTESIAN_POINT ( 'NONE',  ( 0.2362204724409449064, 0.4091458600556404646, -1.166010498687663821 ) ) ;
#45166=CARTESIAN_POINT ( 'NONE',  ( -0.1070741851644056997, 0.3996062992125986035, -2.368766404199475151 ) ) ;
#45167=CARTESIAN_POINT ( 'NONE',  ( 0.1058382717557500713, -0.3949938075777409408, -1.817585301837270739 ) ) ;
#45168=CARTESIAN_POINT ( 'NONE',  ( -0.1958661417322834220, -0.3392501089628018884, -0.3727034120734908362 ) ) ;
#45170=CARTESIAN_POINT ( 'NONE',  ( -0.3917322834645669549, -0.1049643490035306603, -0.8254593175853016662 ) ) ;
#45173=CARTESIAN_POINT ( 'NONE',  ( -0.2891555358219909388, -0.2891555358219912164, -2.498031496062992574 ) ) ;
#45177=CARTESIAN_POINT ( 'NONE',  ( -0.3458507752293906723, -0.3458507752293910609, -2.893700787401574992 ) ) ;
#45179=CARTESIAN_POINT ( 'NONE',  ( 4.893765752498283924E-17, -0.3996062992125986035, -2.440944881889763884 ) ) ;
#45180=CARTESIAN_POINT ( 'NONE',  ( -0.1958661417322836995, 0.3392501089628017219, -0.7972634102700281167 ) ) ;
#45181=DIRECTION ( 'NONE',  ( 1.000000000000000000, 0.000000000000000000, 0.000000000000000000 ) ) ;
#45188=CARTESIAN_POINT ( 'NONE',  ( 0.1958661417322834775, 0.3392501089628018884, -0.07152230971128617498 ) ) ;
#45196=CARTESIAN_POINT ( 'NONE',  ( 0.3917322834645670104, 2.398668435337828261E-17, -0.6751968503937009203 ) ) ;
#45197=CARTESIAN_POINT ( 'NONE',  ( -0.3917322834645670104, -7.196005306013484475E-17, -1.763779527559055094 ) ) ;
#45199=CARTESIAN_POINT ( 'NONE',  ( -0.3917322834645669549, -0.1049643490035306603, -2.557742782152230721 ) ) ;
#45201=CARTESIAN_POINT ( 'NONE',  ( 0.3996062992125986035, 2.446882876249141962E-17, 0.03937007874015746589 ) ) ;
#45206=CARTESIAN_POINT ( 'NONE',  ( -0.3996062992125986035, -7.340648628747425578E-17, -1.456692913385826849 ) ) ;
#45208=CARTESIAN_POINT ( 'NONE',  ( -0.1265901696524993347, 0.4724409448818896462, -2.445538057742782101 ) ) ;
#45210=CARTESIAN_POINT ( 'NONE',  ( 0.3948371832379764523, 0.006307039255732700168, -1.929133858267718882 ) ) ;
#45211=CARTESIAN_POINT ( 'NONE',  ( 0.3917322834645670104, -0.1049643490035303411, -0.8261154855643043637 ) ) ;
#45217=ORIENTED_EDGE ( 'NONE', *, *, #19165, .F. ) ;
#45220=CARTESIAN_POINT ( 'NONE',  ( 0.2362204724409451007, -0.4091458600556402980, -2.139107611548556331 ) ) ;
#45221=CARTESIAN_POINT ( 'NONE',  ( -0.4724409448818917001, 0.1265901696524956710, -2.709973753280840558 ) ) ;
#45229=CARTESIAN_POINT ( 'NONE',  ( -0.2362204724409447953, -0.4091458600556404646, -2.662073490813648746 ) ) ;
#45232=CARTESIAN_POINT ( 'NONE',  ( 0.3917322834645668994, 0.1049643490035304522, -0.6771460385488696776 ) ) ;
#45241=CARTESIAN_POINT ( 'NONE',  ( 0.1958661417322836440, -0.3392501089628017219, -2.761154855643044304 ) ) ;
#45246=CARTESIAN_POINT ( 'NONE',  ( 0.4091458600556404646, -0.2362204724409448231, -1.284120734908136496 ) ) ;
#45260=CARTESIAN_POINT ( 'NONE',  ( -0.1998031496062994405, 0.3460692066303957537, -2.294619422572178102 ) ) ;
#45264=CARTESIAN_POINT ( 'NONE',  ( 0.1998031496062994128, -0.3460692066303957537, -1.270997375328084100 ) ) ;
#45270=CARTESIAN_POINT ( 'NONE',  ( 0.3460692066303958092, 0.1998031496062993018, -0.8379265091863516979 ) ) ;
#45271=CARTESIAN_POINT ( 'NONE',  ( -0.1998031496062991907, -0.3460692066303959757, -0.8530183727034120755 ) ) ;
#45272=CARTESIAN_POINT ( 'NONE',  ( -0.3420746716998661618, 0.1974969037888702206, -0.4986876640419948270 ) ) ;
#45279=CARTESIAN_POINT ( 'NONE',  ( 0.3949938075777409963, 2.418639510665530743E-17, -1.297244094488188892 ) ) ;
#45284=CARTESIAN_POINT ( 'NONE',  ( -0.4724409448818898682, -8.678599364036362592E-17, -1.456692913385826849 ) ) ;
#45285=CARTESIAN_POINT ( 'NONE',  ( -0.1070741851644051862, -0.3996062992125986590, -2.749343832020996636 ) ) ;
#45292=CARTESIAN_POINT ( 'NONE',  ( -0.3392501089628018329, -0.1958661417322836440, -1.864810080543620074 ) ) ;
#45299=CARTESIAN_POINT ( 'NONE',  ( -0.1958661417322836718, 0.3392501089628017219, -1.265091863517060489 ) ) ;
#45302=CARTESIAN_POINT ( 'NONE',  ( -9.674558042662121740E-17, 0.3949938075777409963, -2.047244094488188892 ) ) ;
#45308=CARTESIAN_POINT ( 'NONE',  ( -0.2925321140481932924, 0.2925321140481931814, -0.01968503937007875029 ) ) ;
#45311=SURFACE_SIDE_STYLE ('',( #27215 ) ) ;
#45315=CARTESIAN_POINT ( 'NONE',  ( 0.1049643490035303689, 0.3917322834645670104, -0.2355643044619422921 ) ) ;
#45322=CARTESIAN_POINT ( 'NONE',  ( 0.3996062992125985480, 2.446882876249141654E-17, -2.084645669291338432 ) ) ;
#45327=CARTESIAN_POINT ( 'NONE',  ( -0.4724409448818895907, -0.1265901696524993070, -0.9908136482939633449 ) ) ;
#45329=CARTESIAN_POINT ( 'NONE',  ( 0.1049643490035303689, 0.3917322834645670104, -0.3005249343832020470 ) ) ;
#45330=CARTESIAN_POINT ( 'NONE',  ( 0.3917322834645669549, 0.1049643490035304660, -2.099081364829396446 ) ) ;
#45334=CARTESIAN_POINT ( 'NONE',  ( 0.4724409448818897572, -0.1265901696524988906, -2.708005249343832688 ) ) ;
#45338=CARTESIAN_POINT ( 'NONE',  ( 0.3949938075777409963, 2.418639510665530743E-17, -2.714566929133857887 ) ) ;
#45346=CARTESIAN_POINT ( 'NONE',  ( -0.1049643490035302024, -0.3917322834645671215, -1.481627296587926690 ) ) ;
#45349=CARTESIAN_POINT ( 'NONE',  ( 0.4724409448818898682, 2.892866454678787531E-17, 0.1200787401574803098 ) ) ;
#45362=CARTESIAN_POINT ( 'NONE',  ( -0.1070741851644051862, -0.3996062992125986590, -1.093832020997375087 ) ) ;
#45363=CARTESIAN_POINT ( 'NONE',  ( 4.797336870675656522E-17, -0.3917322834645670104, -2.683070866141731958 ) ) ;
#45374=CARTESIAN_POINT ( 'NONE',  ( -0.1049643490035307158, 0.3917322834645670104, -1.893063935204411186 ) ) ;
#45380=CARTESIAN_POINT ( 'NONE',  ( 0.3917322834645670104, 2.398668435337828261E-17, -1.935039370078740273 ) ) ;
#45387=CARTESIAN_POINT ( 'NONE',  ( -0.3996062992125986035, -7.340648628747425578E-17, -1.141732283464566899 ) ) ;
#45389=CARTESIAN_POINT ( 'NONE',  ( -0.3917322834645670104, -0.1049643490035307020, -0.04267023441700976139 ) ) ;
#45403=CARTESIAN_POINT ( 'NONE',  ( -0.2867679344610365999, 0.2867679344610364889, -0.1692913385826771144 ) ) ;
#45406=CARTESIAN_POINT ( 'NONE',  ( 0.2891555358219910499, -0.2891555358219909944, -0.7283464566929134243 ) ) ;
#45413=CARTESIAN_POINT ( 'NONE',  ( -0.1049643490035302301, -0.3917322834645671770, -1.801200418144043969 ) ) ;
#45419=CARTESIAN_POINT ( 'NONE',  ( 0.3996062992125986590, -0.1070741851644053111, -1.371391076115485053 ) ) ;
#45421=CARTESIAN_POINT ( 'NONE',  ( -0.3996062992125985480, -7.340648628747423112E-17, -0.9035433070866141225 ) ) ;
#45422=CARTESIAN_POINT ( 'NONE',  ( -0.1070741851644051862, -0.3996062992125986590, -0.3064304461942257141 ) ) ;
#45424=CARTESIAN_POINT ( 'NONE',  ( -0.1070741851644056997, 0.3996062992125986035, -2.526246719160104792 ) ) ;
#45425=CARTESIAN_POINT ( 'NONE',  ( -0.1049643490035307020, 0.3917322834645669549, -2.138451443569553412 ) ) ;
#45432=CARTESIAN_POINT ( 'NONE',  ( -0.4724409448818899238, 0.1265901696524986686, -1.369422572178477404 ) ) ;
#45435=CARTESIAN_POINT ( 'NONE',  ( 0.3420746716998660508, 0.1974969037888705814, -1.467847769028871374 ) ) ;
#45445=CARTESIAN_POINT ( 'NONE',  ( -0.2925321140481932369, 0.2925321140481931259, -1.986220472440945128 ) ) ;
#45447=CARTESIAN_POINT ( 'NONE',  ( 0.3917322834645669549, 2.398668435337827645E-17, -2.245387508365142892 ) ) ;
#45461=CARTESIAN_POINT ( 'NONE',  ( -0.3917322834645670104, -7.196005306013484475E-17, -1.383858267716535417 ) ) ;
#45482=CARTESIAN_POINT ( 'NONE',  ( 0.3917322834645670104, 2.398668435337828261E-17, -2.629921259842519898 ) ) ;
#45485=CARTESIAN_POINT ( 'NONE',  ( -0.2362204724409451284, 0.4091458600556402425, -0.8005249343832020470 ) ) ;
#45486=CARTESIAN_POINT ( 'NONE',  ( -0.3996062992125986035, -7.340648628747425578E-17, 0.1181102362204724254 ) ) ;
#45489=CARTESIAN_POINT ( 'NONE',  ( 0.1958661417322836440, -0.3392501089628017219, -1.658792650918635259 ) ) ;
#45493=CARTESIAN_POINT ( 'NONE',  ( 0.4091458600556404646, -0.2362204724409448231, -2.939632545931758489 ) ) ;
#45500=CARTESIAN_POINT ( 'NONE',  ( 0.3917322834645669549, 2.398668435337827645E-17, -1.300505618601362601 ) ) ;
#45507=CARTESIAN_POINT ( 'NONE',  ( -0.1049643490035307158, 0.3917322834645670104, -2.365504880086300776 ) ) ;
#45516=CARTESIAN_POINT ( 'NONE',  ( 0.2867679344610365999, -0.2867679344610365444, -1.915354330708661124 ) ) ;
#45532=CARTESIAN_POINT ( 'NONE',  ( 0.2362204724409451007, -0.4091458600556402980, -0.3261154855643044748 ) ) ;
#45535=CARTESIAN_POINT ( 'NONE',  ( 0.3420746716998660508, -0.1974969037888704149, -0.3392388451443569819 ) ) ;
#45540=CARTESIAN_POINT ( 'NONE',  ( -0.3420746716998662729, 0.1974969037888702206, -0.1030183727034120894 ) ) ;
#45548=CARTESIAN_POINT ( 'NONE',  ( -0.2925321140481930149, -0.2925321140481933480, -0.7657480314960628531 ) ) ;
#45550=CARTESIAN_POINT ( 'NONE',  ( 0.1958661417322834775, 0.3392501089628018884, -0.4514435695538057125 ) ) ;
#45553=CARTESIAN_POINT ( 'NONE',  ( -0.4724409448818898682, -8.678599364036362592E-17, -2.559055118110236560 ) ) ;
#45564=EDGE_CURVE ( 'NONE', #37037, #36386, #40215, .T. ) ;
#45567=CARTESIAN_POINT ( 'NONE',  ( 0.1265901696524990294, -0.4724409448818896462, -2.366797900262467280 ) ) ;
#45584=CARTESIAN_POINT ( 'NONE',  ( -0.3996062992125986035, -7.340648628747425578E-17, -0.5118110236220472231 ) ) ;
#45590=CARTESIAN_POINT ( 'NONE',  ( 0.3996062992125986035, 0.1070741851644054776, -2.801837270341207553 ) ) ;
#45591=CARTESIAN_POINT ( 'NONE',  ( 0.3949938075777409963, 2.418639510665530435E-17, -2.007874015748031482 ) ) ;
#45592=CARTESIAN_POINT ( 'NONE',  ( 0.2867679344610365999, -0.2867679344610365444, -0.5629921259842519676 ) ) ;
#45594=CARTESIAN_POINT ( 'NONE',  ( 0.2867679344610366554, -0.2867679344610365444, -0.8779527559055116948 ) ) ;
#45596=CARTESIAN_POINT ( 'NONE',  ( 0.3917322834645670104, 2.398668435337828261E-17, -0.8976377952755905110 ) ) ;
#45598=CARTESIAN_POINT ( 'NONE',  ( -0.3949938075777408852, -0.1058382717557502933, -2.799868766404199683 ) ) ;
#45604=CARTESIAN_POINT ( 'NONE',  ( -0.1070741851644056997, 0.3996062992125986035, -2.683727034120735322 ) ) ;
#45605=CARTESIAN_POINT ( 'NONE',  ( 0.3917322834645670659, -0.1049643490035303273, -1.053168922081052283 ) ) ;
#45611=CARTESIAN_POINT ( 'NONE',  ( -0.1958661417322836718, 0.3392501089628017219, -0.7276902887139108378 ) ) ;
#45619=CARTESIAN_POINT ( 'NONE',  ( 0.02544847934575847695, -0.3910482532978202808, -1.929133858267716439 ) ) ;
#45620=CARTESIAN_POINT ( 'NONE',  ( -0.1049643490035307020, 0.3917322834645669549, -1.730971128608923992 ) ) ;
#45623=CARTESIAN_POINT ( 'NONE',  ( -0.2925321140481930704, -0.2925321140481933480, 0.09842519685039367860 ) ) ;
#45630=CARTESIAN_POINT ( 'NONE',  ( 0.1958661417322834775, 0.3392501089628018884, -0.8589238845144357981 ) ) ;
#45639=CARTESIAN_POINT ( 'NONE',  ( 0.1265901696524989184, 0.4724409448818898127, -2.670603674540682260 ) ) ;
#45649=CARTESIAN_POINT ( 'NONE',  ( -0.2867679344610366554, 0.2867679344610365444, -0.8871197918297093477 ) ) ;
#45658=CARTESIAN_POINT ( 'NONE',  ( -0.2867679344610365444, -0.2867679344610367664, 0.1016867209635676783 ) ) ;
#45661=CARTESIAN_POINT ( 'NONE',  ( -0.4724409448818898682, -8.678599364036362592E-17, -1.218503937007874072 ) ) ;
#45675=CARTESIAN_POINT ( 'NONE',  ( -9.787531504996566615E-17, 0.3996062992125985480, -2.596456692913385655 ) ) ;
#45679=CARTESIAN_POINT ( 'NONE',  ( 0.3996062992125984925, 0.1070741851644054637, -1.933727034120735100 ) ) ;
#45685=CARTESIAN_POINT ( 'NONE',  ( -0.1070741851644057135, 0.3996062992125984925, -1.028215223097112663 ) ) ;
#45686=CARTESIAN_POINT ( 'NONE',  ( 0.1070741851644053527, 0.3996062992125986590, -1.253280839895013044 ) ) ;
#45687=CARTESIAN_POINT ( 'NONE',  ( 0.1058382717557499880, 0.3949938075777411073, -0.6233595800524935893 ) ) ;
#45693=CARTESIAN_POINT ( 'NONE',  ( -0.2891555358219911054, 0.2891555358219909388, -1.671259842519685179 ) ) ;
#45699=CARTESIAN_POINT ( 'NONE',  ( -0.1265901696524986964, -0.4724409448818899238, -1.489501312335957950 ) ) ;
#45700=CARTESIAN_POINT ( 'NONE',  ( 0.1123167701215799369, 0.3758920641862485423, -2.755905511811022279 ) ) ;
#45708=CARTESIAN_POINT ( 'NONE',  ( -0.1049643490035306742, 0.3917322834645668994, -2.133838951934696304 ) ) ;
#45714=CARTESIAN_POINT ( 'NONE',  ( -0.3917322834645670104, -7.196005306013484475E-17, 0.1909448818897636901 ) ) ;
#45716=CARTESIAN_POINT ( 'NONE',  ( 4.797336870675656522E-17, -0.3917322834645670104, -1.330708661417322691 ) ) ;
#45719=CARTESIAN_POINT ( 'NONE',  ( -0.3420746716998659953, -0.1974969037888706647, -1.784776902887138972 ) ) ;
#45724=CARTESIAN_POINT ( 'NONE',  ( -0.1070741851644056997, 0.3996062992125986035, -0.6364829396325458744 ) ) ;
#45728=( NAMED_UNIT ( * ) PLANE_ANGLE_UNIT ( ) SI_UNIT ( $, .RADIAN. ) );
#45732=CARTESIAN_POINT ( 'NONE',  ( 0.1958661417322836440, -0.3392501089628017219, -0.3339895013123360679 ) ) ;
#45738=ORIENTED_EDGE ( 'NONE', *, *, #31645, .T. ) ;
#45739=CARTESIAN_POINT ( 'NONE',  ( 0.1998031496062992463, 0.3460692066303959202, -1.795931758530183719 ) ) ;
#45744=CARTESIAN_POINT ( 'NONE',  ( 0.2362204724409451007, -0.4091458600556402980, -0.8792650918635170898 ) ) ;
#45746=CARTESIAN_POINT ( 'NONE',  ( -9.594673741351313045E-17, 0.3917322834645670104, -0.4645669291338582751 ) ) ;
#45747=DIRECTION ( 'NONE',  ( 0.000000000000000000, 0.000000000000000000, 1.000000000000000000 ) ) ;
#45751=CARTESIAN_POINT ( 'NONE',  ( -0.3996062992125985480, -7.340648628747423112E-17, 0.1988188976377952277 ) ) ;
#45755=CARTESIAN_POINT ( 'NONE',  ( 0.3420746716998660508, 0.1974969037888705814, -2.570209973753280863 ) ) ;
#45761=CARTESIAN_POINT ( 'NONE',  ( -0.2867679344610364334, -0.2867679344610367109, -1.625984251968503491 ) ) ;
#45764=CARTESIAN_POINT ( 'NONE',  ( -0.4091458600556402980, -0.2362204724409451284, 0.1856955380577427484 ) ) ;
#45778=CARTESIAN_POINT ( 'NONE',  ( -0.3996062992125984925, -0.1070741851644056858, -1.225065616797899937 ) ) ;
#45779=CARTESIAN_POINT ( 'NONE',  ( -0.1958661417322834220, -0.3392501089628018884, -2.827427821522309426 ) ) ;
#45789=CARTESIAN_POINT ( 'NONE',  ( 4.797336870675656522E-17, -0.3917322834645670659, -2.595163672737219596 ) ) ;
#45792=CARTESIAN_POINT ( 'NONE',  ( 0.01930322177395383046, -0.3957358693849765685, -5.613290098372282899E-13 ) ) ;
#45796=CARTESIAN_POINT ( 'NONE',  ( 4.797336870675656522E-17, -0.3917322834645670104, -2.210629921259842590 ) ) ;
#45804=CARTESIAN_POINT ( 'NONE',  ( -0.2925321140481930704, -0.2925321140481933480, -1.161417322834645383 ) ) ;
#45806=CARTESIAN_POINT ( 'NONE',  ( 0.1049643490035304799, -0.3917322834645670104, -0.08204031315716725503 ) ) ;
#45817=CARTESIAN_POINT ( 'NONE',  ( 0.1049643490035304938, -0.3917322834645669549, -0.3923884514435695414 ) ) ;
#45820=CARTESIAN_POINT ( 'NONE',  ( 0.3420746716998659953, 0.1974969037888705536, -0.4461942257217848540 ) ) ;
#45835=CARTESIAN_POINT ( 'NONE',  ( 0.3460692066303959202, 0.1998031496062993295, -1.233595800524934338 ) ) ;
#45837=CARTESIAN_POINT ( 'NONE',  ( 0.3460692066303959202, -0.1998031496062991630, -0.8116797900262466836 ) ) ;
#45838=CARTESIAN_POINT ( 'NONE',  ( 0.1998031496062994128, -0.3460692066303957537, -0.1686351706036745557 ) ) ;
#45840=CARTESIAN_POINT ( 'NONE',  ( 0.3996062992125986035, 0.1070741851644054776, -2.644356955380577912 ) ) ;
#45841=CARTESIAN_POINT ( 'NONE',  ( -0.3917322834645671215, 0.1049643490035301469, -2.164698162729658648 ) ) ;
#45847=CARTESIAN_POINT ( 'NONE',  ( -0.2362204724409451284, 0.4091458600556402425, -1.664698162729658426 ) ) ;
#45850=CARTESIAN_POINT ( 'NONE',  ( 0.2891555358219910499, -0.2891555358219909944, -1.435039370078739829 ) ) ;
#45861=CARTESIAN_POINT ( 'NONE',  ( -0.1070741851644056997, 0.3996062992125984925, -2.130577427821522818 ) ) ;
#45863=CARTESIAN_POINT ( 'NONE',  ( -0.1049643490035306742, 0.3917322834645668994, -2.133838951934696304 ) ) ;
#45875=CARTESIAN_POINT ( 'NONE',  ( -9.787531504996566615E-17, 0.3996062992125985480, -0.07677165354330710290 ) ) ;
#45877=CARTESIAN_POINT ( 'NONE',  ( -0.2867679344610364334, -0.2867679344610367109, -1.561023622047243986 ) ) ;
#45891=VECTOR ( 'NONE', #79735, 39.37007874015748143 ) ;
#45899=CARTESIAN_POINT ( 'NONE',  ( -0.1049643490035301885, -0.3917322834645671215, -2.426509186351705871 ) ) ;
#45902=CARTESIAN_POINT ( 'NONE',  ( 0.1265901696524990294, -0.4724409448818896462, -0.7152230971128609172 ) ) ;
#45903=CARTESIAN_POINT ( 'NONE',  ( -0.3996062992125986035, -0.1070741851644056997, -0.2034120734908136385 ) ) ;
#45904=VERTEX_POINT ( 'NONE', #54490 ) ;
#45906=CARTESIAN_POINT ( 'NONE',  ( -0.3392501089628019995, 0.1958661417322832277, -1.908136482939632561 ) ) ;
#45910=CARTESIAN_POINT ( 'NONE',  ( -0.3458507752293909498, 0.3458507752293907833, -2.696850393700787052 ) ) ;
#45917=CARTESIAN_POINT ( 'NONE',  ( 0.1049643490035304522, -0.3917322834645668994, -1.110216904690602080 ) ) ;
#45923=CARTESIAN_POINT ( 'NONE',  ( 0.1958661417322836718, -0.3392501089628017219, -2.608287032317271770 ) ) ;
#45931=CARTESIAN_POINT ( 'NONE',  ( 0.1049643490035304938, -0.3917322834645669549, -1.744750656167979308 ) ) ;
#45947=CARTESIAN_POINT ( 'NONE',  ( -0.4724409448818898682, -8.678599364036362592E-17, -2.478346456692913868 ) ) ;
#45948=CARTESIAN_POINT ( 'NONE',  ( -1.157146581871515012E-16, 0.4724409448818898682, -0.07677165354330710290 ) ) ;
#45951=CARTESIAN_POINT ( 'NONE',  ( 0.1974969037888704704, 0.3420746716998660508, -0.06364829396325460964 ) ) ;
#45957=CARTESIAN_POINT ( 'NONE',  ( -0.3420746716998660508, -0.1974969037888706924, -0.1292650918635170898 ) ) ;
#45960=VECTOR ( 'NONE', #32032, 39.37007874015748143 ) ;
#45965=CARTESIAN_POINT ( 'NONE',  ( -0.1070741851644051862, -0.3996062992125986590, -0.7788713910761155823 ) ) ;
#45968=CARTESIAN_POINT ( 'NONE',  ( -0.3392501089628017219, -0.1958661417322836718, -0.8320209973753279753 ) ) ;
#45981=CARTESIAN_POINT ( 'NONE',  ( -0.3983403474834782965, -0.03178304480584832892, -1.220472440944881942 ) ) ;
#45983=CARTESIAN_POINT ( 'NONE',  ( 0.3996062992125986035, -0.1070741851644052972, 0.1266404199475064940 ) ) ;
#45990=CARTESIAN_POINT ( 'NONE',  ( 0.4724409448818898682, 2.892866454678787531E-17, -2.007874015748031482 ) ) ;
#46000=CARTESIAN_POINT ( 'NONE',  ( -0.1998031496062994683, 0.3460692066303958092, -0.1706036745406824540 ) ) ;
#46005=CARTESIAN_POINT ( 'NONE',  ( -0.1998031496062991907, -0.3460692066303959757, -2.742782152230971437 ) ) ;
#46006=CARTESIAN_POINT ( 'NONE',  ( -0.1058382717557497937, -0.3949938075777411628, -2.119422572178478070 ) ) ;
#46007=CARTESIAN_POINT ( 'NONE',  ( -0.1049643490035302024, -0.3917322834645671215, -0.6942257217847765949 ) ) ;
#46009=CARTESIAN_POINT ( 'NONE',  ( 0.2867679344610366554, -0.2867679344610365444, -1.192913385826771533 ) ) ;
#46011=CARTESIAN_POINT ( 'NONE',  ( 0.2867679344610365999, -0.2867679344610365444, -1.035433070866141447 ) ) ;
#46014=CARTESIAN_POINT ( 'NONE',  ( -0.3917322834645670659, 0.1049643490035301607, 0.04463873835401757639 ) ) ;
#46021=CARTESIAN_POINT ( 'NONE',  ( -0.3460692066303958092, -0.1998031496062994683, -2.729658792650918375 ) ) ;
#46022=CARTESIAN_POINT ( 'NONE',  ( 0.1049643490035303967, 0.3917322834645670659, -1.407499630742469199 ) ) ;
#46028=CARTESIAN_POINT ( 'NONE',  ( -0.3917322834645671215, 0.1049643490035301469, -0.4324146981627298159 ) ) ;
#46036=CARTESIAN_POINT ( 'NONE',  ( 0.3204081651526057839, -0.2263583204863392762, -1.929133858267716883 ) ) ;
#46037=CARTESIAN_POINT ( 'NONE',  ( -0.1049643490035302024, -0.3917322834645671215, -2.111548556430446144 ) ) ;
#46040=CARTESIAN_POINT ( 'NONE',  ( -0.2925321140481932924, 0.2925321140481931814, 0.1377952755905511584 ) ) ;
#46048=CARTESIAN_POINT ( 'NONE',  ( 0.1049643490035304938, -0.3917322834645669549, -0.9573490813648293241 ) ) ;
#46051=CARTESIAN_POINT ( 'NONE',  ( -0.3979867861067992729, -0.002674255378744507493, -1.929133858267716661 ) ) ;
#46057=CARTESIAN_POINT ( 'NONE',  ( -0.4724409448818898682, -8.678599364036362592E-17, -2.716535433070865757 ) ) ;
#46066=( BOUNDED_SURFACE ( )  B_SPLINE_SURFACE ( 1, 2, ( 
 ( #25163, #342, #44510, #13390, #762, #7914, #18861, #38212, #45764, #7493, #39043, #32314, #58403, #71463, #1188, #6226, #25999, #26424, #45349, #50832, #52076, #51656, #6642, #77784, #83253, #26838, #63887, #70618, #33162, #44921, #31901, #20117, #20536, #65156, #13810, #7066, #14234, #39469, #71046, #78205, #52496, #58830, #25576, #46187, #71884, #64727, #32735, #76942, #65580, #77360, #70198, #19692, #76533, #39893, #33575, #12553, #12974, #19268, #38630, #64308, #54161, #54581, #67236, #20950, #46608, #48266, #41953, #80292, #8325, #47019, #9567, #35237, #60490, #72304, #73963, #27253, #22606, #33991, #52912, #21365, #78626, #16309, #15899, #21773, #60901, #67647, #14650, #73128, #40307, #15479, #53338, #3253, #9982, #59653, #8738, #35650, #1598, #65987, #2009, #27671, #47435, #79047, #28915, #72712, #22193, #15059, #73555, #40715, #34408, #66400, #41136, #2431, #60076, #28088, #53745, #79454, #66826, #9158, #34831, #2840, #28503, #79875, #47850, #41547, #11640, #4071, #30570, #4898, #36467, #17141, #17545, #50324, #37299, #12044, #23013, #80700, #49508, #74792, #56236, #69701, #36062, #23425, #81108, #11222, #10807, #62142, #56637, #29331, #81933, #49090, #48681, #42773, #36882, #23841, #4481, #16720, #62973, #61734, #68469, #29738, #43177, #55401, #74377, #42361, #76022, #75615, #24244, #30151, #68060, #30970, #61312, #54992, #75201, #10405, #49917, #55813, #3668, #17953, #82338, #68874, #5312, #43590, #62560, #24656, #81521, #69291, #18365, #44007, #12451, #63786, #6125, #70099, #240, #31799, #63375, #20429, #38941, #26314, #44405, #38112, #20010, #25892, #658, #64622, #57460, #83153, #25473, #51974, #77255, #51552, #51140, #13704, #19168, #6544, #38529, #6959, #44816, #32630, #76433, #76834, #58293, #70513, #45661, #77680, #12870, #64210, #39359, #58719, #32214, #57873, #71357, #19585, #45246, #65044, #70944, #13289, #18762, #7381, #33049, #1083, #26735, #52389, #78098, #46082, #71775, #5711, #37702, #31381, #57046, #82740, #25060, #50734, #21670, #40202, #65477, #33475, #27983, #1495, #46914, #14129, #40613, #66296, #72608, #54055, #2326, #80189, #7809, #59137, #48167, #14956, #27147, #53643, #73021, #22506, #52811, #78521, #34727, #79770, #79351, #21260, #47331, #60386, #73445, #20845, #8635, #15371, #34306, #39782, #41032, #59967, #78941, #66718, #46498, #15795, #72197, #59551, #22086, #33885, #14551, #9054, #9459, #47745, #2737, #28397, #3149, #41445, #67129, #35133, #60795, #28813, #65886, #54476, #8221, #1906, #27567, #53226, #30874, #42677, #9877, #68375, #24561, #24147, #4382, #81009, #10299, #69187, #49410, #23323, #43080, #43491, #56131, #35546, #61208, #37194, #56541, #11537, #80601, #35965, #81836, #49817, #75103, #3564, #62875, #16203, #5210, #22910, #41850, #61635, #67542, #82242, #4790, #10714, #75517, #73862, #29231, #62045, #54895, #30050, #42261, #17856, #48578, #74275, #48993, #16619, #67956, #3976, #29640, #55301, #74691, #17037, #36371, #23737, #55712, #81421, #17450, #68777, #11121, #36778, #62454, #30467, #6030, #6448, #39262, #563, #988, #11948, #69602, #38430, #63691, #19490, #58620, #24960, #12357, #70002, #139, #83056, #51041, #45567, #18262, #77158, #38015, #37603, #31701, #25795, #12773, #25378, #5618, #51878, #50632, #57360, #76337, #32118, #44312, #63277, #31284, #64944, #64525, #13198, #76742, #56949, #19918, #50227, #43904, #64113, #82646, #45143, #18667, #75923, #6862, #71262, #57776, #26216, #32531, #51455, #13608, #19072, #44720, #7284, #70418, #70847, #38845, #58195, #77584, #32954, #27055, #26643, #53961, #66203, #2225, #7714, #59045, #21573, #53129, #27890, #8542, #33382, #52714, #20753, #53550, #46822, #78840, #78425, #72924, #14455, #59458, #33793, #34208, #40107, #59871, #65379, #46403, #79258, #1399, #47235, #15276 ),
 ( #28299, #66616, #72096, #65794, #40937, #8953, #40524, #14031, #34628, #21166, #60292, #2642, #52297, #8128, #78003, #20331, #14862, #45983, #1809, #71679, #72513, #27471, #39687, #52571, #52152, #32388, #25651, #38287, #13884, #77434, #51313, #71118, #71536, #842, #37877, #63551, #65232, #58903, #39543, #25237, #63963, #26500, #77858, #19769, #5885, #7569, #44175, #33241, #50902, #69868, #6300, #12220, #1263, #32811, #38703, #20187, #26911, #31558, #6718, #57215, #58051, #70274, #45838, #18532, #76602, #77016, #82917, #18933, #44581, #12628, #31976, #64382, #57636, #7370, #19348, #39118, #44998, #7138, #70697, #13050, #417, #26073, #51732, #45422, #13461, #64799, #58478, #8810, #65658, #27748, #78279, #21438, #47094, #53412, #34903, #66475, #60973, #46263, #71958, #28988, #79121, #14311, #34486, #53819, #3324, #39971, #7987, #15553, #60565, #60152, #2083, #28163, #41212, #54236, #59314, #72784, #79533, #15134, #20611, #21847, #40790, #59728, #47511, #27327, #79953, #33651, #40379, #2916, #14726, #1670, #73203, #73629, #28579, #66900, #2504, #67307, #21023, #9230, #22266, #47924, #34065, #15971, #9642, #41618, #52987, #78700, #46684, #35311, #8398, #72377, #66062, #60200, #80414, #34950, #47559, #59777, #35360, #16430, #47978, #53036, #16019, #22726, #34535, #61023, #66947, #28209, #60613, #53459, #78748, #46731, #41261, #14773, #2551, #27374, #53868, #79581, #21896, #67356, #15601, #10109, #21073, #72423, #61441, #73253, #40428, #9279, #2962, #35771, #66109, #8445, #73678, #9689, #28628, #54285, #80002, #41665, #3374, #34115, #22315, #29037, #54708, #2131, #48385, #74084, #8857, #42076, #27799, #67771, #79167, #72833, #21484, #47143, #15183, #40840, #66526, #44833, #38129, #70116, #77272, #76851, #50751, #57890, #32232, #12886, #4193, #70531, #63803, #44421, #12467, #61852, #45264, #57062, #23134, #82755, #38957, #38546, #18778, #10926, #23544, #257, #6141, #37717, #57476, #25909, #64226, #48802, #74500, #51569, #70960, #19601, #10525, #49212, #6560, #13305, #31816, #16848, #3788, #29452, #55110, #36180, #80819, #74917, #42482, #68186, #25490, #29856, #76451, #63391, #83170, #51156, #55519, #81227, #5726, #19184, #25077, #17262, #42891, #31397, #68585, #40223, #13725, #40635, #77698, #26753, #46936, #1102, #71375, #59571, #59990, #21281, #14571, #46519, #53664, #53248, #27169, #34327, #8656, #72628, #65064, #14976, #65905, #20868, #72220, #39379, #21690, #33495, #677, #59157, #15391, #66317, #78543, #71796, #52408, #2348, #8241, #14149, #33907, #28004, #79371, #26331, #51993, #47353, #73042, #64641, #7402, #78117, #6978, #32647, #1927, #20028, #58312, #45679, #33071, #58740, #20450, #46103, #39803, #65496, #78962, #1515, #7828, #52831, #27590, #29251, #60408, #54915, #9482, #49015, #23758, #47769, #48187, #49431, #60817, #73884, #10734, #48599, #61231, #73468, #74712, #30072, #61656, #66739, #29661, #36391, #16224, #17059, #80621, #41871, #74295, #67153, #9077, #2759, #22933, #28418, #67565, #41053, #9897, #35568, #3585, #81032, #16641, #75125, #34748, #54078, #79793, #42281, #22109, #67979, #10322, #15819, #41468, #22525, #35986, #35157, #3169, #3997, #28833, #42698, #55323, #23344, #68395, #62065, #4404, #54497, #80209, #55735, #81443, #75536, #12376, #62895, #24580, #81856, #38034, #12792, #6049, #64132, #6466, #57793, #30894, #49837, #56561, #68797, #17876, #50655, #83076, #24168, #4812, #51061, #43510, #70023, #44332, #75943, #82262, #56968, #32136, #76761, #51473, #62477, #36801, #5637, #50247, #63709, #25813, #160, #17470, #19091, #56153, #18284, #43927, #38448, #11142, #31721, #37216, #30488, #5230, #76357, #63299, #69623, #69210, #44740, #11559, #11968, #37623, #82666, #31304, #24981, #18689, #43101, #57382, #25397, #70435, #32550, #46839, #77176, #70866 ) ),
 .UNSPECIFIED., .F., .F., .F. ) 
 B_SPLINE_SURFACE_WITH_KNOTS ( ( 2, 2 ),
 ( 3, 2, 2, 2, 2, 2, 2, 2, 2, 2, 2, 2, 2, 2, 2, 2, 2, 2, 2, 2, 2, 2, 2, 2, 2, 2, 2, 2, 2, 2, 2, 2, 2, 2, 2, 2, 2, 2, 2, 2, 2, 2, 2, 2, 2, 2, 2, 2, 2, 2, 2, 2, 2, 2, 2, 2, 2, 2, 2, 2, 2, 2, 2, 2, 2, 2, 2, 2, 2, 2, 2, 2, 2, 2, 2, 2, 2, 2, 2, 2, 2, 2, 2, 2, 2, 2, 2, 2, 2, 2, 2, 2, 2, 2, 2, 2, 2, 2, 2, 2, 2, 2, 2, 2, 2, 2, 2, 2, 2, 2, 2, 2, 2, 2, 2, 2, 2, 2, 2, 2, 2, 2, 2, 2, 2, 2, 2, 2, 2, 2, 2, 2, 2, 2, 2, 2, 2, 2, 2, 2, 2, 2, 2, 2, 2, 2, 2, 2, 2, 2, 2, 2, 2, 2, 2, 2, 2, 2, 2, 2, 2, 2, 2, 2, 2, 2, 2, 2, 2, 2, 2, 2, 2, 2, 2, 2, 2, 2, 2, 2, 2, 2, 2, 2, 2, 2, 2, 2, 2, 2, 2, 2, 2, 2, 2, 2, 2, 2, 2, 2, 2, 2, 2, 2, 2, 2, 2, 2, 2, 2, 2, 2, 2, 2, 2, 2, 2, 2, 2, 2, 2, 2, 2, 2, 2, 2, 2, 2, 2, 2, 2, 2, 2, 2, 2, 2, 2, 3 ),
 ( 0.000000000000000000, 1.000000000000000000 ),
 ( 0.000000000000000000, 0.004166666666666666609, 0.008333333333333333218, 0.01250000000000000069, 0.01666666666666666644, 0.02083333333333333218, 0.02500000000000000139, 0.02916666666666666713, 0.03333333333333333287, 0.03749999999999999861, 0.04166666666666666435, 0.04583333333333333010, 0.05000000000000000278, 0.05416666666666666852, 0.05833333333333333426, 0.06250000000000000000, 0.06666666666666666574, 0.07083333333333333148, 0.07499999999999999722, 0.07916666666666666297, 0.08333333333333332871, 0.08749999999999999445, 0.09166666666666666019, 0.09583333333333333981, 0.1000000000000000056, 0.1041666666666666713, 0.1083333333333333370, 0.1125000000000000028, 0.1166666666666666685, 0.1208333333333333343, 0.1250000000000000000, 0.1291666666666666796, 0.1333333333333333315, 0.1375000000000000111, 0.1416666666666666630, 0.1458333333333333426, 0.1499999999999999944, 0.1541666666666666741, 0.1583333333333333259, 0.1625000000000000056, 0.1666666666666666574, 0.1708333333333333370, 0.1749999999999999889, 0.1791666666666666685, 0.1833333333333333204, 0.1875000000000000000, 0.1916666666666666796, 0.1958333333333333315, 0.2000000000000000111, 0.2041666666666666630, 0.2083333333333333426, 0.2124999999999999944, 0.2166666666666666741, 0.2208333333333333259, 0.2250000000000000056, 0.2291666666666666574, 0.2333333333333333370, 0.2374999999999999889, 0.2416666666666666685, 0.2458333333333333204, 0.2500000000000000000, 0.2541666666666666519, 0.2583333333333333592, 0.2625000000000000111, 0.2666666666666666630, 0.2708333333333333148, 0.2750000000000000222, 0.2791666666666666741, 0.2833333333333333259, 0.2874999999999999778, 0.2916666666666666852, 0.2958333333333333370, 0.2999999999999999889, 0.3041666666666666408, 0.3083333333333333481, 0.3125000000000000000, 0.3166666666666666519, 0.3208333333333333592, 0.3250000000000000111, 0.3291666666666666630, 0.3333333333333333148, 0.3375000000000000222, 0.3416666666666666741, 0.3458333333333333259, 0.3499999999999999778, 0.3541666666666666852, 0.3583333333333333370, 0.3624999999999999889, 0.3666666666666666408, 0.3708333333333333481, 0.3750000000000000000, 0.3791666666666666519, 0.3833333333333333592, 0.3875000000000000111, 0.3916666666666666630, 0.3958333333333333148, 0.4000000000000000222, 0.4041666666666666741, 0.4083333333333333259, 0.4124999999999999778, 0.4166666666666666852, 0.4208333333333333370, 0.4249999999999999889, 0.4291666666666666408, 0.4333333333333333481, 0.4375000000000000000, 0.4416666666666666519, 0.4458333333333333592, 0.4500000000000000111, 0.4541666666666666630, 0.4583333333333333148, 0.4625000000000000222, 0.4666666666666666741, 0.4708333333333333259, 0.4749999999999999778, 0.4791666666666666852, 0.4833333333333333370, 0.4874999999999999889, 0.4916666666666666408, 0.4958333333333333481, 0.5000000000000000000, 0.5041666666666666519, 0.5083333333333333037, 0.5124999999999999556, 0.5166666666666667185, 0.5208333333333333703, 0.5250000000000000222, 0.5291666666666666741, 0.5333333333333333259, 0.5374999999999999778, 0.5416666666666666297, 0.5458333333333332815, 0.5500000000000000444, 0.5541666666666666963, 0.5583333333333333481, 0.5625000000000000000, 0.5666666666666666519, 0.5708333333333333037, 0.5749999999999999556, 0.5791666666666667185, 0.5833333333333333703, 0.5875000000000000222, 0.5916666666666666741, 0.5958333333333333259, 0.5999999999999999778, 0.6041666666666666297, 0.6083333333333332815, 0.6125000000000000444, 0.6166666666666666963, 0.6208333333333333481, 0.6250000000000000000, 0.6291666666666666519, 0.6333333333333333037, 0.6374999999999999556, 0.6416666666666667185, 0.6458333333333333703, 0.6500000000000000222, 0.6541666666666666741, 0.6583333333333333259, 0.6624999999999999778, 0.6666666666666666297, 0.6708333333333332815, 0.6750000000000000444, 0.6791666666666666963, 0.6833333333333333481, 0.6875000000000000000, 0.6916666666666666519, 0.6958333333333333037, 0.6999999999999999556, 0.7041666666666667185, 0.7083333333333333703, 0.7125000000000000222, 0.7166666666666666741, 0.7208333333333333259, 0.7249999999999999778, 0.7291666666666666297, 0.7333333333333332815, 0.7375000000000000444, 0.7416666666666666963, 0.7458333333333333481, 0.7500000000000000000, 0.7541666666666666519, 0.7583333333333333037, 0.7624999999999999556, 0.7666666666666667185, 0.7708333333333333703, 0.7750000000000000222, 0.7791666666666666741, 0.7833333333333333259, 0.7874999999999999778, 0.7916666666666666297, 0.7958333333333332815, 0.8000000000000000444, 0.8041666666666666963, 0.8083333333333333481, 0.8125000000000000000, 0.8166666666666666519, 0.8208333333333333037, 0.8249999999999999556, 0.8291666666666667185, 0.8333333333333333703, 0.8375000000000000222, 0.8416666666666666741, 0.8458333333333333259, 0.8499999999999999778, 0.8541666666666666297, 0.8583333333333332815, 0.8625000000000000444, 0.8666666666666666963, 0.8708333333333333481, 0.8750000000000000000, 0.8791666666666666519, 0.8833333333333333037, 0.8874999999999999556, 0.8916666666666667185, 0.8958333333333333703, 0.9000000000000000222, 0.9041666666666666741, 0.9083333333333333259, 0.9124999999999999778, 0.9166666666666666297, 0.9208333333333332815, 0.9250000000000000444, 0.9291666666666666963, 0.9333333333333333481, 0.9375000000000000000, 0.9416666666666666519, 0.9458333333333333037, 0.9499999999999999556, 0.9541666666666667185, 0.9583333333333333703, 0.9625000000000000222, 0.9666666666666666741, 0.9708333333333333259, 0.9749999999999999778, 0.9791666666666666297, 0.9833333333333332815, 0.9875000000000000444 ),
 .UNSPECIFIED. ) 
 GEOMETRIC_REPRESENTATION_ITEM ( )  RATIONAL_B_SPLINE_SURFACE ( (
 ( 1.000000000000000000, 0.9659258262890683122, 1.000000000000000000, 0.9659258262890683122, 1.000000000000000000, 0.9659258262890683122, 1.000000000000000000, 0.9659258262890683122, 1.000000000000000000, 0.9659258262890683122, 1.000000000000000000, 0.9659258262890683122, 1.000000000000000000, 0.9659258262890683122, 1.000000000000000000, 0.9659258262890683122, 1.000000000000000000, 0.9659258262890683122, 1.000000000000000000, 0.9659258262890683122, 1.000000000000000000, 0.9659258262890683122, 1.000000000000000000, 0.9659258262890683122, 1.000000000000000000, 0.9659258262890683122, 1.000000000000000000, 0.9659258262890683122, 1.000000000000000000, 0.9659258262890683122, 1.000000000000000000, 0.9659258262890683122, 1.000000000000000000, 0.9659258262890683122, 1.000000000000000000, 0.9659258262890683122, 1.000000000000000000, 0.9659258262890683122, 1.000000000000000000, 0.9659258262890683122, 1.000000000000000000, 0.9659258262890683122, 1.000000000000000000, 0.9659258262890683122, 1.000000000000000000, 0.9659258262890683122, 1.000000000000000000, 0.9659258262890683122, 1.000000000000000000, 0.9659258262890683122, 1.000000000000000000, 0.9659258262890683122, 1.000000000000000000, 0.9659258262890683122, 1.000000000000000000, 0.9659258262890683122, 1.000000000000000000, 0.9659258262890683122, 1.000000000000000000, 0.9659258262890683122, 1.000000000000000000, 0.9659258262890683122, 1.000000000000000000, 0.9659258262890683122, 1.000000000000000000, 0.9659258262890683122, 1.000000000000000000, 0.9659258262890683122, 1.000000000000000000, 0.9659258262890683122, 1.000000000000000000, 0.9659258262890683122, 1.000000000000000000, 0.9659258262890683122, 1.000000000000000000, 0.9659258262890683122, 1.000000000000000000, 0.9659258262890683122, 1.000000000000000000, 0.9659258262890683122, 1.000000000000000000, 0.9659258262890683122, 1.000000000000000000, 0.9659258262890683122, 1.000000000000000000, 0.9659258262890683122, 1.000000000000000000, 0.9659258262890683122, 1.000000000000000000, 0.9659258262890683122, 1.000000000000000000, 0.9659258262890683122, 1.000000000000000000, 0.9659258262890683122, 1.000000000000000000, 0.9659258262890683122, 1.000000000000000000, 0.9659258262890683122, 1.000000000000000000, 0.9659258262890683122, 1.000000000000000000, 0.9659258262890683122, 1.000000000000000000, 0.9659258262890683122, 1.000000000000000000, 0.9659258262890683122, 1.000000000000000000, 0.9659258262890683122, 1.000000000000000000, 0.9659258262890683122, 1.000000000000000000, 0.9659258262890683122, 1.000000000000000000, 0.9659258262890683122, 1.000000000000000000, 0.9659258262890683122, 1.000000000000000000, 0.9659258262890683122, 1.000000000000000000, 0.9659258262890683122, 1.000000000000000000, 0.9659258262890683122, 1.000000000000000000, 0.9659258262890683122, 1.000000000000000000, 0.9659258262890683122, 1.000000000000000000, 0.9659258262890683122, 1.000000000000000000, 0.9659258262890683122, 1.000000000000000000, 0.9659258262890683122, 1.000000000000000000, 0.9659258262890683122, 1.000000000000000000, 0.9659258262890683122, 1.000000000000000000, 0.9659258262890683122, 1.000000000000000000, 0.9659258262890683122, 1.000000000000000000, 0.9659258262890683122, 1.000000000000000000, 0.9659258262890683122, 1.000000000000000000, 0.9659258262890683122, 1.000000000000000000, 0.9659258262890683122, 1.000000000000000000, 0.9659258262890683122, 1.000000000000000000, 0.9659258262890683122, 1.000000000000000000, 0.9659258262890683122, 1.000000000000000000, 0.9659258262890683122, 1.000000000000000000, 0.9659258262890683122, 1.000000000000000000, 0.9659258262890683122, 1.000000000000000000, 0.9659258262890683122, 1.000000000000000000, 0.9659258262890683122, 1.000000000000000000, 0.9659258262890683122, 1.000000000000000000, 0.9659258262890683122, 1.000000000000000000, 0.9659258262890683122, 1.000000000000000000, 0.9659258262890683122, 1.000000000000000000, 0.9659258262890683122, 1.000000000000000000, 0.9659258262890683122, 1.000000000000000000, 0.9659258262890683122, 1.000000000000000000, 0.9659258262890683122, 1.000000000000000000, 0.9659258262890683122, 1.000000000000000000, 0.9659258262890683122, 1.000000000000000000, 0.9659258262890683122, 1.000000000000000000, 0.9659258262890683122, 1.000000000000000000, 0.9659258262890683122, 1.000000000000000000, 0.9659258262890683122, 1.000000000000000000, 0.9659258262890683122, 1.000000000000000000, 0.9659258262890683122, 1.000000000000000000, 0.9659258262890683122, 1.000000000000000000, 0.9659258262890683122, 1.000000000000000000, 0.9659258262890683122, 1.000000000000000000, 0.9659258262890683122, 1.000000000000000000, 0.9659258262890683122, 1.000000000000000000, 0.9659258262890683122, 1.000000000000000000, 0.9659258262890683122, 1.000000000000000000, 0.9659258262890683122, 1.000000000000000000, 0.9659258262890683122, 1.000000000000000000, 0.9659258262890683122, 1.000000000000000000, 0.9659258262890683122, 1.000000000000000000, 0.9659258262890683122, 1.000000000000000000, 0.9659258262890683122, 1.000000000000000000, 0.9659258262890683122, 1.000000000000000000, 0.9659258262890683122, 1.000000000000000000, 0.9659258262890683122, 1.000000000000000000, 0.9659258262890683122, 1.000000000000000000, 0.9659258262890683122, 1.000000000000000000, 0.9659258262890683122, 1.000000000000000000, 0.9659258262890683122, 1.000000000000000000, 0.9659258262890683122, 1.000000000000000000, 0.9659258262890683122, 1.000000000000000000, 0.9659258262890683122, 1.000000000000000000, 0.9659258262890683122, 1.000000000000000000, 0.9659258262890683122, 1.000000000000000000, 0.9659258262890683122, 1.000000000000000000, 0.9659258262890683122, 1.000000000000000000, 0.9659258262890683122, 1.000000000000000000, 0.9659258262890683122, 1.000000000000000000, 0.9659258262890683122, 1.000000000000000000, 0.9659258262890683122, 1.000000000000000000, 0.9659258262890683122, 1.000000000000000000, 0.9659258262890683122, 1.000000000000000000, 0.9659258262890683122, 1.000000000000000000, 0.9659258262890683122, 1.000000000000000000, 0.9659258262890683122, 1.000000000000000000, 0.9659258262890683122, 1.000000000000000000, 0.9659258262890683122, 1.000000000000000000, 0.9659258262890683122, 1.000000000000000000, 0.9659258262890683122, 1.000000000000000000, 0.9659258262890683122, 1.000000000000000000, 0.9659258262890683122, 1.000000000000000000, 0.9659258262890683122, 1.000000000000000000, 0.9659258262890683122, 1.000000000000000000, 0.9659258262890683122, 1.000000000000000000, 0.9659258262890683122, 1.000000000000000000, 0.9659258262890683122, 1.000000000000000000, 0.9659258262890683122, 1.000000000000000000, 0.9659258262890683122, 1.000000000000000000, 0.9659258262890683122, 1.000000000000000000, 0.9659258262890683122, 1.000000000000000000, 0.9659258262890683122, 1.000000000000000000, 0.9659258262890683122, 1.000000000000000000, 0.9659258262890683122, 1.000000000000000000, 0.9659258262890683122, 1.000000000000000000, 0.9659258262890683122, 1.000000000000000000, 0.9659258262890683122, 1.000000000000000000, 0.9659258262890683122, 1.000000000000000000, 0.9659258262890683122, 1.000000000000000000, 0.9659258262890683122, 1.000000000000000000, 0.9659258262890683122, 1.000000000000000000, 0.9659258262890683122, 1.000000000000000000, 0.9659258262890683122, 1.000000000000000000, 0.9659258262890683122, 1.000000000000000000, 0.9659258262890683122, 1.000000000000000000, 0.9659258262890683122, 1.000000000000000000, 0.9659258262890683122, 1.000000000000000000, 0.9659258262890683122, 1.000000000000000000, 0.9659258262890683122, 1.000000000000000000, 0.9659258262890683122, 1.000000000000000000, 0.9659258262890683122, 1.000000000000000000, 0.9659258262890683122, 1.000000000000000000, 0.9659258262890683122, 1.000000000000000000, 0.9659258262890683122, 1.000000000000000000, 0.9659258262890683122, 1.000000000000000000, 0.9659258262890683122, 1.000000000000000000, 0.9659258262890683122, 1.000000000000000000, 0.9659258262890683122, 1.000000000000000000, 0.9659258262890683122, 1.000000000000000000, 0.9659258262890683122, 1.000000000000000000, 0.9659258262890683122, 1.000000000000000000, 0.9659258262890683122, 1.000000000000000000, 0.9659258262890683122, 1.000000000000000000, 0.9659258262890683122, 1.000000000000000000, 0.9659258262890683122, 1.000000000000000000, 0.9659258262890683122, 1.000000000000000000, 0.9659258262890683122, 1.000000000000000000, 0.9659258262890683122, 1.000000000000000000, 0.9659258262890683122, 1.000000000000000000, 0.9659258262890683122, 1.000000000000000000, 0.9659258262890683122, 1.000000000000000000, 0.9659258262890683122, 1.000000000000000000, 0.9659258262890683122, 1.000000000000000000, 0.9659258262890683122, 1.000000000000000000, 0.9659258262890683122, 1.000000000000000000, 0.9659258262890683122, 1.000000000000000000, 0.9659258262890683122, 1.000000000000000000, 0.9659258262890683122, 1.000000000000000000, 0.9659258262890683122, 1.000000000000000000, 0.9659258262890683122, 1.000000000000000000, 0.9659258262890683122, 1.000000000000000000, 0.9659258262890683122, 1.000000000000000000, 0.9659258262890683122, 1.000000000000000000, 0.9659258262890683122, 1.000000000000000000, 0.9659258262890683122, 1.000000000000000000, 0.9659258262890683122, 1.000000000000000000, 0.9659258262890683122, 1.000000000000000000, 0.9659258262890683122, 1.000000000000000000, 0.9659258262890683122, 1.000000000000000000, 0.9659258262890683122, 1.000000000000000000, 0.9659258262890683122, 1.000000000000000000, 0.9659258262890683122, 1.000000000000000000, 0.9659258262890683122, 1.000000000000000000, 0.9659258262890683122, 1.000000000000000000, 0.9659258262890683122, 1.000000000000000000, 0.9659258262890683122, 1.000000000000000000, 0.9659258262890683122, 1.000000000000000000, 0.9659258262890683122, 1.000000000000000000, 0.9659258262890683122, 1.000000000000000000, 0.9659258262890683122, 1.000000000000000000, 0.9659258262890683122, 1.000000000000000000, 0.9659258262890683122, 1.000000000000000000, 0.9659258262890683122, 1.000000000000000000, 0.9659258262890683122, 1.000000000000000000, 0.9659258262890683122, 1.000000000000000000, 0.9659258262890683122, 1.000000000000000000, 0.9659258262890683122, 1.000000000000000000, 0.9659258262890683122, 1.000000000000000000, 0.9659258262890683122, 1.000000000000000000, 0.9659258262890683122, 1.000000000000000000, 0.9659258262890683122, 1.000000000000000000, 0.9659258262890683122, 1.000000000000000000, 0.9659258262890683122, 1.000000000000000000, 0.9659258262890683122, 1.000000000000000000, 0.9659258262890683122, 1.000000000000000000, 0.9659258262890683122, 1.000000000000000000, 0.9659258262890683122, 1.000000000000000000, 0.9659258262890683122, 1.000000000000000000, 0.9659258262890683122, 1.000000000000000000),
 ( 1.000000000000000000, 0.9659258262890683122, 1.000000000000000000, 0.9659258262890683122, 1.000000000000000000, 0.9659258262890683122, 1.000000000000000000, 0.9659258262890683122, 1.000000000000000000, 0.9659258262890683122, 1.000000000000000000, 0.9659258262890683122, 1.000000000000000000, 0.9659258262890683122, 1.000000000000000000, 0.9659258262890683122, 1.000000000000000000, 0.9659258262890683122, 1.000000000000000000, 0.9659258262890683122, 1.000000000000000000, 0.9659258262890683122, 1.000000000000000000, 0.9659258262890683122, 1.000000000000000000, 0.9659258262890683122, 1.000000000000000000, 0.9659258262890683122, 1.000000000000000000, 0.9659258262890683122, 1.000000000000000000, 0.9659258262890683122, 1.000000000000000000, 0.9659258262890683122, 1.000000000000000000, 0.9659258262890683122, 1.000000000000000000, 0.9659258262890683122, 1.000000000000000000, 0.9659258262890683122, 1.000000000000000000, 0.9659258262890683122, 1.000000000000000000, 0.9659258262890683122, 1.000000000000000000, 0.9659258262890683122, 1.000000000000000000, 0.9659258262890683122, 1.000000000000000000, 0.9659258262890683122, 1.000000000000000000, 0.9659258262890683122, 1.000000000000000000, 0.9659258262890683122, 1.000000000000000000, 0.9659258262890683122, 1.000000000000000000, 0.9659258262890683122, 1.000000000000000000, 0.9659258262890683122, 1.000000000000000000, 0.9659258262890683122, 1.000000000000000000, 0.9659258262890683122, 1.000000000000000000, 0.9659258262890683122, 1.000000000000000000, 0.9659258262890683122, 1.000000000000000000, 0.9659258262890683122, 1.000000000000000000, 0.9659258262890683122, 1.000000000000000000, 0.9659258262890683122, 1.000000000000000000, 0.9659258262890683122, 1.000000000000000000, 0.9659258262890683122, 1.000000000000000000, 0.9659258262890683122, 1.000000000000000000, 0.9659258262890683122, 1.000000000000000000, 0.9659258262890683122, 1.000000000000000000, 0.9659258262890683122, 1.000000000000000000, 0.9659258262890683122, 1.000000000000000000, 0.9659258262890683122, 1.000000000000000000, 0.9659258262890683122, 1.000000000000000000, 0.9659258262890683122, 1.000000000000000000, 0.9659258262890683122, 1.000000000000000000, 0.9659258262890683122, 1.000000000000000000, 0.9659258262890683122, 1.000000000000000000, 0.9659258262890683122, 1.000000000000000000, 0.9659258262890683122, 1.000000000000000000, 0.9659258262890683122, 1.000000000000000000, 0.9659258262890683122, 1.000000000000000000, 0.9659258262890683122, 1.000000000000000000, 0.9659258262890683122, 1.000000000000000000, 0.9659258262890683122, 1.000000000000000000, 0.9659258262890683122, 1.000000000000000000, 0.9659258262890683122, 1.000000000000000000, 0.9659258262890683122, 1.000000000000000000, 0.9659258262890683122, 1.000000000000000000, 0.9659258262890683122, 1.000000000000000000, 0.9659258262890683122, 1.000000000000000000, 0.9659258262890683122, 1.000000000000000000, 0.9659258262890683122, 1.000000000000000000, 0.9659258262890683122, 1.000000000000000000, 0.9659258262890683122, 1.000000000000000000, 0.9659258262890683122, 1.000000000000000000, 0.9659258262890683122, 1.000000000000000000, 0.9659258262890683122, 1.000000000000000000, 0.9659258262890683122, 1.000000000000000000, 0.9659258262890683122, 1.000000000000000000, 0.9659258262890683122, 1.000000000000000000, 0.9659258262890683122, 1.000000000000000000, 0.9659258262890683122, 1.000000000000000000, 0.9659258262890683122, 1.000000000000000000, 0.9659258262890683122, 1.000000000000000000, 0.9659258262890683122, 1.000000000000000000, 0.9659258262890683122, 1.000000000000000000, 0.9659258262890683122, 1.000000000000000000, 0.9659258262890683122, 1.000000000000000000, 0.9659258262890683122, 1.000000000000000000, 0.9659258262890683122, 1.000000000000000000, 0.9659258262890683122, 1.000000000000000000, 0.9659258262890683122, 1.000000000000000000, 0.9659258262890683122, 1.000000000000000000, 0.9659258262890683122, 1.000000000000000000, 0.9659258262890683122, 1.000000000000000000, 0.9659258262890683122, 1.000000000000000000, 0.9659258262890683122, 1.000000000000000000, 0.9659258262890683122, 1.000000000000000000, 0.9659258262890683122, 1.000000000000000000, 0.9659258262890683122, 1.000000000000000000, 0.9659258262890683122, 1.000000000000000000, 0.9659258262890683122, 1.000000000000000000, 0.9659258262890683122, 1.000000000000000000, 0.9659258262890683122, 1.000000000000000000, 0.9659258262890683122, 1.000000000000000000, 0.9659258262890683122, 1.000000000000000000, 0.9659258262890683122, 1.000000000000000000, 0.9659258262890683122, 1.000000000000000000, 0.9659258262890683122, 1.000000000000000000, 0.9659258262890683122, 1.000000000000000000, 0.9659258262890683122, 1.000000000000000000, 0.9659258262890683122, 1.000000000000000000, 0.9659258262890683122, 1.000000000000000000, 0.9659258262890683122, 1.000000000000000000, 0.9659258262890683122, 1.000000000000000000, 0.9659258262890683122, 1.000000000000000000, 0.9659258262890683122, 1.000000000000000000, 0.9659258262890683122, 1.000000000000000000, 0.9659258262890683122, 1.000000000000000000, 0.9659258262890683122, 1.000000000000000000, 0.9659258262890683122, 1.000000000000000000, 0.9659258262890683122, 1.000000000000000000, 0.9659258262890683122, 1.000000000000000000, 0.9659258262890683122, 1.000000000000000000, 0.9659258262890683122, 1.000000000000000000, 0.9659258262890683122, 1.000000000000000000, 0.9659258262890683122, 1.000000000000000000, 0.9659258262890683122, 1.000000000000000000, 0.9659258262890683122, 1.000000000000000000, 0.9659258262890683122, 1.000000000000000000, 0.9659258262890683122, 1.000000000000000000, 0.9659258262890683122, 1.000000000000000000, 0.9659258262890683122, 1.000000000000000000, 0.9659258262890683122, 1.000000000000000000, 0.9659258262890683122, 1.000000000000000000, 0.9659258262890683122, 1.000000000000000000, 0.9659258262890683122, 1.000000000000000000, 0.9659258262890683122, 1.000000000000000000, 0.9659258262890683122, 1.000000000000000000, 0.9659258262890683122, 1.000000000000000000, 0.9659258262890683122, 1.000000000000000000, 0.9659258262890683122, 1.000000000000000000, 0.9659258262890683122, 1.000000000000000000, 0.9659258262890683122, 1.000000000000000000, 0.9659258262890683122, 1.000000000000000000, 0.9659258262890683122, 1.000000000000000000, 0.9659258262890683122, 1.000000000000000000, 0.9659258262890683122, 1.000000000000000000, 0.9659258262890683122, 1.000000000000000000, 0.9659258262890683122, 1.000000000000000000, 0.9659258262890683122, 1.000000000000000000, 0.9659258262890683122, 1.000000000000000000, 0.9659258262890683122, 1.000000000000000000, 0.9659258262890683122, 1.000000000000000000, 0.9659258262890683122, 1.000000000000000000, 0.9659258262890683122, 1.000000000000000000, 0.9659258262890683122, 1.000000000000000000, 0.9659258262890683122, 1.000000000000000000, 0.9659258262890683122, 1.000000000000000000, 0.9659258262890683122, 1.000000000000000000, 0.9659258262890683122, 1.000000000000000000, 0.9659258262890683122, 1.000000000000000000, 0.9659258262890683122, 1.000000000000000000, 0.9659258262890683122, 1.000000000000000000, 0.9659258262890683122, 1.000000000000000000, 0.9659258262890683122, 1.000000000000000000, 0.9659258262890683122, 1.000000000000000000, 0.9659258262890683122, 1.000000000000000000, 0.9659258262890683122, 1.000000000000000000, 0.9659258262890683122, 1.000000000000000000, 0.9659258262890683122, 1.000000000000000000, 0.9659258262890683122, 1.000000000000000000, 0.9659258262890683122, 1.000000000000000000, 0.9659258262890683122, 1.000000000000000000, 0.9659258262890683122, 1.000000000000000000, 0.9659258262890683122, 1.000000000000000000, 0.9659258262890683122, 1.000000000000000000, 0.9659258262890683122, 1.000000000000000000, 0.9659258262890683122, 1.000000000000000000, 0.9659258262890683122, 1.000000000000000000, 0.9659258262890683122, 1.000000000000000000, 0.9659258262890683122, 1.000000000000000000, 0.9659258262890683122, 1.000000000000000000, 0.9659258262890683122, 1.000000000000000000, 0.9659258262890683122, 1.000000000000000000, 0.9659258262890683122, 1.000000000000000000, 0.9659258262890683122, 1.000000000000000000, 0.9659258262890683122, 1.000000000000000000, 0.9659258262890683122, 1.000000000000000000, 0.9659258262890683122, 1.000000000000000000, 0.9659258262890683122, 1.000000000000000000, 0.9659258262890683122, 1.000000000000000000, 0.9659258262890683122, 1.000000000000000000, 0.9659258262890683122, 1.000000000000000000, 0.9659258262890683122, 1.000000000000000000, 0.9659258262890683122, 1.000000000000000000, 0.9659258262890683122, 1.000000000000000000, 0.9659258262890683122, 1.000000000000000000, 0.9659258262890683122, 1.000000000000000000, 0.9659258262890683122, 1.000000000000000000, 0.9659258262890683122, 1.000000000000000000, 0.9659258262890683122, 1.000000000000000000, 0.9659258262890683122, 1.000000000000000000, 0.9659258262890683122, 1.000000000000000000, 0.9659258262890683122, 1.000000000000000000, 0.9659258262890683122, 1.000000000000000000, 0.9659258262890683122, 1.000000000000000000, 0.9659258262890683122, 1.000000000000000000, 0.9659258262890683122, 1.000000000000000000, 0.9659258262890683122, 1.000000000000000000, 0.9659258262890683122, 1.000000000000000000, 0.9659258262890683122, 1.000000000000000000, 0.9659258262890683122, 1.000000000000000000, 0.9659258262890683122, 1.000000000000000000, 0.9659258262890683122, 1.000000000000000000, 0.9659258262890683122, 1.000000000000000000, 0.9659258262890683122, 1.000000000000000000, 0.9659258262890683122, 1.000000000000000000, 0.9659258262890683122, 1.000000000000000000, 0.9659258262890683122, 1.000000000000000000, 0.9659258262890683122, 1.000000000000000000, 0.9659258262890683122, 1.000000000000000000, 0.9659258262890683122, 1.000000000000000000, 0.9659258262890683122, 1.000000000000000000, 0.9659258262890683122, 1.000000000000000000, 0.9659258262890683122, 1.000000000000000000, 0.9659258262890683122, 1.000000000000000000, 0.9659258262890683122, 1.000000000000000000, 0.9659258262890683122, 1.000000000000000000, 0.9659258262890683122, 1.000000000000000000, 0.9659258262890683122, 1.000000000000000000, 0.9659258262890683122, 1.000000000000000000, 0.9659258262890683122, 1.000000000000000000, 0.9659258262890683122, 1.000000000000000000, 0.9659258262890683122, 1.000000000000000000, 0.9659258262890683122, 1.000000000000000000, 0.9659258262890683122, 1.000000000000000000, 0.9659258262890683122, 1.000000000000000000, 0.9659258262890683122, 1.000000000000000000, 0.9659258262890683122, 1.000000000000000000, 0.9659258262890683122, 1.000000000000000000, 0.9659258262890683122, 1.000000000000000000, 0.9659258262890683122, 1.000000000000000000, 0.9659258262890683122, 1.000000000000000000) ) ) 
 REPRESENTATION_ITEM ( '' )  SURFACE ( )  );
#46069=CARTESIAN_POINT ( 'NONE',  ( 0.3392501089628018329, -0.1958661417322834497, -0.6574609991787909724 ) ) ;
#46073=CARTESIAN_POINT ( 'NONE',  ( -0.1958661417322834220, -0.3392501089628018884, -1.095144356955380704 ) ) ;
#46079=CARTESIAN_POINT ( 'NONE',  ( 0.3917322834645670659, -0.1049643490035303273, 0.04919328264335768447 ) ) ;
#46082=CARTESIAN_POINT ( 'NONE',  ( -0.3458507752293909498, 0.3458507752293907833, -1.356299212598425230 ) ) ;
#46099=CARTESIAN_POINT ( 'NONE',  ( 0.1998031496062994128, -0.3460692066303957537, -2.530839895013123453 ) ) ;
#46103=CARTESIAN_POINT ( 'NONE',  ( 0.1070741851644053388, 0.3996062992125986035, -1.959973753280839892 ) ) ;
#46109=CARTESIAN_POINT ( 'NONE',  ( 0.3460692066303959202, -0.1998031496062991630, -1.126640419947506633 ) ) ;
#46110=CARTESIAN_POINT ( 'NONE',  ( -0.1998031496062994683, 0.3460692066303958092, -1.430446194225721834 ) ) ;
#46111=CARTESIAN_POINT ( 'NONE',  ( -0.3949938075777409963, -7.255918531996591613E-17, -0.8267716535433070613 ) ) ;
#46118=CARTESIAN_POINT ( 'NONE',  ( 0.1974969037888706092, -0.3420746716998660508, -1.743438320209973913 ) ) ;
#46123=CARTESIAN_POINT ( 'NONE',  ( -0.4091458600556405756, 0.2362204724409446288, -2.073490813648294129 ) ) ;
#46124=CARTESIAN_POINT ( 'NONE',  ( 0.1208384647389237204, -0.3726288332213487653, -2.755905511811024056 ) ) ;
#46131=CARTESIAN_POINT ( 'NONE',  ( -0.1049643490035301746, -0.3917322834645670659, -2.514416379756218678 ) ) ;
#46137=CARTESIAN_POINT ( 'NONE',  ( 0.1958661417322836162, -0.3392501089628018329, -2.691581734086927469 ) ) ;
#46139=CARTESIAN_POINT ( 'NONE',  ( 0.3917322834645670104, 2.398668435337828261E-17, -1.842519685039370136 ) ) ;
#46141=ORIENTED_EDGE ( 'NONE', *, *, #21932, .F. ) ;
#46142=CARTESIAN_POINT ( 'NONE',  ( 0.3420746716998659953, 0.1974969037888705536, -2.020997375328084100 ) ) ;
#46147=CARTESIAN_POINT ( 'NONE',  ( 0.1070741851644054915, -0.3996062992125986035, -0.7152230971128609172 ) ) ;
#46155=CARTESIAN_POINT ( 'NONE',  ( 0.3392501089628018329, 0.1958661417322835607, -0.3733595800524935338 ) ) ;
#46165=CARTESIAN_POINT ( 'NONE',  ( -0.3458507752293909498, 0.3458507752293907833, -1.122047244094488194 ) ) ;
#46167=CARTESIAN_POINT ( 'NONE',  ( 0.3917322834645670104, 2.398668435337828261E-17, -0.2677165354330708347 ) ) ;
#46168=CARTESIAN_POINT ( 'NONE',  ( 0.3392501089628018884, -0.1958661417322834220, -2.551837270341207109 ) ) ;
#46172=CARTESIAN_POINT ( 'NONE',  ( -9.787531504996566615E-17, 0.3996062992125985480, -0.2342519685039370358 ) ) ;
#46177=CARTESIAN_POINT ( 'NONE',  ( 0.1974969037888706092, -0.3420746716998660508, -2.688320209973753094 ) ) ;
#46184=CARTESIAN_POINT ( 'NONE',  ( -0.1958661417322836718, 0.3392501089628017219, -1.895013123359580165 ) ) ;
#46187=CARTESIAN_POINT ( 'NONE',  ( 0.4724409448818896462, 0.1265901696524990294, -0.04396325459317586282 ) ) ;
#46190=ADVANCED_FACE ( 'NONE', ( #63185 ), #48591, .T. ) ;
#46192=CARTESIAN_POINT ( 'NONE',  ( -0.4091458600556405756, 0.2362204724409446288, -0.7329396325459317518 ) ) ;
#46193=AXIS2_PLACEMENT_3D ( 'NONE', #51299, #31545, #71105 ) ;
#46202=CARTESIAN_POINT ( 'NONE',  ( -0.3460692066303960313, 0.1998031496062989965, -1.205380577427821454 ) ) ;
#46203=( BOUNDED_CURVE ( )  B_SPLINE_CURVE ( 2, ( #54645, #81170, #68528, #79942, #48742, #54225, #9220, #80355, #34893, #49154, #22256, #67710, #60555 ),
 .UNSPECIFIED., .F., .F. ) 
 B_SPLINE_CURVE_WITH_KNOTS ( ( 3, 2, 2, 2, 2, 2, 3 ),
 ( 0.1875000000000000000, 0.1916666666666666796, 0.1958333333333333315, 0.2000000000000000111, 0.2041666666666666907, 0.2083333333333333703, 0.2125000000000000222 ),
 .UNSPECIFIED. ) 
 CURVE ( )  GEOMETRIC_REPRESENTATION_ITEM ( )  RATIONAL_B_SPLINE_CURVE ( ( 1.000000000000000000, 0.9659258262890683122, 1.000000000000000000, 0.9659258262890683122, 1.000000000000000000, 0.9659258262890683122, 1.000000000000000000, 0.9659258262890683122, 1.000000000000000000, 0.9659258262890683122, 1.000000000000000000, 0.9659258262890680902, 1.000000000000000222 ) ) 
 REPRESENTATION_ITEM ( '' )  );
#46204=CARTESIAN_POINT ( 'NONE',  ( 0.1958661417322836440, -0.3392501089628017219, -2.538713910761154491 ) ) ;
#46211=DIRECTION ( 'NONE',  ( 1.000000000000000000, 0.000000000000000000, 0.000000000000000000 ) ) ;
#46213=CARTESIAN_POINT ( 'NONE',  ( -0.3996062992125986035, -7.340648628747425578E-17, -0.1968503937007874127 ) ) ;
#46214=CARTESIAN_POINT ( 'NONE',  ( 0.3917322834645670104, 0.1049643490035304660, -2.641095431267403537 ) ) ;
#46220=CARTESIAN_POINT ( 'NONE',  ( 0.2867679344610365999, -0.2867679344610365444, -2.387795275590551380 ) ) ;
#46225=CARTESIAN_POINT ( 'NONE',  ( -0.1070741851644051862, -0.3996062992125986590, -1.961942257217847763 ) ) ;
#46227=CARTESIAN_POINT ( 'NONE',  ( 4.893765752498283924E-17, -0.3996062992125986035, -1.496062992125984259 ) ) ;
#46229=CARTESIAN_POINT ( 'NONE',  ( -0.3917322834645669549, -0.1049643490035306603, -2.872703412073490448 ) ) ;
#46241=CARTESIAN_POINT ( 'NONE',  ( 0.3917322834645670104, 2.398668435337828261E-17, -0.7401574803149605364 ) ) ;
#46244=CARTESIAN_POINT ( 'NONE',  ( 0.2891555358219910499, 0.2891555358219910499, -0.6102362204724410821 ) ) ;
#46260=CARTESIAN_POINT ( 'NONE',  ( 0.3460692066303959202, 0.1998031496062993295, -1.391076115485564424 ) ) ;
#46262=CARTESIAN_POINT ( 'NONE',  ( -0.1070741851644056997, 0.3996062992125984925, -0.5557742782152230721 ) ) ;
#46263=CARTESIAN_POINT ( 'NONE',  ( -0.1070741851644056997, 0.3996062992125984925, -0.3982939632545932085 ) ) ;
#46265=CARTESIAN_POINT ( 'NONE',  ( 0.4091458600556404646, -0.2362204724409448231, -0.1049868766404199460 ) ) ;
#46266=CARTESIAN_POINT ( 'NONE',  ( 0.3392501089628018329, 0.1958661417322835607, -2.263123359580052618 ) ) ;
#46272=CARTESIAN_POINT ( 'NONE',  ( 0.4724409448818897572, -0.1265901696524988906, -1.920603674540682038 ) ) ;
#46275=CARTESIAN_POINT ( 'NONE',  ( -0.3949938075777408852, -0.1058382717557502933, -1.540026246719160108 ) ) ;
#46285=CARTESIAN_POINT ( 'NONE',  ( -0.3460692066303960313, 0.1998031496062989965, -2.150262467191601079 ) ) ;
#46287=CARTESIAN_POINT ( 'NONE',  ( 0.1049643490035304522, -0.3917322834645668994, -2.212579109415011569 ) ) ;
#46301=CARTESIAN_POINT ( 'NONE',  ( -0.2925321140481932369, 0.2925321140481931259, 0.06102362204724409017 ) ) ;
#46303=CARTESIAN_POINT ( 'NONE',  ( -0.3917322834645670104, -7.196005306013484475E-17, -1.541338582677165503 ) ) ;
#46315=ORIENTED_EDGE ( 'NONE', *, *, #78043, .F. ) ;
#46325=CARTESIAN_POINT ( 'NONE',  ( 0.1049643490035303689, 0.3917322834645670104, -2.347769028871391050 ) ) ;
#46328=CARTESIAN_POINT ( 'NONE',  ( -0.3996062992125986035, -0.1070741851644056997, -0.04593175853018374721 ) ) ;
#46331=CARTESIAN_POINT ( 'NONE',  ( 0.1958661417322836440, -0.3392501089628017219, -1.816272965879265122 ) ) ;
#46332=ORIENTED_EDGE ( 'NONE', *, *, #59403, .T. ) ;
#46341=CARTESIAN_POINT ( 'NONE',  ( 0.3392501089628018329, 0.1958661417322835052, -0.9986683482601557138 ) ) ;
#46347=CARTESIAN_POINT ( 'NONE',  ( 0.3917322834645670659, -0.1049643490035303273, -2.627972071687351363 ) ) ;
#46355=EDGE_CURVE ( 'NONE', #49627, #12829, #31604, .T. ) ;
#46357=CARTESIAN_POINT ( 'NONE',  ( 0.3917322834645670104, -0.1049643490035303411, -1.613517060367454237 ) ) ;
#46371=CARTESIAN_POINT ( 'NONE',  ( 0.1265901696524990294, -0.4724409448818896462, -0.1620734908136483021 ) ) ;
#46375=CARTESIAN_POINT ( 'NONE',  ( 0.3949938075777408852, 0.1058382717557500435, -0.04396325459317585588 ) ) ;
#46380=CARTESIAN_POINT ( 'NONE',  ( 4.837279021331061486E-17, -0.3949938075777409963, -0.1555118110236220486 ) ) ;
#46387=CARTESIAN_POINT ( 'NONE',  ( 0.3460692066303959202, -0.1998031496062991630, -0.8116797900262466836 ) ) ;
#46389=CARTESIAN_POINT ( 'NONE',  ( -0.2867679344610364334, -0.2867679344610367109, -0.5236220472440944462 ) ) ;
#46391=CARTESIAN_POINT ( 'NONE',  ( 0.2362204724409451007, -0.4091458600556402980, -0.4835958005249343938 ) ) ;
#46401=CARTESIAN_POINT ( 'NONE',  ( -0.3963884504522706131, -0.02578378529929505406, -1.220472440944882608 ) ) ;
#46403=CARTESIAN_POINT ( 'NONE',  ( 0.2362204724409451007, -0.4091458600556402980, -2.845800524934383624 ) ) ;
#46421=CARTESIAN_POINT ( 'NONE',  ( 0.2925321140481932369, 0.2925321140481932369, -0.9251968503937008093 ) ) ;
#46427=CARTESIAN_POINT ( 'NONE',  ( 0.1998031496062992740, 0.3460692066303959757, -2.506561679790026087 ) ) ;
#46428=CARTESIAN_POINT ( 'NONE',  ( -0.1974969037888706647, 0.3420746716998658843, -1.902887139107611869 ) ) ;
#46429=CARTESIAN_POINT ( 'NONE',  ( 0.3917322834645670104, 2.398668435337828261E-17, -0.5826771653543306728 ) ) ;
#46430=CARTESIAN_POINT ( 'NONE',  ( -0.3392501089628017219, -0.1958661417322836718, -0.8320209973753279753 ) ) ;
#46432=CARTESIAN_POINT ( 'NONE',  ( 0.3917322834645669549, 0.1049643490035304660, -0.9041994750656167090 ) ) ;
#46434=ADVANCED_FACE ( 'NONE', ( #69909 ), #26121, .T. ) ;
#46435=CARTESIAN_POINT ( 'NONE',  ( -0.1974969037888704149, -0.3420746716998661063, -2.819553805774278388 ) ) ;
#46442=CARTESIAN_POINT ( 'NONE',  ( 0.3460692066303959757, -0.1998031496062991907, -2.782152230971128848 ) ) ;
#46443=CARTESIAN_POINT ( 'NONE',  ( 0.3392501089628018884, -0.1958661417322833942, -1.204087557251655394 ) ) ;
#46449=CARTESIAN_POINT ( 'NONE',  ( 0.1958661417322834775, 0.3392501089628018884, -0.7014435695538058235 ) ) ;
#46457=CARTESIAN_POINT ( 'NONE',  ( 0.2143816077128068154, -0.3285422586328383132, -1.929133858267715551 ) ) ;
#46458=CARTESIAN_POINT ( 'NONE',  ( -0.2867679344610365999, 0.2867679344610364889, -1.901574803149606252 ) ) ;
#46460=CARTESIAN_POINT ( 'NONE',  ( 0.1070741851644054915, -0.3996062992125986035, -0.5577427821522309426 ) ) ;
#46466=CARTESIAN_POINT ( 'NONE',  ( -0.4724409448818888135, -0.1265901696525008335, -1.148293963254593431 ) ) ;
#46467=CARTESIAN_POINT ( 'NONE',  ( -0.3392501089628019995, 0.1958661417322832277, -1.370734908136483021 ) ) ;
#46485=CARTESIAN_POINT ( 'NONE',  ( 0.3392501089628018329, 0.1958661417322835052, -0.6837077183388958757 ) ) ;
#46488=CARTESIAN_POINT ( 'NONE',  ( -1.157146581871515012E-16, 0.4724409448818898682, -0.7874015748031496509 ) ) ;
#46494=CARTESIAN_POINT ( 'NONE',  ( -0.3392501089628019995, 0.1958661417322831999, 0.1344951199136988906 ) ) ;
#46498=CARTESIAN_POINT ( 'NONE',  ( -0.4091458600556405756, 0.2362204724409446288, -1.677821522309711266 ) ) ;
#46507=CARTESIAN_POINT ( 'NONE',  ( -0.1265901696524993347, 0.4724409448818896462, -2.130577427821521930 ) ) ;
#46513=CARTESIAN_POINT ( 'NONE',  ( 0.3996062992125986035, -0.1070741851644052972, -2.865485564304462329 ) ) ;
#46519=CARTESIAN_POINT ( 'NONE',  ( -0.2925321140481932369, 0.2925321140481931259, -1.671259842519685179 ) ) ;
#46526=CARTESIAN_POINT ( 'NONE',  ( 0.3996062992125985480, -0.1070741851644052972, -0.9757217847769029673 ) ) ;
#46527=CARTESIAN_POINT ( 'NONE',  ( 0.1070741851644054915, -0.3996062992125986035, -1.345144356955380704 ) ) ;
#46528=CARTESIAN_POINT ( 'NONE',  ( 0.1974969037888704704, 0.3420746716998660508, -0.4593175853018373056 ) ) ;
#46533=CARTESIAN_POINT ( 'NONE',  ( 4.837279021331061486E-17, -0.3949938075777409963, -1.730314960629921295 ) ) ;
#46538=CARTESIAN_POINT ( 'NONE',  ( 0.1265901696524990294, -0.4724409448818896462, -1.817585301837270517 ) ) ;
#46539=CARTESIAN_POINT ( 'NONE',  ( 0.2661962643027124265, -0.2881610400590444709, -2.755905511811022723 ) ) ;
#46547=CARTESIAN_POINT ( 'NONE',  ( -0.3392501089628018329, -0.1958661417322836440, -2.494731340386139529 ) ) ;
#46553=CARTESIAN_POINT ( 'NONE',  ( -0.3917322834645671215, 0.1049643490035301469, 0.1975065616797899160 ) ) ;
#46555=CARTESIAN_POINT ( 'NONE',  ( 0.1958661417322834775, 0.3392501089628018884, -1.711286089238845287 ) ) ;
#46558=CARTESIAN_POINT ( 'NONE',  ( 0.3949938075777409963, 2.418639510665530435E-17, -2.165354330708661124 ) ) ;
#46563=CARTESIAN_POINT ( 'NONE',  ( 0.1998031496062992740, 0.3460692066303959757, -0.4593175853018372501 ) ) ;
#46571=CARTESIAN_POINT ( 'NONE',  ( -0.1958661417322834220, -0.3392501089628018884, -0.3077427821522311091 ) ) ;
#46583=CARTESIAN_POINT ( 'NONE',  ( -0.2362204724409447953, -0.4091458600556404646, -1.325459317585301777 ) ) ;
#46585=CARTESIAN_POINT ( 'NONE',  ( 0.3917322834645669549, 0.1049643490035304660, -0.4317585301837270628 ) ) ;
#46587=CARTESIAN_POINT ( 'NONE',  ( -0.3392501089628019995, 0.1958661417322832277, -2.315616797900262647 ) ) ;
#46590=CIRCLE ( 'NONE', #68115, 0.4724409448818898682 ) ;
#46591=VECTOR ( 'NONE', #79812, 39.37007874015748143 ) ;
#46592=CARTESIAN_POINT ( 'NONE',  ( -0.1070741851644056997, 0.3996062992125984925, 0.07414698162729654873 ) ) ;
#46597=CARTESIAN_POINT ( 'NONE',  ( 0.3949938075777409963, 2.418639510665530743E-17, -2.872047244094488416 ) ) ;
#46604=CARTESIAN_POINT ( 'NONE',  ( 0.1049643490035304938, -0.3917322834645669549, -1.809711286089239035 ) ) ;
#46608=CARTESIAN_POINT ( 'NONE',  ( 0.4091458600556404646, -0.2362204724409448231, -0.1817585301837270351 ) ) ;
#46612=CARTESIAN_POINT ( 'NONE',  ( 0.4724409448818889246, 0.1265901696525005560, -0.6738845144356956363 ) ) ;
#46619=CARTESIAN_POINT ( 'NONE',  ( 0.4624630002188662159, 0.1438724767639667779, -1.934761428466221789 ) ) ;
#46622=CARTESIAN_POINT ( 'NONE',  ( -0.3996062992125986590, 0.1070741851644051723, -1.369422572178477404 ) ) ;
#46623=CARTESIAN_POINT ( 'NONE',  ( 0.3917322834645670104, -0.1049643490035303411, -2.715879265091863726 ) ) ;
#46631=CARTESIAN_POINT ( 'NONE',  ( 0.2925321140481932369, -0.2925321140481932369, 0.05905511811023619884 ) ) ;
#46632=CARTESIAN_POINT ( 'NONE',  ( 0.3392501089628018884, -0.1958661417322833942, -2.621410391897324832 ) ) ;
#46638=CARTESIAN_POINT ( 'NONE',  ( 0.2867679344610365999, 0.2867679344610365999, -2.427165354330708347 ) ) ;
#46647=CARTESIAN_POINT ( 'NONE',  ( 0.3460692066303959202, 0.1998031496062993295, -1.548556430446194287 ) ) ;
#46649=CARTESIAN_POINT ( 'NONE',  ( -0.3917322834645670659, -7.196005306013484475E-17, -0.5085494995088732928 ) ) ;
#46662=CARTESIAN_POINT ( 'NONE',  ( 0.1958661417322836440, -0.3392501089628017219, -0.7139107611548556331 ) ) ;
#46665=CARTESIAN_POINT ( 'NONE',  ( -0.1058382717557503211, 0.3949938075777409408, -0.6364829396325458744 ) ) ;
#46673=EDGE_CURVE ( 'NONE', #2570, #52886, #44702, .T. ) ;
#46681=CARTESIAN_POINT ( 'NONE',  ( -0.1998031496062994683, 0.3460692066303958092, -1.115485564304461885 ) ) ;
#46683=CARTESIAN_POINT ( 'NONE',  ( -9.787531504996566615E-17, 0.3996062992125985480, -0.5492125984251968740 ) ) ;
#46684=CARTESIAN_POINT ( 'NONE',  ( -0.1998031496062994405, 0.3460692066303957537, -0.7198162729658792447 ) ) ;
#46686=CARTESIAN_POINT ( 'NONE',  ( -0.2362204724409451284, 0.4091458600556402425, -0.1706036745406823985 ) ) ;
#46687=CARTESIAN_POINT ( 'NONE',  ( -0.3917322834645669549, -0.1049643490035306603, -2.177821522309711266 ) ) ;
#46693=CARTESIAN_POINT ( 'NONE',  ( 0.4091458600556404646, -0.2362204724409448231, -2.071522309711285814 ) ) ;
#46696=CARTESIAN_POINT ( 'NONE',  ( 0.1058382717557500852, -0.3949938075777408852, -1.579396325459317740 ) ) ;
#46706=CARTESIAN_POINT ( 'NONE',  ( 0.3460692066303959202, -0.1998031496062991630, -2.543963254593176071 ) ) ;
#46709=CARTESIAN_POINT ( 'NONE',  ( -0.3917322834645669549, -7.196005306013483243E-17, -2.009167035924197098 ) ) ;
#46720=CARTESIAN_POINT ( 'NONE',  ( -0.1998031496062994405, 0.3460692066303957537, 0.2250656167979002698 ) ) ;
#46722=CARTESIAN_POINT ( 'NONE',  ( -0.3917322834645670104, -7.196005306013484475E-17, -1.226377952755905776 ) ) ;
#46731=CARTESIAN_POINT ( 'NONE',  ( -0.1070741851644056997, 0.3996062992125984925, -0.8707349081364830212 ) ) ;
#46744=CARTESIAN_POINT ( 'NONE',  ( 0.2867679344610366554, -0.2867679344610365444, -2.295275590551181022 ) ) ;
#46747=CARTESIAN_POINT ( 'NONE',  ( -0.1998031496062991907, -0.3460692066303959757, -0.3805774278215223183 ) ) ;
#46750=CARTESIAN_POINT ( 'NONE',  ( -0.3392501089628019995, 0.1958661417322832277, -2.380577427821522374 ) ) ;
#46761=CARTESIAN_POINT ( 'NONE',  ( 0.2867679344610365999, -0.2867679344610365999, -0.9658599493100242794 ) ) ;
#46768=CARTESIAN_POINT ( 'NONE',  ( -0.1049643490035302301, -0.3917322834645671770, -2.431121677986564311 ) ) ;
#46778=CARTESIAN_POINT ( 'NONE',  ( -0.3917322834645670104, -7.196005306013484475E-17, -2.013779527559055094 ) ) ;
#46786=CARTESIAN_POINT ( 'NONE',  ( -0.3460692066303958092, -0.1998031496062994683, -1.784776902887138972 ) ) ;
#46791=CARTESIAN_POINT ( 'NONE',  ( -0.3458507752293906723, -0.3458507752293910609, -0.6082677165354329896 ) ) ;
#46794=CARTESIAN_POINT ( 'NONE',  ( 0.3420746716998660508, 0.1974969037888705814, -0.05052493438320211638 ) ) ;
#46799=CARTESIAN_POINT ( 'NONE',  ( -0.3949938075777409963, -7.255918531996591613E-17, -0.4311023622047245318 ) ) ;
#46806=CARTESIAN_POINT ( 'NONE',  ( 0.1998031496062994128, -0.3460692066303957537, -1.270997375328084100 ) ) ;
#46808=CARTESIAN_POINT ( 'NONE',  ( -0.3392501089628019995, 0.1958661417322832277, -0.4908136482939632339 ) ) ;
#46822=CARTESIAN_POINT ( 'NONE',  ( -0.3458507752293909498, 0.3458507752293907833, -2.773622047244094002 ) ) ;
#46838=CARTESIAN_POINT ( 'NONE',  ( -0.3460692066303960868, 0.1998031496062990242, -0.9711286089238845287 ) ) ;
#46839=CARTESIAN_POINT ( 'NONE',  ( 0.3460692066303959202, -0.1998031496062991630, -2.858923884514435798 ) ) ;
#46842=CARTESIAN_POINT ( 'NONE',  ( -0.1998031496062994683, 0.3460692066303958092, -2.532808398950130879 ) ) ;
#46843=CARTESIAN_POINT ( 'NONE',  ( 0.1058382717557499880, 0.3949938075777411073, -1.725721784776902856 ) ) ;
#46844=CARTESIAN_POINT ( 'NONE',  ( 0.1049643490035303689, 0.3917322834645670104, -0.6154855643044617741 ) ) ;
#46847=CARTESIAN_POINT ( 'NONE',  ( 0.3392501089628018884, -0.1958661417322834220, -1.041994750656167756 ) ) ;
#46849=CARTESIAN_POINT ( 'NONE',  ( -9.594673741351310580E-17, 0.3917322834645669549, 0.07744713730414881647 ) ) ;
#46856=CARTESIAN_POINT ( 'NONE',  ( -0.3996062992125987146, 0.1070741851644051862, -2.552493438320210029 ) ) ;
#46857=CARTESIAN_POINT ( 'NONE',  ( 0.2867679344610366554, -0.2867679344610365999, -1.197525877461629307 ) ) ;
#46862=CARTESIAN_POINT ( 'NONE',  ( -9.594673741351313045E-17, 0.3917322834645670104, -0.5570866141732284671 ) ) ;
#46870=CARTESIAN_POINT ( 'NONE',  ( -0.1789624962996142488, -0.3486222174635806859, -1.929133858267717549 ) ) ;
#46871=CARTESIAN_POINT ( 'NONE',  ( 0.3917322834645669549, 0.1049643490035304660, -1.849081364829396223 ) ) ;
#46873=CARTESIAN_POINT ( 'NONE',  ( -0.3996062992125986035, -0.1070741851644056997, -0.5183727034120735322 ) ) ;
#46879=CARTESIAN_POINT ( 'NONE',  ( 0.3970677821444033584, 0.02963302784745526844, -1.929133858267716439 ) ) ;
#46880=CARTESIAN_POINT ( 'NONE',  ( -0.2867679344610364334, -0.2867679344610367109, -1.088582677165354173 ) ) ;
#46882=CARTESIAN_POINT ( 'NONE',  ( -0.3990339831393152625, -0.0003067303410125883515, -1.929133858267716217 ) ) ;
#46901=CARTESIAN_POINT ( 'NONE',  ( 0.3917322834645669549, 2.398668435337827645E-17, -1.300505618601362601 ) ) ;
#46910=CARTESIAN_POINT ( 'NONE',  ( -0.1049643490035307158, 0.3917322834645670104, -0.003300155676852285953 ) ) ;
#46914=CARTESIAN_POINT ( 'NONE',  ( 0.4724409448818898682, 2.892866454678787531E-17, -1.454724409448818756 ) ) ;
#46929=EDGE_LOOP ( 'NONE', ( #7001, #7848, #671, #9621 ) ) ;
#46931=CARTESIAN_POINT ( 'NONE',  ( 0.1070741851644053388, 0.3996062992125986035, -2.747375328083988766 ) ) ;
#46936=CARTESIAN_POINT ( 'NONE',  ( 0.3460692066303958092, 0.1998031496062993018, -1.625328083989501460 ) ) ;
#46942=CARTESIAN_POINT ( 'NONE',  ( 0.1998031496062992740, 0.3460692066303959757, -1.561679790026246684 ) ) ;
#46943=CARTESIAN_POINT ( 'NONE',  ( -0.1058382717557497937, -0.3949938075777411628, -0.5446194225721784354 ) ) ;
#46944=CARTESIAN_POINT ( 'NONE',  ( -9.594673741351313045E-17, 0.3917322834645670104, -0.1496062992125983815 ) ) ;
#46948=CARTESIAN_POINT ( 'NONE',  ( 0.3949938075777408852, 0.1058382717557500435, -1.776246719160105236 ) ) ;
#46952=CARTESIAN_POINT ( 'NONE',  ( 0.3458507752293908943, 0.3458507752293908943, -2.185039370078739829 ) ) ;
#46953=CARTESIAN_POINT ( 'NONE',  ( 0.3788256970788764222, -0.1002886991238087361, -2.755905511811022279 ) ) ;
#46960=CARTESIAN_POINT ( 'NONE',  ( -0.1958661417322836440, 0.3392501089628016664, -2.455361261645982562 ) ) ;
#46967=CARTESIAN_POINT ( 'NONE',  ( 0.3917322834645669549, 2.398668435337827645E-17, -2.717828453247031817 ) ) ;
#46969=CARTESIAN_POINT ( 'NONE',  ( -0.3917322834645670104, -7.196005306013484475E-17, -1.921259842519684957 ) ) ;
#46972=CARTESIAN_POINT ( 'NONE',  ( -9.674558042662121740E-17, 0.3949938075777409963, -2.204724409448819422 ) ) ;
#46977=CARTESIAN_POINT ( 'NONE',  ( -9.787531504996567848E-17, 0.3996062992125986035, -0.7874015748031496509 ) ) ;
#46982=CARTESIAN_POINT ( 'NONE',  ( 0.1958661417322834775, 0.3392501089628018884, -0.07152230971128617498 ) ) ;
#46984=CARTESIAN_POINT ( 'NONE',  ( 0.1958661417322836440, -0.3392501089628017219, -0.8064304461942258806 ) ) ;
#46989=CARTESIAN_POINT ( 'NONE',  ( -0.1049643490035307020, 0.3917322834645669549, 0.001312335958005294862 ) ) ;
#46996=CARTESIAN_POINT ( 'NONE',  ( -1.157146581871515012E-16, 0.4724409448818898682, -1.417322834645669216 ) ) ;
#46998=CARTESIAN_POINT ( 'NONE',  ( -0.1958661417322834220, -0.3392501089628018884, -0.5301837270341206443 ) ) ;
#46999=CARTESIAN_POINT ( 'NONE',  ( -0.1049643490035307020, 0.3917322834645669549, -2.610892388451443669 ) ) ;
#47002=CARTESIAN_POINT ( 'NONE',  ( 0.3996062992125984925, 0.1070741851644054637, -0.2014435695538057958 ) ) ;
#47007=CARTESIAN_POINT ( 'NONE',  ( -0.1049643490035306742, 0.3917322834645668994, 0.07088545751412257678 ) ) ;
#47009=CARTESIAN_POINT ( 'NONE',  ( 0.3917322834645670104, 2.398668435337828261E-17, -0.04527559055118119541 ) ) ;
#47014=CARTESIAN_POINT ( 'NONE',  ( -0.1049643490035302024, -0.3917322834645671215, -1.954068241469816503 ) ) ;
#47019=CARTESIAN_POINT ( 'NONE',  ( 0.3458507752293908943, 0.3458507752293908943, -0.2145669291338583029 ) ) ;
#47028=FACE_OUTER_BOUND ( 'NONE', #61352, .T. ) ;
#47032=CARTESIAN_POINT ( 'NONE',  ( -0.2925321140481930149, -0.2925321140481933480, -1.395669291338582196 ) ) ;
#47040=CARTESIAN_POINT ( 'NONE',  ( 0.1998031496062994128, -0.3460692066303957537, -0.01115485564304463835 ) ) ;
#47042=CARTESIAN_POINT ( 'NONE',  ( 0.3996062992125986590, -0.1070741851644053111, -0.1115485564304461857 ) ) ;
#47043=CARTESIAN_POINT ( 'NONE',  ( -0.3917322834645670659, -7.196005306013484475E-17, -2.713273908957691827 ) ) ;
#47049=CARTESIAN_POINT ( 'NONE',  ( -0.3917322834645669549, -0.1049643490035306603, -2.492782152230970993 ) ) ;
#47057=CARTESIAN_POINT ( 'NONE',  ( 0.3917322834645670659, -0.1049643490035303273, -0.4232476622385321074 ) ) ;
#47071=CARTESIAN_POINT ( 'NONE',  ( -0.2867679344610365999, 0.2867679344610364889, -0.7992125984251968740 ) ) ;
#47074=CARTESIAN_POINT ( 'NONE',  ( 0.3420746716998659953, 0.1974969037888705536, -1.076115485564304475 ) ) ;
#47091=CARTESIAN_POINT ( 'NONE',  ( 0.1998031496062992740, 0.3460692066303959757, -1.876640419947506411 ) ) ;
#47093=CARTESIAN_POINT ( 'NONE',  ( 0.2925321140481932369, 0.2925321140481932369, -1.159448818897637734 ) ) ;
#47094=CARTESIAN_POINT ( 'NONE',  ( 0.3460692066303958092, 0.1998031496062993018, -0.3654855643044619407 ) ) ;
#47096=CARTESIAN_POINT ( 'NONE',  ( 0.3996062992125986035, 2.446882876249141962E-17, -2.952755905511811108 ) ) ;
#47098=CARTESIAN_POINT ( 'NONE',  ( 0.2867679344610365999, -0.2867679344610365444, -1.915354330708661124 ) ) ;
#47104=CARTESIAN_POINT ( 'NONE',  ( 0.4091458600556403535, 0.2362204724409449896, -2.097769028871391050 ) ) ;
#47107=CARTESIAN_POINT ( 'NONE',  ( -0.3949938075777408852, -0.1058382717557502933, -1.382545931758530688 ) ) ;
#47118=CARTESIAN_POINT ( 'NONE',  ( -0.1070741851644056997, 0.3996062992125984925, -2.445538057742782101 ) ) ;
#47119=CARTESIAN_POINT ( 'NONE',  ( -0.3917322834645668994, -0.1049643490035306742, -2.015728715714224517 ) ) ;
#47131=CARTESIAN_POINT ( 'NONE',  ( -0.3996062992125985480, -7.340648628747423112E-17, -0.1161417322834645827 ) ) ;
#47133=CARTESIAN_POINT ( 'NONE',  ( 4.797336870675656522E-17, -0.3917322834645670104, -1.423228346456693050 ) ) ;
#47143=CARTESIAN_POINT ( 'NONE',  ( 0.3996062992125984925, 0.1070741851644054637, -1.146325459317585116 ) ) ;
#47149=CARTESIAN_POINT ( 'NONE',  ( 0.3990339831394616454, 0.0003067303408301115422, -1.220472440944881720 ) ) ;
#47158=CARTESIAN_POINT ( 'NONE',  ( -0.2925321140481930704, -0.2925321140481933480, -0.3740157480314960092 ) ) ;
#47161=CARTESIAN_POINT ( 'NONE',  ( 0.1958661417322836440, -0.3392501089628017219, -2.131233595800524849 ) ) ;
#47173=CARTESIAN_POINT ( 'NONE',  ( -0.1958661417322834497, -0.3392501089628018884, -1.562972810202412521 ) ) ;
#47179=CARTESIAN_POINT ( 'NONE',  ( -0.3949938075777411628, 0.1058382717557497937, 0.1246719160104986374 ) ) ;
#47188=CARTESIAN_POINT ( 'NONE',  ( -0.1958661417322836718, 0.3392501089628017219, -1.672572178477690352 ) ) ;
#47192=CARTESIAN_POINT ( 'NONE',  ( -0.1011035889004385513, 0.3790285851608858336, 9.764066473168825796E-18 ) ) ;
#47196=CARTESIAN_POINT ( 'NONE',  ( 0.1070741851644053388, 0.3996062992125986035, 0.08727034120734905587 ) ) ;
#47198=CARTESIAN_POINT ( 'NONE',  ( 0.3996062992125986035, 0.1070741851644054776, -2.014435695538057569 ) ) ;
#47204=CARTESIAN_POINT ( 'NONE',  ( -0.4724409448818898682, -8.678599364036362592E-17, -0.5885826771653542844 ) ) ;
#47207=CARTESIAN_POINT ( 'NONE',  ( -0.3949938075777411073, 0.1058382717557497660, -0.2670603674540682482 ) ) ;
#47212=CARTESIAN_POINT ( 'NONE',  ( -0.3949938075777409963, -7.255918531996591613E-17, -0.5885826771653542844 ) ) ;
#47216=CARTESIAN_POINT ( 'NONE',  ( 0.4091458600556404646, -0.2362204724409448231, -0.1817585301837270351 ) ) ;
#47220=CARTESIAN_POINT ( 'NONE',  ( -0.2925321140481932369, 0.2925321140481931259, -1.513779527559055094 ) ) ;
#47222=CARTESIAN_POINT ( 'NONE',  ( -0.3392501089628019995, 0.1958661417322832277, -1.278215223097112885 ) ) ;
#47235=CARTESIAN_POINT ( 'NONE',  ( 0.4724409448818897572, -0.1265901696524988906, -2.865485564304462329 ) ) ;
#47252=CARTESIAN_POINT ( 'NONE',  ( -0.2925321140481932369, 0.2925321140481931814, -0.8070866141732283561 ) ) ;
#47256=CARTESIAN_POINT ( 'NONE',  ( -0.1070741851644051862, -0.3996062992125987146, -2.591863517060367439 ) ) ;
#47257=CARTESIAN_POINT ( 'NONE',  ( 0.3420746716998660508, -0.1974969037888703871, -2.309711286089239035 ) ) ;
#47259=CARTESIAN_POINT ( 'NONE',  ( -0.1958661417322836718, 0.3392501089628017219, -0.9501312335958004285 ) ) ;
#47263=CARTESIAN_POINT ( 'NONE',  ( 0.3917322834645670104, -0.1049643490035303411, -1.206036745406823707 ) ) ;
#47265=CARTESIAN_POINT ( 'NONE',  ( 0.2867679344610365999, -0.2867679344610365999, -0.3359386894675047142 ) ) ;
#47270=CARTESIAN_POINT ( 'NONE',  ( -1.157146581871515012E-16, 0.4724409448818898682, -0.07677165354330710290 ) ) ;
#47272=CARTESIAN_POINT ( 'NONE',  ( 0.1958661417322836718, -0.3392501089628017219, -1.820885457514122452 ) ) ;
#47278=CARTESIAN_POINT ( 'NONE',  ( 4.797336870675656522E-17, -0.3917322834645670104, -0.6358267716535433989 ) ) ;
#47287=CARTESIAN_POINT ( 'NONE',  ( -0.3458507752293909498, 0.3458507752293908388, -0.5688976377952755792 ) ) ;
#47288=CARTESIAN_POINT ( 'NONE',  ( 0.1958661417322834775, 0.3392501089628018884, -2.183727034120734878 ) ) ;
#47290=CARTESIAN_POINT ( 'NONE',  ( -0.3460692066303958092, -0.1998031496062994683, -0.5249343832020997302 ) ) ;
#47297=CARTESIAN_POINT ( 'NONE',  ( 0.1958661417322834775, 0.3392501089628018884, -1.173884514435695525 ) ) ;
#47298=CARTESIAN_POINT ( 'NONE',  ( -0.3996062992125985480, -7.340648628747423112E-17, -1.848425196850393526 ) ) ;
#47309=CARTESIAN_POINT ( 'NONE',  ( -0.3392501089628019995, 0.1958661417322832277, 0.1391076115485564701 ) ) ;
#47317=CARTESIAN_POINT ( 'NONE',  ( -0.3392501089628019439, 0.1958661417322832554, -1.366122416501625469 ) ) ;
#47326=CARTESIAN_POINT ( 'NONE',  ( -0.3392501089628019995, 0.1958661417322831999, -0.02298519504693102150 ) ) ;
#47331=CARTESIAN_POINT ( 'NONE',  ( 0.4091458600556404646, -0.2362204724409448231, -1.599081364829396223 ) ) ;
#47348=CARTESIAN_POINT ( 'NONE',  ( -0.3996062992125986590, 0.1070741851644051723, -2.786745406824146620 ) ) ;
#47353=CARTESIAN_POINT ( 'NONE',  ( -0.2925321140481930149, -0.2925321140481933480, -1.868110236220472675 ) ) ;
#47358=CARTESIAN_POINT ( 'NONE',  ( -0.3996062992125984925, -0.1070741851644056719, -0.9101049868766404316 ) ) ;
#47359=CARTESIAN_POINT ( 'NONE',  ( 0.3996062992125986035, 2.446882876249141962E-17, -1.220472440944881942 ) ) ;
#47360=CARTESIAN_POINT ( 'NONE',  ( 0.3949938075777409408, 0.1058382717557500574, -0.9120734908136481911 ) ) ;
#47361=CARTESIAN_POINT ( 'NONE',  ( 0.1070741851644053527, 0.3996062992125986590, -2.670603674540682260 ) ) ;
#47362=CARTESIAN_POINT ( 'NONE',  ( -0.2867679344610366554, 0.2867679344610365444, -0.1692913385826771144 ) ) ;
#47366=CARTESIAN_POINT ( 'NONE',  ( -0.3949938075777408852, -0.1058382717557502933, -1.697506561679790194 ) ) ;
#47371=CARTESIAN_POINT ( 'NONE',  ( -0.2362204724409451284, 0.4091458600556402425, -2.060367454068241511 ) ) ;
#47379=CARTESIAN_POINT ( 'NONE',  ( -0.1958661417322834497, -0.3392501089628018884, -2.350374385005562505 ) ) ;
#47382=CARTESIAN_POINT ( 'NONE',  ( -0.4724409448818898682, -8.678599364036362592E-17, -2.401574803149606474 ) ) ;
#47386=CARTESIAN_POINT ( 'NONE',  ( 0.3917322834645668994, -0.1049643490035303134, -2.868747088417636704 ) ) ;
#47388=CARTESIAN_POINT ( 'NONE',  ( -0.1958661417322834220, -0.3392501089628018884, -1.947506561679789971 ) ) ;
#47391=CARTESIAN_POINT ( 'NONE',  ( -0.3420746716998661618, 0.1974969037888702206, -2.230971128608923770 ) ) ;
#47396=CARTESIAN_POINT ( 'NONE',  ( -0.3460692066303960868, 0.1998031496062990242, -0.4986876640419947715 ) ) ;
#47402=CARTESIAN_POINT ( 'NONE',  ( -0.1958661417322836718, 0.3392501089628017219, 0.05971128608923875758 ) ) ;
#47403=VECTOR ( 'NONE', #12642, 39.37007874015748143 ) ;
#47409=CARTESIAN_POINT ( 'NONE',  ( -0.3917322834645671215, 0.1049643490035301469, -0.02493438320209968861 ) ) ;
#47413=CARTESIAN_POINT ( 'NONE',  ( 0.4724409448818897572, -0.1265901696524988906, -1.371391076115485053 ) ) ;
#47415=CARTESIAN_POINT ( 'NONE',  ( -0.3392501089628019995, 0.1958661417322832277, -0.6482939632545930975 ) ) ;
#47416=CARTESIAN_POINT ( 'NONE',  ( -0.2867679344610364334, -0.2867679344610367109, -2.348425196850393970 ) ) ;
#47419=CARTESIAN_POINT ( 'NONE',  ( 0.2925321140481932369, -0.2925321140481931814, -0.01771653543307089712 ) ) ;
#47424=CARTESIAN_POINT ( 'NONE',  ( -0.2867679344610364334, -0.2867679344610368219, 0.1758723341545424812 ) ) ;
#47431=CARTESIAN_POINT ( 'NONE',  ( -0.1049643490035307020, 0.3917322834645669549, -1.730971128608923992 ) ) ;
#47435=CARTESIAN_POINT ( 'NONE',  ( -0.4091458600556405756, 0.2362204724409446288, -0.4179790026246719137 ) ) ;
#47446=CARTESIAN_POINT ( 'NONE',  ( -0.2925321140481930149, -0.2925321140481933480, -1.710629921259842812 ) ) ;
#47453=B_SPLINE_CURVE_WITH_KNOTS ( 'NONE', 3,
 ( #22808, #23213, #3870, #67023, #3041, #22400, #48883, #28706, #29529, #10190, #16513, #60691, #42156, #60282, #16094, #36262, #54368, #17341, #81310, #21979, #35858, #55599, #53950, #67433, #3454, #23624, #79663, #9767, #74583, #29121, #42970, #61931, #80080, #74996, #47641, #68666, #49295, #67851 ),
 .UNSPECIFIED., .F., .F.,
 ( 4, 2, 2, 2, 2, 2, 2, 2, 2, 2, 2, 2, 2, 2, 2, 2, 2, 2, 4 ),
 ( 0.000000000000000000, 0.003207193274590009260, 0.004810789911885013891, 0.006414386549180018521, 0.007216184867827522137, 0.008017983186475025753, 0.009621579823770036455, 0.01042337814241754181, 0.01122517646106504716, 0.01282877309836005786, 0.01363057141700756147, 0.01443236973565506683, 0.01603596637295007926, 0.01763956301024508649, 0.01924315964754010067, 0.02084675628483511137, 0.02245035292213012207, 0.02405394955942513277, 0.02565754619672014347 ),
 .UNSPECIFIED. ) ;
#47456=CARTESIAN_POINT ( 'NONE',  ( -0.1070741851644051862, -0.3996062992125987146, -0.07217847769028871985 ) ) ;
#47457=CARTESIAN_POINT ( 'NONE',  ( -0.3917322834645670104, -0.1049643490035307020, -2.404874958826459075 ) ) ;
#47459=EDGE_CURVE ( 'NONE', #53683, #35624, #36613, .T. ) ;
#47461=CARTESIAN_POINT ( 'NONE',  ( -0.4724409448818898682, 5.785732909357575061E-17, -2.755905511811024056 ) ) ;
#47463=CARTESIAN_POINT ( 'NONE',  ( 0.1958661417322834775, 0.3392501089628018884, -2.591207349081364519 ) ) ;
#47469=CARTESIAN_POINT ( 'NONE',  ( -0.4724409448818899238, 0.1265901696524986686, -0.6627296587926508886 ) ) ;
#47470=CARTESIAN_POINT ( 'NONE',  ( 0.1998031496062994405, -0.3460692066303958092, -1.981627296587926690 ) ) ;
#47473=CARTESIAN_POINT ( 'NONE',  ( 0.3917322834645670659, -0.1049643490035303273, -0.2657673472779021884 ) ) ;
#47486=EDGE_CURVE ( 'NONE', #23063, #5054, #7628, .T. ) ;
#47487=CARTESIAN_POINT ( 'NONE',  ( 0.3917322834645670104, -0.1049643490035303411, -0.5761154855643042527 ) ) ;
#47490=CARTESIAN_POINT ( 'NONE',  ( 0.2891555358219910499, -0.2891555358219909944, -1.200787401574803237 ) ) ;
#47500=CARTESIAN_POINT ( 'NONE',  ( 0.4724409448818898127, -0.1265901696524988629, -1.056430446194225770 ) ) ;
#47507=CARTESIAN_POINT ( 'NONE',  ( -0.3996062992125986035, -7.340648628747425578E-17, -1.614173228346456712 ) ) ;
#47510=CARTESIAN_POINT ( 'NONE',  ( 0.3996062992125984925, 0.1070741851644054637, -1.303805774278215202 ) ) ;
#47511=CARTESIAN_POINT ( 'NONE',  ( -0.1998031496062994405, 0.3460692066303957537, -0.5623359580052492701 ) ) ;
#47513=CARTESIAN_POINT ( 'NONE',  ( 0.4724409448818896462, 0.1265901696524990294, 0.03280839895013123314 ) ) ;
#47514=CARTESIAN_POINT ( 'NONE',  ( -0.3392501089628019995, 0.1958661417322832277, -2.473097112860892288 ) ) ;
#47520=CARTESIAN_POINT ( 'NONE',  ( -0.4724409448818899238, 0.1265901696524986686, -1.841863517060367439 ) ) ;
#47524=CARTESIAN_POINT ( 'NONE',  ( -0.1974969037888704149, -0.3420746716998661063, -1.717191601049868677 ) ) ;
#47534=CARTESIAN_POINT ( 'NONE',  ( 0.2925321140481932369, 0.2925321140481932369, -2.419291338582676865 ) ) ;
#47535=CARTESIAN_POINT ( 'NONE',  ( -9.594673741351310580E-17, 0.3917322834645669549, -2.284757587105299859 ) ) ;
#47549=CARTESIAN_POINT ( 'NONE',  ( 0.1998031496062994128, -0.3460692066303957537, -0.4835958005249343938 ) ) ;
#47551=CARTESIAN_POINT ( 'NONE',  ( 0.1958661417322834775, 0.3392501089628018884, -1.646325459317585338 ) ) ;
#47559=CARTESIAN_POINT ( 'NONE',  ( -0.1998031496062991630, -0.3460692066303959202, -0.7723097112860892732 ) ) ;
#47566=CARTESIAN_POINT ( 'NONE',  ( 0.3981765293560903807, 0.002049465651542591027, -1.220472440944881720 ) ) ;
#47575=CARTESIAN_POINT ( 'NONE',  ( -0.1070741851644056997, 0.3996062992125986035, -0.4790026246719158998 ) ) ;
#47576=EDGE_LOOP ( 'NONE', ( #16246, #60013, #51948, #37659 ) ) ;
#47579=CARTESIAN_POINT ( 'NONE',  ( 0.1049643490035304938, -0.3917322834645669549, -2.282152230971128404 ) ) ;
#47580=ORIENTED_EDGE ( 'NONE', *, *, #1832, .T. ) ;
#47590=CARTESIAN_POINT ( 'NONE',  ( -0.1958661417322834497, -0.3392501089628018884, -1.720453125163043051 ) ) ;
#47596=CARTESIAN_POINT ( 'NONE',  ( 0.3392501089628018884, -0.1958661417322833942, -2.936371021818584115 ) ) ;
#47605=CARTESIAN_POINT ( 'NONE',  ( -0.3917322834645671215, 0.1049643490035301469, -2.164698162729658648 ) ) ;
#47611=CARTESIAN_POINT ( 'NONE',  ( -0.3996062992125986590, 0.1070741851644051723, 0.04790026246719158304 ) ) ;
#47613=CARTESIAN_POINT ( 'NONE',  ( 4.893765752498283924E-17, -0.3996062992125986035, -1.968503937007873850 ) ) ;
#47615=( BOUNDED_CURVE ( )  B_SPLINE_CURVE ( 2, ( #13085, #78734, #38738, #32422, #58084, #450, #26105, #51767, #19806, #77469, #71153, #13494, #64835 ),
 .UNSPECIFIED., .F., .F. ) 
 B_SPLINE_CURVE_WITH_KNOTS ( ( 3, 2, 2, 2, 2, 2, 3 ),
 ( 0.7875000000000000888, 0.7916666666666667407, 0.7958333333333333925, 0.8000000000000000444, 0.8041666666666666963, 0.8083333333333333481, 0.8125000000000000000 ),
 .UNSPECIFIED. ) 
 CURVE ( )  GEOMETRIC_REPRESENTATION_ITEM ( )  RATIONAL_B_SPLINE_CURVE ( ( 0.9999999999999991118, 0.9659258262890692004, 1.000000000000000000, 0.9659258262890683122, 1.000000000000000000, 0.9659258262890683122, 1.000000000000000000, 0.9659258262890683122, 1.000000000000000000, 0.9659258262890683122, 1.000000000000000000, 0.9659258262890683122, 1.000000000000000000 ) ) 
 REPRESENTATION_ITEM ( '' )  );
#47619=CARTESIAN_POINT ( 'NONE',  ( 0.1265901696524989462, 0.4724409448818897572, -0.8576115485564304031 ) ) ;
#47623=CARTESIAN_POINT ( 'NONE',  ( 0.2891555358219910499, 0.2891555358219910499, -0.3720472440944882497 ) ) ;
#47630=CARTESIAN_POINT ( 'NONE',  ( -0.1058382717557497660, -0.3949938075777411073, -0.6213910761154856077 ) ) ;
#47637=CARTESIAN_POINT ( 'NONE',  ( -0.1070741851644056997, 0.3996062992125984925, -1.343175853018372834 ) ) ;
#47639=CARTESIAN_POINT ( 'NONE',  ( 0.3917322834645670104, 2.398668435337828261E-17, -1.055118110236220375 ) ) ;
#47641=CARTESIAN_POINT ( 'NONE',  ( -0.1716039559346191345, -0.3527845929029423400, -1.489137855930806014E-17 ) ) ;
#47658=CARTESIAN_POINT ( 'NONE',  ( 0.4091458600556403535, 0.2362204724409449896, -2.020997375328084100 ) ) ;
#47668=CARTESIAN_POINT ( 'NONE',  ( -0.3460692066303958092, -0.1998031496062994683, -0.8398950131233595684 ) ) ;
#47672=CARTESIAN_POINT ( 'NONE',  ( 5.785732909357575061E-17, -0.4724409448818898682, 0.07874015748031495954 ) ) ;
#47673=CARTESIAN_POINT ( 'NONE',  ( -0.2891555358219908833, -0.2891555358219912164, -2.421259842519685623 ) ) ;
#47676=CARTESIAN_POINT ( 'NONE',  ( 0.3392501089628018329, 0.1958661417322835607, -1.068241469816272771 ) ) ;
#47682=CARTESIAN_POINT ( 'NONE',  ( -9.594673741351310580E-17, 0.3917322834645669549, -0.2375134926171111049 ) ) ;
#47687=( BOUNDED_SURFACE ( )  B_SPLINE_SURFACE ( 3, 2, ( 
 ( #40276, #9950, #79018, #65959, #22165, #53717, #35623, #54550, #14622, #22581, #28060, #33963, #21744, #48242, #41109, #22989, #41927, #60046, #54968, #59625, #48654, #61286, #73525, #1980, #21337, #46989, #2402, #3638, #79424, #47409, #15450, #66797, #9132, #2813, #34803, #67207, #73938, #67620, #29715, #75177, #56206, #74765, #62117, #30125, #68850, #81907, #17521, #4869, #30542, #49067, #81083, #36444, #4460, #16695, #24219, #74351, #68033, #49484, #43154, #55789, #23400, #42335, #10378, #11198, #36035, #42749, #61709, #36857, #62531, #17114, #10784, #4049, #55377, #81495, #68444, #23811, #59068, #51480, #40546, #25820, #66227, #70874, #45168, #26242, #14479, #51902, #38871, #27079, #27495, #72121, #65403, #14057, #77183, #71703, #32978, #71285, #64550, #78027, #19515, #57800, #26666, #167, #53152, #13223, #6887, #39712, #13633, #78864, #52740, #32144, #40132, #45592, #32557, #39285, #46429, #58645, #14886, #33816, #58220, #46844, #586, #72538, #21190, #7740, #77609, #19942, #64972, #7308, #1013, #52321, #20356, #46007, #33406, #1423, #78449, #20775, #65818, #8151, #59482, #1835, #54824, #23249, #73371, #80115, #16128, #42191, #48918, #80528, #3904, #29564, #22016, #28326, #54403, #22433, #2248, #74619, #16963, #27914, #9802, #29155, #28742, #60318, #80933, #42602, #61137, #10224, #2667, #35891, #48092, #35473, #47259, #53987, #73792, #3489, #72949, #8565, #15300, #53573, #41774, #67467, #34234, #66644, #8981, #74200, #79700, #22840, #34654, #16546, #47676, #79282, #48499, #67886, #15720, #61561, #55226, #41376, #59896, #67057, #21597, #35060, #9390, #40962, #60726, #3077, #24888, #37118, #5953, #55636, #75441, #50557, #11876, #4308, #81345, #17780, #10640, #31208, #36701, #11042, #30387, #69526, #23660, #56053, #75847, #49330, #18996, #82981, #37528, #63203, #5543, #11460, #62375, #50966, #81762, #5136, #56876, #18595, #30801, #24072, #57284, #4713, #49741, #43822, #36295, #29972, #68701, #76260, #56466, #82569, #44238, #75032, #43414, #69112, #69927, #62802, #12283, #18189, #24484, #25300, #82168, #50151, #17377, #37939, #63616, #76663, #31622, #43007, #68304, #61969, #77082, #77926, #78767, #40038, #13118, #913, #26570, #7641, #52223, #45065, #45489, #14380, #58547, #32455, #6370, #38770, #32042, #33311, #51800, #58117, #13956, #57701, #20257, #25717, #26978, #484, #19840, #70768, #33718, #7208, #8057, #63, #1329, #20679, #46331, #59380, #58973, #65724, #64447, #6783, #26139, #1738, #52643, #12696, #27395, #77505, #78347, #51377, #45906, #71186, #13528, #38355, #72024, #53055, #71603, #39184, #44645, #64868, #19414, #32878, #39613, #70342, #65302, #64030, #73695, #67374, #74103, #34967, #8877, #66128, #15201, #8465, #9708, #28228, #34553, #16035, #34135, #28646, #2150, #3394, #60219, #79601, #47161, #10127, #66964, #67791, #59796, #61044, #80433, #22743, #35792, #35379, #16449, #72853, #21503, #2569, #61459, #29057, #72443, #42094, #53887, #54728, #27817, #54306, #21917, #47579, #14792, #48403, #3807, #22335, #15621, #29469, #73272, #53477, #40861, #79187, #55127, #80017, #21091, #41681, #46750, #40449, #66544, #41278, #9297, #47996, #60630, #2981, #4616, #23150, #43725, #49232, #23561, #42908, #82071, #36199, #68603, #5040, #10542, #31527, #12185, #24384, #75750, #18091, #23976, #74935, #63520, #10943, #17683, #50055, #31108, #43313, #36600, #69835, #17280, #62278, #56372, #48819, #42503, #81246, #63109, #69011, #69429, #11782, #4210, #30287, #55953, #37435, #81666, #5447, #30709, #37020, #37842, #11363, #49644, #61869, #56775, #75336, #5850, #18500, #68205, #82475, #24791, #29874, #50459, #80837, #76163, #62701, #44143, #74519, #16866, #55536, #57603, #58017, #70660, #46229, #83293, #25616, #32775, #82885, #18899, #51279, #39509, #19734, #20156, #804, #63930 ),
 ( #12594, #25205, #39085, #13016, #52538, #52118, #57183, #13851, #38670, #50871, #64348, #71503, #382, #39937, #58871, #76982, #71926, #76571, #14275, #20578, #13429, #44549, #70239, #65623, #19311, #7954, #38253, #44964, #32356, #6266, #31942, #45389, #6685, #26038, #77826, #65198, #51698, #45806, #77400, #71086, #64766, #7105, #7534, #58444, #33206, #78246, #26467, #1229, #26878, #79494, #21809, #27294, #16347, #74000, #52952, #34867, #54197, #53782, #2047, #22643, #48303, #2878, #35274, #27711, #60938, #47473, #60528, #72343, #53377, #73165, #28540, #14691, #41990, #40347, #78667, #41173, #66864, #67685, #8363, #34030, #15935, #79085, #15516, #59691, #41582, #21403, #20987, #9194, #79913, #47057, #22230, #47885, #72749, #73592, #15097, #67272, #60117, #40754, #9605, #59279, #3288, #66438, #46649, #8775, #28953, #2468, #33616, #54618, #34448, #1635, #66026, #28127, #80329, #49543, #29368, #61351, #25832, #29776, #57812, #55028, #55437, #68504, #23050, #35686, #55850, #23461, #80736, #4939, #24283, #61770, #56272, #51491, #74833, #81559, #17582, #44758, #77194, #81968, #6486, #32156, #49128, #81146, #23878, #75238, #3705, #19526, #45180, #48717, #11262, #30608, #30187, #4110, #179, #10020, #62597, #12812, #17177, #38467, #43214, #36920, #74415, #42810, #68910, #49954, #16760, #42399, #68097, #10443, #75652, #17992, #36099, #10844, #36504, #70454, #62180, #64152, #4518, #53166, #64987, #64563, #20787, #72134, #71299, #33828, #8163, #45605, #1435, #26679, #27509, #14071, #1026, #14492, #13234, #59494, #78879, #39724, #79294, #6900, #21612, #26256, #600, #7322, #21202, #32991, #77622, #65830, #66239, #46857, #46443, #52754, #32571, #27091, #71716, #52334, #72551, #58660, #14898, #59080, #65417, #38884, #8576, #51915, #58233, #78462, #78040, #34247, #1848, #70885, #40558, #59909, #40145, #7753, #2262, #20370, #19955, #13647, #39300, #27927, #53585, #46022, #33418, #10239, #68318, #34669, #54418, #29580, #74217, #66658, #60332, #80129, #72962, #35909, #15735, #73384, #9404, #48517, #2680, #35074, #54839, #28340, #81362, #61986, #16562, #42207, #67902, #73807, #41390, #29989, #60740, #67482, #61576, #80950, #9817, #3092, #36310, #67072, #28756, #22856, #15313, #8996, #47690, #55243, #35488, #3919, #23265, #54001, #22448, #48109, #48934, #16144, #74635, #80544, #3504, #16978, #4323, #41791, #61152, #42619, #29171, #55652, #10655, #79713, #47272, #40976, #22029, #56892, #57718, #19013, #75458, #63220, #5560, #69944, #31224, #24088, #24501, #76680, #37545, #11478, #68717, #17796, #11059, #12299, #30816, #37134, #76279, #36717, #82585, #4730, #5970, #62819, #82184, #49758, #12712, #69543, #70357, #62393, #63632, #82997, #25318, #38371, #37955, #44661, #43431, #69128, #5152, #64047, #31639, #75046, #6387, #56481, #57299, #30404, #24904, #50167, #75863, #17392, #50982, #18205, #32058, #43841, #11892, #50573, #49347, #23675, #43023, #18611, #56071, #81778, #44254, #38788, #13137, #77523, #65741, #19858, #6802, #78365, #78784, #40054, #33328, #65320, #19431, #39630, #930, #39203, #59397, #45507, #8074, #71621, #77944, #25734, #21109, #64465, #51395, #7658, #64886, #46768, #20696, #81, #33737, #13547, #77099, #7225, #14398, #26587, #66146, #1755, #504, #14809, #45082, #40468, #72460, #58990, #70786, #32473, #8483, #71204, #34152, #58135, #32897, #58564, #26157, #51818, #45923, #52240, #20273, #46347, #27412, #13973, #72042, #1346, #26996, #52659, #53073, #10145, #16883, #22759, #55144, #80855, #73290, #79619, #22352, #48012, #53495, #42521, #68224, #79204, #61060, #80449, #80033, #28245, #48836, #74537, #29073, #61476, #53905, #3824, #73711, #3411, #15219, #21936, #16051, #54744, #40879, #10558, #66561, #21520, #67390, #9724, #59813, #34571, #60238, #42111, #47596, #41697, #2586 ),
 ( #48421, #23167, #16466, #35395, #74120, #47179, #67808, #60647, #15638, #35810, #41295, #29485, #2168, #54324, #27834, #72871, #8894, #66980, #9313, #34983, #2997, #28663, #36216, #76178, #49661, #29890, #43327, #50474, #62717, #18915, #37859, #36617, #50886, #55553, #76586, #82900, #75765, #81262, #4226, #44565, #55969, #25220, #23577, #81682, #11378, #49248, #61885, #82086, #75351, #74951, #31124, #18515, #4632, #82491, #70256, #17699, #24400, #43740, #69850, #17297, #24807, #31542, #57198, #69027, #23993, #50070, #18107, #42924, #68619, #10959, #62295, #37450, #56791, #56387, #30303, #37035, #5055, #5462, #63535, #30725, #5866, #69445, #63124, #11797, #44158, #12201, #39524, #51296, #1652, #76999, #57620, #20170, #45820, #27309, #70678, #13034, #78261, #32371, #52134, #38687, #20592, #6702, #6283, #71519, #13865, #64365, #58885, #33222, #58035, #26483, #51715, #52552, #39101, #26056, #65212, #38269, #1244, #46244, #64783, #21003, #31959, #46665, #19330, #25633, #398, #77416, #52968, #78652, #78682, #59295, #77841, #44982, #63946, #12611, #19752, #45406, #71102, #13445, #7121, #32792, #58461, #821, #7549, #26893, #71940, #14289, #39953, #65639, #7969, #33632, #60544, #79931, #22658, #29383, #35291, #67700, #10036, #2484, #8791, #34883, #2895, #66042, #55043, #80750, #8380, #73609, #9620, #9210, #40770, #61367, #3719, #41597, #74014, #66455, #16361, #28559, #15951, #27727, #34464, #54215, #67287, #53394, #23064, #79101, #34045, #22246, #47901, #72359, #47074, #72765, #54632, #60133, #60953, #15116, #80345, #28143, #59708, #3303, #28968, #53799, #48317, #42006, #79511, #35700, #21827, #14707, #15532, #47490, #40362, #2063, #21420, #73182, #41190, #66880, #42414, #57098, #4125, #61785, #42825, #31023, #68518, #55451, #43640, #44059, #5362, #81984, #30622, #68111, #4952, #49559, #4532, #24708, #10859, #56691, #36934, #43229, #74429, #69751, #29790, #16776, #56287, #30202, #12097, #69343, #48732, #82390, #62195, #10459, #55864, #63024, #75253, #31435, #50376, #36519, #11275, #62612, #36113, #82793, #5766, #81160, #49968, #11694, #68926, #17192, #37755, #63430, #18006, #76074, #81574, #18416, #24298, #75666, #23476, #23893, #37351, #49143, #74848, #17597, #63841, #70153, #32685, #58352, #14186, #83207, #25529, #7441, #44872, #64678, #51194, #33112, #19222, #18815, #713, #26372, #76892, #71416, #45719, #70571, #38995, #64263, #65104, #51607, #38584, #52030, #50787, #13763, #58780, #77312, #33530, #44462, #59193, #6179, #38167, #12925, #1140, #6597, #31854, #20067, #20488, #26790, #77736, #7017, #12506, #39420, #25949, #32269, #52447, #57929, #78157, #13341, #19642, #76488, #46142, #57516, #293, #71837, #45302, #39844, #65533, #25115, #7866, #70998, #78579, #8694, #15858, #28042, #67604, #3210, #1963, #16265, #20905, #41910, #48227, #41092, #46558, #52869, #9935, #21319, #73923, #72256, #46972, #60030, #14605, #27206, #47391, #15015, #40259, #79832, #41507, #53288, #47807, #35607, #66356, #73082, #9115, #35195, #1552, #73510, #80250, #22566, #40671, #60856, #78999, #67192, #15432, #79409, #65942, #8278, #33944, #59608, #66781, #34364, #27625, #22149, #72666, #9523, #2385, #53700, #21728, #28872, #34787, #60446, #54534, #2798, #28457, #54117, #75982, #24617, #17507, #80660, #29290, #18323, #81067, #50284, #22972, #23383, #36429, #74333, #3623, #23796, #74749, #48639, #56191, #75575, #29699, #24204, #43964, #42733, #49468, #68836, #11598, #69660, #49875, #56598, #82298, #17098, #49051, #75162, #43139, #54953, #12004, #61269, #16680, #62515, #81893, #81479, #55362, #42319, #68018, #30528, #62934, #68429, #5267, #11182, #4853, #10362, #10769, #36843, #17915, #36022, #61694, #4034, #62102, #43551, #69252, #4445, #30110, #55772, #37258, #30931, #77214, #38070, #19972, #31759, #31339 ),
 ( #26274, #77640, #6504, #46040, #57005, #71734, #76391, #50694, #57421, #45623, #83115, #44366, #32590, #33007, #71317, #70903, #19543, #82701, #45201, #38487, #76796, #13666, #13253, #38902, #25020, #64582, #64171, #19127, #39318, #25433, #65003, #25850, #32175, #63336, #58677, #18724, #5672, #6919, #44776, #1042, #58253, #37658, #7339, #51099, #70058, #70473, #51935, #57830, #20388, #26696, #63746, #52351, #12412, #78058, #6085, #618, #12830, #198, #51510, #33845, #61901, #59097, #59511, #72567, #27109, #39741, #59926, #27527, #1452, #10160, #29500, #65846, #61492, #29905, #78897, #2282, #21630, #48852, #55569, #3840, #10574, #36231, #53182, #1865, #27944, #53602, #7770, #81277, #23593, #33437, #15331, #35826, #34266, #8179, #4242, #49264, #66676, #16898, #21218, #42537, #79311, #40996, #52772, #46873, #47290, #55160, #78480, #14089, #20804, #46460, #72979, #80870, #65437, #72154, #14509, #23182, #14914, #74553, #40162, #68239, #40574, #66255, #8594, #76192, #75367, #37874, #12217, #49676, #5478, #30739, #31555, #18122, #5070, #18529, #17312, #63548, #57212, #43754, #23531, #68635, #25648, #30318, #4647, #69044, #82914, #11393, #81697, #69865, #70271, #69460, #50899, #17714, #31973, #12625, #36634, #50489, #18930, #24008, #24821, #74966, #38284, #43342, #31139, #56806, #5882, #82505, #37050, #75780, #44578, #44172, #62732, #62310, #56402, #55986, #25234, #82101, #24414, #76599, #50084, #63960, #11810, #6297, #37465, #63138, #57633, #42940, #10974, #14723, #64379, #7984, #27324, #52984, #40376, #39968, #46681, #19766, #51729, #7135, #66059, #33648, #19345, #72374, #39115, #1667, #58048, #58900, #32808, #77855, #44995, #59311, #78697, #52568, #45835, #21020, #64796, #38700, #77431, #414, #8395, #26908, #34062, #20608, #14308, #59725, #6715, #58475, #2080, #78276, #70694, #32385, #839, #77013, #65655, #45419, #71115, #13458, #46260, #26070, #26497, #1260, #52149, #51310, #13047, #71955, #20184, #71533, #13881, #39540, #65228, #7566, #33238, #28984, #61386, #73625, #41208, #16793, #53815, #79529, #3320, #53410, #72781, #28160, #10053, #15967, #74030, #54651, #34483, #21843, #73199, #16377, #47507, #80361, #60969, #67303, #67717, #42430, #2912, #68130, #15549, #66896, #22674, #79118, #15131, #9226, #35716, #41614, #42023, #48333, #60149, #34899, #60561, #3735, #28575, #29399, #55058, #9638, #80766, #10475, #54232, #79949, #23081, #22262, #36128, #48748, #40787, #74447, #61801, #2501, #27745, #21436, #47091, #47920, #35307, #66472, #8807, #82002, #36536, #68944, #76092, #56305, #81594, #23494, #30220, #49160, #63042, #17615, #23911, #69361, #74866, #49986, #17209, #56709, #49576, #43246, #62212, #12115, #4974, #69771, #42842, #31041, #24727, #50395, #37773, #5380, #18436, #4550, #55883, #75272, #63448, #82408, #55467, #44078, #11294, #5784, #68535, #24316, #36953, #62630, #81177, #31454, #4141, #43659, #30640, #29806, #75684, #18025, #11715, #37371, #10875, #54922, #61663, #48607, #42289, #17068, #66750, #3176, #4004, #22940, #15400, #9085, #28841, #21698, #67986, #47777, #22117, #41476, #80629, #34756, #67161, #3593, #60416, #30079, #10741, #74302, #16648, #10331, #22533, #73478, #62073, #9490, #16231, #35993, #29669, #41878, #35164, #42705, #41061, #55330, #23351, #28426, #29258, #79379, #74719, #15828, #35576, #61239, #81039, #49023, #79801, #80217, #68402, #9904, #60825, #2767, #54503, #54086, #36398, #48195, #73891, #4411, #67572, #47361, #73050, #38041, #69218, #30901, #81863, #44747, #18291, #19098, #68804, #12383, #31728, #57392, #70442, #44339, #51068, #24175, #56160, #11566, #12800, #63716, #23767, #76768, #43518, #6057, #62485, #63306, #37225, #82269, #49438, #83083, #25405, #56975, #50254, #38455, #62902, #43108, #49844, #4819, #64141, #31311, #6474, #24989, #18697 ) ),
 .UNSPECIFIED., .F., .F., .F. ) 
 B_SPLINE_SURFACE_WITH_KNOTS ( ( 4, 4 ),
 ( 3, 2, 2, 2, 2, 2, 2, 2, 2, 2, 2, 2, 2, 2, 2, 2, 2, 2, 2, 2, 2, 2, 2, 2, 2, 2, 2, 2, 2, 2, 2, 2, 2, 2, 2, 2, 2, 2, 2, 2, 2, 2, 2, 2, 2, 2, 2, 2, 2, 2, 2, 2, 2, 2, 2, 2, 2, 2, 2, 2, 2, 2, 2, 2, 2, 2, 2, 2, 2, 2, 2, 2, 2, 2, 2, 2, 2, 2, 2, 2, 2, 2, 2, 2, 2, 2, 2, 2, 2, 2, 2, 2, 2, 2, 2, 2, 2, 2, 2, 2, 2, 2, 2, 2, 2, 2, 2, 2, 2, 2, 2, 2, 2, 2, 2, 2, 2, 2, 2, 2, 2, 2, 2, 2, 2, 2, 2, 2, 2, 2, 2, 2, 2, 2, 2, 2, 2, 2, 2, 2, 2, 2, 2, 2, 2, 2, 2, 2, 2, 2, 2, 2, 2, 2, 2, 2, 2, 2, 2, 2, 2, 2, 2, 2, 2, 2, 2, 2, 2, 2, 2, 2, 2, 2, 2, 2, 2, 2, 2, 2, 2, 2, 2, 2, 2, 2, 2, 2, 2, 2, 2, 2, 2, 2, 2, 2, 2, 2, 2, 2, 2, 2, 2, 2, 2, 2, 2, 2, 2, 2, 2, 2, 2, 2, 2, 2, 2, 2, 2, 2, 2, 2, 2, 2, 2, 2, 2, 2, 2, 2, 2, 2, 2, 2, 2, 2, 2, 3 ),
 ( 0.000000000000000000, 1.000000000000000000 ),
 ( 0.000000000000000000, 0.004166666666666666609, 0.008333333333333333218, 0.01250000000000000069, 0.01666666666666666644, 0.02083333333333333218, 0.02500000000000000139, 0.02916666666666666713, 0.03333333333333333287, 0.03749999999999999861, 0.04166666666666666435, 0.04583333333333333010, 0.05000000000000000278, 0.05416666666666666852, 0.05833333333333333426, 0.06250000000000000000, 0.06666666666666666574, 0.07083333333333333148, 0.07499999999999999722, 0.07916666666666666297, 0.08333333333333332871, 0.08749999999999999445, 0.09166666666666666019, 0.09583333333333333981, 0.1000000000000000056, 0.1041666666666666713, 0.1083333333333333370, 0.1125000000000000028, 0.1166666666666666685, 0.1208333333333333343, 0.1250000000000000000, 0.1291666666666666796, 0.1333333333333333315, 0.1375000000000000111, 0.1416666666666666630, 0.1458333333333333426, 0.1499999999999999944, 0.1541666666666666741, 0.1583333333333333259, 0.1625000000000000056, 0.1666666666666666574, 0.1708333333333333370, 0.1749999999999999889, 0.1791666666666666685, 0.1833333333333333204, 0.1875000000000000000, 0.1916666666666666796, 0.1958333333333333315, 0.2000000000000000111, 0.2041666666666666630, 0.2083333333333333426, 0.2124999999999999944, 0.2166666666666666741, 0.2208333333333333259, 0.2250000000000000056, 0.2291666666666666574, 0.2333333333333333370, 0.2374999999999999889, 0.2416666666666666685, 0.2458333333333333204, 0.2500000000000000000, 0.2541666666666666519, 0.2583333333333333592, 0.2625000000000000111, 0.2666666666666666630, 0.2708333333333333148, 0.2750000000000000222, 0.2791666666666666741, 0.2833333333333333259, 0.2874999999999999778, 0.2916666666666666852, 0.2958333333333333370, 0.2999999999999999889, 0.3041666666666666408, 0.3083333333333333481, 0.3125000000000000000, 0.3166666666666666519, 0.3208333333333333592, 0.3250000000000000111, 0.3291666666666666630, 0.3333333333333333148, 0.3375000000000000222, 0.3416666666666666741, 0.3458333333333333259, 0.3499999999999999778, 0.3541666666666666852, 0.3583333333333333370, 0.3624999999999999889, 0.3666666666666666408, 0.3708333333333333481, 0.3750000000000000000, 0.3791666666666666519, 0.3833333333333333592, 0.3875000000000000111, 0.3916666666666666630, 0.3958333333333333148, 0.4000000000000000222, 0.4041666666666666741, 0.4083333333333333259, 0.4124999999999999778, 0.4166666666666666852, 0.4208333333333333370, 0.4249999999999999889, 0.4291666666666666408, 0.4333333333333333481, 0.4375000000000000000, 0.4416666666666666519, 0.4458333333333333592, 0.4500000000000000111, 0.4541666666666666630, 0.4583333333333333148, 0.4625000000000000222, 0.4666666666666666741, 0.4708333333333333259, 0.4749999999999999778, 0.4791666666666666852, 0.4833333333333333370, 0.4874999999999999889, 0.4916666666666666408, 0.4958333333333333481, 0.5000000000000000000, 0.5041666666666666519, 0.5083333333333333037, 0.5124999999999999556, 0.5166666666666667185, 0.5208333333333333703, 0.5250000000000000222, 0.5291666666666666741, 0.5333333333333333259, 0.5374999999999999778, 0.5416666666666666297, 0.5458333333333332815, 0.5500000000000000444, 0.5541666666666666963, 0.5583333333333333481, 0.5625000000000000000, 0.5666666666666666519, 0.5708333333333333037, 0.5749999999999999556, 0.5791666666666667185, 0.5833333333333333703, 0.5875000000000000222, 0.5916666666666666741, 0.5958333333333333259, 0.5999999999999999778, 0.6041666666666666297, 0.6083333333333332815, 0.6125000000000000444, 0.6166666666666666963, 0.6208333333333333481, 0.6250000000000000000, 0.6291666666666666519, 0.6333333333333333037, 0.6374999999999999556, 0.6416666666666667185, 0.6458333333333333703, 0.6500000000000000222, 0.6541666666666666741, 0.6583333333333333259, 0.6624999999999999778, 0.6666666666666666297, 0.6708333333333332815, 0.6750000000000000444, 0.6791666666666666963, 0.6833333333333333481, 0.6875000000000000000, 0.6916666666666666519, 0.6958333333333333037, 0.6999999999999999556, 0.7041666666666667185, 0.7083333333333333703, 0.7125000000000000222, 0.7166666666666666741, 0.7208333333333333259, 0.7249999999999999778, 0.7291666666666666297, 0.7333333333333332815, 0.7375000000000000444, 0.7416666666666666963, 0.7458333333333333481, 0.7500000000000000000, 0.7541666666666666519, 0.7583333333333333037, 0.7624999999999999556, 0.7666666666666667185, 0.7708333333333333703, 0.7750000000000000222, 0.7791666666666666741, 0.7833333333333333259, 0.7874999999999999778, 0.7916666666666666297, 0.7958333333333332815, 0.8000000000000000444, 0.8041666666666666963, 0.8083333333333333481, 0.8125000000000000000, 0.8166666666666666519, 0.8208333333333333037, 0.8249999999999999556, 0.8291666666666667185, 0.8333333333333333703, 0.8375000000000000222, 0.8416666666666666741, 0.8458333333333333259, 0.8499999999999999778, 0.8541666666666666297, 0.8583333333333332815, 0.8625000000000000444, 0.8666666666666666963, 0.8708333333333333481, 0.8750000000000000000, 0.8791666666666666519, 0.8833333333333333037, 0.8874999999999999556, 0.8916666666666667185, 0.8958333333333333703, 0.9000000000000000222, 0.9041666666666666741, 0.9083333333333333259, 0.9124999999999999778, 0.9166666666666666297, 0.9208333333333332815, 0.9250000000000000444, 0.9291666666666666963, 0.9333333333333333481, 0.9375000000000000000, 0.9416666666666666519, 0.9458333333333333037, 0.9499999999999999556, 0.9541666666666667185, 0.9583333333333333703, 0.9625000000000000222, 0.9666666666666666741, 0.9708333333333333259, 0.9749999999999999778, 0.9791666666666666297, 0.9833333333333332815, 0.9875000000000000444 ),
 .UNSPECIFIED. ) 
 GEOMETRIC_REPRESENTATION_ITEM ( )  RATIONAL_B_SPLINE_SURFACE ( (
 ( 1.000000000000000000, 0.9659258262890683122, 1.000000000000000000, 0.9659258262890683122, 1.000000000000000000, 0.9659258262890683122, 1.000000000000000000, 0.9659258262890683122, 1.000000000000000000, 0.9659258262890683122, 1.000000000000000000, 0.9659258262890683122, 1.000000000000000000, 0.9659258262890683122, 1.000000000000000000, 0.9659258262890683122, 1.000000000000000000, 0.9659258262890683122, 1.000000000000000000, 0.9659258262890683122, 1.000000000000000000, 0.9659258262890683122, 1.000000000000000000, 0.9659258262890683122, 1.000000000000000000, 0.9659258262890683122, 1.000000000000000000, 0.9659258262890683122, 1.000000000000000000, 0.9659258262890683122, 1.000000000000000000, 0.9659258262890683122, 1.000000000000000000, 0.9659258262890683122, 1.000000000000000000, 0.9659258262890683122, 1.000000000000000000, 0.9659258262890683122, 1.000000000000000000, 0.9659258262890683122, 1.000000000000000000, 0.9659258262890683122, 1.000000000000000000, 0.9659258262890683122, 1.000000000000000000, 0.9659258262890683122, 1.000000000000000000, 0.9659258262890683122, 1.000000000000000000, 0.9659258262890683122, 1.000000000000000000, 0.9659258262890683122, 1.000000000000000000, 0.9659258262890683122, 1.000000000000000000, 0.9659258262890683122, 1.000000000000000000, 0.9659258262890683122, 1.000000000000000000, 0.9659258262890683122, 1.000000000000000000, 0.9659258262890683122, 1.000000000000000000, 0.9659258262890683122, 1.000000000000000000, 0.9659258262890683122, 1.000000000000000000, 0.9659258262890683122, 1.000000000000000000, 0.9659258262890683122, 1.000000000000000000, 0.9659258262890683122, 1.000000000000000000, 0.9659258262890683122, 1.000000000000000000, 0.9659258262890683122, 1.000000000000000000, 0.9659258262890683122, 1.000000000000000000, 0.9659258262890683122, 1.000000000000000000, 0.9659258262890683122, 1.000000000000000000, 0.9659258262890683122, 1.000000000000000000, 0.9659258262890683122, 1.000000000000000000, 0.9659258262890683122, 1.000000000000000000, 0.9659258262890683122, 1.000000000000000000, 0.9659258262890683122, 1.000000000000000000, 0.9659258262890683122, 1.000000000000000000, 0.9659258262890683122, 1.000000000000000000, 0.9659258262890683122, 1.000000000000000000, 0.9659258262890683122, 1.000000000000000000, 0.9659258262890683122, 1.000000000000000000, 0.9659258262890683122, 1.000000000000000000, 0.9659258262890683122, 1.000000000000000000, 0.9659258262890683122, 1.000000000000000000, 0.9659258262890683122, 1.000000000000000000, 0.9659258262890683122, 1.000000000000000000, 0.9659258262890683122, 1.000000000000000000, 0.9659258262890683122, 1.000000000000000000, 0.9659258262890683122, 1.000000000000000000, 0.9659258262890683122, 1.000000000000000000, 0.9659258262890683122, 1.000000000000000000, 0.9659258262890683122, 1.000000000000000000, 0.9659258262890683122, 1.000000000000000000, 0.9659258262890683122, 1.000000000000000000, 0.9659258262890683122, 1.000000000000000000, 0.9659258262890683122, 1.000000000000000000, 0.9659258262890683122, 1.000000000000000000, 0.9659258262890683122, 1.000000000000000000, 0.9659258262890683122, 1.000000000000000000, 0.9659258262890683122, 1.000000000000000000, 0.9659258262890683122, 1.000000000000000000, 0.9659258262890683122, 1.000000000000000000, 0.9659258262890683122, 1.000000000000000000, 0.9659258262890683122, 1.000000000000000000, 0.9659258262890683122, 1.000000000000000000, 0.9659258262890683122, 1.000000000000000000, 0.9659258262890683122, 1.000000000000000000, 0.9659258262890683122, 1.000000000000000000, 0.9659258262890683122, 1.000000000000000000, 0.9659258262890683122, 1.000000000000000000, 0.9659258262890683122, 1.000000000000000000, 0.9659258262890683122, 1.000000000000000000, 0.9659258262890683122, 1.000000000000000000, 0.9659258262890683122, 1.000000000000000000, 0.9659258262890683122, 1.000000000000000000, 0.9659258262890683122, 1.000000000000000000, 0.9659258262890683122, 1.000000000000000000, 0.9659258262890683122, 1.000000000000000000, 0.9659258262890683122, 1.000000000000000000, 0.9659258262890683122, 1.000000000000000000, 0.9659258262890683122, 1.000000000000000000, 0.9659258262890683122, 1.000000000000000000, 0.9659258262890683122, 1.000000000000000000, 0.9659258262890683122, 1.000000000000000000, 0.9659258262890683122, 1.000000000000000000, 0.9659258262890683122, 1.000000000000000000, 0.9659258262890683122, 1.000000000000000000, 0.9659258262890683122, 1.000000000000000000, 0.9659258262890683122, 1.000000000000000000, 0.9659258262890683122, 1.000000000000000000, 0.9659258262890683122, 1.000000000000000000, 0.9659258262890683122, 1.000000000000000000, 0.9659258262890683122, 1.000000000000000000, 0.9659258262890683122, 1.000000000000000000, 0.9659258262890683122, 1.000000000000000000, 0.9659258262890683122, 1.000000000000000000, 0.9659258262890683122, 1.000000000000000000, 0.9659258262890683122, 1.000000000000000000, 0.9659258262890683122, 1.000000000000000000, 0.9659258262890683122, 1.000000000000000000, 0.9659258262890683122, 1.000000000000000000, 0.9659258262890683122, 1.000000000000000000, 0.9659258262890683122, 1.000000000000000000, 0.9659258262890683122, 1.000000000000000000, 0.9659258262890683122, 1.000000000000000000, 0.9659258262890683122, 1.000000000000000000, 0.9659258262890683122, 1.000000000000000000, 0.9659258262890683122, 1.000000000000000000, 0.9659258262890683122, 1.000000000000000000, 0.9659258262890683122, 1.000000000000000000, 0.9659258262890683122, 1.000000000000000000, 0.9659258262890683122, 1.000000000000000000, 0.9659258262890683122, 1.000000000000000000, 0.9659258262890683122, 1.000000000000000000, 0.9659258262890683122, 1.000000000000000000, 0.9659258262890683122, 1.000000000000000000, 0.9659258262890683122, 1.000000000000000000, 0.9659258262890683122, 1.000000000000000000, 0.9659258262890683122, 1.000000000000000000, 0.9659258262890683122, 1.000000000000000000, 0.9659258262890683122, 1.000000000000000000, 0.9659258262890683122, 1.000000000000000000, 0.9659258262890683122, 1.000000000000000000, 0.9659258262890683122, 1.000000000000000000, 0.9659258262890683122, 1.000000000000000000, 0.9659258262890683122, 1.000000000000000000, 0.9659258262890683122, 1.000000000000000000, 0.9659258262890683122, 1.000000000000000000, 0.9659258262890683122, 1.000000000000000000, 0.9659258262890683122, 1.000000000000000000, 0.9659258262890683122, 1.000000000000000000, 0.9659258262890683122, 1.000000000000000000, 0.9659258262890683122, 1.000000000000000000, 0.9659258262890683122, 1.000000000000000000, 0.9659258262890683122, 1.000000000000000000, 0.9659258262890683122, 1.000000000000000000, 0.9659258262890683122, 1.000000000000000000, 0.9659258262890683122, 1.000000000000000000, 0.9659258262890683122, 1.000000000000000000, 0.9659258262890683122, 1.000000000000000000, 0.9659258262890683122, 1.000000000000000000, 0.9659258262890683122, 1.000000000000000000, 0.9659258262890683122, 1.000000000000000000, 0.9659258262890683122, 1.000000000000000000, 0.9659258262890683122, 1.000000000000000000, 0.9659258262890683122, 1.000000000000000000, 0.9659258262890683122, 1.000000000000000000, 0.9659258262890683122, 1.000000000000000000, 0.9659258262890683122, 1.000000000000000000, 0.9659258262890683122, 1.000000000000000000, 0.9659258262890683122, 1.000000000000000000, 0.9659258262890683122, 1.000000000000000000, 0.9659258262890683122, 1.000000000000000000, 0.9659258262890683122, 1.000000000000000000, 0.9659258262890683122, 1.000000000000000000, 0.9659258262890683122, 1.000000000000000000, 0.9659258262890683122, 1.000000000000000000, 0.9659258262890683122, 1.000000000000000000, 0.9659258262890683122, 1.000000000000000000, 0.9659258262890683122, 1.000000000000000000, 0.9659258262890683122, 1.000000000000000000, 0.9659258262890683122, 1.000000000000000000, 0.9659258262890683122, 1.000000000000000000, 0.9659258262890683122, 1.000000000000000000, 0.9659258262890683122, 1.000000000000000000, 0.9659258262890683122, 1.000000000000000000, 0.9659258262890683122, 1.000000000000000000, 0.9659258262890683122, 1.000000000000000000, 0.9659258262890683122, 1.000000000000000000, 0.9659258262890683122, 1.000000000000000000, 0.9659258262890683122, 1.000000000000000000, 0.9659258262890683122, 1.000000000000000000, 0.9659258262890683122, 1.000000000000000000, 0.9659258262890683122, 1.000000000000000000, 0.9659258262890683122, 1.000000000000000000, 0.9659258262890683122, 1.000000000000000000, 0.9659258262890683122, 1.000000000000000000, 0.9659258262890683122, 1.000000000000000000, 0.9659258262890683122, 1.000000000000000000, 0.9659258262890683122, 1.000000000000000000, 0.9659258262890683122, 1.000000000000000000, 0.9659258262890683122, 1.000000000000000000, 0.9659258262890683122, 1.000000000000000000, 0.9659258262890683122, 1.000000000000000000, 0.9659258262890683122, 1.000000000000000000, 0.9659258262890683122, 1.000000000000000000, 0.9659258262890683122, 1.000000000000000000, 0.9659258262890683122, 1.000000000000000000, 0.9659258262890683122, 1.000000000000000000, 0.9659258262890683122, 1.000000000000000000, 0.9659258262890683122, 1.000000000000000000, 0.9659258262890683122, 1.000000000000000000, 0.9659258262890683122, 1.000000000000000000, 0.9659258262890683122, 1.000000000000000000, 0.9659258262890683122, 1.000000000000000000, 0.9659258262890683122, 1.000000000000000000, 0.9659258262890683122, 1.000000000000000000, 0.9659258262890683122, 1.000000000000000000, 0.9659258262890683122, 1.000000000000000000, 0.9659258262890683122, 1.000000000000000000, 0.9659258262890683122, 1.000000000000000000, 0.9659258262890683122, 1.000000000000000000, 0.9659258262890683122, 1.000000000000000000, 0.9659258262890683122, 1.000000000000000000, 0.9659258262890683122, 1.000000000000000000, 0.9659258262890683122, 1.000000000000000000, 0.9659258262890683122, 1.000000000000000000, 0.9659258262890683122, 1.000000000000000000, 0.9659258262890683122, 1.000000000000000000, 0.9659258262890683122, 1.000000000000000000, 0.9659258262890683122, 1.000000000000000000, 0.9659258262890683122, 1.000000000000000000, 0.9659258262890683122, 1.000000000000000000, 0.9659258262890683122, 1.000000000000000000, 0.9659258262890683122, 1.000000000000000000, 0.9659258262890683122, 1.000000000000000000, 0.9659258262890683122, 1.000000000000000000, 0.9659258262890683122, 1.000000000000000000, 0.9659258262890683122, 1.000000000000000000, 0.9659258262890683122, 1.000000000000000000, 0.9659258262890683122, 1.000000000000000000, 0.9659258262890683122, 1.000000000000000000, 0.9659258262890683122, 1.000000000000000000, 0.9659258262890683122, 1.000000000000000000, 0.9659258262890683122, 1.000000000000000000, 0.9659258262890683122, 1.000000000000000000, 0.9659258262890683122, 1.000000000000000000),
 ( 0.8047378541243613848, 0.7773170766911654539, 0.8047378541243613848, 0.7773170766911654539, 0.8047378541243613848, 0.7773170766911654539, 0.8047378541243613848, 0.7773170766911654539, 0.8047378541243613848, 0.7773170766911654539, 0.8047378541243613848, 0.7773170766911654539, 0.8047378541243613848, 0.7773170766911654539, 0.8047378541243613848, 0.7773170766911654539, 0.8047378541243613848, 0.7773170766911654539, 0.8047378541243613848, 0.7773170766911654539, 0.8047378541243613848, 0.7773170766911654539, 0.8047378541243613848, 0.7773170766911654539, 0.8047378541243613848, 0.7773170766911654539, 0.8047378541243613848, 0.7773170766911654539, 0.8047378541243613848, 0.7773170766911654539, 0.8047378541243613848, 0.7773170766911654539, 0.8047378541243613848, 0.7773170766911654539, 0.8047378541243613848, 0.7773170766911654539, 0.8047378541243613848, 0.7773170766911654539, 0.8047378541243613848, 0.7773170766911654539, 0.8047378541243613848, 0.7773170766911654539, 0.8047378541243613848, 0.7773170766911654539, 0.8047378541243613848, 0.7773170766911654539, 0.8047378541243613848, 0.7773170766911654539, 0.8047378541243613848, 0.7773170766911654539, 0.8047378541243613848, 0.7773170766911654539, 0.8047378541243613848, 0.7773170766911654539, 0.8047378541243613848, 0.7773170766911654539, 0.8047378541243613848, 0.7773170766911654539, 0.8047378541243613848, 0.7773170766911654539, 0.8047378541243613848, 0.7773170766911654539, 0.8047378541243613848, 0.7773170766911654539, 0.8047378541243613848, 0.7773170766911654539, 0.8047378541243613848, 0.7773170766911654539, 0.8047378541243613848, 0.7773170766911654539, 0.8047378541243613848, 0.7773170766911654539, 0.8047378541243613848, 0.7773170766911654539, 0.8047378541243613848, 0.7773170766911654539, 0.8047378541243613848, 0.7773170766911654539, 0.8047378541243613848, 0.7773170766911654539, 0.8047378541243613848, 0.7773170766911654539, 0.8047378541243613848, 0.7773170766911654539, 0.8047378541243613848, 0.7773170766911654539, 0.8047378541243613848, 0.7773170766911654539, 0.8047378541243613848, 0.7773170766911654539, 0.8047378541243613848, 0.7773170766911654539, 0.8047378541243613848, 0.7773170766911654539, 0.8047378541243613848, 0.7773170766911654539, 0.8047378541243613848, 0.7773170766911654539, 0.8047378541243613848, 0.7773170766911654539, 0.8047378541243613848, 0.7773170766911654539, 0.8047378541243613848, 0.7773170766911654539, 0.8047378541243613848, 0.7773170766911654539, 0.8047378541243613848, 0.7773170766911654539, 0.8047378541243613848, 0.7773170766911654539, 0.8047378541243613848, 0.7773170766911654539, 0.8047378541243613848, 0.7773170766911654539, 0.8047378541243613848, 0.7773170766911654539, 0.8047378541243613848, 0.7773170766911654539, 0.8047378541243613848, 0.7773170766911654539, 0.8047378541243613848, 0.7773170766911654539, 0.8047378541243613848, 0.7773170766911654539, 0.8047378541243613848, 0.7773170766911654539, 0.8047378541243613848, 0.7773170766911654539, 0.8047378541243613848, 0.7773170766911654539, 0.8047378541243613848, 0.7773170766911654539, 0.8047378541243613848, 0.7773170766911654539, 0.8047378541243613848, 0.7773170766911654539, 0.8047378541243613848, 0.7773170766911654539, 0.8047378541243613848, 0.7773170766911654539, 0.8047378541243613848, 0.7773170766911654539, 0.8047378541243613848, 0.7773170766911654539, 0.8047378541243613848, 0.7773170766911654539, 0.8047378541243613848, 0.7773170766911654539, 0.8047378541243613848, 0.7773170766911654539, 0.8047378541243613848, 0.7773170766911654539, 0.8047378541243613848, 0.7773170766911654539, 0.8047378541243613848, 0.7773170766911654539, 0.8047378541243613848, 0.7773170766911654539, 0.8047378541243613848, 0.7773170766911654539, 0.8047378541243613848, 0.7773170766911654539, 0.8047378541243613848, 0.7773170766911654539, 0.8047378541243613848, 0.7773170766911654539, 0.8047378541243613848, 0.7773170766911654539, 0.8047378541243613848, 0.7773170766911654539, 0.8047378541243613848, 0.7773170766911654539, 0.8047378541243613848, 0.7773170766911654539, 0.8047378541243613848, 0.7773170766911654539, 0.8047378541243613848, 0.7773170766911654539, 0.8047378541243613848, 0.7773170766911654539, 0.8047378541243613848, 0.7773170766911654539, 0.8047378541243613848, 0.7773170766911654539, 0.8047378541243613848, 0.7773170766911654539, 0.8047378541243613848, 0.7773170766911654539, 0.8047378541243613848, 0.7773170766911654539, 0.8047378541243613848, 0.7773170766911654539, 0.8047378541243613848, 0.7773170766911654539, 0.8047378541243613848, 0.7773170766911654539, 0.8047378541243613848, 0.7773170766911654539, 0.8047378541243613848, 0.7773170766911654539, 0.8047378541243613848, 0.7773170766911654539, 0.8047378541243613848, 0.7773170766911654539, 0.8047378541243613848, 0.7773170766911654539, 0.8047378541243613848, 0.7773170766911654539, 0.8047378541243613848, 0.7773170766911654539, 0.8047378541243613848, 0.7773170766911654539, 0.8047378541243613848, 0.7773170766911654539, 0.8047378541243613848, 0.7773170766911654539, 0.8047378541243613848, 0.7773170766911654539, 0.8047378541243613848, 0.7773170766911654539, 0.8047378541243613848, 0.7773170766911654539, 0.8047378541243613848, 0.7773170766911654539, 0.8047378541243613848, 0.7773170766911654539, 0.8047378541243613848, 0.7773170766911654539, 0.8047378541243613848, 0.7773170766911654539, 0.8047378541243613848, 0.7773170766911654539, 0.8047378541243613848, 0.7773170766911654539, 0.8047378541243613848, 0.7773170766911654539, 0.8047378541243613848, 0.7773170766911654539, 0.8047378541243613848, 0.7773170766911654539, 0.8047378541243613848, 0.7773170766911654539, 0.8047378541243613848, 0.7773170766911654539, 0.8047378541243613848, 0.7773170766911654539, 0.8047378541243613848, 0.7773170766911654539, 0.8047378541243613848, 0.7773170766911654539, 0.8047378541243613848, 0.7773170766911654539, 0.8047378541243613848, 0.7773170766911654539, 0.8047378541243613848, 0.7773170766911654539, 0.8047378541243613848, 0.7773170766911654539, 0.8047378541243613848, 0.7773170766911654539, 0.8047378541243613848, 0.7773170766911654539, 0.8047378541243613848, 0.7773170766911654539, 0.8047378541243613848, 0.7773170766911654539, 0.8047378541243613848, 0.7773170766911654539, 0.8047378541243613848, 0.7773170766911654539, 0.8047378541243613848, 0.7773170766911654539, 0.8047378541243613848, 0.7773170766911654539, 0.8047378541243613848, 0.7773170766911654539, 0.8047378541243613848, 0.7773170766911654539, 0.8047378541243613848, 0.7773170766911654539, 0.8047378541243613848, 0.7773170766911654539, 0.8047378541243613848, 0.7773170766911654539, 0.8047378541243613848, 0.7773170766911654539, 0.8047378541243613848, 0.7773170766911654539, 0.8047378541243613848, 0.7773170766911654539, 0.8047378541243613848, 0.7773170766911654539, 0.8047378541243613848, 0.7773170766911654539, 0.8047378541243613848, 0.7773170766911654539, 0.8047378541243613848, 0.7773170766911654539, 0.8047378541243613848, 0.7773170766911654539, 0.8047378541243613848, 0.7773170766911654539, 0.8047378541243613848, 0.7773170766911654539, 0.8047378541243613848, 0.7773170766911654539, 0.8047378541243613848, 0.7773170766911654539, 0.8047378541243613848, 0.7773170766911654539, 0.8047378541243613848, 0.7773170766911654539, 0.8047378541243613848, 0.7773170766911654539, 0.8047378541243613848, 0.7773170766911654539, 0.8047378541243613848, 0.7773170766911654539, 0.8047378541243613848, 0.7773170766911654539, 0.8047378541243613848, 0.7773170766911654539, 0.8047378541243613848, 0.7773170766911654539, 0.8047378541243613848, 0.7773170766911654539, 0.8047378541243613848, 0.7773170766911654539, 0.8047378541243613848, 0.7773170766911654539, 0.8047378541243613848, 0.7773170766911654539, 0.8047378541243613848, 0.7773170766911654539, 0.8047378541243613848, 0.7773170766911654539, 0.8047378541243613848, 0.7773170766911654539, 0.8047378541243613848, 0.7773170766911654539, 0.8047378541243613848, 0.7773170766911654539, 0.8047378541243613848, 0.7773170766911654539, 0.8047378541243613848, 0.7773170766911654539, 0.8047378541243613848, 0.7773170766911654539, 0.8047378541243613848, 0.7773170766911654539, 0.8047378541243613848, 0.7773170766911654539, 0.8047378541243613848, 0.7773170766911654539, 0.8047378541243613848, 0.7773170766911654539, 0.8047378541243613848, 0.7773170766911654539, 0.8047378541243613848, 0.7773170766911654539, 0.8047378541243613848, 0.7773170766911654539, 0.8047378541243613848, 0.7773170766911654539, 0.8047378541243613848, 0.7773170766911654539, 0.8047378541243613848, 0.7773170766911654539, 0.8047378541243613848, 0.7773170766911654539, 0.8047378541243613848, 0.7773170766911654539, 0.8047378541243613848, 0.7773170766911654539, 0.8047378541243613848, 0.7773170766911654539, 0.8047378541243613848, 0.7773170766911654539, 0.8047378541243613848, 0.7773170766911654539, 0.8047378541243613848, 0.7773170766911654539, 0.8047378541243613848, 0.7773170766911654539, 0.8047378541243613848, 0.7773170766911654539, 0.8047378541243613848, 0.7773170766911654539, 0.8047378541243613848, 0.7773170766911654539, 0.8047378541243613848, 0.7773170766911654539, 0.8047378541243613848, 0.7773170766911654539, 0.8047378541243613848, 0.7773170766911654539, 0.8047378541243613848, 0.7773170766911654539, 0.8047378541243613848, 0.7773170766911654539, 0.8047378541243613848, 0.7773170766911654539, 0.8047378541243613848, 0.7773170766911654539, 0.8047378541243613848, 0.7773170766911654539, 0.8047378541243613848, 0.7773170766911654539, 0.8047378541243613848, 0.7773170766911654539, 0.8047378541243613848, 0.7773170766911654539, 0.8047378541243613848, 0.7773170766911654539, 0.8047378541243613848, 0.7773170766911654539, 0.8047378541243613848, 0.7773170766911654539, 0.8047378541243613848, 0.7773170766911654539, 0.8047378541243613848, 0.7773170766911654539, 0.8047378541243613848, 0.7773170766911654539, 0.8047378541243613848, 0.7773170766911654539, 0.8047378541243613848, 0.7773170766911654539, 0.8047378541243613848, 0.7773170766911654539, 0.8047378541243613848, 0.7773170766911654539, 0.8047378541243613848, 0.7773170766911654539, 0.8047378541243613848, 0.7773170766911654539, 0.8047378541243613848, 0.7773170766911654539, 0.8047378541243613848, 0.7773170766911654539, 0.8047378541243613848, 0.7773170766911654539, 0.8047378541243613848, 0.7773170766911654539, 0.8047378541243613848, 0.7773170766911654539, 0.8047378541243613848, 0.7773170766911654539, 0.8047378541243613848, 0.7773170766911654539, 0.8047378541243613848, 0.7773170766911654539, 0.8047378541243613848, 0.7773170766911654539, 0.8047378541243613848, 0.7773170766911654539, 0.8047378541243613848, 0.7773170766911654539, 0.8047378541243613848, 0.7773170766911654539, 0.8047378541243613848, 0.7773170766911654539, 0.8047378541243613848, 0.7773170766911654539, 0.8047378541243613848, 0.7773170766911654539, 0.8047378541243613848, 0.7773170766911654539, 0.8047378541243613848, 0.7773170766911654539, 0.8047378541243613848, 0.7773170766911654539, 0.8047378541243613848, 0.7773170766911654539, 0.8047378541243613848),
 ( 0.8047378541243613848, 0.7773170766911654539, 0.8047378541243613848, 0.7773170766911654539, 0.8047378541243613848, 0.7773170766911654539, 0.8047378541243613848, 0.7773170766911654539, 0.8047378541243613848, 0.7773170766911654539, 0.8047378541243613848, 0.7773170766911654539, 0.8047378541243613848, 0.7773170766911654539, 0.8047378541243613848, 0.7773170766911654539, 0.8047378541243613848, 0.7773170766911654539, 0.8047378541243613848, 0.7773170766911654539, 0.8047378541243613848, 0.7773170766911654539, 0.8047378541243613848, 0.7773170766911654539, 0.8047378541243613848, 0.7773170766911654539, 0.8047378541243613848, 0.7773170766911654539, 0.8047378541243613848, 0.7773170766911654539, 0.8047378541243613848, 0.7773170766911654539, 0.8047378541243613848, 0.7773170766911654539, 0.8047378541243613848, 0.7773170766911654539, 0.8047378541243613848, 0.7773170766911654539, 0.8047378541243613848, 0.7773170766911654539, 0.8047378541243613848, 0.7773170766911654539, 0.8047378541243613848, 0.7773170766911654539, 0.8047378541243613848, 0.7773170766911654539, 0.8047378541243613848, 0.7773170766911654539, 0.8047378541243613848, 0.7773170766911654539, 0.8047378541243613848, 0.7773170766911654539, 0.8047378541243613848, 0.7773170766911654539, 0.8047378541243613848, 0.7773170766911654539, 0.8047378541243613848, 0.7773170766911654539, 0.8047378541243613848, 0.7773170766911654539, 0.8047378541243613848, 0.7773170766911654539, 0.8047378541243613848, 0.7773170766911654539, 0.8047378541243613848, 0.7773170766911654539, 0.8047378541243613848, 0.7773170766911654539, 0.8047378541243613848, 0.7773170766911654539, 0.8047378541243613848, 0.7773170766911654539, 0.8047378541243613848, 0.7773170766911654539, 0.8047378541243613848, 0.7773170766911654539, 0.8047378541243613848, 0.7773170766911654539, 0.8047378541243613848, 0.7773170766911654539, 0.8047378541243613848, 0.7773170766911654539, 0.8047378541243613848, 0.7773170766911654539, 0.8047378541243613848, 0.7773170766911654539, 0.8047378541243613848, 0.7773170766911654539, 0.8047378541243613848, 0.7773170766911654539, 0.8047378541243613848, 0.7773170766911654539, 0.8047378541243613848, 0.7773170766911654539, 0.8047378541243613848, 0.7773170766911654539, 0.8047378541243613848, 0.7773170766911654539, 0.8047378541243613848, 0.7773170766911654539, 0.8047378541243613848, 0.7773170766911654539, 0.8047378541243613848, 0.7773170766911654539, 0.8047378541243613848, 0.7773170766911654539, 0.8047378541243613848, 0.7773170766911654539, 0.8047378541243613848, 0.7773170766911654539, 0.8047378541243613848, 0.7773170766911654539, 0.8047378541243613848, 0.7773170766911654539, 0.8047378541243613848, 0.7773170766911654539, 0.8047378541243613848, 0.7773170766911654539, 0.8047378541243613848, 0.7773170766911654539, 0.8047378541243613848, 0.7773170766911654539, 0.8047378541243613848, 0.7773170766911654539, 0.8047378541243613848, 0.7773170766911654539, 0.8047378541243613848, 0.7773170766911654539, 0.8047378541243613848, 0.7773170766911654539, 0.8047378541243613848, 0.7773170766911654539, 0.8047378541243613848, 0.7773170766911654539, 0.8047378541243613848, 0.7773170766911654539, 0.8047378541243613848, 0.7773170766911654539, 0.8047378541243613848, 0.7773170766911654539, 0.8047378541243613848, 0.7773170766911654539, 0.8047378541243613848, 0.7773170766911654539, 0.8047378541243613848, 0.7773170766911654539, 0.8047378541243613848, 0.7773170766911654539, 0.8047378541243613848, 0.7773170766911654539, 0.8047378541243613848, 0.7773170766911654539, 0.8047378541243613848, 0.7773170766911654539, 0.8047378541243613848, 0.7773170766911654539, 0.8047378541243613848, 0.7773170766911654539, 0.8047378541243613848, 0.7773170766911654539, 0.8047378541243613848, 0.7773170766911654539, 0.8047378541243613848, 0.7773170766911654539, 0.8047378541243613848, 0.7773170766911654539, 0.8047378541243613848, 0.7773170766911654539, 0.8047378541243613848, 0.7773170766911654539, 0.8047378541243613848, 0.7773170766911654539, 0.8047378541243613848, 0.7773170766911654539, 0.8047378541243613848, 0.7773170766911654539, 0.8047378541243613848, 0.7773170766911654539, 0.8047378541243613848, 0.7773170766911654539, 0.8047378541243613848, 0.7773170766911654539, 0.8047378541243613848, 0.7773170766911654539, 0.8047378541243613848, 0.7773170766911654539, 0.8047378541243613848, 0.7773170766911654539, 0.8047378541243613848, 0.7773170766911654539, 0.8047378541243613848, 0.7773170766911654539, 0.8047378541243613848, 0.7773170766911654539, 0.8047378541243613848, 0.7773170766911654539, 0.8047378541243613848, 0.7773170766911654539, 0.8047378541243613848, 0.7773170766911654539, 0.8047378541243613848, 0.7773170766911654539, 0.8047378541243613848, 0.7773170766911654539, 0.8047378541243613848, 0.7773170766911654539, 0.8047378541243613848, 0.7773170766911654539, 0.8047378541243613848, 0.7773170766911654539, 0.8047378541243613848, 0.7773170766911654539, 0.8047378541243613848, 0.7773170766911654539, 0.8047378541243613848, 0.7773170766911654539, 0.8047378541243613848, 0.7773170766911654539, 0.8047378541243613848, 0.7773170766911654539, 0.8047378541243613848, 0.7773170766911654539, 0.8047378541243613848, 0.7773170766911654539, 0.8047378541243613848, 0.7773170766911654539, 0.8047378541243613848, 0.7773170766911654539, 0.8047378541243613848, 0.7773170766911654539, 0.8047378541243613848, 0.7773170766911654539, 0.8047378541243613848, 0.7773170766911654539, 0.8047378541243613848, 0.7773170766911654539, 0.8047378541243613848, 0.7773170766911654539, 0.8047378541243613848, 0.7773170766911654539, 0.8047378541243613848, 0.7773170766911654539, 0.8047378541243613848, 0.7773170766911654539, 0.8047378541243613848, 0.7773170766911654539, 0.8047378541243613848, 0.7773170766911654539, 0.8047378541243613848, 0.7773170766911654539, 0.8047378541243613848, 0.7773170766911654539, 0.8047378541243613848, 0.7773170766911654539, 0.8047378541243613848, 0.7773170766911654539, 0.8047378541243613848, 0.7773170766911654539, 0.8047378541243613848, 0.7773170766911654539, 0.8047378541243613848, 0.7773170766911654539, 0.8047378541243613848, 0.7773170766911654539, 0.8047378541243613848, 0.7773170766911654539, 0.8047378541243613848, 0.7773170766911654539, 0.8047378541243613848, 0.7773170766911654539, 0.8047378541243613848, 0.7773170766911654539, 0.8047378541243613848, 0.7773170766911654539, 0.8047378541243613848, 0.7773170766911654539, 0.8047378541243613848, 0.7773170766911654539, 0.8047378541243613848, 0.7773170766911654539, 0.8047378541243613848, 0.7773170766911654539, 0.8047378541243613848, 0.7773170766911654539, 0.8047378541243613848, 0.7773170766911654539, 0.8047378541243613848, 0.7773170766911654539, 0.8047378541243613848, 0.7773170766911654539, 0.8047378541243613848, 0.7773170766911654539, 0.8047378541243613848, 0.7773170766911654539, 0.8047378541243613848, 0.7773170766911654539, 0.8047378541243613848, 0.7773170766911654539, 0.8047378541243613848, 0.7773170766911654539, 0.8047378541243613848, 0.7773170766911654539, 0.8047378541243613848, 0.7773170766911654539, 0.8047378541243613848, 0.7773170766911654539, 0.8047378541243613848, 0.7773170766911654539, 0.8047378541243613848, 0.7773170766911654539, 0.8047378541243613848, 0.7773170766911654539, 0.8047378541243613848, 0.7773170766911654539, 0.8047378541243613848, 0.7773170766911654539, 0.8047378541243613848, 0.7773170766911654539, 0.8047378541243613848, 0.7773170766911654539, 0.8047378541243613848, 0.7773170766911654539, 0.8047378541243613848, 0.7773170766911654539, 0.8047378541243613848, 0.7773170766911654539, 0.8047378541243613848, 0.7773170766911654539, 0.8047378541243613848, 0.7773170766911654539, 0.8047378541243613848, 0.7773170766911654539, 0.8047378541243613848, 0.7773170766911654539, 0.8047378541243613848, 0.7773170766911654539, 0.8047378541243613848, 0.7773170766911654539, 0.8047378541243613848, 0.7773170766911654539, 0.8047378541243613848, 0.7773170766911654539, 0.8047378541243613848, 0.7773170766911654539, 0.8047378541243613848, 0.7773170766911654539, 0.8047378541243613848, 0.7773170766911654539, 0.8047378541243613848, 0.7773170766911654539, 0.8047378541243613848, 0.7773170766911654539, 0.8047378541243613848, 0.7773170766911654539, 0.8047378541243613848, 0.7773170766911654539, 0.8047378541243613848, 0.7773170766911654539, 0.8047378541243613848, 0.7773170766911654539, 0.8047378541243613848, 0.7773170766911654539, 0.8047378541243613848, 0.7773170766911654539, 0.8047378541243613848, 0.7773170766911654539, 0.8047378541243613848, 0.7773170766911654539, 0.8047378541243613848, 0.7773170766911654539, 0.8047378541243613848, 0.7773170766911654539, 0.8047378541243613848, 0.7773170766911654539, 0.8047378541243613848, 0.7773170766911654539, 0.8047378541243613848, 0.7773170766911654539, 0.8047378541243613848, 0.7773170766911654539, 0.8047378541243613848, 0.7773170766911654539, 0.8047378541243613848, 0.7773170766911654539, 0.8047378541243613848, 0.7773170766911654539, 0.8047378541243613848, 0.7773170766911654539, 0.8047378541243613848, 0.7773170766911654539, 0.8047378541243613848, 0.7773170766911654539, 0.8047378541243613848, 0.7773170766911654539, 0.8047378541243613848, 0.7773170766911654539, 0.8047378541243613848, 0.7773170766911654539, 0.8047378541243613848, 0.7773170766911654539, 0.8047378541243613848, 0.7773170766911654539, 0.8047378541243613848, 0.7773170766911654539, 0.8047378541243613848, 0.7773170766911654539, 0.8047378541243613848, 0.7773170766911654539, 0.8047378541243613848, 0.7773170766911654539, 0.8047378541243613848, 0.7773170766911654539, 0.8047378541243613848, 0.7773170766911654539, 0.8047378541243613848, 0.7773170766911654539, 0.8047378541243613848, 0.7773170766911654539, 0.8047378541243613848, 0.7773170766911654539, 0.8047378541243613848, 0.7773170766911654539, 0.8047378541243613848, 0.7773170766911654539, 0.8047378541243613848, 0.7773170766911654539, 0.8047378541243613848, 0.7773170766911654539, 0.8047378541243613848, 0.7773170766911654539, 0.8047378541243613848, 0.7773170766911654539, 0.8047378541243613848, 0.7773170766911654539, 0.8047378541243613848, 0.7773170766911654539, 0.8047378541243613848, 0.7773170766911654539, 0.8047378541243613848, 0.7773170766911654539, 0.8047378541243613848, 0.7773170766911654539, 0.8047378541243613848, 0.7773170766911654539, 0.8047378541243613848, 0.7773170766911654539, 0.8047378541243613848, 0.7773170766911654539, 0.8047378541243613848, 0.7773170766911654539, 0.8047378541243613848, 0.7773170766911654539, 0.8047378541243613848, 0.7773170766911654539, 0.8047378541243613848, 0.7773170766911654539, 0.8047378541243613848, 0.7773170766911654539, 0.8047378541243613848, 0.7773170766911654539, 0.8047378541243613848, 0.7773170766911654539, 0.8047378541243613848, 0.7773170766911654539, 0.8047378541243613848, 0.7773170766911654539, 0.8047378541243613848, 0.7773170766911654539, 0.8047378541243613848, 0.7773170766911654539, 0.8047378541243613848, 0.7773170766911654539, 0.8047378541243613848, 0.7773170766911654539, 0.8047378541243613848),
 ( 1.000000000000000000, 0.9659258262890683122, 1.000000000000000000, 0.9659258262890683122, 1.000000000000000000, 0.9659258262890683122, 1.000000000000000000, 0.9659258262890683122, 1.000000000000000000, 0.9659258262890683122, 1.000000000000000000, 0.9659258262890683122, 1.000000000000000000, 0.9659258262890683122, 1.000000000000000000, 0.9659258262890683122, 1.000000000000000000, 0.9659258262890683122, 1.000000000000000000, 0.9659258262890683122, 1.000000000000000000, 0.9659258262890683122, 1.000000000000000000, 0.9659258262890683122, 1.000000000000000000, 0.9659258262890683122, 1.000000000000000000, 0.9659258262890683122, 1.000000000000000000, 0.9659258262890683122, 1.000000000000000000, 0.9659258262890683122, 1.000000000000000000, 0.9659258262890683122, 1.000000000000000000, 0.9659258262890683122, 1.000000000000000000, 0.9659258262890683122, 1.000000000000000000, 0.9659258262890683122, 1.000000000000000000, 0.9659258262890683122, 1.000000000000000000, 0.9659258262890683122, 1.000000000000000000, 0.9659258262890683122, 1.000000000000000000, 0.9659258262890683122, 1.000000000000000000, 0.9659258262890683122, 1.000000000000000000, 0.9659258262890683122, 1.000000000000000000, 0.9659258262890683122, 1.000000000000000000, 0.9659258262890683122, 1.000000000000000000, 0.9659258262890683122, 1.000000000000000000, 0.9659258262890683122, 1.000000000000000000, 0.9659258262890683122, 1.000000000000000000, 0.9659258262890683122, 1.000000000000000000, 0.9659258262890683122, 1.000000000000000000, 0.9659258262890683122, 1.000000000000000000, 0.9659258262890683122, 1.000000000000000000, 0.9659258262890683122, 1.000000000000000000, 0.9659258262890683122, 1.000000000000000000, 0.9659258262890683122, 1.000000000000000000, 0.9659258262890683122, 1.000000000000000000, 0.9659258262890683122, 1.000000000000000000, 0.9659258262890683122, 1.000000000000000000, 0.9659258262890683122, 1.000000000000000000, 0.9659258262890683122, 1.000000000000000000, 0.9659258262890683122, 1.000000000000000000, 0.9659258262890683122, 1.000000000000000000, 0.9659258262890683122, 1.000000000000000000, 0.9659258262890683122, 1.000000000000000000, 0.9659258262890683122, 1.000000000000000000, 0.9659258262890683122, 1.000000000000000000, 0.9659258262890683122, 1.000000000000000000, 0.9659258262890683122, 1.000000000000000000, 0.9659258262890683122, 1.000000000000000000, 0.9659258262890683122, 1.000000000000000000, 0.9659258262890683122, 1.000000000000000000, 0.9659258262890683122, 1.000000000000000000, 0.9659258262890683122, 1.000000000000000000, 0.9659258262890683122, 1.000000000000000000, 0.9659258262890683122, 1.000000000000000000, 0.9659258262890683122, 1.000000000000000000, 0.9659258262890683122, 1.000000000000000000, 0.9659258262890683122, 1.000000000000000000, 0.9659258262890683122, 1.000000000000000000, 0.9659258262890683122, 1.000000000000000000, 0.9659258262890683122, 1.000000000000000000, 0.9659258262890683122, 1.000000000000000000, 0.9659258262890683122, 1.000000000000000000, 0.9659258262890683122, 1.000000000000000000, 0.9659258262890683122, 1.000000000000000000, 0.9659258262890683122, 1.000000000000000000, 0.9659258262890683122, 1.000000000000000000, 0.9659258262890683122, 1.000000000000000000, 0.9659258262890683122, 1.000000000000000000, 0.9659258262890683122, 1.000000000000000000, 0.9659258262890683122, 1.000000000000000000, 0.9659258262890683122, 1.000000000000000000, 0.9659258262890683122, 1.000000000000000000, 0.9659258262890683122, 1.000000000000000000, 0.9659258262890683122, 1.000000000000000000, 0.9659258262890683122, 1.000000000000000000, 0.9659258262890683122, 1.000000000000000000, 0.9659258262890683122, 1.000000000000000000, 0.9659258262890683122, 1.000000000000000000, 0.9659258262890683122, 1.000000000000000000, 0.9659258262890683122, 1.000000000000000000, 0.9659258262890683122, 1.000000000000000000, 0.9659258262890683122, 1.000000000000000000, 0.9659258262890683122, 1.000000000000000000, 0.9659258262890683122, 1.000000000000000000, 0.9659258262890683122, 1.000000000000000000, 0.9659258262890683122, 1.000000000000000000, 0.9659258262890683122, 1.000000000000000000, 0.9659258262890683122, 1.000000000000000000, 0.9659258262890683122, 1.000000000000000000, 0.9659258262890683122, 1.000000000000000000, 0.9659258262890683122, 1.000000000000000000, 0.9659258262890683122, 1.000000000000000000, 0.9659258262890683122, 1.000000000000000000, 0.9659258262890683122, 1.000000000000000000, 0.9659258262890683122, 1.000000000000000000, 0.9659258262890683122, 1.000000000000000000, 0.9659258262890683122, 1.000000000000000000, 0.9659258262890683122, 1.000000000000000000, 0.9659258262890683122, 1.000000000000000000, 0.9659258262890683122, 1.000000000000000000, 0.9659258262890683122, 1.000000000000000000, 0.9659258262890683122, 1.000000000000000000, 0.9659258262890683122, 1.000000000000000000, 0.9659258262890683122, 1.000000000000000000, 0.9659258262890683122, 1.000000000000000000, 0.9659258262890683122, 1.000000000000000000, 0.9659258262890683122, 1.000000000000000000, 0.9659258262890683122, 1.000000000000000000, 0.9659258262890683122, 1.000000000000000000, 0.9659258262890683122, 1.000000000000000000, 0.9659258262890683122, 1.000000000000000000, 0.9659258262890683122, 1.000000000000000000, 0.9659258262890683122, 1.000000000000000000, 0.9659258262890683122, 1.000000000000000000, 0.9659258262890683122, 1.000000000000000000, 0.9659258262890683122, 1.000000000000000000, 0.9659258262890683122, 1.000000000000000000, 0.9659258262890683122, 1.000000000000000000, 0.9659258262890683122, 1.000000000000000000, 0.9659258262890683122, 1.000000000000000000, 0.9659258262890683122, 1.000000000000000000, 0.9659258262890683122, 1.000000000000000000, 0.9659258262890683122, 1.000000000000000000, 0.9659258262890683122, 1.000000000000000000, 0.9659258262890683122, 1.000000000000000000, 0.9659258262890683122, 1.000000000000000000, 0.9659258262890683122, 1.000000000000000000, 0.9659258262890683122, 1.000000000000000000, 0.9659258262890683122, 1.000000000000000000, 0.9659258262890683122, 1.000000000000000000, 0.9659258262890683122, 1.000000000000000000, 0.9659258262890683122, 1.000000000000000000, 0.9659258262890683122, 1.000000000000000000, 0.9659258262890683122, 1.000000000000000000, 0.9659258262890683122, 1.000000000000000000, 0.9659258262890683122, 1.000000000000000000, 0.9659258262890683122, 1.000000000000000000, 0.9659258262890683122, 1.000000000000000000, 0.9659258262890683122, 1.000000000000000000, 0.9659258262890683122, 1.000000000000000000, 0.9659258262890683122, 1.000000000000000000, 0.9659258262890683122, 1.000000000000000000, 0.9659258262890683122, 1.000000000000000000, 0.9659258262890683122, 1.000000000000000000, 0.9659258262890683122, 1.000000000000000000, 0.9659258262890683122, 1.000000000000000000, 0.9659258262890683122, 1.000000000000000000, 0.9659258262890683122, 1.000000000000000000, 0.9659258262890683122, 1.000000000000000000, 0.9659258262890683122, 1.000000000000000000, 0.9659258262890683122, 1.000000000000000000, 0.9659258262890683122, 1.000000000000000000, 0.9659258262890683122, 1.000000000000000000, 0.9659258262890683122, 1.000000000000000000, 0.9659258262890683122, 1.000000000000000000, 0.9659258262890683122, 1.000000000000000000, 0.9659258262890683122, 1.000000000000000000, 0.9659258262890683122, 1.000000000000000000, 0.9659258262890683122, 1.000000000000000000, 0.9659258262890683122, 1.000000000000000000, 0.9659258262890683122, 1.000000000000000000, 0.9659258262890683122, 1.000000000000000000, 0.9659258262890683122, 1.000000000000000000, 0.9659258262890683122, 1.000000000000000000, 0.9659258262890683122, 1.000000000000000000, 0.9659258262890683122, 1.000000000000000000, 0.9659258262890683122, 1.000000000000000000, 0.9659258262890683122, 1.000000000000000000, 0.9659258262890683122, 1.000000000000000000, 0.9659258262890683122, 1.000000000000000000, 0.9659258262890683122, 1.000000000000000000, 0.9659258262890683122, 1.000000000000000000, 0.9659258262890683122, 1.000000000000000000, 0.9659258262890683122, 1.000000000000000000, 0.9659258262890683122, 1.000000000000000000, 0.9659258262890683122, 1.000000000000000000, 0.9659258262890683122, 1.000000000000000000, 0.9659258262890683122, 1.000000000000000000, 0.9659258262890683122, 1.000000000000000000, 0.9659258262890683122, 1.000000000000000000, 0.9659258262890683122, 1.000000000000000000, 0.9659258262890683122, 1.000000000000000000, 0.9659258262890683122, 1.000000000000000000, 0.9659258262890683122, 1.000000000000000000, 0.9659258262890683122, 1.000000000000000000, 0.9659258262890683122, 1.000000000000000000, 0.9659258262890683122, 1.000000000000000000, 0.9659258262890683122, 1.000000000000000000, 0.9659258262890683122, 1.000000000000000000, 0.9659258262890683122, 1.000000000000000000, 0.9659258262890683122, 1.000000000000000000, 0.9659258262890683122, 1.000000000000000000, 0.9659258262890683122, 1.000000000000000000, 0.9659258262890683122, 1.000000000000000000, 0.9659258262890683122, 1.000000000000000000, 0.9659258262890683122, 1.000000000000000000, 0.9659258262890683122, 1.000000000000000000, 0.9659258262890683122, 1.000000000000000000, 0.9659258262890683122, 1.000000000000000000, 0.9659258262890683122, 1.000000000000000000, 0.9659258262890683122, 1.000000000000000000, 0.9659258262890683122, 1.000000000000000000, 0.9659258262890683122, 1.000000000000000000, 0.9659258262890683122, 1.000000000000000000, 0.9659258262890683122, 1.000000000000000000, 0.9659258262890683122, 1.000000000000000000, 0.9659258262890683122, 1.000000000000000000, 0.9659258262890683122, 1.000000000000000000, 0.9659258262890683122, 1.000000000000000000, 0.9659258262890683122, 1.000000000000000000, 0.9659258262890683122, 1.000000000000000000, 0.9659258262890683122, 1.000000000000000000, 0.9659258262890683122, 1.000000000000000000, 0.9659258262890683122, 1.000000000000000000, 0.9659258262890683122, 1.000000000000000000, 0.9659258262890683122, 1.000000000000000000, 0.9659258262890683122, 1.000000000000000000, 0.9659258262890683122, 1.000000000000000000, 0.9659258262890683122, 1.000000000000000000, 0.9659258262890683122, 1.000000000000000000, 0.9659258262890683122, 1.000000000000000000, 0.9659258262890683122, 1.000000000000000000, 0.9659258262890683122, 1.000000000000000000, 0.9659258262890683122, 1.000000000000000000, 0.9659258262890683122, 1.000000000000000000, 0.9659258262890683122, 1.000000000000000000, 0.9659258262890683122, 1.000000000000000000, 0.9659258262890683122, 1.000000000000000000, 0.9659258262890683122, 1.000000000000000000, 0.9659258262890683122, 1.000000000000000000, 0.9659258262890683122, 1.000000000000000000, 0.9659258262890683122, 1.000000000000000000, 0.9659258262890683122, 1.000000000000000000) ) ) 
 REPRESENTATION_ITEM ( '' )  SURFACE ( )  );
#47688=DIRECTION ( 'NONE',  ( 1.000000000000000000, 0.000000000000000000, 0.000000000000000000 ) ) ;
#47689=CARTESIAN_POINT ( 'NONE',  ( 0.4724409448818897017, 0.1265901696524990294, -1.069553805774278166 ) ) ;
#47690=CARTESIAN_POINT ( 'NONE',  ( 0.3392501089628018884, -0.1958661417322833942, -1.676528502133545206 ) ) ;
#47696=CARTESIAN_POINT ( 'NONE',  ( 0.1049643490035303689, 0.3917322834645670104, -0.8654855643044619962 ) ) ;
#47705=CARTESIAN_POINT ( 'NONE',  ( 0.2867679344610365999, -0.2867679344610365444, -2.452755905511811108 ) ) ;
#47713=CARTESIAN_POINT ( 'NONE',  ( 0.3917322834645670104, -0.1049643490035303411, -1.298556430446194510 ) ) ;
#47716=CARTESIAN_POINT ( 'NONE',  ( 0.3460692066303958092, 0.1998031496062993018, -2.255249343832020692 ) ) ;
#47733=CARTESIAN_POINT ( 'NONE',  ( -0.3392501089628018329, -0.1958661417322836440, -1.392369135661730262 ) ) ;
#47742=CARTESIAN_POINT ( 'NONE',  ( -0.2867679344610367109, 0.2867679344610365444, -0.4888644601387945876 ) ) ;
#47745=CARTESIAN_POINT ( 'NONE',  ( 0.1265901696524990294, -0.4724409448818896462, -1.736876640419947604 ) ) ;
#47757=DIRECTION ( 'NONE',  ( 1.000000000000000000, 0.000000000000000000, 0.000000000000000000 ) ) ;
#47760=DIRECTION ( 'NONE',  ( 1.000000000000000000, 8.462065736472229849E-17, -0.000000000000000000 ) ) ;
#47764=CARTESIAN_POINT ( 'NONE',  ( -0.3996062992125984925, -0.1070741851644056858, -2.799868766404198794 ) ) ;
#47769=CARTESIAN_POINT ( 'NONE',  ( 0.1070741851644054776, -0.3996062992125984925, -2.051837270341207109 ) ) ;
#47775=CARTESIAN_POINT ( 'NONE',  ( 0.3460692066303959202, 0.1998031496062993295, -1.863517060367454015 ) ) ;
#47776=CARTESIAN_POINT ( 'NONE',  ( -0.2891555358219911054, 0.2891555358219909388, -0.9645669291338583307 ) ) ;
#47777=CARTESIAN_POINT ( 'NONE',  ( 0.1070741851644053527, 0.3996062992125986590, -2.355643044619422533 ) ) ;
#47782=CARTESIAN_POINT ( 'NONE',  ( 0.3949938075777409963, 2.418639510665530743E-17, -2.084645669291338876 ) ) ;
#47786=CARTESIAN_POINT ( 'NONE',  ( -0.1265901696524986964, -0.4724409448818899238, -1.961942257217847763 ) ) ;
#47787=CARTESIAN_POINT ( 'NONE',  ( 0.1265901696524989184, 0.4724409448818898127, -2.747375328083989210 ) ) ;
#47789=EDGE_LOOP ( 'NONE', ( #19857, #82391, #71939, #12523 ) ) ;
#47794=CARTESIAN_POINT ( 'NONE',  ( -9.594673741351310580E-17, 0.3917322834645669549, -2.284757587105299859 ) ) ;
#47801=CARTESIAN_POINT ( 'NONE',  ( 0.2867679344610365999, -0.2867679344610365444, -0.3405511811023621549 ) ) ;
#47804=CARTESIAN_POINT ( 'NONE',  ( 0.1958661417322834775, 0.3392501089628018884, -2.026246719160105236 ) ) ;
#47807=CARTESIAN_POINT ( 'NONE',  ( -0.1974969037888703871, -0.3420746716998661063, -2.270341207349081181 ) ) ;
#47812=CARTESIAN_POINT ( 'NONE',  ( 0.1998031496062994405, -0.3460692066303958092, -0.8792650918635170898 ) ) ;
#47817=CARTESIAN_POINT ( 'NONE',  ( -0.3917322834645671215, 0.1049643490035301469, 0.04002624671916000382 ) ) ;
#47827=DIRECTION ( 'NONE',  ( 1.000000000000000000, 0.000000000000000000, 0.000000000000000000 ) ) ;
#47828=CARTESIAN_POINT ( 'NONE',  ( 0.4091458600556404646, -0.2362204724409448231, -1.364829396325459188 ) ) ;
#47830=CARTESIAN_POINT ( 'NONE',  ( -0.2867679344610364334, -0.2867679344610367109, -0.8385826771653541734 ) ) ;
#47831=CARTESIAN_POINT ( 'NONE',  ( 0.3917322834645669549, 0.1049643490035304660, -2.571522309711285814 ) ) ;
#47834=CARTESIAN_POINT ( 'NONE',  ( -0.3460692066303960313, 0.1998031496062989965, -0.1030183727034120894 ) ) ;
#47839=CARTESIAN_POINT ( 'NONE',  ( 0.3917322834645668994, -0.1049643490035303134, -0.03410141912629739008 ) ) ;
#47841=CARTESIAN_POINT ( 'NONE',  ( 0.3392501089628018329, 0.1958661417322835607, -0.2158792650918636147 ) ) ;
#47846=CARTESIAN_POINT ( 'NONE',  ( -0.1958661417322836718, 0.3392501089628017219, -1.737532808398950079 ) ) ;
#47850=CARTESIAN_POINT ( 'NONE',  ( -0.2362204724409451284, 0.4091458600556402425, -0.5623359580052492701 ) ) ;
#47851=VECTOR ( 'NONE', #75394, 39.37007874015748143 ) ;
#47860=CARTESIAN_POINT ( 'NONE',  ( 0.1070741851644054776, -0.3996062992125984925, -1.736876640419947604 ) ) ;
#47869=CARTESIAN_POINT ( 'NONE',  ( -0.2925321140481930149, -0.2925321140481933480, -0.1358267716535433156 ) ) ;
#47870=CARTESIAN_POINT ( 'NONE',  ( -9.787531504996567848E-17, 0.3996062992125986035, -0.4724409448818898127 ) ) ;
#47871=CARTESIAN_POINT ( 'NONE',  ( -0.1049643490035302301, -0.3917322834645671770, -2.746082307907824038 ) ) ;
#47876=CARTESIAN_POINT ( 'NONE',  ( -9.674558042662122972E-17, 0.3949938075777409963, -1.021653543307086798 ) ) ;
#47881=CARTESIAN_POINT ( 'NONE',  ( -0.4724409448818899238, 0.1265901696524986686, -0.8202099737532806412 ) ) ;
#47882=CARTESIAN_POINT ( 'NONE',  ( -0.2925321140481932369, 0.2925321140481931814, -2.066929133858267598 ) ) ;
#47885=CARTESIAN_POINT ( 'NONE',  ( 0.3917322834645670104, 0.1049643490035304660, -0.4363710218185846146 ) ) ;
#47898=CARTESIAN_POINT ( 'NONE',  ( 0.3917322834645669549, 0.1049643490035304660, -0.4317585301837270628 ) ) ;
#47901=CARTESIAN_POINT ( 'NONE',  ( 0.3949938075777409963, 2.418639510665530435E-17, -1.062992125984251857 ) ) ;
#47915=CARTESIAN_POINT ( 'NONE',  ( -0.4724409448818898682, -8.678599364036362592E-17, -0.5885826771653542844 ) ) ;
#47920=CARTESIAN_POINT ( 'NONE',  ( 0.1070741851644053527, 0.3996062992125986590, -1.883202099737532276 ) ) ;
#47923=CARTESIAN_POINT ( 'NONE',  ( -0.2925321140481932369, 0.2925321140481931259, -1.356299212598425230 ) ) ;
#47924=CARTESIAN_POINT ( 'NONE',  ( 0.3996062992125984925, 0.1070741851644054637, -0.6738845144356955252 ) ) ;
#47927=CARTESIAN_POINT ( 'NONE',  ( -0.1265901696524986964, -0.4724409448818899238, 0.08530183727034119923 ) ) ;
#47929=CARTESIAN_POINT ( 'NONE',  ( -0.3917322834645669549, -0.1049643490035306603, -2.492782152230970993 ) ) ;
#47936=CARTESIAN_POINT ( 'NONE',  ( 0.4724409448818896462, 0.1265901696524990294, -1.776246719160104570 ) ) ;
#47939=CARTESIAN_POINT ( 'NONE',  ( 0.1974969037888704704, 0.3420746716998660508, -1.638451443569553634 ) ) ;
#47949=CARTESIAN_POINT ( 'NONE',  ( 0.3460692066303958092, 0.1998031496062993018, -2.412729658792650778 ) ) ;
#47950=CARTESIAN_POINT ( 'NONE',  ( 0.3917322834645668994, -0.1049643490035303134, -2.396306143535746447 ) ) ;
#47959=CARTESIAN_POINT ( 'NONE',  ( -0.4091458600556402980, -0.2362204724409451284, -0.8398950131233595684 ) ) ;
#47963=EDGE_CURVE ( 'NONE', #7865, #65743, #77809, .T. ) ;
#47964=CARTESIAN_POINT ( 'NONE',  ( 4.893765752498283308E-17, -0.3996062992125985480, -0.3129921259842520231 ) ) ;
#47967=CARTESIAN_POINT ( 'NONE',  ( 0.3392501089628018884, -0.1958661417322834220, -1.764435695538057791 ) ) ;
#47978=CARTESIAN_POINT ( 'NONE',  ( 0.1998031496062994128, -0.3460692066303957537, -0.7985564304461942875 ) ) ;
#47993=CARTESIAN_POINT ( 'NONE',  ( -0.3996062992125986035, -0.1070741851644056997, -0.3608923884514435576 ) ) ;
#47996=CARTESIAN_POINT ( 'NONE',  ( -0.2867679344610364334, -0.2867679344610367109, -2.413385826771653253 ) ) ;
#47997=VERTEX_POINT ( 'NONE', #63501 ) ;
#48003=CARTESIAN_POINT ( 'NONE',  ( -0.1265901696524986964, -0.4724409448818899238, -2.038713910761154491 ) ) ;
#48006=CARTESIAN_POINT ( 'NONE',  ( -9.594673741351310580E-17, 0.3917322834645669549, -1.654836327262780182 ) ) ;
#48012=CARTESIAN_POINT ( 'NONE',  ( -0.2867679344610365444, -0.2867679344610367664, -2.732958948327771420 ) ) ;
#48014=ORIENTED_EDGE ( 'NONE', *, *, #35272, .F. ) ;
#48020=CARTESIAN_POINT ( 'NONE',  ( 0.3917322834645670659, -0.1049643490035303273, -1.368129552002311788 ) ) ;
#48022=CARTESIAN_POINT ( 'NONE',  ( -0.3917322834645669549, -0.1049643490035306603, -2.177821522309711266 ) ) ;
#48029=CARTESIAN_POINT ( 'NONE',  ( 0.1998031496062992463, 0.3460692066303959202, 0.09383202099737532331 ) ) ;
#48031=CARTESIAN_POINT ( 'NONE',  ( 0.2925321140481932369, 0.2925321140481932369, -1.870078740157480546 ) ) ;
#48037=CARTESIAN_POINT ( 'NONE',  ( 0.4724409448818896462, 0.1265901696524990294, -0.6738845144356955252 ) ) ;
#48040=CARTESIAN_POINT ( 'NONE',  ( 0.1058382717557499880, 0.3949938075777409408, -0.7001312335958006505 ) ) ;
#48046=CARTESIAN_POINT ( 'NONE',  ( 0.2891555358219910499, -0.2891555358219909944, -0.6476377952755905110 ) ) ;
#48053=CARTESIAN_POINT ( 'NONE',  ( -0.1998031496062991630, -0.3460692066303959202, -1.244750656167979086 ) ) ;
#48055=CARTESIAN_POINT ( 'NONE',  ( -0.1958661417322836718, 0.3392501089628017219, -0.9501312335958004285 ) ) ;
#48069=CARTESIAN_POINT ( 'NONE',  ( 0.3458507752293908943, -0.3458507752293908943, -0.3326771653543306728 ) ) ;
#48087=EDGE_CURVE ( 'NONE', #71224, #21828, #67860, .T. ) ;
#48088=CARTESIAN_POINT ( 'NONE',  ( -0.3458507752293906723, -0.3458507752293910609, 0.09842519685039372024 ) ) ;
#48089=CARTESIAN_POINT ( 'NONE',  ( -0.3949938075777411628, 0.1058382717557497937, -2.237532808398950301 ) ) ;
#48092=CARTESIAN_POINT ( 'NONE',  ( -9.594673741351313045E-17, 0.3917322834645670104, -0.9370078740157480324 ) ) ;
#48100=CARTESIAN_POINT ( 'NONE',  ( -0.3392501089628018329, -0.1958661417322836440, -0.2900069309373210502 ) ) ;
#48107=CARTESIAN_POINT ( 'NONE',  ( -0.4724409448818899238, 0.1265901696524986964, -0.03280839895013123314 ) ) ;
#48108=CARTESIAN_POINT ( 'NONE',  ( 0.4091458600556403535, 0.2362204724409449896, -1.076115485564304475 ) ) ;
#48109=CARTESIAN_POINT ( 'NONE',  ( 0.1049643490035303967, 0.3917322834645670659, -1.722460260663728926 ) ) ;
#48115=CARTESIAN_POINT ( 'NONE',  ( -0.3917322834645669549, -0.1049643490035306603, -0.9179790026246721357 ) ) ;
#48125=CARTESIAN_POINT ( 'NONE',  ( -0.3392501089628019995, 0.1958661417322832277, -2.538057742782152015 ) ) ;
#48131=CARTESIAN_POINT ( 'NONE',  ( 0.4724409448818899238, -0.1265901696524985298, -0.03083989501312338691 ) ) ;
#48133=CARTESIAN_POINT ( 'NONE',  ( 0.1049643490035304938, -0.3917322834645669549, -1.429790026246719359 ) ) ;
#48134=ADVANCED_FACE ( 'NONE', ( #64331 ), #82351, .T. ) ;
#48135=CARTESIAN_POINT ( 'NONE',  ( -0.1070741851644056997, 0.3996062992125984925, -2.445538057742782101 ) ) ;
#48144=CARTESIAN_POINT ( 'NONE',  ( 0.3911666210184634451, 0.1216921365961784601, -1.934761428466221123 ) ) ;
#48147=CARTESIAN_POINT ( 'NONE',  ( 0.1049643490035303689, 0.3917322834645670104, 0.01443569553805778768 ) ) ;
#48155=CARTESIAN_POINT ( 'NONE',  ( 0.3917322834645668994, -0.1049643490035303134, -1.136463623850706650 ) ) ;
#48164=CARTESIAN_POINT ( 'NONE',  ( -0.3392501089628019995, 0.1958661417322831999, -0.3379458249681908666 ) ) ;
#48167=CARTESIAN_POINT ( 'NONE',  ( -0.4091458600556405756, 0.2362204724409446288, -1.520341207349081181 ) ) ;
#48182=ORIENTED_EDGE ( 'NONE', *, *, #42744, .F. ) ;
#48187=CARTESIAN_POINT ( 'NONE',  ( 0.1998031496062994128, -0.3460692066303957537, -2.058398950131233640 ) ) ;
#48191=LINE ( 'NONE', #24064, #11690 ) ;
#48193=CARTESIAN_POINT ( 'NONE',  ( 0.3996062992125986035, 0.1070741851644054776, -1.856955380577427928 ) ) ;
#48194=CARTESIAN_POINT ( 'NONE',  ( 0.1974969037888706369, -0.3420746716998659953, -0.8792650918635170898 ) ) ;
#48195=CARTESIAN_POINT ( 'NONE',  ( 0.3996062992125986035, 0.1070741851644054776, -2.644356955380577912 ) ) ;
#48198=CARTESIAN_POINT ( 'NONE',  ( -0.2867679344610366554, 0.2867679344610365444, -0.3267716535433070058 ) ) ;
#48202=CARTESIAN_POINT ( 'NONE',  ( 0.1974969037888704704, 0.3420746716998660508, -2.268372703412073754 ) ) ;
#48206=CARTESIAN_POINT ( 'NONE',  ( 0.3458507752293908943, -0.3458507752293908943, -2.460629921259842146 ) ) ;
#48207=CARTESIAN_POINT ( 'NONE',  ( -0.3460692066303960868, 0.1998031496062990242, -1.916010498687664043 ) ) ;
#48215=CARTESIAN_POINT ( 'NONE',  ( 0.1958661417322836162, -0.3392501089628018329, -2.691581734086927469 ) ) ;
#48218=CARTESIAN_POINT ( 'NONE',  ( -0.2362204724409447953, -0.4091458600556404646, -2.427821522309711266 ) ) ;
#48222=CARTESIAN_POINT ( 'NONE',  ( -0.1958661417322836718, 0.3392501089628017219, -0.09776902887139117537 ) ) ;
#48224=CARTESIAN_POINT ( 'NONE',  ( 0.3392501089628018884, -0.1958661417322834220, -2.301837270341207553 ) ) ;
#48227=CARTESIAN_POINT ( 'NONE',  ( 0.3420746716998660508, -0.1974969037888703871, -2.152230971128608950 ) ) ;
#48228=ORIENTED_EDGE ( 'NONE', *, *, #55825, .F. ) ;
#48231=CARTESIAN_POINT ( 'NONE',  ( -0.1998031496062991907, -0.3460692066303959757, -1.167979002624671914 ) ) ;
#48235=CARTESIAN_POINT ( 'NONE',  ( 0.4724409448818898682, 0.000000000000000000, -2.755905511811024056 ) ) ;
#48236=CARTESIAN_POINT ( 'NONE',  ( 0.1049643490035304938, -0.3917322834645669549, -0.1699475065616798397 ) ) ;
#48242=CARTESIAN_POINT ( 'NONE',  ( 0.1049643490035304938, -0.3917322834645669549, 0.08005249343832024356 ) ) ;
#48246=CARTESIAN_POINT ( 'NONE',  ( 0.3458507752293908943, -0.3458507752293908943, -1.515748031496062742 ) ) ;
#48248=CARTESIAN_POINT ( 'NONE',  ( 4.797336870675656522E-17, -0.3917322834645670104, -0.7007874015748030150 ) ) ;
#48253=CARTESIAN_POINT ( 'NONE',  ( -0.4724409448818896462, -0.1265901696524993070, -1.935695538057742526 ) ) ;
#48256=CARTESIAN_POINT ( 'NONE',  ( -0.1958661417322834497, -0.3392501089628018884, 0.01183033940388633805 ) ) ;
#48258=CARTESIAN_POINT ( 'NONE',  ( -0.1958661417322836718, 0.3392501089628017219, -0.5702099737532808632 ) ) ;
#48263=CARTESIAN_POINT ( 'NONE',  ( -0.3392501089628017219, -0.1958661417322836718, -2.249343832020997525 ) ) ;
#48266=CARTESIAN_POINT ( 'NONE',  ( 0.4724409448818897572, -0.1265901696524988906, -0.1883202099737532054 ) ) ;
#48274=CARTESIAN_POINT ( 'NONE',  ( -0.4724409448818882584, 0.1265901696525017217, -1.999343832020997525 ) ) ;
#48276=CARTESIAN_POINT ( 'NONE',  ( 0.3460692066303958092, 0.1998031496062993018, -1.467847769028871596 ) ) ;
#48283=( BOUNDED_CURVE ( )  B_SPLINE_CURVE ( 1, ( #62352, #4690 ),
 .UNSPECIFIED., .F., .F. ) 
 B_SPLINE_CURVE_WITH_KNOTS ( ( 2, 2 ),
 ( 1.738108305489988542E-18, 0.001850000000000003118 ),
 .UNSPECIFIED. ) 
 CURVE ( )  GEOMETRIC_REPRESENTATION_ITEM ( )  RATIONAL_B_SPLINE_CURVE ( ( 0.9911642120908008557, 0.9911642120908008557 ) ) 
 REPRESENTATION_ITEM ( '' )  );
#48286=CARTESIAN_POINT ( 'NONE',  ( 0.3996062992125985480, 2.446882876249141654E-17, -0.3523622047244094335 ) ) ;
#48287=EDGE_CURVE ( 'NONE', #81066, #64662, #57002, .T. ) ;
#48288=CARTESIAN_POINT ( 'NONE',  ( -0.2925321140481932924, 0.2925321140481931814, -0.6496062992125984925 ) ) ;
#48289=CARTESIAN_POINT ( 'NONE',  ( -0.3949938075777411628, 0.1058382717557497937, 0.1246719160104986374 ) ) ;
#48294=CARTESIAN_POINT ( 'NONE',  ( -0.1058382717557497660, -0.3949938075777411073, -1.093832020997375309 ) ) ;
#48299=CARTESIAN_POINT ( 'NONE',  ( -0.4724409448818899238, 0.1265901696524986686, -1.135170603674540590 ) ) ;
#48300=CARTESIAN_POINT ( 'NONE',  ( 0.3996062992125985480, 0.1070741851644054637, -2.171916010498687211 ) ) ;
#48303=CARTESIAN_POINT ( 'NONE',  ( 4.797336870675656522E-17, -0.3917322834645670659, -0.2329589483277709483 ) ) ;
#48314=CARTESIAN_POINT ( 'NONE',  ( -0.3392501089628017219, -0.1958661417322836718, -1.146981627296587813 ) ) ;
#48317=CARTESIAN_POINT ( 'NONE',  ( -0.3420746716998659953, -0.1974969037888706647, -1.154855643044619518 ) ) ;
#48333=CARTESIAN_POINT ( 'NONE',  ( 0.1070741851644053527, 0.3996062992125986590, -1.725721784776903078 ) ) ;
#48336=CARTESIAN_POINT ( 'NONE',  ( -0.3996062992125986590, 0.1070741851644051723, -1.211942257217847541 ) ) ;
#48340=CARTESIAN_POINT ( 'NONE',  ( 0.4091458600556404646, -0.2362204724409448231, -0.2624671916010498651 ) ) ;
#48341=CARTESIAN_POINT ( 'NONE',  ( -9.594673741351313045E-17, 0.3917322834645670104, -2.604330708661416693 ) ) ;
#48347=CARTESIAN_POINT ( 'NONE',  ( -0.1265901696524986964, -0.4724409448818899238, -2.196194225721784576 ) ) ;
#48350=CARTESIAN_POINT ( 'NONE',  ( 0.3949938075777409963, 2.418639510665530743E-17, -1.927165354330708569 ) ) ;
#48360=CARTESIAN_POINT ( 'NONE',  ( 0.1958661417322834497, 0.3392501089628018329, -2.586594857446507412 ) ) ;
#48373=CARTESIAN_POINT ( 'NONE',  ( -0.3996062992125984925, -0.1070741851644056858, -0.1227034120734908362 ) ) ;
#48376=CARTESIAN_POINT ( 'NONE',  ( 4.797336870675656522E-17, -0.3917322834645670104, -1.895669291338582640 ) ) ;
#48385=CARTESIAN_POINT ( 'NONE',  ( -0.1998031496062991630, -0.3460692066303959202, -1.087270341207349000 ) ) ;
#48393=CARTESIAN_POINT ( 'NONE',  ( -0.1958661417322834220, -0.3392501089628018884, -1.725065616797900381 ) ) ;
#48394=CARTESIAN_POINT ( 'NONE',  ( -0.1265901696524986964, -0.4724409448818899238, -2.119422572178477626 ) ) ;
#48398=CARTESIAN_POINT ( 'NONE',  ( -9.787531504996566615E-17, 0.3996062992125985480, -2.596456692913385655 ) ) ;
#48400=CARTESIAN_POINT ( 'NONE',  ( -0.3460692066303960868, 0.1998031496062990242, -0.4986876640419947715 ) ) ;
#48403=CARTESIAN_POINT ( 'NONE',  ( 0.2867679344610365999, -0.2867679344610365444, -2.295275590551181022 ) ) ;
#48404=ORIENTED_EDGE ( 'NONE', *, *, #17250, .F. ) ;
#48413=CARTESIAN_POINT ( 'NONE',  ( 0.2867679344610365999, -0.2867679344610365999, -1.753261524113173708 ) ) ;
#48421=CARTESIAN_POINT ( 'NONE',  ( -9.674558042662121740E-17, 0.3949938075777409963, 0.1574803149606298636 ) ) ;
#48430=CARTESIAN_POINT ( 'NONE',  ( 0.3392501089628018329, 0.1958661417322835607, -1.387814591372390272 ) ) ;
#48432=CARTESIAN_POINT ( 'NONE',  ( -0.2867679344610364334, -0.2867679344610367109, -2.348425196850393970 ) ) ;
#48440=CARTESIAN_POINT ( 'NONE',  ( -0.3996062992125986035, -7.340648628747425578E-17, -1.771653543307086576 ) ) ;
#48445=CARTESIAN_POINT ( 'NONE',  ( -0.4091458600556405756, 0.2362204724409446288, -0.7329396325459317518 ) ) ;
#48448=CARTESIAN_POINT ( 'NONE',  ( -0.1974969037888704149, -0.3420746716998661063, -0.4573490813648294906 ) ) ;
#48453=CARTESIAN_POINT ( 'NONE',  ( 0.3420746716998660508, 0.1974969037888705814, -0.6804461942257220564 ) ) ;
#48461=CARTESIAN_POINT ( 'NONE',  ( -0.1070741851644056997, 0.3996062992125984925, -1.500656167979002253 ) ) ;
#48463=CARTESIAN_POINT ( 'NONE',  ( 0.3917322834645670104, -0.1049643490035303411, -1.048556430446194287 ) ) ;
#48478=FACE_OUTER_BOUND ( 'NONE', #5225, .T. ) ;
#48495=CARTESIAN_POINT ( 'NONE',  ( 0.1265901696524990294, -0.4724409448818896462, -0.08530183727034119923 ) ) ;
#48496=CARTESIAN_POINT ( 'NONE',  ( -0.1058382717557497937, -0.3949938075777411628, -2.434383202099737353 ) ) ;
#48499=CARTESIAN_POINT ( 'NONE',  ( 0.1958661417322834775, 0.3392501089628018884, -1.081364829396325389 ) ) ;
#48501=CARTESIAN_POINT ( 'NONE',  ( -0.3458507752293906723, -0.3458507752293910609, -2.421259842519684735 ) ) ;
#48509=CARTESIAN_POINT ( 'NONE',  ( -9.594673741351310580E-17, 0.3917322834645669549, -0.3949938075777409963 ) ) ;
#48516=CARTESIAN_POINT ( 'NONE',  ( 0.1998031496062994405, -0.3460692066303958092, -2.926509186351706315 ) ) ;
#48517=CARTESIAN_POINT ( 'NONE',  ( 0.2867679344610366554, -0.2867679344610365999, -1.512486507382889256 ) ) ;
#48523=CARTESIAN_POINT ( 'NONE',  ( 4.797336870675656522E-17, -0.3917322834645670104, -0.9507874015748032370 ) ) ;
#48531=CARTESIAN_POINT ( 'NONE',  ( -0.1265901696524986964, -0.4724409448818899238, -0.9363517060367454459 ) ) ;
#48532=CARTESIAN_POINT ( 'NONE',  ( 0.2867679344610365999, -0.2867679344610365444, -2.295275590551181022 ) ) ;
#48540=CARTESIAN_POINT ( 'NONE',  ( 4.797336870675656522E-17, -0.3917322834645670104, -0.9507874015748032370 ) ) ;
#48544=CARTESIAN_POINT ( 'NONE',  ( -0.3392501089628019995, 0.1958661417322832277, -1.528215223097112885 ) ) ;
#48546=CARTESIAN_POINT ( 'NONE',  ( 0.2925321140481932369, -0.2925321140481931814, -2.222440944881889813 ) ) ;
#48556=CARTESIAN_POINT ( 'NONE',  ( 0.2925321140481931814, 0.2925321140481931814, -1.946850393700787496 ) ) ;
#48558=CARTESIAN_POINT ( 'NONE',  ( 0.1958661417322836440, -0.3392501089628017219, 0.07349081364829400387 ) ) ;
#48565=CARTESIAN_POINT ( 'NONE',  ( -0.1958661417322836440, 0.3392501089628016664, -1.195518741960943210 ) ) ;
#48574=CARTESIAN_POINT ( 'NONE',  ( 0.2867679344610366554, -0.2867679344610365999, -0.4101243026584795448 ) ) ;
#48578=CARTESIAN_POINT ( 'NONE',  ( -1.157146581871515012E-16, 0.4724409448818898682, -2.124015748031495843 ) ) ;
#48588=LINE ( 'NONE', #68386, #43397 ) ;
#48591=CYLINDRICAL_SURFACE ( 'NONE', #59538, 0.4724409448818898682 ) ;
#48598=CARTESIAN_POINT ( 'NONE',  ( -9.787531504996567848E-17, 0.3996062992125986035, -1.920830620545185230E-17 ) ) ;
#48599=CARTESIAN_POINT ( 'NONE',  ( 0.3996062992125984925, 0.1070741851644054637, -2.091207349081364963 ) ) ;
#48605=CARTESIAN_POINT ( 'NONE',  ( -0.2925321140481932924, 0.2925321140481931814, -1.594488188976378229 ) ) ;
#48606=CARTESIAN_POINT ( 'NONE',  ( -0.1058382717557497937, -0.3949938075777411628, -1.017060367454068359 ) ) ;
#48607=CARTESIAN_POINT ( 'NONE',  ( -0.1070741851644051862, -0.3996062992125987146, -2.276902887139107268 ) ) ;
#48608=CARTESIAN_POINT ( 'NONE',  ( 0.2362204724409449064, 0.4091458600556404646, -0.6167979002624671692 ) ) ;
#48609=CARTESIAN_POINT ( 'NONE',  ( -0.1049643490035301885, -0.3917322834645671215, -0.06430446194225716838 ) ) ;
#48614=CARTESIAN_POINT ( 'NONE',  ( 0.3949938075777409408, -0.1058382717557499186, -2.078083989501312345 ) ) ;
#48618=CARTESIAN_POINT ( 'NONE',  ( -0.4724409448818899238, 0.1265901696524986686, -2.237532808398950301 ) ) ;
#48619=CARTESIAN_POINT ( 'NONE',  ( -0.2925321140481930704, -0.2925321140481933480, -1.948818897637795144 ) ) ;
#48626=CARTESIAN_POINT ( 'NONE',  ( 0.2867679344610365999, -0.2867679344610365999, -2.698143413876953556 ) ) ;
#48633=CARTESIAN_POINT ( 'NONE',  ( -0.1049643490035302024, -0.3917322834645671215, -0.1568241469816273603 ) ) ;
#48635=CARTESIAN_POINT ( 'NONE',  ( -0.1049643490035302024, -0.3917322834645671215, -2.111548556430446144 ) ) ;
#48639=CARTESIAN_POINT ( 'NONE',  ( 0.1058382717557500713, -0.3949938075777409408, -2.604986876640420501 ) ) ;
#48643=CARTESIAN_POINT ( 'NONE',  ( 0.3460692066303959202, 0.1998031496062993295, -1.076115485564304475 ) ) ;
#48645=CARTESIAN_POINT ( 'NONE',  ( 0.4091458600556404646, -0.2362204724409448231, -0.8116797900262466836 ) ) ;
#48647=CARTESIAN_POINT ( 'NONE',  ( 0.005815251566305920140, -0.3972027188793976760, -2.755905511808609099 ) ) ;
#48648=CARTESIAN_POINT ( 'NONE',  ( 0.1958661417322834775, 0.3392501089628018884, 0.08595800524934374409 ) ) ;
#48654=CARTESIAN_POINT ( 'NONE',  ( 0.3392501089628018329, 0.1958661417322835607, 0.03412073490813653104 ) ) ;
#48658=CARTESIAN_POINT ( 'NONE',  ( 0.4091458600556404646, -0.2362204724409448231, -1.679790026246719137 ) ) ;
#48659=CARTESIAN_POINT ( 'NONE',  ( -1.157146581871515012E-16, 0.4724409448818898682, 0.000000000000000000 ) ) ;
#48660=CARTESIAN_POINT ( 'NONE',  ( -0.3917322834645671215, 0.1049643490035301469, -0.8123359580052491591 ) ) ;
#48661=CARTESIAN_POINT ( 'NONE',  ( -0.1049643490035301885, -0.3917322834645671215, -2.676509186351705871 ) ) ;
#48669=CARTESIAN_POINT ( 'NONE',  ( -0.1958661417322834497, -0.3392501089628018884, -0.1456499755567436105 ) ) ;
#48671=CARTESIAN_POINT ( 'NONE',  ( 0.1049643490035304799, -0.3917322834645669549, -0.4849081364829397334 ) ) ;
#48676=AXIS2_PLACEMENT_3D ( 'NONE', #32003, #76626, #69890 ) ;
#48678=CARTESIAN_POINT ( 'NONE',  ( -0.3917322834645670104, -7.196005306013484475E-17, -2.393700787401574992 ) ) ;
#48681=CARTESIAN_POINT ( 'NONE',  ( -0.4724409448818898682, -8.678599364036362592E-17, -0.7460629921259841479 ) ) ;
#48684=CARTESIAN_POINT ( 'NONE',  ( -0.4724409448818898682, -8.678599364036362592E-17, -0.6692913385826770867 ) ) ;
#48691=CARTESIAN_POINT ( 'NONE',  ( -0.1070741851644051862, -0.3996062992125986590, -2.038713910761154491 ) ) ;
#48699=CARTESIAN_POINT ( 'NONE',  ( -0.3996062992125986035, 0.1070741851644051584, -0.1095800524934383430 ) ) ;
#48700=CARTESIAN_POINT ( 'NONE',  ( 0.3460692066303959757, -0.1998031496062991907, -0.4199475065616797842 ) ) ;
#48701=CARTESIAN_POINT ( 'NONE',  ( 0.1974969037888706369, -0.3420746716998659953, 0.06561679790026241077 ) ) ;
#48708=CARTESIAN_POINT ( 'NONE',  ( 0.3949938075777409408, -0.1058382717557499186, -0.9757217847769031893 ) ) ;
#48713=CARTESIAN_POINT ( 'NONE',  ( -0.4724409448818899238, 0.1265901696524986686, -0.9776902887139107268 ) ) ;
#48714=CARTESIAN_POINT ( 'NONE',  ( 0.3460692066303959757, -0.1998031496062991907, -2.467191601049868677 ) ) ;
#48717=CARTESIAN_POINT ( 'NONE',  ( -0.2867679344610367109, 0.2867679344610365444, -0.8038250900600545368 ) ) ;
#48729=CARTESIAN_POINT ( 'NONE',  ( -0.3392501089628017219, -0.1958661417322836718, -0.8320209973753279753 ) ) ;
#48732=CARTESIAN_POINT ( 'NONE',  ( -0.3420746716998661618, 0.1974969037888702206, -1.443569553805774230 ) ) ;
#48736=CARTESIAN_POINT ( 'NONE',  ( -9.787531504996567848E-17, 0.3996062992125986035, 0.1574803149606299191 ) ) ;
#48742=CARTESIAN_POINT ( 'NONE',  ( 0.2362204724409449064, 0.4091458600556404646, -0.3786089238845143923 ) ) ;
#48743=CARTESIAN_POINT ( 'NONE',  ( -0.1265901696524986964, -0.4724409448818899238, -0.6213910761154856077 ) ) ;
#48748=CARTESIAN_POINT ( 'NONE',  ( 0.2925321140481932369, -0.2925321140481932369, -1.830708661417322913 ) ) ;
#48750=ORIENTED_EDGE ( 'NONE', *, *, #67228, .T. ) ;
#48751=CARTESIAN_POINT ( 'NONE',  ( -0.1070741851644056997, 0.3996062992125984925, -1.028215223097112663 ) ) ;
#48755=CARTESIAN_POINT ( 'NONE',  ( 0.4091458600556404646, -0.2362204724409448231, -0.4199475065616797842 ) ) ;
#48757=CARTESIAN_POINT ( 'NONE',  ( -0.3917322834645670104, -7.196005306013484475E-17, -2.328740157480315265 ) ) ;
#48763=CARTESIAN_POINT ( 'NONE',  ( 0.4091458600556404646, -0.2362204724409448231, -2.386482939632545985 ) ) ;
#48766=CARTESIAN_POINT ( 'NONE',  ( 0.1058382717557500852, -0.3949938075777408852, -1.894356955380577245 ) ) ;
#48776=CARTESIAN_POINT ( 'NONE',  ( 0.1958661417322836162, -0.3392501089628018329, -2.534101419126297827 ) ) ;
#48791=CARTESIAN_POINT ( 'NONE',  ( -0.1070741851644056997, 0.3996062992125984925, -0.3982939632545932085 ) ) ;
#48793=CARTESIAN_POINT ( 'NONE',  ( 0.3917322834645669549, 0.1049643490035304660, -1.941601049868766582 ) ) ;
#48802=CARTESIAN_POINT ( 'NONE',  ( -0.3996062992125986590, 0.1070741851644051723, -1.369422572178477404 ) ) ;
#48804=CARTESIAN_POINT ( 'NONE',  ( -0.1265901696524993347, 0.4724409448818896462, -2.211286089238845065 ) ) ;
#48809=CARTESIAN_POINT ( 'NONE',  ( 4.797336870675656522E-17, -0.3917322834645670104, -1.738188976377952777 ) ) ;
#48810=CARTESIAN_POINT ( 'NONE',  ( 0.3458507752293908943, -0.3458507752293908943, -2.145669291338582418 ) ) ;
#48813=CARTESIAN_POINT ( 'NONE',  ( 0.06192927228921586008, -0.3917322834645669549, -2.751902906291787687 ) ) ;
#48814=CARTESIAN_POINT ( 'NONE',  ( 0.1070741851644053527, 0.3996062992125985480, -2.432414698162729483 ) ) ;
#48816=CARTESIAN_POINT ( 'NONE',  ( 0.2925321140481932369, -0.2925321140481932369, -0.8858267716535430658 ) ) ;
#48819=CARTESIAN_POINT ( 'NONE',  ( 0.3917322834645670104, -0.1049643490035303411, -2.623359580052493367 ) ) ;
#48829=CARTESIAN_POINT ( 'NONE',  ( -0.3392501089628019439, 0.1958661417322832554, -1.366122416501625469 ) ) ;
#48833=CARTESIAN_POINT ( 'NONE',  ( -0.3917322834645671215, 0.1049643490035301469, -2.637139107611548461 ) ) ;
#48835=VERTEX_POINT ( 'NONE', #29168 ) ;
#48836=CARTESIAN_POINT ( 'NONE',  ( 0.3917322834645670659, 2.398668435337828261E-17, -2.792014066438007092 ) ) ;
#48845=CARTESIAN_POINT ( 'NONE',  ( 0.3392501089628018329, 0.1958661417322835607, -1.230334276411760186 ) ) ;
#48847=CARTESIAN_POINT ( 'NONE',  ( 0.1049643490035303689, 0.3917322834645670104, -2.440288713910760521 ) ) ;
#48852=CARTESIAN_POINT ( 'NONE',  ( -0.3996062992125987146, 0.1070741851644051862, -0.3477690288713909950 ) ) ;
#48854=CARTESIAN_POINT ( 'NONE',  ( -0.1998031496062991630, -0.3460692066303959202, 0.1725721784776902690 ) ) ;
#48856=CARTESIAN_POINT ( 'NONE',  ( -0.3996062992125986035, -0.1070741851644056997, -2.250656167979002920 ) ) ;
#48857=EDGE_CURVE ( 'NONE', #25753, #35562, #65661, .T. ) ;
#48862=CARTESIAN_POINT ( 'NONE',  ( -0.4724409448818895907, -0.1265901696524993070, -0.9101049868766404316 ) ) ;
#48865=ADVANCED_FACE ( 'NONE', ( #61984 ), #80127, .F. ) ;
#48866=CARTESIAN_POINT ( 'NONE',  ( -0.2891555358219909388, -0.2891555358219912164, -0.6082677165354331006 ) ) ;
#48875=CARTESIAN_POINT ( 'NONE',  ( -0.1265901696524986964, -0.4724409448818899238, -0.1489501312335957672 ) ) ;
#48879=CARTESIAN_POINT ( 'NONE',  ( 0.3996062992125984925, 0.1070741851644054637, -1.933727034120735100 ) ) ;
#48881=CARTESIAN_POINT ( 'NONE',  ( -0.3917322834645670104, -7.196005306013484475E-17, -0.9763779527559053317 ) ) ;
#48883=CARTESIAN_POINT ( 'NONE',  ( -0.3089825338611873473, 0.2417350488526503194, 6.867566722516314874E-18 ) ) ;
#48903=CARTESIAN_POINT ( 'NONE',  ( -0.3917322834645670659, -7.196005306013484475E-17, -2.083352649115172373 ) ) ;
#48907=( BOUNDED_SURFACE ( )  B_SPLINE_SURFACE ( 3, 2, ( 
 ( #13089, #58516, #46720, #77473, #58941, #51770, #13924, #72412, #78317, #77051, #14761, #8025, #59349, #6753, #7176, #40417, #38742, #13497, #40008, #71995, #33280, #27363, #77896, #39153, #20647, #26109, #39581, #46301, #58088, #19810, #1299, #32847, #65270, #6340, #33688, #19384, #32012, #1708, #57672, #453, #879, #34, #52192, #20227, #25687, #51348, #26948, #45036, #45875, #71573, #52611, #2540, #16007, #80403, #47131, #48373, #28616, #29026, #9678, #72822, #8846, #28198, #54693, #15172, #41654, #22715, #35760, #74073, #40828, #53857, #61011, #16419, #61427, #8434, #42065, #66098, #34522, #79156, #9268, #15590, #41248, #67760, #3776, #22303, #47964, #10095, #73666, #66514, #66935, #29440, #79990, #35349, #2951, #23123, #34104, #55099, #80807, #48791, #79569, #53448, #67345, #60189, #74489, #16836, #59765, #2119, #21885, #3362, #27785, #21473, #47549, #73240, #34939, #60602, #54274, #76133, #76545, #4183, #61842, #81217, #49615, #44117, #17252, #36992, #82856, #4588, #62672, #81637, #17655, #43697, #5012, #30682, #18064, #36168, #11754, #82448, #63490, #23947, #12158, #5824, #25176, #69809, #37410, #24357, #36573, #29845, #55509, #75309, #55923, #50845, #31496, #42471, #75724, #11332, #23533, #56343, #57156, #82044, #63082, #49202, #37814, #50026, #68173, #69402, #5420, #10515, #68574, #74903, #42880, #10916, #62251, #31082, #56749, #18474, #30259, #24764, #43287, #68984, #50432, #19704, #33588, #20550, #77372, #51669, #76954, #18873, #354, #1201, #38642, #25589, #13824, #14248, #58843, #52088, #775, #32328, #19282, #13402, #57989, #77798, #26437, #32749, #64320, #45362, #6237, #59253, #26011, #39483, #71058, #44522, #20130, #52926, #52510, #58416, #39056, #12566, #64740, #33175, #7078, #1610, #46202, #44933, #27266, #45778, #65170, #70630, #70210, #51252, #6654, #26851, #78218, #65594, #63900, #71476, #7506, #83266, #71897, #39906, #12987, #38224, #7927, #57574, #31913, #2021, #60912, #46622, #8339, #14664, #66836, #47032, #3263, #60090, #53351, #34005, #9170, #54172, #79060, #15072, #21378, #67658, #48276, #66000, #40730, #35660, #53757, #22616, #41964, #72726, #79886, #66414, #40321, #27686, #41558, #28102, #73565, #34841, #59667, #79468, #78640, #15909, #72317, #9995, #20963, #29342, #73974, #61323, #8750, #34423, #16320, #73141, #67247, #2444, #3678, #15490, #21785, #60503, #2852, #47446, #41147, #28515, #22204, #47860, #9578, #35248, #28924, #54592, #80302, #75212, #18379, #55413, #4495, #55824, #69713, #56650, #30162, #81532, #29750, #55003, #36479, #37311, #74805, #61745, #49929, #50337, #11653, #4910, #36895, #68480, #81120, #49519, #10818, #30581, #62571, #68885, #17152, #23852, #42373, #12057, #62154, #75627, #17556, #80710, #56247, #5723, #5324, #11235, #43189, #48691, #81943, #69304, #24256, #37714, #82350, #23436, #63388, #17965, #43602, #49101, #23025, #4082, #42785, #62985, #30982, #44020, #16732, #24669, #76034, #36074, #74388, #68071, #10416, #14145, #65060, #70112, #64222, #38125, #13721, #82751, #44417, #50747, #19597, #83166, #39375, #12882, #6137, #12463, #45260, #6974, #31812, #51152, #57472, #20446, #1098, #18774, #76846, #71792, #6556, #58736, #78113, #25486, #32643, #19180, #76446, #63799, #77694, #32228, #26327, #70956, #44829, #57886, #31394, #51989, #25073, #13301, #70526, #253, #26749, #38953, #673, #51565, #39797, #57059, #46099, #65492, #38542, #25904, #77268, #64637, #58307, #7397, #20024, #52404, #45675, #71371, #33066, #2343, #9477, #40218, #60403, #15386, #8236, #52826, #2753, #35151, #27164, #1510, #20863, #78957, #54073, #14566, #66312, #41463, #59566, #8651, #53242, #46931, #21685, #34322, #40630, #79366, #59153, #47348, #9072, #47764, #21275, #79788, #73462, #67148, #22104, #73037, #27999, #33902, #78538, #46513, #72623 ),
 ( #65900, #72214, #7824, #33491, #14971, #15814, #1922, #27585, #41048, #59984, #53658, #66733, #34743, #28413, #14432, #1377, #58169, #32506, #57751, #83029, #64498, #65353, #19465, #6421, #77977, #78397, #39663, #32931, #64921, #13170, #113, #77559, #38820, #58596, #7259, #13582, #45115, #538, #70390, #40084, #6836, #20307, #26191, #25352, #965, #33769, #33358, #39236, #51852, #76713, #19893, #14006, #45540, #51014, #20729, #71238, #45957, #38404, #52689, #26619, #46380, #52273, #71654, #72073, #25768, #32090, #19046, #44693, #12745, #7691, #59021, #27028, #64084, #65771, #8103, #51429, #77132, #70823, #74153, #61092, #34606, #8929, #34184, #59430, #40913, #41728, #79236, #66180, #54357, #54777, #16083, #9345, #41332, #72902, #59848, #53939, #15254, #35016, #67012, #73324, #21551, #60271, #46799, #16500, #66594, #80069, #2621, #1785, #60680, #10178, #9755, #15670, #28277, #53106, #79651, #73747, #21968, #42144, #3443, #2200, #67839, #3029, #22386, #27868, #27445, #8517, #47212, #67422, #35427, #22793, #21144, #47630, #28695, #40499, #29107, #48046, #53528, #78815, #80480, #14839, #48453, #72490, #61341, #61761, #11253, #55840, #56263, #67263, #41573, #60929, #29359, #23867, #80318, #16750, #62587, #67675, #42389, #3694, #80727, #23452, #68088, #10433, #81136, #15926, #74823, #62170, #43205, #55018, #75228, #68900, #4929, #49534, #17167, #4099, #16338, #9596, #35264, #23041, #35676, #30597, #3279, #22220, #81549, #17572, #22633, #48708, #36911, #28943, #74406, #30178, #4509, #49117, #47876, #36090, #29767, #10835, #41981, #55428, #36494, #54609, #73580, #42801, #68495, #48294, #73991, #10011, #44037, #44848, #63001, #31830, #70546, #51584, #6575, #30999, #69729, #76867, #64240, #77286, #24274, #32246, #81959, #50353, #11671, #25093, #31412, #57076, #271, #19617, #38145, #63817, #12901, #6156, #82367, #82770, #45279, #12481, #51171, #18792, #38972, #49945, #70974, #13319, #64655, #12074, #69320, #57491, #5340, #57906, #6993, #32661, #75643, #76051, #83183, #25505, #17982, #24686, #50765, #37732, #19199, #43619, #25926, #37328, #56667, #18395, #63405, #5741, #76466, #44437, #70130, #38560, #20465, #78556, #14163, #33507, #59584, #20881, #52845, #33919, #52007, #27603, #14990, #79384, #39819, #28016, #21703, #15407, #60005, #53263, #40235, #52422, #20042, #45693, #65508, #71812, #66756, #47366, #9090, #8255, #27181, #39395, #46533, #73057, #46118, #78974, #7840, #65918, #41067, #46948, #66331, #58328, #71390, #59169, #1527, #65079, #8669, #21295, #7417, #690, #34340, #13739, #72233, #2360, #53676, #77712, #14582, #33087, #1941, #26767, #26346, #72640, #58754, #1116, #40647, #78132, #35170, #54509, #9497, #23773, #4417, #22123, #80223, #75138, #9910, #62079, #81456, #60831, #35999, #3183, #79807, #67167, #81045, #67578, #29674, #48614, #47782, #35582, #34762, #55336, #2773, #49444, #60422, #68811, #30086, #29264, #23358, #73484, #55748, #54928, #17483, #74308, #16655, #43114, #28847, #41482, #28433, #54092, #15834, #67992, #49029, #10747, #22539, #80635, #48202, #73897, #61245, #3599, #16237, #36404, #22946, #42295, #41885, #10337, #61669, #17074, #4010, #74725, #42711, #68407, #51073, #44344, #76369, #24593, #69224, #5650, #50261, #70035, #18702, #24995, #56574, #69635, #81869, #25826, #75959, #6062, #18296, #36815, #12389, #45173, #44752, #50669, #43941, #4825, #11981, #25410, #37635, #77188, #12806, #11572, #51485, #38046, #31733, #37231, #62491, #17889, #82275, #76772, #62909, #30504, #43526, #63311, #19104, #70448, #57806, #56166, #31316, #56981, #75550, #38460, #57398, #5243, #19520, #64146, #49850, #82678, #6480, #32149, #24181, #63722, #30907, #83088, #172, #11157, #52327, #45598, #26249, #59073, #46435, #71292, #7315, #13639, #59901, #40551, #58226, #32984, #27919 ),
 ( #20363, #70879, #8156, #38878, #34240, #13228, #21605, #66232, #65408, #33821, #51908, #8570, #7746, #2254, #27084, #1428, #53578, #39293, #77615, #64556, #6894, #32564, #20780, #59487, #46849, #19948, #33411, #79287, #64979, #46014, #71709, #593, #72544, #14063, #39717, #58652, #1019, #78033, #53158, #26672, #52747, #65823, #78454, #27501, #72126, #14484, #40138, #1841, #78870, #21195, #14891, #54832, #61145, #9396, #22441, #34661, #61979, #60733, #42199, #3085, #72955, #22848, #81355, #80942, #3497, #54411, #40969, #80122, #61569, #73799, #29981, #48927, #47682, #4316, #29163, #67895, #28332, #67475, #10648, #73377, #48100, #16136, #55644, #74627, #41782, #9809, #22022, #47265, #28749, #29573, #67064, #53994, #10233, #42611, #3912, #80537, #48509, #35481, #15727, #74209, #16555, #35900, #55235, #23257, #35067, #16971, #60324, #15306, #68311, #36303, #66651, #8987, #2673, #79706, #41382, #37537, #30809, #17385, #56474, #37948, #50160, #6379, #25311, #24080, #38364, #5553, #18604, #49750, #49339, #30395, #69120, #5962, #31632, #70350, #68710, #11469, #82177, #4721, #57292, #44247, #56061, #32051, #82990, #62384, #24493, #50975, #76673, #43016, #11885, #11051, #63213, #75450, #19005, #5144, #81770, #17788, #31217, #82578, #43423, #37126, #62810, #12705, #44654, #36709, #75856, #64040, #18198, #57711, #23667, #43833, #24897, #69535, #56885, #50566, #69936, #76270, #12292, #63625, #75039, #32889, #74, #20690, #51387, #46761, #25727, #34146, #78778, #77937, #46341, #38781, #53067, #20267, #21103, #39624, #13967, #72454, #26150, #6795, #77092, #19424, #45076, #33322, #72035, #59391, #1339, #45917, #71615, #58984, #70779, #52653, #40049, #14803, #39196, #40461, #66139, #8477, #1749, #78359, #65313, #77516, #13130, #64458, #7218, #13540, #32466, #58128, #495, #26990, #52234, #51811, #7652, #19851, #71197, #14391, #45500, #65735, #64879, #8068, #58558, #924, #27406, #26581, #33730, #34977, #48829, #40873, #66974, #67801, #42104, #3404, #15213, #74113, #29478, #9307, #34565, #59807, #41289, #10138, #79612, #66555, #54738, #55137, #16459, #9718, #41691, #73284, #60230, #54316, #15632, #35389, #67384, #73705, #21929, #60641, #47173, #74530, #2991, #80443, #28657, #2162, #61054, #10552, #35802, #16045, #80027, #53488, #22346, #61469, #48006, #42513, #3817, #2580, #16876, #29067, #22753, #28239, #27828, #8888, #47590, #80848, #23160, #68216, #21514, #48413, #79198, #53899, #72864, #57920, #42918, #20055, #70988, #74945, #70143, #13332, #7007, #29884, #25519, #55547, #51184, #4626, #45292, #18806, #10953, #17290, #76882, #12916, #36610, #55963, #62289, #26360, #32675, #23571, #51598, #68613, #19631, #83197, #284, #64254, #30297, #81676, #23987, #25939, #49654, #70560, #77300, #58341, #38985, #76479, #44451, #32259, #64668, #703, #61879, #52020, #36210, #12495, #49242, #63831, #38158, #6169, #77726, #45708, #19213, #44861, #71404, #38573, #31844, #57506, #4220, #6588, #81256, #33932, #54104, #13752, #60434, #2785, #79820, #27194, #1129, #21307, #78145, #79396, #28445, #66769, #47794, #7853, #27614, #78987, #22136, #14175, #72245, #52858, #53277, #39409, #47379, #65092, #58766, #33100, #52435, #20894, #15419, #71825, #8267, #7430, #59182, #59597, #78568, #14594, #15002, #1952, #46960, #72652, #26779, #66344, #53688, #34775, #46547, #9102, #20477, #46131, #41080, #8682, #40659, #33519, #39833, #65522, #40247, #65930, #1539, #34352, #60018, #2373, #28030, #21715, #73070, #4841, #61257, #42721, #35594, #81055, #36830, #62090, #60844, #56178, #49456, #43126, #48215, #48626, #62503, #54522, #80647, #81467, #55761, #17084, #23785, #24193, #74736, #68417, #9923, #23371, #68824, #29686, #4022, #11169, #16251, #80237, #73498, #15846, #35183, #49039, #10757, #75150, #22553, #10350, #30516 ),
 ( #36417, #73911, #41898, #3611, #4432, #67592, #30098, #17495, #81881, #41495, #29277, #54941, #67181, #9510, #3196, #28860, #22960, #74321, #16668, #42307, #68005, #36011, #61681, #55349, #70891, #6073, #31747, #12818, #57409, #50273, #50682, #19531, #63734, #19115, #70046, #6906, #49862, #13241, #38890, #32578, #63323, #37246, #83102, #30919, #32162, #64569, #45188, #606, #43952, #25421, #51086, #58240, #75970, #25009, #5661, #76783, #75562, #185, #17902, #11586, #69238, #5255, #56993, #51497, #24604, #44355, #43539, #11992, #12400, #31328, #76380, #44764, #38057, #70461, #38475, #62922, #64159, #6492, #56585, #82690, #82286, #18311, #69648, #77202, #57818, #25838, #37646, #18714, #13652, #33425, #39730, #34675, #72968, #60338, #59500, #78468, #7328, #20793, #40984, #27515, #53171, #46028, #1853, #40563, #32996, #8582, #72142, #72556, #78886, #58666, #52340, #71722, #14903, #1031, #21207, #66244, #79300, #34254, #26685, #14078, #46862, #59915, #21618, #51923, #2270, #26262, #78047, #39305, #52760, #59086, #1441, #27933, #47278, #65835, #8168, #53591, #33833, #20376, #27098, #15319, #40151, #66664, #46449, #9003, #77628, #19960, #45611, #71305, #65426, #64992, #7759, #14498, #68324, #49355, #55658, #36723, #80135, #16568, #67909, #11065, #3098, #61159, #41797, #42213, #75052, #36317, #2686, #47696, #22036, #41396, #9824, #4329, #60746, #80550, #43029, #48115, #22862, #67488, #3510, #3927, #48523, #74223, #61582, #79719, #55249, #42627, #23681, #35494, #81368, #17399, #68724, #29995, #80956, #10245, #22456, #73391, #15742, #29179, #16150, #28346, #54007, #67078, #35916, #54846, #9410, #29586, #35080, #73813, #23271, #48940, #74642, #28762, #16984, #54425, #10662, #61992, #32065, #37140, #37553, #51405, #43437, #69551, #70364, #44669, #5977, #12719, #13146, #31648, #38379, #62399, #63639, #57306, #82191, #12306, #76687, #69134, #64055, #24912, #25325, #83004, #11486, #5160, #24508, #50989, #62825, #37963, #19021, #57726, #6395, #30824, #50175, #89, #25742, #77107, #4738, #19439, #30411, #56489, #75464, #5567, #11899, #63227, #45090, #70794, #18618, #44261, #56079, #69952, #75870, #31232, #81784, #76287, #24095, #82593, #49764, #17803, #18213, #43848, #56899, #50580, #26166, #46357, #19867, #21118, #2177, #8494, #72880, #32906, #52667, #20705, #47188, #39211, #13982, #77953, #78374, #27844, #72469, #38797, #513, #58144, #77532, #45931, #40477, #13555, #33337, #79213, #938, #58998, #20282, #39638, #40062, #1354, #27005, #14408, #32481, #8082, #78794, #59822, #71630, #34161, #53505, #21529, #66155, #33745, #72051, #58573, #51827, #45516, #65329, #52248, #64473, #6810, #71212, #65749, #7666, #64896, #59406, #7233, #26596, #1763, #27420, #53081, #46778, #14818, #2596, #81272, #74548, #68234, #73299, #73722, #4236, #79628, #22363, #23177, #80865, #28254, #34992, #55564, #16061, #42532, #61895, #41304, #16476, #15648, #60248, #47605, #61487, #48022, #10155, #29084, #53915, #41708, #15229, #35821, #66570, #29900, #40888, #49259, #10569, #9735, #3835, #21946, #36226, #35406, #23588, #54754, #80460, #8904, #66990, #9322, #34580, #60657, #3006, #48432, #29495, #16893, #28673, #61070, #54334, #80044, #67400, #74131, #3421, #55154, #22769, #42123, #67818, #48847, #56397, #57208, #11388, #81692, #69860, #70266, #31551, #24816, #56801, #5065, #49671, #69455, #30734, #50483, #82500, #5472, #37045, #50079, #62305, #6293, #82095, #12211, #24409, #17307, #76187, #25643, #25230, #31134, #75775, #68629, #18116, #5878, #43749, #57629, #76595, #75361, #31968, #18524, #37869, #17709, #42935, #24003, #62727, #82909, #50895, #38280, #36628, #11805, #37460, #55981, #18925, #63544, #43337, #42331, #44574, #30313, #63133, #12621, #63956, #10969, #44167, #4642, #74961, #69038, #59306, #32804, #26066 ) ),
 .UNSPECIFIED., .F., .F., .F. ) 
 B_SPLINE_SURFACE_WITH_KNOTS ( ( 4, 4 ),
 ( 3, 2, 2, 2, 2, 2, 2, 2, 2, 2, 2, 2, 2, 2, 2, 2, 2, 2, 2, 2, 2, 2, 2, 2, 2, 2, 2, 2, 2, 2, 2, 2, 2, 2, 2, 2, 2, 2, 2, 2, 2, 2, 2, 2, 2, 2, 2, 2, 2, 2, 2, 2, 2, 2, 2, 2, 2, 2, 2, 2, 2, 2, 2, 2, 2, 2, 2, 2, 2, 2, 2, 2, 2, 2, 2, 2, 2, 2, 2, 2, 2, 2, 2, 2, 2, 2, 2, 2, 2, 2, 2, 2, 2, 2, 2, 2, 2, 2, 2, 2, 2, 2, 2, 2, 2, 2, 2, 2, 2, 2, 2, 2, 2, 2, 2, 2, 2, 2, 2, 2, 2, 2, 2, 2, 2, 2, 2, 2, 2, 2, 2, 2, 2, 2, 2, 2, 2, 2, 2, 2, 2, 2, 2, 2, 2, 2, 2, 2, 2, 2, 2, 2, 2, 2, 2, 2, 2, 2, 2, 2, 2, 2, 2, 2, 2, 2, 2, 2, 2, 2, 2, 2, 2, 2, 2, 2, 2, 2, 2, 2, 2, 2, 2, 2, 2, 2, 2, 2, 2, 2, 2, 2, 2, 2, 2, 2, 2, 2, 2, 2, 2, 2, 2, 2, 2, 2, 2, 2, 2, 2, 2, 2, 2, 2, 2, 2, 2, 2, 2, 2, 2, 2, 2, 2, 2, 2, 2, 2, 2, 2, 2, 2, 2, 2, 2, 2, 2, 3 ),
 ( 0.000000000000000000, 1.000000000000000000 ),
 ( 0.000000000000000000, 0.004166666666666666609, 0.008333333333333333218, 0.01250000000000000069, 0.01666666666666666644, 0.02083333333333333218, 0.02500000000000000139, 0.02916666666666666713, 0.03333333333333333287, 0.03749999999999999861, 0.04166666666666666435, 0.04583333333333333010, 0.05000000000000000278, 0.05416666666666666852, 0.05833333333333333426, 0.06250000000000000000, 0.06666666666666666574, 0.07083333333333333148, 0.07499999999999999722, 0.07916666666666666297, 0.08333333333333332871, 0.08749999999999999445, 0.09166666666666666019, 0.09583333333333333981, 0.1000000000000000056, 0.1041666666666666713, 0.1083333333333333370, 0.1125000000000000028, 0.1166666666666666685, 0.1208333333333333343, 0.1250000000000000000, 0.1291666666666666796, 0.1333333333333333315, 0.1375000000000000111, 0.1416666666666666630, 0.1458333333333333426, 0.1499999999999999944, 0.1541666666666666741, 0.1583333333333333259, 0.1625000000000000056, 0.1666666666666666574, 0.1708333333333333370, 0.1749999999999999889, 0.1791666666666666685, 0.1833333333333333204, 0.1875000000000000000, 0.1916666666666666796, 0.1958333333333333315, 0.2000000000000000111, 0.2041666666666666630, 0.2083333333333333426, 0.2124999999999999944, 0.2166666666666666741, 0.2208333333333333259, 0.2250000000000000056, 0.2291666666666666574, 0.2333333333333333370, 0.2374999999999999889, 0.2416666666666666685, 0.2458333333333333204, 0.2500000000000000000, 0.2541666666666666519, 0.2583333333333333592, 0.2625000000000000111, 0.2666666666666666630, 0.2708333333333333148, 0.2750000000000000222, 0.2791666666666666741, 0.2833333333333333259, 0.2874999999999999778, 0.2916666666666666852, 0.2958333333333333370, 0.2999999999999999889, 0.3041666666666666408, 0.3083333333333333481, 0.3125000000000000000, 0.3166666666666666519, 0.3208333333333333592, 0.3250000000000000111, 0.3291666666666666630, 0.3333333333333333148, 0.3375000000000000222, 0.3416666666666666741, 0.3458333333333333259, 0.3499999999999999778, 0.3541666666666666852, 0.3583333333333333370, 0.3624999999999999889, 0.3666666666666666408, 0.3708333333333333481, 0.3750000000000000000, 0.3791666666666666519, 0.3833333333333333592, 0.3875000000000000111, 0.3916666666666666630, 0.3958333333333333148, 0.4000000000000000222, 0.4041666666666666741, 0.4083333333333333259, 0.4124999999999999778, 0.4166666666666666852, 0.4208333333333333370, 0.4249999999999999889, 0.4291666666666666408, 0.4333333333333333481, 0.4375000000000000000, 0.4416666666666666519, 0.4458333333333333592, 0.4500000000000000111, 0.4541666666666666630, 0.4583333333333333148, 0.4625000000000000222, 0.4666666666666666741, 0.4708333333333333259, 0.4749999999999999778, 0.4791666666666666852, 0.4833333333333333370, 0.4874999999999999889, 0.4916666666666666408, 0.4958333333333333481, 0.5000000000000000000, 0.5041666666666666519, 0.5083333333333333037, 0.5124999999999999556, 0.5166666666666667185, 0.5208333333333333703, 0.5250000000000000222, 0.5291666666666666741, 0.5333333333333333259, 0.5374999999999999778, 0.5416666666666666297, 0.5458333333333332815, 0.5500000000000000444, 0.5541666666666666963, 0.5583333333333333481, 0.5625000000000000000, 0.5666666666666666519, 0.5708333333333333037, 0.5749999999999999556, 0.5791666666666667185, 0.5833333333333333703, 0.5875000000000000222, 0.5916666666666666741, 0.5958333333333333259, 0.5999999999999999778, 0.6041666666666666297, 0.6083333333333332815, 0.6125000000000000444, 0.6166666666666666963, 0.6208333333333333481, 0.6250000000000000000, 0.6291666666666666519, 0.6333333333333333037, 0.6374999999999999556, 0.6416666666666667185, 0.6458333333333333703, 0.6500000000000000222, 0.6541666666666666741, 0.6583333333333333259, 0.6624999999999999778, 0.6666666666666666297, 0.6708333333333332815, 0.6750000000000000444, 0.6791666666666666963, 0.6833333333333333481, 0.6875000000000000000, 0.6916666666666666519, 0.6958333333333333037, 0.6999999999999999556, 0.7041666666666667185, 0.7083333333333333703, 0.7125000000000000222, 0.7166666666666666741, 0.7208333333333333259, 0.7249999999999999778, 0.7291666666666666297, 0.7333333333333332815, 0.7375000000000000444, 0.7416666666666666963, 0.7458333333333333481, 0.7500000000000000000, 0.7541666666666666519, 0.7583333333333333037, 0.7624999999999999556, 0.7666666666666667185, 0.7708333333333333703, 0.7750000000000000222, 0.7791666666666666741, 0.7833333333333333259, 0.7874999999999999778, 0.7916666666666666297, 0.7958333333333332815, 0.8000000000000000444, 0.8041666666666666963, 0.8083333333333333481, 0.8125000000000000000, 0.8166666666666666519, 0.8208333333333333037, 0.8249999999999999556, 0.8291666666666667185, 0.8333333333333333703, 0.8375000000000000222, 0.8416666666666666741, 0.8458333333333333259, 0.8499999999999999778, 0.8541666666666666297, 0.8583333333333332815, 0.8625000000000000444, 0.8666666666666666963, 0.8708333333333333481, 0.8750000000000000000, 0.8791666666666666519, 0.8833333333333333037, 0.8874999999999999556, 0.8916666666666667185, 0.8958333333333333703, 0.9000000000000000222, 0.9041666666666666741, 0.9083333333333333259, 0.9124999999999999778, 0.9166666666666666297, 0.9208333333333332815, 0.9250000000000000444, 0.9291666666666666963, 0.9333333333333333481, 0.9375000000000000000, 0.9416666666666666519, 0.9458333333333333037, 0.9499999999999999556, 0.9541666666666667185, 0.9583333333333333703, 0.9625000000000000222, 0.9666666666666666741, 0.9708333333333333259, 0.9749999999999999778, 0.9791666666666666297, 0.9833333333333332815, 0.9875000000000000444 ),
 .UNSPECIFIED. ) 
 GEOMETRIC_REPRESENTATION_ITEM ( )  RATIONAL_B_SPLINE_SURFACE ( (
 ( 1.000000000000000000, 0.9659258262890683122, 1.000000000000000000, 0.9659258262890683122, 1.000000000000000000, 0.9659258262890683122, 1.000000000000000000, 0.9659258262890683122, 1.000000000000000000, 0.9659258262890683122, 1.000000000000000000, 0.9659258262890683122, 1.000000000000000000, 0.9659258262890683122, 1.000000000000000000, 0.9659258262890683122, 1.000000000000000000, 0.9659258262890683122, 1.000000000000000000, 0.9659258262890683122, 1.000000000000000000, 0.9659258262890683122, 1.000000000000000000, 0.9659258262890683122, 1.000000000000000000, 0.9659258262890683122, 1.000000000000000000, 0.9659258262890683122, 1.000000000000000000, 0.9659258262890683122, 1.000000000000000000, 0.9659258262890683122, 1.000000000000000000, 0.9659258262890683122, 1.000000000000000000, 0.9659258262890683122, 1.000000000000000000, 0.9659258262890683122, 1.000000000000000000, 0.9659258262890683122, 1.000000000000000000, 0.9659258262890683122, 1.000000000000000000, 0.9659258262890683122, 1.000000000000000000, 0.9659258262890683122, 1.000000000000000000, 0.9659258262890683122, 1.000000000000000000, 0.9659258262890683122, 1.000000000000000000, 0.9659258262890683122, 1.000000000000000000, 0.9659258262890683122, 1.000000000000000000, 0.9659258262890683122, 1.000000000000000000, 0.9659258262890683122, 1.000000000000000000, 0.9659258262890683122, 1.000000000000000000, 0.9659258262890683122, 1.000000000000000000, 0.9659258262890683122, 1.000000000000000000, 0.9659258262890683122, 1.000000000000000000, 0.9659258262890683122, 1.000000000000000000, 0.9659258262890683122, 1.000000000000000000, 0.9659258262890683122, 1.000000000000000000, 0.9659258262890683122, 1.000000000000000000, 0.9659258262890683122, 1.000000000000000000, 0.9659258262890683122, 1.000000000000000000, 0.9659258262890683122, 1.000000000000000000, 0.9659258262890683122, 1.000000000000000000, 0.9659258262890683122, 1.000000000000000000, 0.9659258262890683122, 1.000000000000000000, 0.9659258262890683122, 1.000000000000000000, 0.9659258262890683122, 1.000000000000000000, 0.9659258262890683122, 1.000000000000000000, 0.9659258262890683122, 1.000000000000000000, 0.9659258262890683122, 1.000000000000000000, 0.9659258262890683122, 1.000000000000000000, 0.9659258262890683122, 1.000000000000000000, 0.9659258262890683122, 1.000000000000000000, 0.9659258262890683122, 1.000000000000000000, 0.9659258262890683122, 1.000000000000000000, 0.9659258262890683122, 1.000000000000000000, 0.9659258262890683122, 1.000000000000000000, 0.9659258262890683122, 1.000000000000000000, 0.9659258262890683122, 1.000000000000000000, 0.9659258262890683122, 1.000000000000000000, 0.9659258262890683122, 1.000000000000000000, 0.9659258262890683122, 1.000000000000000000, 0.9659258262890683122, 1.000000000000000000, 0.9659258262890683122, 1.000000000000000000, 0.9659258262890683122, 1.000000000000000000, 0.9659258262890683122, 1.000000000000000000, 0.9659258262890683122, 1.000000000000000000, 0.9659258262890683122, 1.000000000000000000, 0.9659258262890683122, 1.000000000000000000, 0.9659258262890683122, 1.000000000000000000, 0.9659258262890683122, 1.000000000000000000, 0.9659258262890683122, 1.000000000000000000, 0.9659258262890683122, 1.000000000000000000, 0.9659258262890683122, 1.000000000000000000, 0.9659258262890683122, 1.000000000000000000, 0.9659258262890683122, 1.000000000000000000, 0.9659258262890683122, 1.000000000000000000, 0.9659258262890683122, 1.000000000000000000, 0.9659258262890683122, 1.000000000000000000, 0.9659258262890683122, 1.000000000000000000, 0.9659258262890683122, 1.000000000000000000, 0.9659258262890683122, 1.000000000000000000, 0.9659258262890683122, 1.000000000000000000, 0.9659258262890683122, 1.000000000000000000, 0.9659258262890683122, 1.000000000000000000, 0.9659258262890683122, 1.000000000000000000, 0.9659258262890683122, 1.000000000000000000, 0.9659258262890683122, 1.000000000000000000, 0.9659258262890683122, 1.000000000000000000, 0.9659258262890683122, 1.000000000000000000, 0.9659258262890683122, 1.000000000000000000, 0.9659258262890683122, 1.000000000000000000, 0.9659258262890683122, 1.000000000000000000, 0.9659258262890683122, 1.000000000000000000, 0.9659258262890683122, 1.000000000000000000, 0.9659258262890683122, 1.000000000000000000, 0.9659258262890683122, 1.000000000000000000, 0.9659258262890683122, 1.000000000000000000, 0.9659258262890683122, 1.000000000000000000, 0.9659258262890683122, 1.000000000000000000, 0.9659258262890683122, 1.000000000000000000, 0.9659258262890683122, 1.000000000000000000, 0.9659258262890683122, 1.000000000000000000, 0.9659258262890683122, 1.000000000000000000, 0.9659258262890683122, 1.000000000000000000, 0.9659258262890683122, 1.000000000000000000, 0.9659258262890683122, 1.000000000000000000, 0.9659258262890683122, 1.000000000000000000, 0.9659258262890683122, 1.000000000000000000, 0.9659258262890683122, 1.000000000000000000, 0.9659258262890683122, 1.000000000000000000, 0.9659258262890683122, 1.000000000000000000, 0.9659258262890683122, 1.000000000000000000, 0.9659258262890683122, 1.000000000000000000, 0.9659258262890683122, 1.000000000000000000, 0.9659258262890683122, 1.000000000000000000, 0.9659258262890683122, 1.000000000000000000, 0.9659258262890683122, 1.000000000000000000, 0.9659258262890683122, 1.000000000000000000, 0.9659258262890683122, 1.000000000000000000, 0.9659258262890683122, 1.000000000000000000, 0.9659258262890683122, 1.000000000000000000, 0.9659258262890683122, 1.000000000000000000, 0.9659258262890683122, 1.000000000000000000, 0.9659258262890683122, 1.000000000000000000, 0.9659258262890683122, 1.000000000000000000, 0.9659258262890683122, 1.000000000000000000, 0.9659258262890683122, 1.000000000000000000, 0.9659258262890683122, 1.000000000000000000, 0.9659258262890683122, 1.000000000000000000, 0.9659258262890683122, 1.000000000000000000, 0.9659258262890683122, 1.000000000000000000, 0.9659258262890683122, 1.000000000000000000, 0.9659258262890683122, 1.000000000000000000, 0.9659258262890683122, 1.000000000000000000, 0.9659258262890683122, 1.000000000000000000, 0.9659258262890683122, 1.000000000000000000, 0.9659258262890683122, 1.000000000000000000, 0.9659258262890683122, 1.000000000000000000, 0.9659258262890683122, 1.000000000000000000, 0.9659258262890683122, 1.000000000000000000, 0.9659258262890683122, 1.000000000000000000, 0.9659258262890683122, 1.000000000000000000, 0.9659258262890683122, 1.000000000000000000, 0.9659258262890683122, 1.000000000000000000, 0.9659258262890683122, 1.000000000000000000, 0.9659258262890683122, 1.000000000000000000, 0.9659258262890683122, 1.000000000000000000, 0.9659258262890683122, 1.000000000000000000, 0.9659258262890683122, 1.000000000000000000, 0.9659258262890683122, 1.000000000000000000, 0.9659258262890683122, 1.000000000000000000, 0.9659258262890683122, 1.000000000000000000, 0.9659258262890683122, 1.000000000000000000, 0.9659258262890683122, 1.000000000000000000, 0.9659258262890683122, 1.000000000000000000, 0.9659258262890683122, 1.000000000000000000, 0.9659258262890683122, 1.000000000000000000, 0.9659258262890683122, 1.000000000000000000, 0.9659258262890683122, 1.000000000000000000, 0.9659258262890683122, 1.000000000000000000, 0.9659258262890683122, 1.000000000000000000, 0.9659258262890683122, 1.000000000000000000, 0.9659258262890683122, 1.000000000000000000, 0.9659258262890683122, 1.000000000000000000, 0.9659258262890683122, 1.000000000000000000, 0.9659258262890683122, 1.000000000000000000, 0.9659258262890683122, 1.000000000000000000, 0.9659258262890683122, 1.000000000000000000, 0.9659258262890683122, 1.000000000000000000, 0.9659258262890683122, 1.000000000000000000, 0.9659258262890683122, 1.000000000000000000, 0.9659258262890683122, 1.000000000000000000, 0.9659258262890683122, 1.000000000000000000, 0.9659258262890683122, 1.000000000000000000, 0.9659258262890683122, 1.000000000000000000, 0.9659258262890683122, 1.000000000000000000, 0.9659258262890683122, 1.000000000000000000, 0.9659258262890683122, 1.000000000000000000, 0.9659258262890683122, 1.000000000000000000, 0.9659258262890683122, 1.000000000000000000, 0.9659258262890683122, 1.000000000000000000, 0.9659258262890683122, 1.000000000000000000, 0.9659258262890683122, 1.000000000000000000, 0.9659258262890683122, 1.000000000000000000, 0.9659258262890683122, 1.000000000000000000, 0.9659258262890683122, 1.000000000000000000, 0.9659258262890683122, 1.000000000000000000, 0.9659258262890683122, 1.000000000000000000, 0.9659258262890683122, 1.000000000000000000, 0.9659258262890683122, 1.000000000000000000, 0.9659258262890683122, 1.000000000000000000, 0.9659258262890683122, 1.000000000000000000, 0.9659258262890683122, 1.000000000000000000, 0.9659258262890683122, 1.000000000000000000, 0.9659258262890683122, 1.000000000000000000, 0.9659258262890683122, 1.000000000000000000, 0.9659258262890683122, 1.000000000000000000, 0.9659258262890683122, 1.000000000000000000, 0.9659258262890683122, 1.000000000000000000, 0.9659258262890683122, 1.000000000000000000, 0.9659258262890683122, 1.000000000000000000, 0.9659258262890683122, 1.000000000000000000, 0.9659258262890683122, 1.000000000000000000, 0.9659258262890683122, 1.000000000000000000, 0.9659258262890683122, 1.000000000000000000, 0.9659258262890683122, 1.000000000000000000, 0.9659258262890683122, 1.000000000000000000, 0.9659258262890683122, 1.000000000000000000, 0.9659258262890683122, 1.000000000000000000, 0.9659258262890683122, 1.000000000000000000, 0.9659258262890683122, 1.000000000000000000, 0.9659258262890683122, 1.000000000000000000, 0.9659258262890683122, 1.000000000000000000, 0.9659258262890683122, 1.000000000000000000, 0.9659258262890683122, 1.000000000000000000, 0.9659258262890683122, 1.000000000000000000, 0.9659258262890683122, 1.000000000000000000, 0.9659258262890683122, 1.000000000000000000, 0.9659258262890683122, 1.000000000000000000, 0.9659258262890683122, 1.000000000000000000, 0.9659258262890683122, 1.000000000000000000, 0.9659258262890683122, 1.000000000000000000, 0.9659258262890683122, 1.000000000000000000, 0.9659258262890683122, 1.000000000000000000, 0.9659258262890683122, 1.000000000000000000, 0.9659258262890683122, 1.000000000000000000, 0.9659258262890683122, 1.000000000000000000, 0.9659258262890683122, 1.000000000000000000, 0.9659258262890683122, 1.000000000000000000, 0.9659258262890683122, 1.000000000000000000, 0.9659258262890683122, 1.000000000000000000, 0.9659258262890683122, 1.000000000000000000, 0.9659258262890683122, 1.000000000000000000, 0.9659258262890683122, 1.000000000000000000, 0.9659258262890683122, 1.000000000000000000, 0.9659258262890683122, 1.000000000000000000, 0.9659258262890683122, 1.000000000000000000, 0.9659258262890683122, 1.000000000000000000),
 ( 0.8047378541243631611, 0.7773170766911672303, 0.8047378541243631611, 0.7773170766911672303, 0.8047378541243631611, 0.7773170766911672303, 0.8047378541243631611, 0.7773170766911672303, 0.8047378541243631611, 0.7773170766911672303, 0.8047378541243631611, 0.7773170766911672303, 0.8047378541243631611, 0.7773170766911672303, 0.8047378541243631611, 0.7773170766911672303, 0.8047378541243631611, 0.7773170766911672303, 0.8047378541243631611, 0.7773170766911672303, 0.8047378541243631611, 0.7773170766911672303, 0.8047378541243631611, 0.7773170766911672303, 0.8047378541243631611, 0.7773170766911672303, 0.8047378541243631611, 0.7773170766911672303, 0.8047378541243631611, 0.7773170766911672303, 0.8047378541243631611, 0.7773170766911672303, 0.8047378541243631611, 0.7773170766911672303, 0.8047378541243631611, 0.7773170766911672303, 0.8047378541243631611, 0.7773170766911672303, 0.8047378541243631611, 0.7773170766911672303, 0.8047378541243631611, 0.7773170766911672303, 0.8047378541243631611, 0.7773170766911672303, 0.8047378541243631611, 0.7773170766911672303, 0.8047378541243631611, 0.7773170766911672303, 0.8047378541243631611, 0.7773170766911672303, 0.8047378541243631611, 0.7773170766911672303, 0.8047378541243631611, 0.7773170766911672303, 0.8047378541243631611, 0.7773170766911672303, 0.8047378541243631611, 0.7773170766911672303, 0.8047378541243631611, 0.7773170766911672303, 0.8047378541243631611, 0.7773170766911672303, 0.8047378541243631611, 0.7773170766911672303, 0.8047378541243631611, 0.7773170766911672303, 0.8047378541243631611, 0.7773170766911672303, 0.8047378541243631611, 0.7773170766911672303, 0.8047378541243631611, 0.7773170766911672303, 0.8047378541243631611, 0.7773170766911672303, 0.8047378541243631611, 0.7773170766911672303, 0.8047378541243631611, 0.7773170766911672303, 0.8047378541243631611, 0.7773170766911672303, 0.8047378541243631611, 0.7773170766911672303, 0.8047378541243631611, 0.7773170766911672303, 0.8047378541243631611, 0.7773170766911672303, 0.8047378541243631611, 0.7773170766911672303, 0.8047378541243631611, 0.7773170766911672303, 0.8047378541243631611, 0.7773170766911672303, 0.8047378541243631611, 0.7773170766911672303, 0.8047378541243631611, 0.7773170766911672303, 0.8047378541243631611, 0.7773170766911672303, 0.8047378541243631611, 0.7773170766911672303, 0.8047378541243631611, 0.7773170766911672303, 0.8047378541243631611, 0.7773170766911672303, 0.8047378541243631611, 0.7773170766911672303, 0.8047378541243631611, 0.7773170766911672303, 0.8047378541243631611, 0.7773170766911672303, 0.8047378541243631611, 0.7773170766911672303, 0.8047378541243631611, 0.7773170766911672303, 0.8047378541243631611, 0.7773170766911672303, 0.8047378541243631611, 0.7773170766911672303, 0.8047378541243631611, 0.7773170766911672303, 0.8047378541243631611, 0.7773170766911672303, 0.8047378541243631611, 0.7773170766911672303, 0.8047378541243631611, 0.7773170766911672303, 0.8047378541243631611, 0.7773170766911672303, 0.8047378541243631611, 0.7773170766911672303, 0.8047378541243631611, 0.7773170766911672303, 0.8047378541243631611, 0.7773170766911672303, 0.8047378541243631611, 0.7773170766911672303, 0.8047378541243631611, 0.7773170766911672303, 0.8047378541243631611, 0.7773170766911672303, 0.8047378541243631611, 0.7773170766911672303, 0.8047378541243631611, 0.7773170766911672303, 0.8047378541243631611, 0.7773170766911672303, 0.8047378541243631611, 0.7773170766911672303, 0.8047378541243631611, 0.7773170766911672303, 0.8047378541243631611, 0.7773170766911672303, 0.8047378541243631611, 0.7773170766911672303, 0.8047378541243631611, 0.7773170766911672303, 0.8047378541243631611, 0.7773170766911672303, 0.8047378541243631611, 0.7773170766911672303, 0.8047378541243631611, 0.7773170766911672303, 0.8047378541243631611, 0.7773170766911672303, 0.8047378541243631611, 0.7773170766911672303, 0.8047378541243631611, 0.7773170766911672303, 0.8047378541243631611, 0.7773170766911672303, 0.8047378541243631611, 0.7773170766911672303, 0.8047378541243631611, 0.7773170766911672303, 0.8047378541243631611, 0.7773170766911672303, 0.8047378541243631611, 0.7773170766911672303, 0.8047378541243631611, 0.7773170766911672303, 0.8047378541243631611, 0.7773170766911672303, 0.8047378541243631611, 0.7773170766911672303, 0.8047378541243631611, 0.7773170766911672303, 0.8047378541243631611, 0.7773170766911672303, 0.8047378541243631611, 0.7773170766911672303, 0.8047378541243631611, 0.7773170766911672303, 0.8047378541243631611, 0.7773170766911672303, 0.8047378541243631611, 0.7773170766911672303, 0.8047378541243631611, 0.7773170766911672303, 0.8047378541243631611, 0.7773170766911672303, 0.8047378541243631611, 0.7773170766911672303, 0.8047378541243631611, 0.7773170766911672303, 0.8047378541243631611, 0.7773170766911672303, 0.8047378541243631611, 0.7773170766911672303, 0.8047378541243631611, 0.7773170766911672303, 0.8047378541243631611, 0.7773170766911672303, 0.8047378541243631611, 0.7773170766911672303, 0.8047378541243631611, 0.7773170766911672303, 0.8047378541243631611, 0.7773170766911672303, 0.8047378541243631611, 0.7773170766911672303, 0.8047378541243631611, 0.7773170766911672303, 0.8047378541243631611, 0.7773170766911672303, 0.8047378541243631611, 0.7773170766911672303, 0.8047378541243631611, 0.7773170766911672303, 0.8047378541243631611, 0.7773170766911672303, 0.8047378541243631611, 0.7773170766911672303, 0.8047378541243631611, 0.7773170766911672303, 0.8047378541243631611, 0.7773170766911672303, 0.8047378541243631611, 0.7773170766911672303, 0.8047378541243631611, 0.7773170766911672303, 0.8047378541243631611, 0.7773170766911672303, 0.8047378541243631611, 0.7773170766911672303, 0.8047378541243631611, 0.7773170766911672303, 0.8047378541243631611, 0.7773170766911672303, 0.8047378541243631611, 0.7773170766911672303, 0.8047378541243631611, 0.7773170766911672303, 0.8047378541243631611, 0.7773170766911672303, 0.8047378541243631611, 0.7773170766911672303, 0.8047378541243631611, 0.7773170766911672303, 0.8047378541243631611, 0.7773170766911672303, 0.8047378541243631611, 0.7773170766911672303, 0.8047378541243631611, 0.7773170766911672303, 0.8047378541243631611, 0.7773170766911672303, 0.8047378541243631611, 0.7773170766911672303, 0.8047378541243631611, 0.7773170766911672303, 0.8047378541243631611, 0.7773170766911672303, 0.8047378541243631611, 0.7773170766911672303, 0.8047378541243631611, 0.7773170766911672303, 0.8047378541243631611, 0.7773170766911672303, 0.8047378541243631611, 0.7773170766911672303, 0.8047378541243631611, 0.7773170766911672303, 0.8047378541243631611, 0.7773170766911672303, 0.8047378541243631611, 0.7773170766911672303, 0.8047378541243631611, 0.7773170766911672303, 0.8047378541243631611, 0.7773170766911672303, 0.8047378541243631611, 0.7773170766911672303, 0.8047378541243631611, 0.7773170766911672303, 0.8047378541243631611, 0.7773170766911672303, 0.8047378541243631611, 0.7773170766911672303, 0.8047378541243631611, 0.7773170766911672303, 0.8047378541243631611, 0.7773170766911672303, 0.8047378541243631611, 0.7773170766911672303, 0.8047378541243631611, 0.7773170766911672303, 0.8047378541243631611, 0.7773170766911672303, 0.8047378541243631611, 0.7773170766911672303, 0.8047378541243631611, 0.7773170766911672303, 0.8047378541243631611, 0.7773170766911672303, 0.8047378541243631611, 0.7773170766911672303, 0.8047378541243631611, 0.7773170766911672303, 0.8047378541243631611, 0.7773170766911672303, 0.8047378541243631611, 0.7773170766911672303, 0.8047378541243631611, 0.7773170766911672303, 0.8047378541243631611, 0.7773170766911672303, 0.8047378541243631611, 0.7773170766911672303, 0.8047378541243631611, 0.7773170766911672303, 0.8047378541243631611, 0.7773170766911672303, 0.8047378541243631611, 0.7773170766911672303, 0.8047378541243631611, 0.7773170766911672303, 0.8047378541243631611, 0.7773170766911672303, 0.8047378541243631611, 0.7773170766911672303, 0.8047378541243631611, 0.7773170766911672303, 0.8047378541243631611, 0.7773170766911672303, 0.8047378541243631611, 0.7773170766911672303, 0.8047378541243631611, 0.7773170766911672303, 0.8047378541243631611, 0.7773170766911672303, 0.8047378541243631611, 0.7773170766911672303, 0.8047378541243631611, 0.7773170766911672303, 0.8047378541243631611, 0.7773170766911672303, 0.8047378541243631611, 0.7773170766911672303, 0.8047378541243631611, 0.7773170766911672303, 0.8047378541243631611, 0.7773170766911672303, 0.8047378541243631611, 0.7773170766911672303, 0.8047378541243631611, 0.7773170766911672303, 0.8047378541243631611, 0.7773170766911672303, 0.8047378541243631611, 0.7773170766911672303, 0.8047378541243631611, 0.7773170766911672303, 0.8047378541243631611, 0.7773170766911672303, 0.8047378541243631611, 0.7773170766911672303, 0.8047378541243631611, 0.7773170766911672303, 0.8047378541243631611, 0.7773170766911672303, 0.8047378541243631611, 0.7773170766911672303, 0.8047378541243631611, 0.7773170766911672303, 0.8047378541243631611, 0.7773170766911672303, 0.8047378541243631611, 0.7773170766911672303, 0.8047378541243631611, 0.7773170766911672303, 0.8047378541243631611, 0.7773170766911672303, 0.8047378541243631611, 0.7773170766911672303, 0.8047378541243631611, 0.7773170766911672303, 0.8047378541243631611, 0.7773170766911672303, 0.8047378541243631611, 0.7773170766911672303, 0.8047378541243631611, 0.7773170766911672303, 0.8047378541243631611, 0.7773170766911672303, 0.8047378541243631611, 0.7773170766911672303, 0.8047378541243631611, 0.7773170766911672303, 0.8047378541243631611, 0.7773170766911672303, 0.8047378541243631611, 0.7773170766911672303, 0.8047378541243631611, 0.7773170766911672303, 0.8047378541243631611, 0.7773170766911672303, 0.8047378541243631611, 0.7773170766911672303, 0.8047378541243631611, 0.7773170766911672303, 0.8047378541243631611, 0.7773170766911672303, 0.8047378541243631611, 0.7773170766911672303, 0.8047378541243631611, 0.7773170766911672303, 0.8047378541243631611, 0.7773170766911672303, 0.8047378541243631611, 0.7773170766911672303, 0.8047378541243631611, 0.7773170766911672303, 0.8047378541243631611, 0.7773170766911672303, 0.8047378541243631611, 0.7773170766911672303, 0.8047378541243631611, 0.7773170766911672303, 0.8047378541243631611, 0.7773170766911672303, 0.8047378541243631611, 0.7773170766911672303, 0.8047378541243631611, 0.7773170766911672303, 0.8047378541243631611, 0.7773170766911672303, 0.8047378541243631611, 0.7773170766911672303, 0.8047378541243631611, 0.7773170766911672303, 0.8047378541243631611, 0.7773170766911672303, 0.8047378541243631611, 0.7773170766911672303, 0.8047378541243631611, 0.7773170766911672303, 0.8047378541243631611, 0.7773170766911672303, 0.8047378541243631611, 0.7773170766911672303, 0.8047378541243631611, 0.7773170766911672303, 0.8047378541243631611, 0.7773170766911672303, 0.8047378541243631611, 0.7773170766911672303, 0.8047378541243631611, 0.7773170766911672303, 0.8047378541243631611, 0.7773170766911672303, 0.8047378541243631611, 0.7773170766911672303, 0.8047378541243631611, 0.7773170766911672303, 0.8047378541243631611),
 ( 0.8047378541243631611, 0.7773170766911672303, 0.8047378541243631611, 0.7773170766911672303, 0.8047378541243631611, 0.7773170766911672303, 0.8047378541243631611, 0.7773170766911672303, 0.8047378541243631611, 0.7773170766911672303, 0.8047378541243631611, 0.7773170766911672303, 0.8047378541243631611, 0.7773170766911672303, 0.8047378541243631611, 0.7773170766911672303, 0.8047378541243631611, 0.7773170766911672303, 0.8047378541243631611, 0.7773170766911672303, 0.8047378541243631611, 0.7773170766911672303, 0.8047378541243631611, 0.7773170766911672303, 0.8047378541243631611, 0.7773170766911672303, 0.8047378541243631611, 0.7773170766911672303, 0.8047378541243631611, 0.7773170766911672303, 0.8047378541243631611, 0.7773170766911672303, 0.8047378541243631611, 0.7773170766911672303, 0.8047378541243631611, 0.7773170766911672303, 0.8047378541243631611, 0.7773170766911672303, 0.8047378541243631611, 0.7773170766911672303, 0.8047378541243631611, 0.7773170766911672303, 0.8047378541243631611, 0.7773170766911672303, 0.8047378541243631611, 0.7773170766911672303, 0.8047378541243631611, 0.7773170766911672303, 0.8047378541243631611, 0.7773170766911672303, 0.8047378541243631611, 0.7773170766911672303, 0.8047378541243631611, 0.7773170766911672303, 0.8047378541243631611, 0.7773170766911672303, 0.8047378541243631611, 0.7773170766911672303, 0.8047378541243631611, 0.7773170766911672303, 0.8047378541243631611, 0.7773170766911672303, 0.8047378541243631611, 0.7773170766911672303, 0.8047378541243631611, 0.7773170766911672303, 0.8047378541243631611, 0.7773170766911672303, 0.8047378541243631611, 0.7773170766911672303, 0.8047378541243631611, 0.7773170766911672303, 0.8047378541243631611, 0.7773170766911672303, 0.8047378541243631611, 0.7773170766911672303, 0.8047378541243631611, 0.7773170766911672303, 0.8047378541243631611, 0.7773170766911672303, 0.8047378541243631611, 0.7773170766911672303, 0.8047378541243631611, 0.7773170766911672303, 0.8047378541243631611, 0.7773170766911672303, 0.8047378541243631611, 0.7773170766911672303, 0.8047378541243631611, 0.7773170766911672303, 0.8047378541243631611, 0.7773170766911672303, 0.8047378541243631611, 0.7773170766911672303, 0.8047378541243631611, 0.7773170766911672303, 0.8047378541243631611, 0.7773170766911672303, 0.8047378541243631611, 0.7773170766911672303, 0.8047378541243631611, 0.7773170766911672303, 0.8047378541243631611, 0.7773170766911672303, 0.8047378541243631611, 0.7773170766911672303, 0.8047378541243631611, 0.7773170766911672303, 0.8047378541243631611, 0.7773170766911672303, 0.8047378541243631611, 0.7773170766911672303, 0.8047378541243631611, 0.7773170766911672303, 0.8047378541243631611, 0.7773170766911672303, 0.8047378541243631611, 0.7773170766911672303, 0.8047378541243631611, 0.7773170766911672303, 0.8047378541243631611, 0.7773170766911672303, 0.8047378541243631611, 0.7773170766911672303, 0.8047378541243631611, 0.7773170766911672303, 0.8047378541243631611, 0.7773170766911672303, 0.8047378541243631611, 0.7773170766911672303, 0.8047378541243631611, 0.7773170766911672303, 0.8047378541243631611, 0.7773170766911672303, 0.8047378541243631611, 0.7773170766911672303, 0.8047378541243631611, 0.7773170766911672303, 0.8047378541243631611, 0.7773170766911672303, 0.8047378541243631611, 0.7773170766911672303, 0.8047378541243631611, 0.7773170766911672303, 0.8047378541243631611, 0.7773170766911672303, 0.8047378541243631611, 0.7773170766911672303, 0.8047378541243631611, 0.7773170766911672303, 0.8047378541243631611, 0.7773170766911672303, 0.8047378541243631611, 0.7773170766911672303, 0.8047378541243631611, 0.7773170766911672303, 0.8047378541243631611, 0.7773170766911672303, 0.8047378541243631611, 0.7773170766911672303, 0.8047378541243631611, 0.7773170766911672303, 0.8047378541243631611, 0.7773170766911672303, 0.8047378541243631611, 0.7773170766911672303, 0.8047378541243631611, 0.7773170766911672303, 0.8047378541243631611, 0.7773170766911672303, 0.8047378541243631611, 0.7773170766911672303, 0.8047378541243631611, 0.7773170766911672303, 0.8047378541243631611, 0.7773170766911672303, 0.8047378541243631611, 0.7773170766911672303, 0.8047378541243631611, 0.7773170766911672303, 0.8047378541243631611, 0.7773170766911672303, 0.8047378541243631611, 0.7773170766911672303, 0.8047378541243631611, 0.7773170766911672303, 0.8047378541243631611, 0.7773170766911672303, 0.8047378541243631611, 0.7773170766911672303, 0.8047378541243631611, 0.7773170766911672303, 0.8047378541243631611, 0.7773170766911672303, 0.8047378541243631611, 0.7773170766911672303, 0.8047378541243631611, 0.7773170766911672303, 0.8047378541243631611, 0.7773170766911672303, 0.8047378541243631611, 0.7773170766911672303, 0.8047378541243631611, 0.7773170766911672303, 0.8047378541243631611, 0.7773170766911672303, 0.8047378541243631611, 0.7773170766911672303, 0.8047378541243631611, 0.7773170766911672303, 0.8047378541243631611, 0.7773170766911672303, 0.8047378541243631611, 0.7773170766911672303, 0.8047378541243631611, 0.7773170766911672303, 0.8047378541243631611, 0.7773170766911672303, 0.8047378541243631611, 0.7773170766911672303, 0.8047378541243631611, 0.7773170766911672303, 0.8047378541243631611, 0.7773170766911672303, 0.8047378541243631611, 0.7773170766911672303, 0.8047378541243631611, 0.7773170766911672303, 0.8047378541243631611, 0.7773170766911672303, 0.8047378541243631611, 0.7773170766911672303, 0.8047378541243631611, 0.7773170766911672303, 0.8047378541243631611, 0.7773170766911672303, 0.8047378541243631611, 0.7773170766911672303, 0.8047378541243631611, 0.7773170766911672303, 0.8047378541243631611, 0.7773170766911672303, 0.8047378541243631611, 0.7773170766911672303, 0.8047378541243631611, 0.7773170766911672303, 0.8047378541243631611, 0.7773170766911672303, 0.8047378541243631611, 0.7773170766911672303, 0.8047378541243631611, 0.7773170766911672303, 0.8047378541243631611, 0.7773170766911672303, 0.8047378541243631611, 0.7773170766911672303, 0.8047378541243631611, 0.7773170766911672303, 0.8047378541243631611, 0.7773170766911672303, 0.8047378541243631611, 0.7773170766911672303, 0.8047378541243631611, 0.7773170766911672303, 0.8047378541243631611, 0.7773170766911672303, 0.8047378541243631611, 0.7773170766911672303, 0.8047378541243631611, 0.7773170766911672303, 0.8047378541243631611, 0.7773170766911672303, 0.8047378541243631611, 0.7773170766911672303, 0.8047378541243631611, 0.7773170766911672303, 0.8047378541243631611, 0.7773170766911672303, 0.8047378541243631611, 0.7773170766911672303, 0.8047378541243631611, 0.7773170766911672303, 0.8047378541243631611, 0.7773170766911672303, 0.8047378541243631611, 0.7773170766911672303, 0.8047378541243631611, 0.7773170766911672303, 0.8047378541243631611, 0.7773170766911672303, 0.8047378541243631611, 0.7773170766911672303, 0.8047378541243631611, 0.7773170766911672303, 0.8047378541243631611, 0.7773170766911672303, 0.8047378541243631611, 0.7773170766911672303, 0.8047378541243631611, 0.7773170766911672303, 0.8047378541243631611, 0.7773170766911672303, 0.8047378541243631611, 0.7773170766911672303, 0.8047378541243631611, 0.7773170766911672303, 0.8047378541243631611, 0.7773170766911672303, 0.8047378541243631611, 0.7773170766911672303, 0.8047378541243631611, 0.7773170766911672303, 0.8047378541243631611, 0.7773170766911672303, 0.8047378541243631611, 0.7773170766911672303, 0.8047378541243631611, 0.7773170766911672303, 0.8047378541243631611, 0.7773170766911672303, 0.8047378541243631611, 0.7773170766911672303, 0.8047378541243631611, 0.7773170766911672303, 0.8047378541243631611, 0.7773170766911672303, 0.8047378541243631611, 0.7773170766911672303, 0.8047378541243631611, 0.7773170766911672303, 0.8047378541243631611, 0.7773170766911672303, 0.8047378541243631611, 0.7773170766911672303, 0.8047378541243631611, 0.7773170766911672303, 0.8047378541243631611, 0.7773170766911672303, 0.8047378541243631611, 0.7773170766911672303, 0.8047378541243631611, 0.7773170766911672303, 0.8047378541243631611, 0.7773170766911672303, 0.8047378541243631611, 0.7773170766911672303, 0.8047378541243631611, 0.7773170766911672303, 0.8047378541243631611, 0.7773170766911672303, 0.8047378541243631611, 0.7773170766911672303, 0.8047378541243631611, 0.7773170766911672303, 0.8047378541243631611, 0.7773170766911672303, 0.8047378541243631611, 0.7773170766911672303, 0.8047378541243631611, 0.7773170766911672303, 0.8047378541243631611, 0.7773170766911672303, 0.8047378541243631611, 0.7773170766911672303, 0.8047378541243631611, 0.7773170766911672303, 0.8047378541243631611, 0.7773170766911672303, 0.8047378541243631611, 0.7773170766911672303, 0.8047378541243631611, 0.7773170766911672303, 0.8047378541243631611, 0.7773170766911672303, 0.8047378541243631611, 0.7773170766911672303, 0.8047378541243631611, 0.7773170766911672303, 0.8047378541243631611, 0.7773170766911672303, 0.8047378541243631611, 0.7773170766911672303, 0.8047378541243631611, 0.7773170766911672303, 0.8047378541243631611, 0.7773170766911672303, 0.8047378541243631611, 0.7773170766911672303, 0.8047378541243631611, 0.7773170766911672303, 0.8047378541243631611, 0.7773170766911672303, 0.8047378541243631611, 0.7773170766911672303, 0.8047378541243631611, 0.7773170766911672303, 0.8047378541243631611, 0.7773170766911672303, 0.8047378541243631611, 0.7773170766911672303, 0.8047378541243631611, 0.7773170766911672303, 0.8047378541243631611, 0.7773170766911672303, 0.8047378541243631611, 0.7773170766911672303, 0.8047378541243631611, 0.7773170766911672303, 0.8047378541243631611, 0.7773170766911672303, 0.8047378541243631611, 0.7773170766911672303, 0.8047378541243631611, 0.7773170766911672303, 0.8047378541243631611, 0.7773170766911672303, 0.8047378541243631611, 0.7773170766911672303, 0.8047378541243631611, 0.7773170766911672303, 0.8047378541243631611, 0.7773170766911672303, 0.8047378541243631611, 0.7773170766911672303, 0.8047378541243631611, 0.7773170766911672303, 0.8047378541243631611, 0.7773170766911672303, 0.8047378541243631611, 0.7773170766911672303, 0.8047378541243631611, 0.7773170766911672303, 0.8047378541243631611, 0.7773170766911672303, 0.8047378541243631611, 0.7773170766911672303, 0.8047378541243631611, 0.7773170766911672303, 0.8047378541243631611, 0.7773170766911672303, 0.8047378541243631611, 0.7773170766911672303, 0.8047378541243631611, 0.7773170766911672303, 0.8047378541243631611, 0.7773170766911672303, 0.8047378541243631611, 0.7773170766911672303, 0.8047378541243631611, 0.7773170766911672303, 0.8047378541243631611, 0.7773170766911672303, 0.8047378541243631611, 0.7773170766911672303, 0.8047378541243631611, 0.7773170766911672303, 0.8047378541243631611, 0.7773170766911672303, 0.8047378541243631611, 0.7773170766911672303, 0.8047378541243631611, 0.7773170766911672303, 0.8047378541243631611, 0.7773170766911672303, 0.8047378541243631611, 0.7773170766911672303, 0.8047378541243631611, 0.7773170766911672303, 0.8047378541243631611, 0.7773170766911672303, 0.8047378541243631611, 0.7773170766911672303, 0.8047378541243631611, 0.7773170766911672303, 0.8047378541243631611),
 ( 1.000000000000000000, 0.9659258262890683122, 1.000000000000000000, 0.9659258262890683122, 1.000000000000000000, 0.9659258262890683122, 1.000000000000000000, 0.9659258262890683122, 1.000000000000000000, 0.9659258262890683122, 1.000000000000000000, 0.9659258262890683122, 1.000000000000000000, 0.9659258262890683122, 1.000000000000000000, 0.9659258262890683122, 1.000000000000000000, 0.9659258262890683122, 1.000000000000000000, 0.9659258262890683122, 1.000000000000000000, 0.9659258262890683122, 1.000000000000000000, 0.9659258262890683122, 1.000000000000000000, 0.9659258262890683122, 1.000000000000000000, 0.9659258262890683122, 1.000000000000000000, 0.9659258262890683122, 1.000000000000000000, 0.9659258262890683122, 1.000000000000000000, 0.9659258262890683122, 1.000000000000000000, 0.9659258262890683122, 1.000000000000000000, 0.9659258262890683122, 1.000000000000000000, 0.9659258262890683122, 1.000000000000000000, 0.9659258262890683122, 1.000000000000000000, 0.9659258262890683122, 1.000000000000000000, 0.9659258262890683122, 1.000000000000000000, 0.9659258262890683122, 1.000000000000000000, 0.9659258262890683122, 1.000000000000000000, 0.9659258262890683122, 1.000000000000000000, 0.9659258262890683122, 1.000000000000000000, 0.9659258262890683122, 1.000000000000000000, 0.9659258262890683122, 1.000000000000000000, 0.9659258262890683122, 1.000000000000000000, 0.9659258262890683122, 1.000000000000000000, 0.9659258262890683122, 1.000000000000000000, 0.9659258262890683122, 1.000000000000000000, 0.9659258262890683122, 1.000000000000000000, 0.9659258262890683122, 1.000000000000000000, 0.9659258262890683122, 1.000000000000000000, 0.9659258262890683122, 1.000000000000000000, 0.9659258262890683122, 1.000000000000000000, 0.9659258262890683122, 1.000000000000000000, 0.9659258262890683122, 1.000000000000000000, 0.9659258262890683122, 1.000000000000000000, 0.9659258262890683122, 1.000000000000000000, 0.9659258262890683122, 1.000000000000000000, 0.9659258262890683122, 1.000000000000000000, 0.9659258262890683122, 1.000000000000000000, 0.9659258262890683122, 1.000000000000000000, 0.9659258262890683122, 1.000000000000000000, 0.9659258262890683122, 1.000000000000000000, 0.9659258262890683122, 1.000000000000000000, 0.9659258262890683122, 1.000000000000000000, 0.9659258262890683122, 1.000000000000000000, 0.9659258262890683122, 1.000000000000000000, 0.9659258262890683122, 1.000000000000000000, 0.9659258262890683122, 1.000000000000000000, 0.9659258262890683122, 1.000000000000000000, 0.9659258262890683122, 1.000000000000000000, 0.9659258262890683122, 1.000000000000000000, 0.9659258262890683122, 1.000000000000000000, 0.9659258262890683122, 1.000000000000000000, 0.9659258262890683122, 1.000000000000000000, 0.9659258262890683122, 1.000000000000000000, 0.9659258262890683122, 1.000000000000000000, 0.9659258262890683122, 1.000000000000000000, 0.9659258262890683122, 1.000000000000000000, 0.9659258262890683122, 1.000000000000000000, 0.9659258262890683122, 1.000000000000000000, 0.9659258262890683122, 1.000000000000000000, 0.9659258262890683122, 1.000000000000000000, 0.9659258262890683122, 1.000000000000000000, 0.9659258262890683122, 1.000000000000000000, 0.9659258262890683122, 1.000000000000000000, 0.9659258262890683122, 1.000000000000000000, 0.9659258262890683122, 1.000000000000000000, 0.9659258262890683122, 1.000000000000000000, 0.9659258262890683122, 1.000000000000000000, 0.9659258262890683122, 1.000000000000000000, 0.9659258262890683122, 1.000000000000000000, 0.9659258262890683122, 1.000000000000000000, 0.9659258262890683122, 1.000000000000000000, 0.9659258262890683122, 1.000000000000000000, 0.9659258262890683122, 1.000000000000000000, 0.9659258262890683122, 1.000000000000000000, 0.9659258262890683122, 1.000000000000000000, 0.9659258262890683122, 1.000000000000000000, 0.9659258262890683122, 1.000000000000000000, 0.9659258262890683122, 1.000000000000000000, 0.9659258262890683122, 1.000000000000000000, 0.9659258262890683122, 1.000000000000000000, 0.9659258262890683122, 1.000000000000000000, 0.9659258262890683122, 1.000000000000000000, 0.9659258262890683122, 1.000000000000000000, 0.9659258262890683122, 1.000000000000000000, 0.9659258262890683122, 1.000000000000000000, 0.9659258262890683122, 1.000000000000000000, 0.9659258262890683122, 1.000000000000000000, 0.9659258262890683122, 1.000000000000000000, 0.9659258262890683122, 1.000000000000000000, 0.9659258262890683122, 1.000000000000000000, 0.9659258262890683122, 1.000000000000000000, 0.9659258262890683122, 1.000000000000000000, 0.9659258262890683122, 1.000000000000000000, 0.9659258262890683122, 1.000000000000000000, 0.9659258262890683122, 1.000000000000000000, 0.9659258262890683122, 1.000000000000000000, 0.9659258262890683122, 1.000000000000000000, 0.9659258262890683122, 1.000000000000000000, 0.9659258262890683122, 1.000000000000000000, 0.9659258262890683122, 1.000000000000000000, 0.9659258262890683122, 1.000000000000000000, 0.9659258262890683122, 1.000000000000000000, 0.9659258262890683122, 1.000000000000000000, 0.9659258262890683122, 1.000000000000000000, 0.9659258262890683122, 1.000000000000000000, 0.9659258262890683122, 1.000000000000000000, 0.9659258262890683122, 1.000000000000000000, 0.9659258262890683122, 1.000000000000000000, 0.9659258262890683122, 1.000000000000000000, 0.9659258262890683122, 1.000000000000000000, 0.9659258262890683122, 1.000000000000000000, 0.9659258262890683122, 1.000000000000000000, 0.9659258262890683122, 1.000000000000000000, 0.9659258262890683122, 1.000000000000000000, 0.9659258262890683122, 1.000000000000000000, 0.9659258262890683122, 1.000000000000000000, 0.9659258262890683122, 1.000000000000000000, 0.9659258262890683122, 1.000000000000000000, 0.9659258262890683122, 1.000000000000000000, 0.9659258262890683122, 1.000000000000000000, 0.9659258262890683122, 1.000000000000000000, 0.9659258262890683122, 1.000000000000000000, 0.9659258262890683122, 1.000000000000000000, 0.9659258262890683122, 1.000000000000000000, 0.9659258262890683122, 1.000000000000000000, 0.9659258262890683122, 1.000000000000000000, 0.9659258262890683122, 1.000000000000000000, 0.9659258262890683122, 1.000000000000000000, 0.9659258262890683122, 1.000000000000000000, 0.9659258262890683122, 1.000000000000000000, 0.9659258262890683122, 1.000000000000000000, 0.9659258262890683122, 1.000000000000000000, 0.9659258262890683122, 1.000000000000000000, 0.9659258262890683122, 1.000000000000000000, 0.9659258262890683122, 1.000000000000000000, 0.9659258262890683122, 1.000000000000000000, 0.9659258262890683122, 1.000000000000000000, 0.9659258262890683122, 1.000000000000000000, 0.9659258262890683122, 1.000000000000000000, 0.9659258262890683122, 1.000000000000000000, 0.9659258262890683122, 1.000000000000000000, 0.9659258262890683122, 1.000000000000000000, 0.9659258262890683122, 1.000000000000000000, 0.9659258262890683122, 1.000000000000000000, 0.9659258262890683122, 1.000000000000000000, 0.9659258262890683122, 1.000000000000000000, 0.9659258262890683122, 1.000000000000000000, 0.9659258262890683122, 1.000000000000000000, 0.9659258262890683122, 1.000000000000000000, 0.9659258262890683122, 1.000000000000000000, 0.9659258262890683122, 1.000000000000000000, 0.9659258262890683122, 1.000000000000000000, 0.9659258262890683122, 1.000000000000000000, 0.9659258262890683122, 1.000000000000000000, 0.9659258262890683122, 1.000000000000000000, 0.9659258262890683122, 1.000000000000000000, 0.9659258262890683122, 1.000000000000000000, 0.9659258262890683122, 1.000000000000000000, 0.9659258262890683122, 1.000000000000000000, 0.9659258262890683122, 1.000000000000000000, 0.9659258262890683122, 1.000000000000000000, 0.9659258262890683122, 1.000000000000000000, 0.9659258262890683122, 1.000000000000000000, 0.9659258262890683122, 1.000000000000000000, 0.9659258262890683122, 1.000000000000000000, 0.9659258262890683122, 1.000000000000000000, 0.9659258262890683122, 1.000000000000000000, 0.9659258262890683122, 1.000000000000000000, 0.9659258262890683122, 1.000000000000000000, 0.9659258262890683122, 1.000000000000000000, 0.9659258262890683122, 1.000000000000000000, 0.9659258262890683122, 1.000000000000000000, 0.9659258262890683122, 1.000000000000000000, 0.9659258262890683122, 1.000000000000000000, 0.9659258262890683122, 1.000000000000000000, 0.9659258262890683122, 1.000000000000000000, 0.9659258262890683122, 1.000000000000000000, 0.9659258262890683122, 1.000000000000000000, 0.9659258262890683122, 1.000000000000000000, 0.9659258262890683122, 1.000000000000000000, 0.9659258262890683122, 1.000000000000000000, 0.9659258262890683122, 1.000000000000000000, 0.9659258262890683122, 1.000000000000000000, 0.9659258262890683122, 1.000000000000000000, 0.9659258262890683122, 1.000000000000000000, 0.9659258262890683122, 1.000000000000000000, 0.9659258262890683122, 1.000000000000000000, 0.9659258262890683122, 1.000000000000000000, 0.9659258262890683122, 1.000000000000000000, 0.9659258262890683122, 1.000000000000000000, 0.9659258262890683122, 1.000000000000000000, 0.9659258262890683122, 1.000000000000000000, 0.9659258262890683122, 1.000000000000000000, 0.9659258262890683122, 1.000000000000000000, 0.9659258262890683122, 1.000000000000000000, 0.9659258262890683122, 1.000000000000000000, 0.9659258262890683122, 1.000000000000000000, 0.9659258262890683122, 1.000000000000000000, 0.9659258262890683122, 1.000000000000000000, 0.9659258262890683122, 1.000000000000000000, 0.9659258262890683122, 1.000000000000000000, 0.9659258262890683122, 1.000000000000000000, 0.9659258262890683122, 1.000000000000000000, 0.9659258262890683122, 1.000000000000000000, 0.9659258262890683122, 1.000000000000000000, 0.9659258262890683122, 1.000000000000000000, 0.9659258262890683122, 1.000000000000000000, 0.9659258262890683122, 1.000000000000000000, 0.9659258262890683122, 1.000000000000000000, 0.9659258262890683122, 1.000000000000000000, 0.9659258262890683122, 1.000000000000000000, 0.9659258262890683122, 1.000000000000000000, 0.9659258262890683122, 1.000000000000000000, 0.9659258262890683122, 1.000000000000000000, 0.9659258262890683122, 1.000000000000000000, 0.9659258262890683122, 1.000000000000000000, 0.9659258262890683122, 1.000000000000000000, 0.9659258262890683122, 1.000000000000000000, 0.9659258262890683122, 1.000000000000000000, 0.9659258262890683122, 1.000000000000000000, 0.9659258262890683122, 1.000000000000000000, 0.9659258262890683122, 1.000000000000000000, 0.9659258262890683122, 1.000000000000000000, 0.9659258262890683122, 1.000000000000000000, 0.9659258262890683122, 1.000000000000000000, 0.9659258262890683122, 1.000000000000000000, 0.9659258262890683122, 1.000000000000000000, 0.9659258262890683122, 1.000000000000000000, 0.9659258262890683122, 1.000000000000000000) ) ) 
 REPRESENTATION_ITEM ( '' )  SURFACE ( )  );
#48914=CARTESIAN_POINT ( 'NONE',  ( 0.2925321140481932369, -0.2925321140481932369, -2.933070866141732402 ) ) ;
#48915=CARTESIAN_POINT ( 'NONE',  ( -0.2891555358219908833, -0.2891555358219912164, -2.263779527559055094 ) ) ;
#48918=CARTESIAN_POINT ( 'NONE',  ( -0.1958661417322836718, 0.3392501089628017219, -0.7926509186351704539 ) ) ;
#48921=CARTESIAN_POINT ( 'NONE',  ( -0.4091458600556405756, 0.2362204724409446288, -2.545931758530183497 ) ) ;
#48927=CARTESIAN_POINT ( 'NONE',  ( 0.1049643490035303689, 0.3917322834645668994, -0.2309518128270847681 ) ) ;
#48933=CARTESIAN_POINT ( 'NONE',  ( -0.1998031496062994683, 0.3460692066303958092, -2.847769028871391050 ) ) ;
#48934=CARTESIAN_POINT ( 'NONE',  ( -9.594673741351313045E-17, 0.3917322834645670659, -1.729021940453755013 ) ) ;
#48940=CARTESIAN_POINT ( 'NONE',  ( 0.3917322834645670104, -0.1049643490035303411, -1.141076115485564202 ) ) ;
#48951=CARTESIAN_POINT ( 'NONE',  ( -0.1958661417322836718, 0.3392501089628017219, -2.367454068241469756 ) ) ;
#48958=CARTESIAN_POINT ( 'NONE',  ( 0.1049643490035303689, 0.3917322834645670104, -0.8654855643044619962 ) ) ;
#48959=CARTESIAN_POINT ( 'NONE',  ( 0.4091458600556404646, -0.2362204724409448231, -0.02427821522309711946 ) ) ;
#48961=AXIS2_PLACEMENT_3D ( 'NONE', #25316, #11890, #55651 ) ;
#48962=CARTESIAN_POINT ( 'NONE',  ( 0.3996062992125985480, 2.446882876249141654E-17, -2.242125984251968518 ) ) ;
#48971=CARTESIAN_POINT ( 'NONE',  ( 0.3996062992125984925, 0.1070741851644054499, -2.091207349081364963 ) ) ;
#48973=FACE_OUTER_BOUND ( 'NONE', #62889, .T. ) ;
#48980=CARTESIAN_POINT ( 'NONE',  ( -0.3917322834645670659, 0.1049643490035301607, -1.530164411252281420 ) ) ;
#48990=CARTESIAN_POINT ( 'NONE',  ( -0.1958661417322833942, -0.3392501089628018884, -0.6922765336296082817 ) ) ;
#48993=CARTESIAN_POINT ( 'NONE',  ( -0.2362204724409451284, 0.4091458600556402425, -2.137139107611548905 ) ) ;
#49011=ADVANCED_FACE ( 'NONE', ( #75044 ), #43021, .T. ) ;
#49015=CARTESIAN_POINT ( 'NONE',  ( -0.1070741851644051862, -0.3996062992125986590, -2.038713910761154491 ) ) ;
#49020=CARTESIAN_POINT ( 'NONE',  ( -0.3996062992125986035, -7.340648628747425578E-17, -1.771653543307086576 ) ) ;
#49022=CARTESIAN_POINT ( 'NONE',  ( 0.1974969037888706369, -0.3420746716998659953, -1.036745406824147064 ) ) ;
#49023=CARTESIAN_POINT ( 'NONE',  ( -0.2925321140481930704, -0.2925321140481933480, -2.578740157480315265 ) ) ;
#49025=CARTESIAN_POINT ( 'NONE',  ( 0.3392501089628018884, -0.1958661417322834220, -0.4120734908136482466 ) ) ;
#49029=CARTESIAN_POINT ( 'NONE',  ( 0.3949938075777409963, 2.418639510665530743E-17, -2.242125984251968518 ) ) ;
#49032=CARTESIAN_POINT ( 'NONE',  ( -0.3458507752293909498, 0.3458507752293907833, -2.381889763779527325 ) ) ;
#49033=CARTESIAN_POINT ( 'NONE',  ( -0.2925321140481930704, -0.2925321140481933480, -1.633858267716534973 ) ) ;
#49039=CARTESIAN_POINT ( 'NONE',  ( 0.1049643490035304522, -0.3917322834645668994, -2.842500369257531023 ) ) ;
#49046=CARTESIAN_POINT ( 'NONE',  ( -0.1049643490035307020, 0.3917322834645669549, -0.09120734908136493568 ) ) ;
#49048=CARTESIAN_POINT ( 'NONE',  ( 0.1049643490035304938, -0.3917322834645669549, -2.439632545931758045 ) ) ;
#49051=CARTESIAN_POINT ( 'NONE',  ( -0.3420746716998661618, 0.1974969037888702206, -2.703412073490814027 ) ) ;
#49055=CARTESIAN_POINT ( 'NONE',  ( -0.1070741851644051862, -0.3996062992125987146, -1.017060367454067915 ) ) ;
#49060=CARTESIAN_POINT ( 'NONE',  ( 0.3917322834645670104, -0.1049643490035303411, -0.5111548556430445256 ) ) ;
#49067=CARTESIAN_POINT ( 'NONE',  ( -0.1049643490035307020, 0.3917322834645669549, -0.1561679790026246351 ) ) ;
#49070=DIRECTION ( 'NONE',  ( 1.000000000000000000, 0.000000000000000000, 0.000000000000000000 ) ) ;
#49071=CARTESIAN_POINT ( 'NONE',  ( -0.4091458600556402980, -0.2362204724409451284, -1.784776902887138972 ) ) ;
#49080=CARTESIAN_POINT ( 'NONE',  ( 0.2867679344610365999, 0.2867679344610365999, -0.5327890831682923212 ) ) ;
#49082=CARTESIAN_POINT ( 'NONE',  ( 0.2867679344610366554, 0.2867679344610366554, -0.2224409448818898127 ) ) ;
#49087=CARTESIAN_POINT ( 'NONE',  ( 0.2867679344610365999, -0.2867679344610365444, -2.137795275590551380 ) ) ;
#49090=CARTESIAN_POINT ( 'NONE',  ( -0.4724409448818899238, 0.1265901696524986686, -0.7395013123359580609 ) ) ;
#49101=CARTESIAN_POINT ( 'NONE',  ( 0.2925321140481932369, 0.2925321140481932369, -2.104330708661417138 ) ) ;
#49109=CARTESIAN_POINT ( 'NONE',  ( 0.2925321140481931814, 0.2925321140481931814, -0.05708661417322837689 ) ) ;
#49110=CARTESIAN_POINT ( 'NONE',  ( 0.2925321140481932369, 0.2925321140481932369, -0.6102362204724409711 ) ) ;
#49111=CARTESIAN_POINT ( 'NONE',  ( -0.2891555358219911054, 0.2891555358219909388, 0.1377952755905511306 ) ) ;
#49117=CARTESIAN_POINT ( 'NONE',  ( 0.1058382717557499880, 0.3949938075777409408, -1.015091863517060489 ) ) ;
#49122=CARTESIAN_POINT ( 'NONE',  ( 0.4724409448818897572, -0.1265901696524988906, -1.213910761154855189 ) ) ;
#49123=CARTESIAN_POINT ( 'NONE',  ( -0.1998031496062994683, 0.3460692066303958092, -2.217847769028871596 ) ) ;
#49128=CARTESIAN_POINT ( 'NONE',  ( 0.3392501089628018329, 0.1958661417322835607, -0.7578933315298707063 ) ) ;
#49140=CARTESIAN_POINT ( 'NONE',  ( 0.2867679344610365999, -0.2867679344610365444, -1.192913385826771755 ) ) ;
#49142=ORIENTED_EDGE ( 'NONE', *, *, #28554, .T. ) ;
#49143=CARTESIAN_POINT ( 'NONE',  ( -0.1058382717557497937, -0.3949938075777411628, -1.646981627296588035 ) ) ;
#49144=VERTEX_POINT ( 'NONE', #18202 ) ;
#49154=CARTESIAN_POINT ( 'NONE',  ( -0.3458507752293909498, 0.3458507752293908388, -0.4114173228346456046 ) ) ;
#49155=CARTESIAN_POINT ( 'NONE',  ( -0.2867679344610365999, 0.2867679344610364889, 0.2106299212598424508 ) ) ;
#49160=CARTESIAN_POINT ( 'NONE',  ( -0.1070741851644051862, -0.3996062992125987146, -1.961942257217847763 ) ) ;
#49163=CARTESIAN_POINT ( 'NONE',  ( -0.3460692066303960313, 0.1998031496062989965, -1.520341207349081181 ) ) ;
#49164=CARTESIAN_POINT ( 'NONE',  ( -0.4724409448818898682, -8.678599364036362592E-17, -2.401574803149606474 ) ) ;
#49167=CARTESIAN_POINT ( 'NONE',  ( 0.4724409448818897572, -0.1265901696524988906, -0.5839895013123358458 ) ) ;
#49170=CARTESIAN_POINT ( 'NONE',  ( 0.2867679344610365999, -0.2867679344610365444, -2.387795275590551380 ) ) ;
#49177=CARTESIAN_POINT ( 'NONE',  ( -0.4724409448818898682, -8.678599364036362592E-17, -2.163385826771653697 ) ) ;
#49180=CARTESIAN_POINT ( 'NONE',  ( 0.2891555358219910499, 0.2891555358219910499, -2.419291338582677753 ) ) ;
#49199=CARTESIAN_POINT ( 'NONE',  ( 5.785732909357575061E-17, -0.4724409448818898682, -2.755905511811023612 ) ) ;
#49202=CARTESIAN_POINT ( 'NONE',  ( 0.2925321140481932369, -0.2925321140481931814, -0.8051181102362205966 ) ) ;
#49203=CARTESIAN_POINT ( 'NONE',  ( 0.1958661417322834775, 0.3392501089628018884, -1.961286089238845287 ) ) ;
#49212=CARTESIAN_POINT ( 'NONE',  ( -0.1070741851644051862, -0.3996062992125986590, -1.408792650918635259 ) ) ;
#49219=CARTESIAN_POINT ( 'NONE',  ( -0.3392501089628019995, 0.1958661417322832277, -1.685695538057742970 ) ) ;
#49225=CARTESIAN_POINT ( 'NONE',  ( 0.1070741851644054637, -0.3996062992125984925, -2.366797900262467280 ) ) ;
#49229=CARTESIAN_POINT ( 'NONE',  ( 0.3996062992125986035, 0.1070741851644054776, -0.7545931758530182165 ) ) ;
#49230=ORIENTED_EDGE ( 'NONE', *, *, #76425, .F. ) ;
#49232=CARTESIAN_POINT ( 'NONE',  ( 0.2867679344610365999, -0.2867679344610365444, -2.452755905511811108 ) ) ;
#49242=CARTESIAN_POINT ( 'NONE',  ( 0.3392501089628018329, 0.1958661417322835052, -2.101030552984564981 ) ) ;
#49245=CARTESIAN_POINT ( 'NONE',  ( -0.3917322834645670104, -7.196005306013484475E-17, -2.643700787401574548 ) ) ;
#49248=CARTESIAN_POINT ( 'NONE',  ( 0.2891555358219910499, 0.2891555358219910499, -0.1377952755905512694 ) ) ;
#49257=CARTESIAN_POINT ( 'NONE',  ( -9.594673741351313045E-17, 0.3917322834645670659, -1.099100680611235559 ) ) ;
#49259=CARTESIAN_POINT ( 'NONE',  ( 0.3917322834645670104, -0.1049643490035303411, -2.243438320209974357 ) ) ;
#49264=CARTESIAN_POINT ( 'NONE',  ( 0.1070741851644053527, 0.3996062992125986590, -0.4658792650918635592 ) ) ;
#49266=CARTESIAN_POINT ( 'NONE',  ( 4.893765752498283308E-17, -0.3996062992125985480, -0.3129921259842520231 ) ) ;
#49268=CARTESIAN_POINT ( 'NONE',  ( -9.787531504996567848E-17, 0.3996062992125986035, -2.362204724409448620 ) ) ;
#49273=CARTESIAN_POINT ( 'NONE',  ( 0.2362204724409449064, 0.4091458600556404646, -1.166010498687663821 ) ) ;
#49276=CARTESIAN_POINT ( 'NONE',  ( -0.3420746716998660508, -0.1974969037888706924, -0.6017060367454067915 ) ) ;
#49289=CARTESIAN_POINT ( 'NONE',  ( 0.3460692066303958092, 0.1998031496062993018, -1.625328083989501460 ) ) ;
#49292=CARTESIAN_POINT ( 'NONE',  ( 0.2867679344610365999, 0.2867679344610365999, -1.704724409448818978 ) ) ;
#49294=LINE ( 'NONE', #22399, #60054 ) ;
#49295=CARTESIAN_POINT ( 'NONE',  ( -0.1123167701215806169, -0.3758920641862485978, -1.519619016692322133E-17 ) ) ;
#49315=CARTESIAN_POINT ( 'NONE',  ( -0.3392501089628017219, -0.1958661417322836995, -2.253956323655855076 ) ) ;
#49323=CARTESIAN_POINT ( 'NONE',  ( -0.3917322834645671215, 0.1049643490035301469, -2.072178477690288734 ) ) ;
#49326=CARTESIAN_POINT ( 'NONE',  ( -0.2362204724409451284, 0.4091458600556402425, -0.4855643044619422644 ) ) ;
#49327=CARTESIAN_POINT ( 'NONE',  ( 0.3949938075777409963, 2.418639510665530435E-17, -2.637795275590551380 ) ) ;
#49330=CARTESIAN_POINT ( 'NONE',  ( -0.3917322834645669549, -0.1049643490035306603, -1.297900262467191590 ) ) ;
#49333=CARTESIAN_POINT ( 'NONE',  ( 5.785732909357575061E-17, -0.4724409448818898682, -2.440944881889763884 ) ) ;
#49339=CARTESIAN_POINT ( 'NONE',  ( -0.3392501089628018329, -0.1958661417322836440, -0.6049675608585809439 ) ) ;
#49347=CARTESIAN_POINT ( 'NONE',  ( -0.1958661417322836995, 0.3392501089628017219, -2.214586244915697222 ) ) ;
#49355=CARTESIAN_POINT ( 'NONE',  ( -0.2867679344610364334, -0.2867679344610367109, -0.7736220472440945573 ) ) ;
#49365=CARTESIAN_POINT ( 'NONE',  ( 0.1049643490035304938, -0.3917322834645669549, -2.754593175853017328 ) ) ;
#49371=CARTESIAN_POINT ( 'NONE',  ( 0.000000000000000000, 0.000000000000000000, -2.755905511811024056 ) ) ;
#49372=CARTESIAN_POINT ( 'NONE',  ( 0.3917322834645670104, -0.1049643490035303411, -0.9835958005249345604 ) ) ;
#49373=CARTESIAN_POINT ( 'NONE',  ( -0.2362204724409451284, 0.4091458600556402425, 0.2250656167979002698 ) ) ;
#49375=CARTESIAN_POINT ( 'NONE',  ( -9.787531504996566615E-17, 0.3996062992125985480, -2.438976377952756014 ) ) ;
#49385=CARTESIAN_POINT ( 'NONE',  ( 0.1998031496062992463, 0.3460692066303959202, -0.3786089238845143923 ) ) ;
#49387=CARTESIAN_POINT ( 'NONE',  ( 0.1049643490035304938, -0.3917322834645669549, -0.2349081364829396223 ) ) ;
#49395=CARTESIAN_POINT ( 'NONE',  ( 0.3917322834645668994, -0.1049643490035303134, -1.451424253771966599 ) ) ;
#49404=CARTESIAN_POINT ( 'NONE',  ( 0.1049643490035304799, -0.3917322834645670104, -0.5544812580390570123 ) ) ;
#49410=CARTESIAN_POINT ( 'NONE',  ( 0.2362204724409451007, -0.4091458600556402980, -1.900918635170603554 ) ) ;
#49431=CARTESIAN_POINT ( 'NONE',  ( 0.2925321140481932369, -0.2925321140481931814, -2.064960629921259727 ) ) ;
#49436=CARTESIAN_POINT ( 'NONE',  ( -0.3996062992125987146, 0.1070741851644051862, -1.765091863517059823 ) ) ;
#49437=CARTESIAN_POINT ( 'NONE',  ( 0.3420746716998659953, 0.1974969037888705536, -1.706036745406824151 ) ) ;
#49438=CARTESIAN_POINT ( 'NONE',  ( -0.3460692066303960868, 0.1998031496062990242, -2.860892388451443669 ) ) ;
#49440=CARTESIAN_POINT ( 'NONE',  ( 0.1958661417322834775, 0.3392501089628018884, -0.7664041994750655507 ) ) ;
#49444=CARTESIAN_POINT ( 'NONE',  ( 0.1058382717557499880, 0.3949938075777409408, -2.117454068241470200 ) ) ;
#49448=CARTESIAN_POINT ( 'NONE',  ( -1.157146581871515012E-16, 0.4724409448818898682, -2.519685039370078705 ) ) ;
#49449=CARTESIAN_POINT ( 'NONE',  ( -0.3996062992125986035, -0.1070741851644056997, -1.620734908136482799 ) ) ;
#49456=CARTESIAN_POINT ( 'NONE',  ( 4.797336870675655290E-17, -0.3917322834645669549, -2.678458374506874851 ) ) ;
#49463=CARTESIAN_POINT ( 'NONE',  ( 0.3917322834645670104, 2.398668435337828261E-17, -0.2027559055118111353 ) ) ;
#49465=CARTESIAN_POINT ( 'NONE',  ( -0.2867679344610364334, -0.2867679344610367109, -2.098425196850393526 ) ) ;
#49468=CARTESIAN_POINT ( 'NONE',  ( 0.3420746716998659953, 0.1974969037888705536, -2.650918635170603554 ) ) ;
#49473=CARTESIAN_POINT ( 'NONE',  ( 0.1998031496062994405, -0.3460692066303958092, -1.194225721784776928 ) ) ;
#49478=CARTESIAN_POINT ( 'NONE',  ( -0.2867679344610364334, -0.2867679344610367109, -0.3011811023622048000 ) ) ;
#49484=CARTESIAN_POINT ( 'NONE',  ( -0.2867679344610364334, -0.2867679344610367109, -0.2086614173228345248 ) ) ;
#49488=CARTESIAN_POINT ( 'NONE',  ( -0.4091458600556405756, 0.2362204724409446288, -1.601049868766404094 ) ) ;
#49489=CARTESIAN_POINT ( 'NONE',  ( 0.4724409448818898682, 2.892866454678787531E-17, -2.242125984251968518 ) ) ;
#49491=CARTESIAN_POINT ( 'NONE',  ( 0.4091458600556403535, 0.2362204724409449896, -0.9186351706036745002 ) ) ;
#49498=CARTESIAN_POINT ( 'NONE',  ( -0.3917322834645670659, 0.1049643490035301607, -0.4278022065278722641 ) ) ;
#49500=CARTESIAN_POINT ( 'NONE',  ( 0.3917322834645669549, 0.1049643490035304660, -0.3667979002624672802 ) ) ;
#49505=CARTESIAN_POINT ( 'NONE',  ( -0.3917322834645671215, 0.1049643490035301469, -2.229658792650918819 ) ) ;
#49508=CARTESIAN_POINT ( 'NONE',  ( 0.4091458600556404646, -0.2362204724409448231, -0.6541994750656167090 ) ) ;
#49519=CARTESIAN_POINT ( 'NONE',  ( 0.3996062992125986035, -0.1070741851644052972, -1.920603674540682038 ) ) ;
#49527=CARTESIAN_POINT ( 'NONE',  ( -0.3996062992125985480, -7.340648628747423112E-17, -0.4311023622047244208 ) ) ;
#49528=CARTESIAN_POINT ( 'NONE',  ( -0.3996062992125986035, -7.340648628747425578E-17, -0.6692913385826770867 ) ) ;
#49529=CARTESIAN_POINT ( 'NONE',  ( 0.1058382717557499880, 0.3949938075777411073, 0.006561679790026190250 ) ) ;
#49534=CARTESIAN_POINT ( 'NONE',  ( -0.2891555358219911054, 0.2891555358219909388, -0.8838582677165351953 ) ) ;
#49539=CARTESIAN_POINT ( 'NONE',  ( -0.4724409448818898682, -8.678599364036362592E-17, -1.299212598425196985 ) ) ;
#49540=CARTESIAN_POINT ( 'NONE',  ( 0.1998031496062992740, 0.3460692066303959757, -2.349081364829396446 ) ) ;
#49543=CARTESIAN_POINT ( 'NONE',  ( 0.3917322834645670659, -0.1049643490035303273, -0.5807279771991620265 ) ) ;
#49556=CARTESIAN_POINT ( 'NONE',  ( -9.594673741351313045E-17, 0.3917322834645670104, -0.9370078740157480324 ) ) ;
#49559=CARTESIAN_POINT ( 'NONE',  ( 0.1058382717557500713, -0.3949938075777409408, -1.345144356955380704 ) ) ;
#49570=CARTESIAN_POINT ( 'NONE',  ( 0.3917322834645670104, -0.1049643490035303411, 0.1187664041994749703 ) ) ;
#49576=CARTESIAN_POINT ( 'NONE',  ( 0.3460692066303959202, 0.1998031496062993295, -2.020997375328084100 ) ) ;
#49579=CARTESIAN_POINT ( 'NONE',  ( -0.1998031496062991630, -0.3460692066303959202, -1.717191601049868677 ) ) ;
#49583=CARTESIAN_POINT ( 'NONE',  ( 0.4724409448818896462, 0.1265901696524990294, -0.2821522309711286258 ) ) ;
#49585=EDGE_CURVE ( 'NONE', #70572, #10673, #51096, .T. ) ;
#49586=CARTESIAN_POINT ( 'NONE',  ( -0.1049643490035302024, -0.3917322834645671215, -2.833989501312335957 ) ) ;
#49592=CARTESIAN_POINT ( 'NONE',  ( -0.2362204724409451284, 0.4091458600556402425, -2.137139107611548905 ) ) ;
#49595=CARTESIAN_POINT ( 'NONE',  ( 0.3420746716998660508, -0.1974969037888704149, -2.386482939632546429 ) ) ;
#49601=CARTESIAN_POINT ( 'NONE',  ( -0.4724409448818898682, -8.678599364036362592E-17, -2.163385826771653697 ) ) ;
#49613=ADVANCED_FACE ( 'NONE', ( #38690 ), #82494, .T. ) ;
#49615=CARTESIAN_POINT ( 'NONE',  ( -9.787531504996566615E-17, 0.3996062992125985480, -0.5492125984251968740 ) ) ;
#49616=CARTESIAN_POINT ( 'NONE',  ( 0.1958661417322836440, -0.3392501089628017219, -2.223753280839895208 ) ) ;
#49626=CARTESIAN_POINT ( 'NONE',  ( -0.1265901696524993347, 0.4724409448818896462, -2.603018372703412187 ) ) ;
#49627=VERTEX_POINT ( 'NONE', #64368 ) ;
#49633=CARTESIAN_POINT ( 'NONE',  ( -0.3917322834645669549, -0.1049643490035306603, -1.547900262467191590 ) ) ;
#49634=CARTESIAN_POINT ( 'NONE',  ( 0.1002886991238245706, 0.3788256970788722588, -1.220472440944881054 ) ) ;
#49637=CARTESIAN_POINT ( 'NONE',  ( 0.2362204724409449064, 0.4091458600556404646, -0.4593175853018372501 ) ) ;
#49638=CARTESIAN_POINT ( 'NONE',  ( -0.3996062992125984925, -0.1070741851644056719, -2.327427821522309870 ) ) ;
#49641=CARTESIAN_POINT ( 'NONE',  ( -0.1998031496062991907, -0.3460692066303959757, -1.010498687664042050 ) ) ;
#49644=CARTESIAN_POINT ( 'NONE',  ( -0.1958661417322834220, -0.3392501089628018884, -2.734908136482939511 ) ) ;
#49651=CARTESIAN_POINT ( 'NONE',  ( 0.000000000000000000, 0.000000000000000000, -2.755905511811024056 ) ) ;
#49654=CARTESIAN_POINT ( 'NONE',  ( -0.3917322834645669549, -7.196005306013483243E-17, -2.009167035924197098 ) ) ;
#49658=CARTESIAN_POINT ( 'NONE',  ( -0.3917322834645670104, -7.196005306013484475E-17, -2.801181102362204633 ) ) ;
#49661=CARTESIAN_POINT ( 'NONE',  ( -9.674558042662121740E-17, 0.3949938075777409963, -5.756223643949423463E-17 ) ) ;
#49669=CARTESIAN_POINT ( 'NONE',  ( -0.1049643490035307158, 0.3917322834645670104, -1.105662360401261868 ) ) ;
#49671=CARTESIAN_POINT ( 'NONE',  ( -0.1958661417322834220, -0.3392501089628018884, -2.512467191601049699 ) ) ;
#49676=CARTESIAN_POINT ( 'NONE',  ( -0.3996062992125986035, -0.1070741851644056997, -0.6758530183727035068 ) ) ;
#49678=CARTESIAN_POINT ( 'NONE',  ( 0.1070741851644054776, -0.3996062992125984925, -0.3195538057742782212 ) ) ;
#49680=CARTESIAN_POINT ( 'NONE',  ( -0.1998031496062991907, -0.3460692066303959757, -2.270341207349081181 ) ) ;
#49684=CARTESIAN_POINT ( 'NONE',  ( -0.4091458600556405756, 0.2362204724409446288, -0.8904199475065617264 ) ) ;
#49687=CARTESIAN_POINT ( 'NONE',  ( 0.3949938075777408852, 0.1058382717557500435, -0.8313648293963256108 ) ) ;
#49699=CARTESIAN_POINT ( 'NONE',  ( 0.1998031496062992463, 0.3460692066303959202, -1.795931758530183719 ) ) ;
#49701=CARTESIAN_POINT ( 'NONE',  ( 0.3917322834645670104, 2.398668435337828261E-17, -1.527559055118110409 ) ) ;
#49705=EDGE_CURVE ( 'NONE', #51988, #5969, #25223, .T. ) ;
#49716=CARTESIAN_POINT ( 'NONE',  ( 0.2867679344610365999, -0.2867679344610365444, -1.127952755905512028 ) ) ;
#49730=CARTESIAN_POINT ( 'NONE',  ( -0.4091458600556402980, -0.2362204724409451284, -0.5249343832020997302 ) ) ;
#49732=CARTESIAN_POINT ( 'NONE',  ( 0.1070741851644054915, -0.3996062992125985480, -1.187664041994750619 ) ) ;
#49737=CARTESIAN_POINT ( 'NONE',  ( -0.4724409448818898682, -8.678599364036362592E-17, -0.1968503937007874127 ) ) ;
#49738=CARTESIAN_POINT ( 'NONE',  ( 0.1974969037888706369, -0.3420746716998659953, -2.611548556430445700 ) ) ;
#49741=CARTESIAN_POINT ( 'NONE',  ( -9.594673741351313045E-17, 0.3917322834645670104, -1.409448818897637734 ) ) ;
#49743=CARTESIAN_POINT ( 'NONE',  ( -0.4724409448818899238, 0.1265901696524986686, -2.395013123359580387 ) ) ;
#49744=CARTESIAN_POINT ( 'NONE',  ( -0.4724409448818899238, 0.1265901696524986964, -0.8969816272965878134 ) ) ;
#49750=CARTESIAN_POINT ( 'NONE',  ( -0.3917322834645668994, -0.1049643490035306742, -0.5984058810685547458 ) ) ;
#49758=CARTESIAN_POINT ( 'NONE',  ( 0.3917322834645670104, 0.1049643490035304660, -2.011174171424884083 ) ) ;
#49764=CARTESIAN_POINT ( 'NONE',  ( -0.1958661417322834220, -0.3392501089628018884, -1.567585301837270295 ) ) ;
#49774=CARTESIAN_POINT ( 'NONE',  ( 0.1958661417322836440, -0.3392501089628017219, -2.603674540682414218 ) ) ;
#49775=ORIENTED_EDGE ( 'NONE', *, *, #78723, .T. ) ;
#49781=CARTESIAN_POINT ( 'NONE',  ( -0.3917322834645670104, -7.196005306013484475E-17, -0.9114173228346457156 ) ) ;
#49782=CARTESIAN_POINT ( 'NONE',  ( -1.157146581871515012E-16, 0.4724409448818898682, 0.2381889763779527491 ) ) ;
#49784=CARTESIAN_POINT ( 'NONE',  ( -0.2891555358219909388, -0.2891555358219912164, 0.1791338582677165503 ) ) ;
#49793=CARTESIAN_POINT ( 'NONE',  ( -0.1070741851644051862, -0.3996062992125986590, -0.6213910761154856077 ) ) ;
#49795=CARTESIAN_POINT ( 'NONE',  ( -0.3917322834645671215, 0.1049643490035301469, -0.3398950131233596239 ) ) ;
#49803=CARTESIAN_POINT ( 'NONE',  ( -0.2867679344610366554, 0.2867679344610365444, -1.832001681593488751 ) ) ;
#49813=CARTESIAN_POINT ( 'NONE',  ( -0.3917322834645670659, -7.196005306013484475E-17, -0.8235101294301331309 ) ) ;
#49817=CARTESIAN_POINT ( 'NONE',  ( -0.3458507752293909498, 0.3458507752293907833, -1.986220472440944906 ) ) ;
#49832=VERTEX_POINT ( 'NONE', #57202 ) ;
#49836=CARTESIAN_POINT ( 'NONE',  ( -0.1070741851644051862, -0.3996062992125986590, -0.07217847769028871985 ) ) ;
#49837=CARTESIAN_POINT ( 'NONE',  ( -0.1070741851644051862, -0.3996062992125986590, -2.511154855643044748 ) ) ;
#49842=CARTESIAN_POINT ( 'NONE',  ( -0.3996062992125986035, -0.1070741851644056997, -2.408136482939632561 ) ) ;
#49843=CARTESIAN_POINT ( 'NONE',  ( 0.1974969037888706369, -0.3420746716998659953, -1.351706036745407014 ) ) ;
#49844=CARTESIAN_POINT ( 'NONE',  ( 4.893765752498283924E-17, -0.3996062992125986035, -2.913385826771653697 ) ) ;
#49846=CARTESIAN_POINT ( 'NONE',  ( 0.1049643490035303689, 0.3917322834645670104, -0.7729658792650917487 ) ) ;
#49850=CARTESIAN_POINT ( 'NONE',  ( 0.3420746716998660508, 0.1974969037888705814, -2.727690288713910949 ) ) ;
#49854=CARTESIAN_POINT ( 'NONE',  ( 0.3458507752293908943, -0.3458507752293908943, -2.303149606299212060 ) ) ;
#49855=CARTESIAN_POINT ( 'NONE',  ( 0.1070741851644053527, 0.3996062992125986590, -2.198162729658792447 ) ) ;
#49862=CARTESIAN_POINT ( 'NONE',  ( 4.797336870675656522E-17, -0.3917322834645670104, -0.005905511811023714773 ) ) ;
#49870=CARTESIAN_POINT ( 'NONE',  ( -0.3392501089628019995, 0.1958661417322832277, -0.5833333333333334814 ) ) ;
#49871=CARTESIAN_POINT ( 'NONE',  ( -0.1049643490035302024, -0.3917322834645671215, -1.481627296587926690 ) ) ;
#49872=CARTESIAN_POINT ( 'NONE',  ( -0.3392501089628019995, 0.1958661417322832277, -2.380577427821522374 ) ) ;
#49875=CARTESIAN_POINT ( 'NONE',  ( -9.674558042662121740E-17, 0.3949938075777409963, -2.677165354330708347 ) ) ;
#49879=CARTESIAN_POINT ( 'NONE',  ( -0.3996062992125986035, -7.340648628747425578E-17, -1.299212598425196985 ) ) ;
#49881=CARTESIAN_POINT ( 'NONE',  ( 0.4724409448818898127, -0.1265901696524988629, -0.8182414698162728817 ) ) ;
#49884=CARTESIAN_POINT ( 'NONE',  ( -0.1049643490035302024, -0.3917322834645671215, -0.4717847769028871152 ) ) ;
#49891=ORIENTED_EDGE ( 'NONE', *, *, #48087, .T. ) ;
#49895=CARTESIAN_POINT ( 'NONE',  ( 0.1265901696524989462, 0.4724409448818897572, -1.568241469816272993 ) ) ;
#49902=CARTESIAN_POINT ( 'NONE',  ( 0.1265901696524990572, -0.4724409448818897017, -2.290026246719159886 ) ) ;
#49906=CARTESIAN_POINT ( 'NONE',  ( -0.1049643490035306742, 0.3917322834645668994, -0.5590358023283972244 ) ) ;
#49909=CARTESIAN_POINT ( 'NONE',  ( -0.3917322834645671215, 0.1049643490035301469, -0.7473753280839894320 ) ) ;
#49914=CARTESIAN_POINT ( 'NONE',  ( -0.3392501089628017219, -0.1958661417322836718, -2.721784776902886893 ) ) ;
#49917=CARTESIAN_POINT ( 'NONE',  ( -0.4724409448818898682, -8.678599364036362592E-17, -0.9035433070866141225 ) ) ;
#49929=CARTESIAN_POINT ( 'NONE',  ( -0.1998031496062991630, -0.3460692066303959202, -1.874671916010498762 ) ) ;
#49937=CARTESIAN_POINT ( 'NONE',  ( 4.893765752498283308E-17, -0.3996062992125985480, -0.6279527559055118058 ) ) ;
#49938=CARTESIAN_POINT ( 'NONE',  ( 0.1070741851644054915, -0.3996062992125986035, -1.030183727034120533 ) ) ;
#49939=CARTESIAN_POINT ( 'NONE',  ( -0.2891555358219908833, -0.2891555358219912164, -0.05905511811023628904 ) ) ;
#49945=CARTESIAN_POINT ( 'NONE',  ( 0.1058382717557499880, 0.3949938075777409408, -1.330052493438319994 ) ) ;
#49950=CARTESIAN_POINT ( 'NONE',  ( 0.2362204724409451007, -0.4091458600556402980, -1.036745406824147064 ) ) ;
#49951=CARTESIAN_POINT ( 'NONE',  ( -9.787531504996567848E-17, 0.3996062992125986035, -2.519685039370078705 ) ) ;
#49954=CARTESIAN_POINT ( 'NONE',  ( 0.3917322834645670104, 0.1049643490035304660, -0.9088119667004745938 ) ) ;
#49965=CARTESIAN_POINT ( 'NONE',  ( -0.1958661417322834220, -0.3392501089628018884, -1.002624671916010568 ) ) ;
#49968=CARTESIAN_POINT ( 'NONE',  ( 0.3420746716998659953, 0.1974969037888705536, -1.548556430446194065 ) ) ;
#49980=CARTESIAN_POINT ( 'NONE',  ( -0.2867679344610365999, 0.2867679344610364889, -0.1043307086614174151 ) ) ;
#49986=CARTESIAN_POINT ( 'NONE',  ( 0.3996062992125986590, -0.1070741851644053111, -2.001312335958005395 ) ) ;
#49989=CARTESIAN_POINT ( 'NONE',  ( -0.3460692066303960313, 0.1998031496062989965, -1.677821522309711266 ) ) ;
#49994=CARTESIAN_POINT ( 'NONE',  ( -0.4724409448818899238, 0.1265901696524986686, -0.5052493438320209140 ) ) ;
#49996=CARTESIAN_POINT ( 'NONE',  ( -0.2867679344610365999, 0.2867679344610364889, -2.781496062992125040 ) ) ;
#50002=CARTESIAN_POINT ( 'NONE',  ( -0.4091458600556402980, -0.2362204724409451284, -2.491469816272966042 ) ) ;
#50004=CARTESIAN_POINT ( 'NONE',  ( -0.1974969037888704149, -0.3420746716998661063, -2.189632545931758489 ) ) ;
#50015=DIRECTION ( 'NONE',  ( 0.000000000000000000, 0.000000000000000000, 1.000000000000000000 ) ) ;
#50017=DIRECTION ( 'NONE',  ( 0.000000000000000000, 0.000000000000000000, 1.000000000000000000 ) ) ;
#50026=CARTESIAN_POINT ( 'NONE',  ( 0.3996062992125986035, -0.1070741851644052972, -0.8182414698162727706 ) ) ;
#50028=CARTESIAN_POINT ( 'NONE',  ( -0.2867679344610365999, 0.2867679344610364889, -2.151574803149605586 ) ) ;
#50037=CARTESIAN_POINT ( 'NONE',  ( 0.1265901696524989184, 0.4724409448818898127, -2.198162729658792447 ) ) ;
#50045=CARTESIAN_POINT ( 'NONE',  ( 0.3917322834645670104, -0.1049643490035303411, -1.613517060367454237 ) ) ;
#50046=CARTESIAN_POINT ( 'NONE',  ( -0.3808816823641234528, 0.09156050430092053938, -1.220472440944881942 ) ) ;
#50051=CARTESIAN_POINT ( 'NONE',  ( 0.3460692066303959202, -0.1998031496062991630, -2.543963254593176071 ) ) ;
#50053=CARTESIAN_POINT ( 'NONE',  ( -0.3460692066303960868, 0.1998031496062990242, -0.9711286089238845287 ) ) ;
#50055=CARTESIAN_POINT ( 'NONE',  ( -0.2867679344610364334, -0.2867679344610367109, -2.570866141732283339 ) ) ;
#50067=CARTESIAN_POINT ( 'NONE',  ( -0.3392501089628019995, 0.1958661417322832277, -2.630577427821522374 ) ) ;
#50070=CARTESIAN_POINT ( 'NONE',  ( 0.3949938075777411073, -0.1058382717557499464, -0.2690288713910761742 ) ) ;
#50073=CARTESIAN_POINT ( 'NONE',  ( 0.2362204724409449064, 0.4091458600556404646, -0.1443569553805774397 ) ) ;
#50077=CARTESIAN_POINT ( 'NONE',  ( -0.1958661417322836995, 0.3392501089628017219, -1.584664985073177546 ) ) ;
#50079=CARTESIAN_POINT ( 'NONE',  ( 0.3917322834645670104, -0.1049643490035303411, -2.558398950131233196 ) ) ;
#50084=CARTESIAN_POINT ( 'NONE',  ( -0.1998031496062991907, -0.3460692066303959757, -1.010498687664042050 ) ) ;
#50086=CARTESIAN_POINT ( 'NONE',  ( 4.893765752498283308E-17, -0.3996062992125985480, -0.4704724409448819422 ) ) ;
#50088=CARTESIAN_POINT ( 'NONE',  ( -0.1998031496062991907, -0.3460692066303959757, -2.427821522309711266 ) ) ;
#50089=CARTESIAN_POINT ( 'NONE',  ( 0.3917322834645670104, 2.398668435337828261E-17, -1.620078740157480324 ) ) ;
#50093=CARTESIAN_POINT ( 'NONE',  ( 5.785732909357575061E-17, -0.4724409448818898682, -0.9429133858267716439 ) ) ;
#50096=CARTESIAN_POINT ( 'NONE',  ( 0.1058382717557500852, -0.3949938075777408852, -1.106955380577427706 ) ) ;
#50108=CARTESIAN_POINT ( 'NONE',  ( -9.787531504996566615E-17, 0.3996062992125985480, -1.809055118110236560 ) ) ;
#50122=CARTESIAN_POINT ( 'NONE',  ( -0.3392501089628019995, 0.1958661417322832277, -0.8982939632545933195 ) ) ;
#50133=AXIS2_PLACEMENT_3D ( 'NONE', #51983, #83161, #44412 ) ;
#50139=CARTESIAN_POINT ( 'NONE',  ( 0.1265901696524990572, -0.4724409448818897017, -0.5577427821522309426 ) ) ;
#50143=CARTESIAN_POINT ( 'NONE',  ( 0.3917322834645669549, 0.1049643490035304660, -2.006561679790026531 ) ) ;
#50146=CARTESIAN_POINT ( 'NONE',  ( 0.3458507752293908943, 0.3458507752293908943, -0.2952755905511811330 ) ) ;
#50147=CARTESIAN_POINT ( 'NONE',  ( -0.2891555358219908833, -0.2891555358219912164, -2.893700787401575436 ) ) ;
#50150=VECTOR ( 'NONE', #12263, 39.37007874015748143 ) ;
#50151=CARTESIAN_POINT ( 'NONE',  ( 0.3917322834645669549, 0.1049643490035304660, -1.534120734908136052 ) ) ;
#50153=CARTESIAN_POINT ( 'NONE',  ( 0.4724409448818896462, 0.1265901696524990294, -2.486876640419947382 ) ) ;
#50154=CARTESIAN_POINT ( 'NONE',  ( -0.3458507752293909498, 0.3458507752293908388, -0.8838582677165351953 ) ) ;
#50160=CARTESIAN_POINT ( 'NONE',  ( -9.594673741351310580E-17, 0.3917322834645669549, -0.5524741225383709153 ) ) ;
#50167=CARTESIAN_POINT ( 'NONE',  ( 0.3917322834645670659, -0.1049643490035303273, -2.155531126805461550 ) ) ;
#50175=CARTESIAN_POINT ( 'NONE',  ( -0.1958661417322834220, -0.3392501089628018884, -1.410104986876640654 ) ) ;
#50184=CARTESIAN_POINT ( 'NONE',  ( 0.1958661417322836440, -0.3392501089628017219, -2.761154855643044304 ) ) ;
#50191=CARTESIAN_POINT ( 'NONE',  ( 0.1049643490035303689, 0.3917322834645670104, -1.022965879265091749 ) ) ;
#50192=CARTESIAN_POINT ( 'NONE',  ( 0.3458507752293908943, -0.3458507752293908943, 0.1397637795275590289 ) ) ;
#50194=CARTESIAN_POINT ( 'NONE',  ( 0.3949938075777409963, 2.418639510665530743E-17, 0.1200787401574803376 ) ) ;
#50204=CARTESIAN_POINT ( 'NONE',  ( -0.3996062992125984925, -0.1070741851644056858, -0.4376640419947506744 ) ) ;
#50206=CARTESIAN_POINT ( 'NONE',  ( 4.797336870675656522E-17, -0.3917322834645670104, -0.3858267716535432879 ) ) ;
#50214=AXIS2_PLACEMENT_3D ( 'NONE', #80948, #55241, #80542 ) ;
#50223=CARTESIAN_POINT ( 'NONE',  ( -0.1958661417322833942, -0.3392501089628018884, -1.007237163550868120 ) ) ;
#50227=CARTESIAN_POINT ( 'NONE',  ( 0.1265901696524990294, -0.4724409448818896462, -2.524278215223096478 ) ) ;
#50247=CARTESIAN_POINT ( 'NONE',  ( -0.3460692066303957537, -0.1998031496062994405, -2.648950131233595684 ) ) ;
#50252=CARTESIAN_POINT ( 'NONE',  ( 0.3996062992125986590, -0.1070741851644053111, -2.316272965879265122 ) ) ;
#50253=CARTESIAN_POINT ( 'NONE',  ( -0.1058382717557503211, 0.3949938075777409408, -1.423884514435695969 ) ) ;
#50254=CARTESIAN_POINT ( 'NONE',  ( -0.3460692066303958092, -0.1998031496062994683, -2.887139107611548461 ) ) ;
#50257=CARTESIAN_POINT ( 'NONE',  ( -0.3392501089628017219, -0.1958661417322836718, -0.6745406824146981117 ) ) ;
#50261=CARTESIAN_POINT ( 'NONE',  ( 0.3420746716998660508, 0.1974969037888705814, -2.412729658792650778 ) ) ;
#50265=CARTESIAN_POINT ( 'NONE',  ( 0.1265901696524990294, -0.4724409448818896462, -2.919947506561679784 ) ) ;
#50266=CARTESIAN_POINT ( 'NONE',  ( -0.1998031496062991907, -0.3460692066303959757, -2.112860892388451539 ) ) ;
#50273=CARTESIAN_POINT ( 'NONE',  ( -0.3917322834645671215, 0.1049643490035301469, 0.04002624671916000382 ) ) ;
#50279=CARTESIAN_POINT ( 'NONE',  ( -0.3917322834645671215, 0.1049643490035301469, -0.5898950131233595684 ) ) ;
#50280=CARTESIAN_POINT ( 'NONE',  ( -0.3917322834645670104, -7.196005306013484475E-17, -1.606299212598425452 ) ) ;
#50281=CARTESIAN_POINT ( 'NONE',  ( -0.2867679344610364334, -0.2867679344610367109, -2.570866141732283339 ) ) ;
#50284=CARTESIAN_POINT ( 'NONE',  ( -0.3949938075777411628, 0.1058382717557497937, -2.552493438320210473 ) ) ;
#50288=CARTESIAN_POINT ( 'NONE',  ( -0.3460692066303958092, -0.1998031496062994683, -1.469816272965879245 ) ) ;
#50290=CARTESIAN_POINT ( 'NONE',  ( -0.1265901696524986964, -0.4724409448818899238, -0.7788713910761155823 ) ) ;
#50292=CARTESIAN_POINT ( 'NONE',  ( -0.4724409448818898682, -8.678599364036362592E-17, -1.929133858267716439 ) ) ;
#50293=CARTESIAN_POINT ( 'NONE',  ( -0.3917322834645670104, -7.196005306013484475E-17, -0.5964566929133858775 ) ) ;
#50303=CARTESIAN_POINT ( 'NONE',  ( 0.4724409448818898682, 2.892866454678787531E-17, -2.165354330708661568 ) ) ;
#50313=CARTESIAN_POINT ( 'NONE',  ( -0.1958661417322834497, -0.3392501089628018884, -0.3031302905173735573 ) ) ;
#50315=CARTESIAN_POINT ( 'NONE',  ( 0.3392501089628018884, -0.1958661417322834220, -0.6620734908136483021 ) ) ;
#50321=CARTESIAN_POINT ( 'NONE',  ( 0.3917322834645669549, 0.1049643490035304660, -2.793963254593175183 ) ) ;
#50324=CARTESIAN_POINT ( 'NONE',  ( -0.1265901696524986964, -0.4724409448818899238, -0.6213910761154856077 ) ) ;
#50332=DIRECTION ( 'NONE',  ( -0.000000000000000000, -0.000000000000000000, -1.000000000000000000 ) ) ;
#50337=CARTESIAN_POINT ( 'NONE',  ( -0.1070741851644051862, -0.3996062992125986590, -1.881233595800524849 ) ) ;
#50343=CARTESIAN_POINT ( 'NONE',  ( 0.2362204724409451007, -0.4091458600556402980, -0.09186351706036745279 ) ) ;
#50345=CARTESIAN_POINT ( 'NONE',  ( 0.1070741851644054637, -0.3996062992125984925, -0.7919947506561678674 ) ) ;
#50346=CARTESIAN_POINT ( 'NONE',  ( 0.1070741851644053527, 0.3996062992125986590, -0.9383202099737533164 ) ) ;
#50347=CARTESIAN_POINT ( 'NONE',  ( -0.2891555358219908833, -0.2891555358219912164, -0.2165354330708662567 ) ) ;
#50353=CARTESIAN_POINT ( 'NONE',  ( -0.3949938075777411073, 0.1058382717557497660, -1.211942257217847763 ) ) ;
#50359=CARTESIAN_POINT ( 'NONE',  ( -0.1265901696524986964, -0.4724409448818899238, -1.804461942257217677 ) ) ;
#50360=CARTESIAN_POINT ( 'NONE',  ( -0.3996062992125985480, -0.1070741851644057135, -2.565616797900262647 ) ) ;
#50373=CARTESIAN_POINT ( 'NONE',  ( -0.1958661417322834220, -0.3392501089628018884, -1.475065616797900381 ) ) ;
#50375=ORIENTED_EDGE ( 'NONE', *, *, #39222, .F. ) ;
#50376=CARTESIAN_POINT ( 'NONE',  ( 4.837279021331060870E-17, -0.3949938075777409963, -1.496062992125984037 ) ) ;
#50381=CARTESIAN_POINT ( 'NONE',  ( 0.3996062992125986035, 2.446882876249141962E-17, -0.1181102362204724671 ) ) ;
#50389=FACE_OUTER_BOUND ( 'NONE', #47576, .T. ) ;
#50395=CARTESIAN_POINT ( 'NONE',  ( -0.3996062992125987146, 0.1070741851644051862, -2.080052493438320216 ) ) ;
#50398=CARTESIAN_POINT ( 'NONE',  ( 0.1998031496062994128, -0.3460692066303957537, -1.743438320209973469 ) ) ;
#50402=CARTESIAN_POINT ( 'NONE',  ( 0.4724409448818898682, 2.892866454678787531E-17, -0.9055118110236221041 ) ) ;
#50404=CARTESIAN_POINT ( 'NONE',  ( -0.1049643490035307020, 0.3917322834645669549, -2.768372703412072866 ) ) ;
#50406=CARTESIAN_POINT ( 'NONE',  ( -0.1049643490035307020, 0.3917322834645669549, -1.980971128608923992 ) ) ;
#50410=CARTESIAN_POINT ( 'NONE',  ( 0.1070741851644054776, -0.3996062992125984925, 0.1528871391076114805 ) ) ;
#50412=CARTESIAN_POINT ( 'NONE',  ( -0.3420746716998660508, -0.1974969037888706924, -2.333989501312335957 ) ) ;
#50432=CARTESIAN_POINT ( 'NONE',  ( -0.1998031496062991630, -0.3460692066303959202, -0.9297900262467192478 ) ) ;
#50433=CARTESIAN_POINT ( 'NONE',  ( -0.3917322834645670104, -7.196005306013484475E-17, -2.328740157480315265 ) ) ;
#50449=CARTESIAN_POINT ( 'NONE',  ( 0.3917322834645670104, -0.1049643490035303411, -1.928477690288713742 ) ) ;
#50450=CARTESIAN_POINT ( 'NONE',  ( 0.1308238996069422677, 0.3698506310978945111, -1.220472440944881942 ) ) ;
#50457=CARTESIAN_POINT ( 'NONE',  ( -0.1998031496062994683, 0.3460692066303958092, -0.9580052493438320216 ) ) ;
#50459=CARTESIAN_POINT ( 'NONE',  ( 0.3392501089628018329, 0.1958661417322835607, -2.800524934383201714 ) ) ;
#50471=CARTESIAN_POINT ( 'NONE',  ( -0.3917322834645669549, -0.1049643490035306603, -0.1955380577427821009 ) ) ;
#50474=CARTESIAN_POINT ( 'NONE',  ( -0.2891555358219911054, 0.2891555358219909388, -0.01968503937007880233 ) ) ;
#50481=CARTESIAN_POINT ( 'NONE',  ( -0.3392501089628019995, 0.1958661417322831999, -1.755268659613860249 ) ) ;
#50483=CARTESIAN_POINT ( 'NONE',  ( 0.1049643490035304938, -0.3917322834645669549, -2.532152230971127960 ) ) ;
#50489=CARTESIAN_POINT ( 'NONE',  ( -0.1070741851644051862, -0.3996062992125987146, -0.8595800524934383846 ) ) ;
#50491=CARTESIAN_POINT ( 'NONE',  ( 0.1998031496062994128, -0.3460692066303957537, -0.1686351706036745557 ) ) ;
#50493=CARTESIAN_POINT ( 'NONE',  ( 0.3996062992125986035, 2.446882876249141962E-17, -2.480314960629921295 ) ) ;
#50494=CARTESIAN_POINT ( 'NONE',  ( -0.3917322834645670104, -7.196005306013484475E-17, -1.856299212598425230 ) ) ;
#50499=CARTESIAN_POINT ( 'NONE',  ( 0.4091458600556403535, 0.2362204724409449896, -1.467847769028871596 ) ) ;
#50502=CARTESIAN_POINT ( 'NONE',  ( 0.3949938075777409963, 2.418639510665530743E-17, -1.139763779527559251 ) ) ;
#50512=CARTESIAN_POINT ( 'NONE',  ( -0.3996062992125985480, -7.340648628747423112E-17, -1.848425196850393748 ) ) ;
#50514=ADVANCED_FACE ( 'NONE', ( #23068 ), #51459, .T. ) ;
#50528=CARTESIAN_POINT ( 'NONE',  ( 0.3917322834645669549, 0.1049643490035304660, -0.8392388451443569819 ) ) ;
#50533=FACE_BOUND ( 'NONE', #21002, .T. ) ;
#50538=CARTESIAN_POINT ( 'NONE',  ( 0.2362204724409451007, -0.4091458600556402980, -2.611548556430446144 ) ) ;
#50545=CARTESIAN_POINT ( 'NONE',  ( -0.4724409448818895907, -0.01881781417526964470, -1.219479340321617311 ) ) ;
#50549=CARTESIAN_POINT ( 'NONE',  ( 0.2867679344610366554, -0.2867679344610365444, -1.980314960629921073 ) ) ;
#50553=CARTESIAN_POINT ( 'NONE',  ( -0.3458507752293909498, 0.3458507752293907833, -0.1771653543307086520 ) ) ;
#50554=CARTESIAN_POINT ( 'NONE',  ( 0.3949938075777409408, 0.1058382717557500574, -2.644356955380577912 ) ) ;
#50557=CARTESIAN_POINT ( 'NONE',  ( 0.3917322834645670104, -0.1049643490035303411, -1.206036745406823707 ) ) ;
#50559=CARTESIAN_POINT ( 'NONE',  ( 0.01966910102760669257, 0.3928700489057007639, -2.755905511811024944 ) ) ;
#50560=CARTESIAN_POINT ( 'NONE',  ( -0.1265901696524993347, 0.4724409448818896462, -0.8707349081364829102 ) ) ;
#50566=CARTESIAN_POINT ( 'NONE',  ( -0.3917322834645670659, 0.1049643490035301607, -0.9002431514097621879 ) ) ;
#50573=CARTESIAN_POINT ( 'NONE',  ( -0.1049643490035307158, 0.3917322834645670104, -2.208024565125671135 ) ) ;
#50580=CARTESIAN_POINT ( 'NONE',  ( 0.2867679344610365999, -0.2867679344610365444, -1.600393700787401619 ) ) ;
#50587=CARTESIAN_POINT ( 'NONE',  ( 0.4724409448818898682, 2.892866454678787531E-17, -0.9822834645669291653 ) ) ;
#50589=CARTESIAN_POINT ( 'NONE',  ( -9.594673741351313045E-17, 0.3917322834645670104, -2.669291338582676865 ) ) ;
#50591=ORIENTED_EDGE ( 'NONE', *, *, #26304, .T. ) ;
#50596=CARTESIAN_POINT ( 'NONE',  ( 0.4091458600556404646, -0.2362204724409448231, -0.4199475065616797842 ) ) ;
#50597=CARTESIAN_POINT ( 'NONE',  ( 0.3392501089628018329, 0.1958661417322835607, -1.160761154855643129 ) ) ;
#50598=CARTESIAN_POINT ( 'NONE',  ( -0.4091458600556405756, 0.2362204724409446288, 0.2119422572178477626 ) ) ;
#50600=CARTESIAN_POINT ( 'NONE',  ( -0.3460692066303960313, 0.1998031496062989965, -2.780183727034120977 ) ) ;
#50610=CARTESIAN_POINT ( 'NONE',  ( 0.3460692066303959202, -0.1998031496062991630, -0.6541994750656167090 ) ) ;
#50613=CARTESIAN_POINT ( 'NONE',  ( 0.3917322834645670104, -0.1049643490035303411, -0.4186351706036745557 ) ) ;
#50616=DIRECTION ( 'NONE',  ( 1.000000000000000000, 0.000000000000000000, 0.000000000000000000 ) ) ;
#50622=CARTESIAN_POINT ( 'NONE',  ( 0.2017716535433070613, -0.2017716535433070890, -0.3937007874015748254 ) ) ;
#50628=CARTESIAN_POINT ( 'NONE',  ( 0.2867679344610366554, -0.2867679344610365999, -1.040045562500999443 ) ) ;
#50632=CARTESIAN_POINT ( 'NONE',  ( -1.157146581871515012E-16, 0.4724409448818898682, -2.438976377952756014 ) ) ;
#50646=EDGE_CURVE ( 'NONE', #57846, #57445, #7478, .T. ) ;
#50654=CARTESIAN_POINT ( 'NONE',  ( 0.1070741851644053666, 0.3996062992125986035, -0.3083989501312335846 ) ) ;
#50655=CARTESIAN_POINT ( 'NONE',  ( 0.2925321140481932369, -0.2925321140481931814, -2.537401574803149984 ) ) ;
#50662=CARTESIAN_POINT ( 'NONE',  ( 0.1070741851644053527, 0.3996062992125986590, -2.198162729658792447 ) ) ;
#50663=CARTESIAN_POINT ( 'NONE',  ( -0.2891555358219911054, 0.2891555358219909388, -1.594488188976378007 ) ) ;
#50666=CARTESIAN_POINT ( 'NONE',  ( -0.3917322834645670104, -7.196005306013484475E-17, -0.6614173228346454936 ) ) ;
#50669=CARTESIAN_POINT ( 'NONE',  ( -0.1058382717557497660, -0.3949938075777411073, -2.511154855643044748 ) ) ;
#50675=CARTESIAN_POINT ( 'NONE',  ( -0.1070741851644056997, 0.3996062992125986035, -2.053805774278214979 ) ) ;
#50682=CARTESIAN_POINT ( 'NONE',  ( -0.3917322834645670104, -7.196005306013484475E-17, 0.03346456692913377107 ) ) ;
#50689=CARTESIAN_POINT ( 'NONE',  ( -0.1958661417322836718, 0.3392501089628017219, -0.7276902887139108378 ) ) ;
#50690=CARTESIAN_POINT ( 'NONE',  ( 0.1958661417322834775, 0.3392501089628018884, -1.396325459317585338 ) ) ;
#50691=CARTESIAN_POINT ( 'NONE',  ( -0.3392501089628017219, -0.1958661417322836718, -2.564304461942256808 ) ) ;
#50694=CARTESIAN_POINT ( 'NONE',  ( -0.3996062992125986035, -0.1070741851644056997, 0.1115485564304461580 ) ) ;
#50698=CARTESIAN_POINT ( 'NONE',  ( 0.2925321140481932369, 0.2925321140481932369, -1.240157480314960647 ) ) ;
#50703=CARTESIAN_POINT ( 'NONE',  ( 0.1958661417322834775, 0.3392501089628018884, -0.3864829396325459854 ) ) ;
#50712=CARTESIAN_POINT ( 'NONE',  ( -0.4724409448818895907, -0.1265901696524993070, -2.250656167979002920 ) ) ;
#50718=AXIS2_PLACEMENT_3D ( 'NONE', #49651, #5454, #82483 ) ;
#50724=CARTESIAN_POINT ( 'NONE',  ( -0.2867679344610364334, -0.2867679344610368219, -0.2965686107273473038 ) ) ;
#50726=CARTESIAN_POINT ( 'NONE',  ( -0.2867679344610364334, -0.2867679344610367109, -0.9311023622047244208 ) ) ;
#50731=CARTESIAN_POINT ( 'NONE',  ( 0.1049643490035304938, -0.3917322834645669549, -2.912073490813647858 ) ) ;
#50734=CARTESIAN_POINT ( 'NONE',  ( -0.1265901696524986964, -0.4724409448818899238, -1.408792650918635259 ) ) ;
#50747=CARTESIAN_POINT ( 'NONE',  ( 0.3996062992125984925, 0.1070741851644054637, -2.248687664041994605 ) ) ;
#50751=CARTESIAN_POINT ( 'NONE',  ( -0.3460692066303960313, 0.1998031496062989965, -1.205380577427821454 ) ) ;
#50755=CARTESIAN_POINT ( 'NONE',  ( 0.4091458600556404646, -0.2362204724409448231, -0.1049868766404199460 ) ) ;
#50757=CARTESIAN_POINT ( 'NONE',  ( -0.3460692066303957537, -0.1998031496062994405, -0.6017060367454067915 ) ) ;
#50758=CARTESIAN_POINT ( 'NONE',  ( -0.3460692066303960868, 0.1998031496062990242, -1.128608923884514503 ) ) ;
#50759=CARTESIAN_POINT ( 'NONE',  ( 0.3420746716998659953, 0.1974969037888705536, -0.4461942257217848540 ) ) ;
#50765=CARTESIAN_POINT ( 'NONE',  ( 0.3420746716998660508, -0.1974969037888704149, -1.441601049868766804 ) ) ;
#50770=CARTESIAN_POINT ( 'NONE',  ( 0.1265901696524990294, -0.4724409448818896462, -1.660104986876640210 ) ) ;
#50772=CARTESIAN_POINT ( 'NONE',  ( 0.2925321140481932369, -0.2925321140481931814, -2.618110236220472675 ) ) ;
#50784=CARTESIAN_POINT ( 'NONE',  ( -0.3917322834645670104, -7.196005306013484475E-17, -1.291338582677165503 ) ) ;
#50787=CARTESIAN_POINT ( 'NONE',  ( 0.3420746716998660508, -0.1974969037888703871, -1.837270341207348556 ) ) ;
#50792=CARTESIAN_POINT ( 'NONE',  ( -0.1070741851644056997, 0.3996062992125986035, -0.006561679790026256169 ) ) ;
#50799=CARTESIAN_POINT ( 'NONE',  ( -0.3392501089628017219, -0.1958661417322836718, 0.1778215223097112108 ) ) ;
#50806=CARTESIAN_POINT ( 'NONE',  ( -0.1998031496062991630, -0.3460692066303959202, -1.559711286089238591 ) ) ;
#50811=CARTESIAN_POINT ( 'NONE',  ( -0.1265901696524993347, 0.4724409448818895907, -0.9514435695538056015 ) ) ;
#50813=CARTESIAN_POINT ( 'NONE',  ( 0.2867679344610365999, 0.2867679344610365999, -2.742125984251967630 ) ) ;
#50815=CARTESIAN_POINT ( 'NONE',  ( 0.3392501089628018329, 0.1958661417322835607, -2.105643044619422533 ) ) ;
#50819=CARTESIAN_POINT ( 'NONE',  ( 0.4091458600556404646, -0.2362204724409448231, -2.701443569553806157 ) ) ;
#50822=CARTESIAN_POINT ( 'NONE',  ( 4.837279021331061486E-17, -0.3949938075777409963, -2.045275590551181022 ) ) ;
#50832=CARTESIAN_POINT ( 'NONE',  ( 0.4724409448818896462, 0.1265901696524990294, 0.1135170603674540563 ) ) ;
#50845=CARTESIAN_POINT ( 'NONE',  ( -0.3996062992125986590, 0.1070741851644051723, -0.7395013123359580609 ) ) ;
#50846=CARTESIAN_POINT ( 'NONE',  ( 0.2867679344610365999, -0.2867679344610365444, -2.230314960629921295 ) ) ;
#50855=CARTESIAN_POINT ( 'NONE',  ( 0.4091458600556404646, -0.2362204724409448231, -0.7349081364829396223 ) ) ;
#50856=CARTESIAN_POINT ( 'NONE',  ( 0.3917322834645670104, 0.1049643490035304660, -2.168654486385513724 ) ) ;
#50862=CARTESIAN_POINT ( 'NONE',  ( -0.2867679344610364334, -0.2867679344610367109, -2.033464566929133355 ) ) ;
#50863=CARTESIAN_POINT ( 'NONE',  ( -0.3078094465263064294, 0.2432155562301229479, -1.220472440944882164 ) ) ;
#50867=CARTESIAN_POINT ( 'NONE',  ( 4.893765752498283308E-17, -0.3996062992125985480, -2.675196850393700920 ) ) ;
#50869=CARTESIAN_POINT ( 'NONE',  ( 0.3460692066303959757, -0.1998031496062991907, -1.522309711286089273 ) ) ;
#50871=CARTESIAN_POINT ( 'NONE',  ( -0.2867679344610365444, -0.2867679344610367664, 0.1016867209635676783 ) ) ;
#50883=CARTESIAN_POINT ( 'NONE',  ( -0.2867679344610364334, -0.2867679344610367109, -0.05118110236220468900 ) ) ;
#50886=CARTESIAN_POINT ( 'NONE',  ( -0.3420746716998659953, -0.1974969037888706647, -0.05249343832021002854 ) ) ;
#50887=VERTEX_POINT ( 'NONE', #49164 ) ;
#50889=CARTESIAN_POINT ( 'NONE',  ( 0.4724409448818898682, 0.000000000000000000, -2.755905511811024056 ) ) ;
#50893=CARTESIAN_POINT ( 'NONE',  ( 0.3917322834645670659, -0.1049643490035303273, -1.683090181923571294 ) ) ;
#50895=CARTESIAN_POINT ( 'NONE',  ( 0.3392501089628018329, 0.1958661417322835607, -2.735564304461941987 ) ) ;
#50899=CARTESIAN_POINT ( 'NONE',  ( -0.3996062992125986035, -7.340648628747425578E-17, -0.8267716535433070613 ) ) ;
#50901=CARTESIAN_POINT ( 'NONE',  ( -0.1998031496062991630, -0.3460692066303959202, -0.2998687664041995160 ) ) ;
#50902=CARTESIAN_POINT ( 'NONE',  ( -9.787531504996566615E-17, 0.3996062992125985480, -0.07677165354330711677 ) ) ;
#50904=CARTESIAN_POINT ( 'NONE',  ( 0.1998031496062994405, -0.3460692066303958092, -2.611548556430446144 ) ) ;
#50905=CARTESIAN_POINT ( 'NONE',  ( 0.3917322834645669549, 0.1049643490035304660, -1.784120734908136274 ) ) ;
#50910=CARTESIAN_POINT ( 'NONE',  ( -0.4091458600556405756, 0.2362204724409446288, -1.520341207349081181 ) ) ;
#50914=CARTESIAN_POINT ( 'NONE',  ( -0.3420746716998660508, -0.1974969037888706924, -1.074146981627296826 ) ) ;
#50923=CARTESIAN_POINT ( 'NONE',  ( -0.3996062992125986590, 0.1070741851644051723, -1.999343832020997525 ) ) ;
#50940=CARTESIAN_POINT ( 'NONE',  ( 0.1958661417322836440, -0.3392501089628017219, -0.8064304461942258806 ) ) ;
#50959=CARTESIAN_POINT ( 'NONE',  ( 0.1958661417322834775, 0.3392501089628018884, -2.026246719160105236 ) ) ;
#50962=CARTESIAN_POINT ( 'NONE',  ( -0.1265901696524993347, 0.4724409448818895907, -0.3215223097112860362 ) ) ;
#50963=CARTESIAN_POINT ( 'NONE',  ( 0.3949938075777409963, 2.418639510665530435E-17, -2.795275590551181022 ) ) ;
#50966=CARTESIAN_POINT ( 'NONE',  ( 0.2867679344610365999, -0.2867679344610365444, -1.350393700787401619 ) ) ;
#50968=CARTESIAN_POINT ( 'NONE',  ( -0.02707642104390568794, 0.3965571307776177834, -2.755905511811025388 ) ) ;
#50975=CARTESIAN_POINT ( 'NONE',  ( -0.1049643490035306742, 0.3917322834645668994, -0.7165161172890270880 ) ) ;
#50982=CARTESIAN_POINT ( 'NONE',  ( 0.3392501089628018329, 0.1958661417322835607, -2.175216166175539811 ) ) ;
#50989=CARTESIAN_POINT ( 'NONE',  ( -0.2867679344610365999, 0.2867679344610364889, -1.364173228346456268 ) ) ;
#50998=CARTESIAN_POINT ( 'NONE',  ( 4.797336870675656522E-17, -0.3917322834645670104, -2.905511811023621771 ) ) ;
#51004=DIRECTION ( 'NONE',  ( -0.000000000000000000, -0.000000000000000000, 1.000000000000000000 ) ) ;
#51005=CARTESIAN_POINT ( 'NONE',  ( 0.3917322834645670104, 2.398668435337828261E-17, -1.305118110236220375 ) ) ;
#51006=CARTESIAN_POINT ( 'NONE',  ( -0.4091458600556402980, -0.2362204724409451284, -0.2867454068241469534 ) ) ;
#51009=CARTESIAN_POINT ( 'NONE',  ( -0.3420746716998660508, -0.1974969037888706924, 0.1856955380577428039 ) ) ;
#51014=CARTESIAN_POINT ( 'NONE',  ( -0.3949938075777411073, 0.1058382717557497660, -0.1095800524934383707 ) ) ;
#51022=CARTESIAN_POINT ( 'NONE',  ( -9.787531504996566615E-17, 0.3996062992125985480, -0.3917322834645669549 ) ) ;
#51024=CARTESIAN_POINT ( 'NONE',  ( 0.2867679344610365999, 0.2867679344610365999, -0.2874015748031494843 ) ) ;
#51037=CARTESIAN_POINT ( 'NONE',  ( -0.1049643490035302301, -0.3917322834645671770, -0.6988382134196345907 ) ) ;
#51041=CARTESIAN_POINT ( 'NONE',  ( 5.785732909357575061E-17, -0.4724409448818898682, -2.360236220472441193 ) ) ;
#51060=CARTESIAN_POINT ( 'NONE',  ( -0.1998031496062994683, 0.3460692066303958092, -0.3280839895013123453 ) ) ;
#51061=CARTESIAN_POINT ( 'NONE',  ( 0.3996062992125984925, 0.1070741851644054637, -2.563648293963254776 ) ) ;
#51066=CARTESIAN_POINT ( 'NONE',  ( -0.2925321140481932924, 0.2925321140481931814, -2.066929133858267154 ) ) ;
#51067=CARTESIAN_POINT ( 'NONE',  ( 0.1974969037888704704, 0.3420746716998660508, -1.561679790026246684 ) ) ;
#51068=CARTESIAN_POINT ( 'NONE',  ( 0.1998031496062994405, -0.3460692066303958092, -2.769028871391076230 ) ) ;
#51069=CARTESIAN_POINT ( 'NONE',  ( 0.3458507752293908943, 0.3458507752293908943, -2.500000000000000000 ) ) ;
#51070=CARTESIAN_POINT ( 'NONE',  ( -0.1049643490035301885, -0.3917322834645671215, -0.8517060367454067915 ) ) ;
#51073=CARTESIAN_POINT ( 'NONE',  ( 0.1974969037888706092, -0.3420746716998660508, -2.373359580052493811 ) ) ;
#51078=CARTESIAN_POINT ( 'NONE',  ( -0.2362204724409447953, -0.4091458600556404646, -2.900262467191600635 ) ) ;
#51079=CARTESIAN_POINT ( 'NONE',  ( 0.3460692066303959202, 0.1998031496062993295, -2.020997375328084100 ) ) ;
#51086=CARTESIAN_POINT ( 'NONE',  ( -0.1958661417322836718, 0.3392501089628017219, -0.09776902887139117537 ) ) ;
#51094=CARTESIAN_POINT ( 'NONE',  ( 0.3392501089628018884, -0.1958661417322834220, -0.5045931758530184386 ) ) ;
#51095=CARTESIAN_POINT ( 'NONE',  ( -0.2867679344610364334, -0.2867679344610367109, -1.625984251968503491 ) ) ;
#51096=( BOUNDED_CURVE ( )  B_SPLINE_CURVE ( 2, ( #23997, #69031, #11382, #37039, #50073, #37453, #29078, #22763, #38272, #18918, #19333, #52138, #13448 ),
 .UNSPECIFIED., .F., .F. ) 
 B_SPLINE_CURVE_WITH_KNOTS ( ( 3, 2, 2, 2, 2, 2, 3 ),
 ( 0.08750000000000000833, 0.09166666666666667407, 0.09583333333333335369, 0.1000000000000000056, 0.1041666666666666713, 0.1083333333333333370, 0.1125000000000000028 ),
 .UNSPECIFIED. ) 
 CURVE ( )  GEOMETRIC_REPRESENTATION_ITEM ( )  RATIONAL_B_SPLINE_CURVE ( ( 0.9999999999999998890, 0.9659258262890684232, 1.000000000000000000, 0.9659258262890683122, 1.000000000000000000, 0.9659258262890683122, 1.000000000000000000, 0.9659258262890683122, 1.000000000000000000, 0.9659258262890683122, 1.000000000000000000, 0.9659258262890683122, 1.000000000000000000 ) ) 
 REPRESENTATION_ITEM ( '' )  );
#51097=CARTESIAN_POINT ( 'NONE',  ( 0.3917322834645670104, 2.398668435337828261E-17, -2.629921259842519898 ) ) ;
#51099=CARTESIAN_POINT ( 'NONE',  ( 0.3996062992125986035, 0.1070741851644054776, -0.1246719160104987068 ) ) ;
#51103=CARTESIAN_POINT ( 'NONE',  ( -0.1998031496062991907, -0.3460692066303959757, -1.325459317585301777 ) ) ;
#51105=CARTESIAN_POINT ( 'NONE',  ( -0.4724409448818898682, -8.678599364036362592E-17, -2.478346456692913868 ) ) ;
#51107=CARTESIAN_POINT ( 'NONE',  ( 0.3857547143408419088, -0.07128922432405931930, -1.929133858267716661 ) ) ;
#51108=CARTESIAN_POINT ( 'NONE',  ( 0.2867679344610365999, 0.2867679344610365999, -0.6948818897637795144 ) ) ;
#51118=CARTESIAN_POINT ( 'NONE',  ( -0.2362204724409451284, 0.4091458600556402425, -2.060367454068241511 ) ) ;
#51119=CARTESIAN_POINT ( 'NONE',  ( 0.4091458600556403535, 0.2362204724409449896, -2.650918635170603554 ) ) ;
#51125=CARTESIAN_POINT ( 'NONE',  ( 0.4091458600556404646, -0.2362204724409448231, -2.543963254593176071 ) ) ;
#51126=CARTESIAN_POINT ( 'NONE',  ( 0.3458507752293908943, -0.3458507752293908943, -2.694881889763779625 ) ) ;
#51129=CARTESIAN_POINT ( 'NONE',  ( 0.1049643490035303689, 0.3917322834645668994, -1.018353387630234419 ) ) ;
#51131=CARTESIAN_POINT ( 'NONE',  ( 0.3917322834645670104, -0.1049643490035303273, -0.6686351706036747222 ) ) ;
#51136=CARTESIAN_POINT ( 'NONE',  ( -0.3392501089628017219, -0.1958661417322836718, -2.564304461942256808 ) ) ;
#51140=CARTESIAN_POINT ( 'NONE',  ( 0.4724409448818898682, 2.892866454678787531E-17, -1.139763779527559029 ) ) ;
#51147=FACE_OUTER_BOUND ( 'NONE', #56894, .T. ) ;
#51151=ORIENTED_EDGE ( 'NONE', *, *, #35152, .F. ) ;
#51152=CARTESIAN_POINT ( 'NONE',  ( -0.3996062992125986590, 0.1070741851644051723, -2.314304461942256808 ) ) ;
#51156=CARTESIAN_POINT ( 'NONE',  ( -0.3996062992125986590, 0.1070741851644051723, -1.526902887139107490 ) ) ;
#51160=CARTESIAN_POINT ( 'NONE',  ( -0.4091458600556402980, -0.2362204724409451284, -0.05249343832020997302 ) ) ;
#51162=CARTESIAN_POINT ( 'NONE',  ( 0.3996062992125985480, 2.446882876249141654E-17, -0.5098425196850393526 ) ) ;
#51163=CARTESIAN_POINT ( 'NONE',  ( 0.3996062992125986035, 2.446882876249141962E-17, -0.9055118110236221041 ) ) ;
#51164=CARTESIAN_POINT ( 'NONE',  ( 0.1058382717557500713, -0.3949938075777409408, -0.2427821522309712154 ) ) ;
#51171=CARTESIAN_POINT ( 'NONE',  ( 0.3420746716998660508, 0.1974969037888705814, -1.310367454068241511 ) ) ;
#51176=CARTESIAN_POINT ( 'NONE',  ( 0.4724409448818897572, -0.1265901696524988906, -1.528871391076114916 ) ) ;
#51184=CARTESIAN_POINT ( 'NONE',  ( -0.3917322834645669549, -7.196005306013483243E-17, -1.851686720963567456 ) ) ;
#51185=CARTESIAN_POINT ( 'NONE',  ( -0.3460692066303960313, 0.1998031496062989965, -2.780183727034120977 ) ) ;
#51191=CARTESIAN_POINT ( 'NONE',  ( 0.3917322834645669549, 0.1049643490035304660, -1.376640419947506189 ) ) ;
#51193=ORIENTED_EDGE ( 'NONE', *, *, #61945, .T. ) ;
#51194=CARTESIAN_POINT ( 'NONE',  ( -9.674558042662121740E-17, 0.3949938075777409963, -1.732283464566929165 ) ) ;
#51199=CARTESIAN_POINT ( 'NONE',  ( 4.893765752498283924E-17, -0.3996062992125986035, -0.2362204724409449064 ) ) ;
#51207=CARTESIAN_POINT ( 'NONE',  ( 0.3917322834645669549, 0.1049643490035304660, -0.2093175853018373611 ) ) ;
#51215=CARTESIAN_POINT ( 'NONE',  ( -0.3996062992125985480, -7.340648628747423112E-17, -2.005905511811023612 ) ) ;
#51220=CARTESIAN_POINT ( 'NONE',  ( -0.4091458600556405756, 0.2362204724409446288, -0.9711286089238845287 ) ) ;
#51222=CARTESIAN_POINT ( 'NONE',  ( 0.3917322834645670104, -0.1049643490035303411, 0.05380577427821527092 ) ) ;
#51223=CARTESIAN_POINT ( 'NONE',  ( -0.3917322834645670104, -7.196005306013484475E-17, -2.013779527559055094 ) ) ;
#51227=CARTESIAN_POINT ( 'NONE',  ( 0.1265901696524989462, 0.4724409448818897572, -2.589895013123359568 ) ) ;
#51231=CARTESIAN_POINT ( 'NONE',  ( -0.1974969037888704149, -0.3420746716998661063, -2.504593175853018661 ) ) ;
#51238=CARTESIAN_POINT ( 'NONE',  ( -0.3392501089628017219, -0.1958661417322836718, -1.619422572178477848 ) ) ;
#51244=CARTESIAN_POINT ( 'NONE',  ( 0.4724409448818898682, 2.892866454678787531E-17, -0.1181102362204724532 ) ) ;
#51252=CARTESIAN_POINT ( 'NONE',  ( -0.1070741851644051862, -0.3996062992125986590, -1.251312335958005173 ) ) ;
#51253=CARTESIAN_POINT ( 'NONE',  ( 0.1049643490035303689, 0.3917322834645670104, -2.125328083989501682 ) ) ;
#51264=CARTESIAN_POINT ( 'NONE',  ( 0.3917322834645670659, 2.398668435337828261E-17, -2.004612491634857552 ) ) ;
#51270=CARTESIAN_POINT ( 'NONE',  ( -0.3917322834645671215, 0.1049643490035301469, -1.849737532808399143 ) ) ;
#51271=CARTESIAN_POINT ( 'NONE',  ( -0.3428707098288043542, 0.1906283239483336500, -1.220472440944882386 ) ) ;
#51275=CARTESIAN_POINT ( 'NONE',  ( 0.3460692066303959202, -0.1998031496062991630, -2.701443569553806157 ) ) ;
#51277=CARTESIAN_POINT ( 'NONE',  ( -0.1070741851644056997, 0.3996062992125986035, -1.266404199475065440 ) ) ;
#51278=ORIENTED_EDGE ( 'NONE', *, *, #61945, .F. ) ;
#51279=CARTESIAN_POINT ( 'NONE',  ( 0.1049643490035304938, -0.3917322834645669549, -2.912073490813647858 ) ) ;
#51293=CARTESIAN_POINT ( 'NONE',  ( -0.3917322834645670104, -7.196005306013484475E-17, -0.1889763779527558474 ) ) ;
#51296=CARTESIAN_POINT ( 'NONE',  ( 0.2891555358219910499, -0.2891555358219909944, -0.4133858267716535861 ) ) ;
#51299=CARTESIAN_POINT ( 'NONE',  ( 0.000000000000000000, 0.000000000000000000, -2.755905511811024056 ) ) ;
#51304=CARTESIAN_POINT ( 'NONE',  ( 4.797336870675656522E-17, -0.3917322834645670659, -1.650281782973440192 ) ) ;
#51310=CARTESIAN_POINT ( 'NONE',  ( -0.1070741851644056997, 0.3996062992125986035, -1.423884514435695525 ) ) ;
#51312=CARTESIAN_POINT ( 'NONE',  ( -0.1998031496062994405, 0.3460692066303957537, -0.8772965879265091083 ) ) ;
#51313=CARTESIAN_POINT ( 'NONE',  ( -0.3996062992125985480, -7.340648628747423112E-17, 0.04133858267716532947 ) ) ;
#51315=CARTESIAN_POINT ( 'NONE',  ( -0.1998031496062991907, -0.3460692066303959757, -2.585301837270341352 ) ) ;
#51316=CARTESIAN_POINT ( 'NONE',  ( 4.797336870675656522E-17, -0.3917322834645670104, -1.895669291338582640 ) ) ;
#51322=CARTESIAN_POINT ( 'NONE',  ( -0.3458507752293906723, -0.3458507752293910609, -1.395669291338582196 ) ) ;
#51325=CARTESIAN_POINT ( 'NONE',  ( 0.2891555358219910499, -0.2891555358219909944, -0.8051181102362204856 ) ) ;
#51334=CARTESIAN_POINT ( 'NONE',  ( -0.1998031496062991630, -0.3460692066303959202, -2.189632545931758489 ) ) ;
#51336=CARTESIAN_POINT ( 'NONE',  ( -0.3392501089628018329, -0.1958661417322836440, -1.707329765582990211 ) ) ;
#51348=CARTESIAN_POINT ( 'NONE',  ( 0.2925321140481932369, 0.2925321140481932369, -0.05708661417322836301 ) ) ;
#51350=CARTESIAN_POINT ( 'NONE',  ( 0.3917322834645670104, 2.398668435337828261E-17, -0.9901574803149607584 ) ) ;
#51370=CARTESIAN_POINT ( 'NONE',  ( 0.3917322834645670104, -0.1049643490035303273, -2.623359580052492923 ) ) ;
#51373=CARTESIAN_POINT ( 'NONE',  ( 0.2362204724409449064, 0.4091458600556404646, -0.9317585301837270073 ) ) ;
#51374=CARTESIAN_POINT ( 'NONE',  ( -0.1070741851644056997, 0.3996062992125986035, -0.006561679790026264843 ) ) ;
#51377=CARTESIAN_POINT ( 'NONE',  ( -0.2867679344610365999, 0.2867679344610364889, -1.901574803149606252 ) ) ;
#51380=CARTESIAN_POINT ( 'NONE',  ( 0.1265901696524990294, -0.4724409448818896462, -2.762467191601049255 ) ) ;
#51387=CARTESIAN_POINT ( 'NONE',  ( 0.1958661417322836162, -0.3392501089628018329, -0.9592982695199985255 ) ) ;
#51395=CARTESIAN_POINT ( 'NONE',  ( -0.3392501089628017219, -0.1958661417322836995, -2.411436638616484718 ) ) ;
#51402=AXIS2_PLACEMENT_3D ( 'NONE', #60876, #3228, #49070 ) ;
#51405=CARTESIAN_POINT ( 'NONE',  ( -0.2867679344610365999, 0.2867679344610364889, -1.206692913385826627 ) ) ;
#51420=CARTESIAN_POINT ( 'NONE',  ( 0.1049643490035304938, -0.3917322834645669549, -1.114829396325459410 ) ) ;
#51421=CARTESIAN_POINT ( 'NONE',  ( -0.1265901696524986964, -0.4724409448818899238, -0.3064304461942257141 ) ) ;
#51424=CARTESIAN_POINT ( 'NONE',  ( -0.1974969037888706924, 0.3420746716998658843, 0.06758530183727033680 ) ) ;
#51429=CARTESIAN_POINT ( 'NONE',  ( -0.2891555358219911054, 0.2891555358219909388, -0.2539370078740157410 ) ) ;
#51436=CARTESIAN_POINT ( 'NONE',  ( -0.3460692066303960313, 0.1998031496062989965, -0.8904199475065617264 ) ) ;
#51438=CARTESIAN_POINT ( 'NONE',  ( 0.2867679344610365999, -0.2867679344610365444, -0.7204724409448818312 ) ) ;
#51455=CARTESIAN_POINT ( 'NONE',  ( -0.1265901696524993347, 0.4724409448818895907, -2.603018372703412631 ) ) ;
#51459=( BOUNDED_SURFACE ( )  B_SPLINE_SURFACE ( 1, 2, ( 
 ( #48736, #17196, #16780, #42418, #11280, #9624, #81581, #68118, #3307, #10463, #75258, #29794, #81164, #23480, #43234, #68931, #36939, #56292, #15955, #60957, #28972, #63029, #64683, #6602, #38590, #50792, #31028, #45308, #75671, #69348, #38172, #5367, #70576, #56696, #57521, #44064, #7022, #64268, #51612, #32274, #83212, #13346, #50381, #76493, #32690, #82395, #76079, #18423, #69756, #24713, #63846, #12102, #18011, #58357, #82798, #25534, #12930, #77317, #37760, #25122, #51199, #12511, #43645, #76897, #18820, #57103, #19227, #63435, #19647, #5771, #31440, #57934, #44467, #70158, #298, #71003, #25954, #44877, #39000, #719, #26377, #6184, #11702, #37356, #31862, #52452, #34370, #27631, #8283, #33949, #26795, #9121, #20910, #71421, #46563, #2802, #2391, #65947, #59198, #71842, #47396, #53293, #1557, #78584, #79005, #27211, #34791, #13768, #15437, #60450, #73087, #58787, #14192, #60035, #28047, #20493, #39425, #52037, #20072, #41098, #1145, #45724, #39849, #65109, #66786, #66361, #72262, #53705, #21733, #7447, #40264, #33117, #59613, #46147, #79414, #77741, #78162, #52874, #65540, #7871, #33535, #14610, #1968, #21324, #46977, #72671, #15020, #40676, #8699, #17102, #81484, #35611, #62106, #68023, #29295, #36026, #54539, #79836, #47812, #42323, #15863, #61274, #28461, #54957, #80664, #3627, #68433, #16684, #11186, #22153, #73514, #62519, #22976, #41511, #10366, #80254, #23800, #9527, #61698, #49055, #10773, #4038, #35199, #67196, #4449, #22571, #81071, #55366, #48643, #67608, #29703, #17511, #30114, #54122, #60860, #3214, #23387, #41914, #74754, #36847, #28876, #73927, #48231, #42737, #74337, #36433, #49473, #16269, #55776, #9939, #75166, #43143, #68840, #50698, #63340, #43555, #6509, #62938, #24621, #30935, #70062, #82302, #49879, #75579, #77218, #19131, #51103, #5675, #69256, #57834, #4858, #81897, #76396, #17919, #83119, #11603, #12416, #56602, #19547, #76800, #64175, #44780, #38074, #25854, #5271, #31343, #45206, #37262, #50288, #75986, #18328, #43968, #18728, #69665, #30532, #70906, #6089, #70477, #12008, #37662, #12834, #44370, #38492, #31764, #57009, #82705, #25025, #32179, #63750, #57425, #25437, #202, #51514, #13257, #38906, #56196, #24208, #60667, #21127, #8504, #35001, #66164, #73733, #9331, #15238, #40898, #67408, #3429, #14826, #34170, #16070, #66579, #21955, #41716, #48440, #8914, #46786, #3015, #61079, #54343, #29092, #54762, #22779, #79222, #9743, #72889, #35414, #41316, #15657, #48031, #80468, #34590, #74140, #66999, #28682, #16484, #72477, #53090, #64586, #59833, #80053, #22372, #60257, #21538, #47613, #6923, #32594, #59415, #27429, #1772, #53925, #47198, #78802, #40486, #2186, #27854, #53514, #2605, #28263, #79637, #73309, #10164, #69048, #61905, #29504, #4247, #75372, #4651, #17316, #80874, #43758, #16902, #29909, #68243, #24012, #36235, #3844, #55164, #31143, #56406, #5074, #42944, #23186, #11814, #42131, #35830, #30322, #48856, #37054, #74557, #49680, #10578, #56810, #30743, #18126, #82105, #17718, #63142, #42541, #68639, #82509, #55573, #81281, #23597, #49268, #74970, #55990, #10978, #67826, #24825, #43346, #24418, #36638, #62314, #50088, #81701, #75784, #11397, #62737, #69464, #37469, #5483, #50493, #76196, #61496, #77860, #83309, #70699, #19350, #45424, #25653, #13463, #57217, #44583, #71120, #18935, #26502, #39120, #51315, #77018, #20189, #39545, #50904, #70276, #52155, #45000, #58053, #45840, #1265, #13052, #82919, #64801, #13886, #7140, #65234, #7571, #58905, #31978, #32813, #71538, #25239, #38705, #77436, #64384, #18534, #19771, #6720, #32390, #58480, #76604, #33243, #31560, #63965, #844, #38289, #12630, #26913, #52573, #44177, #51734, #419, #69870, #12222, #26075, #37879, #63553, #5887, #6302, #57638, #53821, #34488, #60154, #52989, #35314, #47096 ),
 ( #21440, #59316, #73205, #73632, #66902, #41621, #67310, #60976, #8400, #2919, #2085, #47927, #79535, #28165, #60568, #1672, #65660, #28582, #21026, #47513, #21849, #53414, #34067, #2506, #9645, #54239, #28991, #39973, #14313, #66477, #59730, #15555, #3327, #78702, #40381, #14728, #41214, #27750, #79123, #15974, #46265, #9232, #66064, #7989, #72786, #34905, #40792, #15136, #33653, #79956, #46686, #8812, #72379, #22269, #78282, #27329, #20613, #71960, #68951, #17622, #29813, #10060, #24324, #54657, #48340, #17216, #42030, #49583, #35723, #36543, #23088, #69368, #43254, #30647, #11301, #62219, #75691, #29406, #36960, #56312, #62637, #4557, #18032, #55065, #55474, #43666, #61393, #80773, #48755, #74454, #3742, #42849, #16800, #80368, #37378, #55890, #4981, #42437, #68137, #82009, #68542, #49994, #81601, #10482, #36135, #61808, #11722, #10883, #30227, #4148, #63048, #81184, #23501, #49167, #23918, #74873, #75279, #5387, #22681, #74037, #16384, #67724, #57952, #63866, #6203, #32712, #52055, #63457, #31462, #39019, #31881, #70596, #64703, #13787, #57541, #12123, #25973, #26397, #19665, #77761, #20093, #71439, #44486, #7043, #38191, #740, #6621, #64286, #13366, #37781, #18443, #58378, #57124, #320, #51632, #83232, #70178, #12950, #45744, #39444, #65132, #76099, #50402, #19246, #12530, #77336, #31048, #5792, #76512, #50811, #32292, #25553, #51220, #56718, #82415, #45327, #18841, #44085, #76917, #71022, #44897, #38608, #69779, #24734, #82818, #25142, #33553, #72689, #1577, #52474, #78182, #79852, #21749, #53722, #65965, #46165, #60467, #7467, #1165, #53311, #20513, #2407, #71861, #15037, #59215, #22169, #60051, #15878, #65558, #52891, #27232, #40692, #40283, #8301, #2817, #58807, #34386, #78604, #14211, #20927, #66378, #79024, #33969, #39868, #9137, #7891, #46583, #72281, #8715, #14628, #59630, #1986, #47828, #47413, #79430, #27649, #21342, #28478, #33136, #26816, #46996, #28065, #73103, #15455, #41113, #66802, #73531, #34808, #54138, #41526, #74770, #4874, #41931, #42340, #56211, #48246, #67625, #9957, #35628, #16287, #29719, #61290, #9545, #49895, #68448, #55793, #73942, #3644, #49488, #55381, #30129, #10788, #29311, #54972, #80679, #81499, #23404, #81087, #22993, #43158, #48658, #36041, #68038, #36448, #74356, #62121, #22585, #16699, #4464, #10384, #75181, #23818, #61713, #4052, #68854, #30547, #49071, #17118, #17526, #42754, #11203, #36862, #75594, #62536, #81912, #24224, #17933, #67212, #35214, #60878, #3229, #28894, #54555, #80270, #32192, #31777, #6104, #70491, #56617, #5289, #38507, #76001, #25451, #57439, #82719, #5689, #12430, #51529, #64188, #70921, #62953, #37277, #70077, #63355, #12023, #12848, #69680, #82316, #51118, #57849, #6523, #83132, #38089, #25867, #19145, #44383, #216, #77232, #19561, #18343, #45220, #76813, #63763, #44795, #50303, #43569, #76411, #30950, #18741, #69270, #11616, #24636, #43983, #37679, #31359, #57025, #25039, #50712, #11044, #10642, #18191, #54826, #82170, #75849, #30803, #42193, #80935, #17782, #43416, #3906, #22842, #43824, #3491, #56469, #67888, #29157, #55228, #80530, #24486, #49743, #55638, #11462, #5138, #48501, #23662, #74202, #49333, #29566, #69114, #69528, #10226, #42604, #35475, #50153, #16549, #61139, #61563, #81348, #35893, #37120, #23251, #56055, #48921, #24074, #74621, #68306, #62804, #75034, #36297, #43009, #16965, #61971, #4310, #17379, #29974, #68703, #36703, #62377, #4715, #30389, #75443, #81764, #77930, #63206, #5545, #45910, #44647, #31210, #66, #37941, #7212, #76262, #25720, #32459, #77509, #51380, #18998, #45069, #58121, #71190, #18597, #70344, #70772, #32044, #11878, #13123, #12698, #76665, #38774, #44240, #13532, #24890, #63618, #57703, #69929, #19844, #917, #488, #37530, #26143, #64872, #38357, #45493, #77085, #64033 ) ),
 .UNSPECIFIED., .F., .F., .F. ) 
 B_SPLINE_SURFACE_WITH_KNOTS ( ( 2, 2 ),
 ( 3, 2, 2, 2, 2, 2, 2, 2, 2, 2, 2, 2, 2, 2, 2, 2, 2, 2, 2, 2, 2, 2, 2, 2, 2, 2, 2, 2, 2, 2, 2, 2, 2, 2, 2, 2, 2, 2, 2, 2, 2, 2, 2, 2, 2, 2, 2, 2, 2, 2, 2, 2, 2, 2, 2, 2, 2, 2, 2, 2, 2, 2, 2, 2, 2, 2, 2, 2, 2, 2, 2, 2, 2, 2, 2, 2, 2, 2, 2, 2, 2, 2, 2, 2, 2, 2, 2, 2, 2, 2, 2, 2, 2, 2, 2, 2, 2, 2, 2, 2, 2, 2, 2, 2, 2, 2, 2, 2, 2, 2, 2, 2, 2, 2, 2, 2, 2, 2, 2, 2, 2, 2, 2, 2, 2, 2, 2, 2, 2, 2, 2, 2, 2, 2, 2, 2, 2, 2, 2, 2, 2, 2, 2, 2, 2, 2, 2, 2, 2, 2, 2, 2, 2, 2, 2, 2, 2, 2, 2, 2, 2, 2, 2, 2, 2, 2, 2, 2, 2, 2, 2, 2, 2, 2, 2, 2, 2, 2, 2, 2, 2, 2, 2, 2, 2, 2, 2, 2, 2, 2, 2, 2, 2, 2, 2, 2, 2, 2, 2, 2, 2, 2, 2, 2, 2, 2, 2, 2, 2, 2, 2, 2, 2, 2, 2, 2, 2, 2, 2, 2, 2, 2, 2, 2, 2, 2, 2, 2, 2, 2, 2, 2, 2, 2, 2, 2, 2, 3 ),
 ( 0.000000000000000000, 1.000000000000000000 ),
 ( 0.000000000000000000, 0.004166666666666666609, 0.008333333333333333218, 0.01250000000000000069, 0.01666666666666666644, 0.02083333333333333218, 0.02500000000000000139, 0.02916666666666666713, 0.03333333333333333287, 0.03749999999999999861, 0.04166666666666666435, 0.04583333333333333010, 0.05000000000000000278, 0.05416666666666666852, 0.05833333333333333426, 0.06250000000000000000, 0.06666666666666666574, 0.07083333333333333148, 0.07499999999999999722, 0.07916666666666666297, 0.08333333333333332871, 0.08749999999999999445, 0.09166666666666666019, 0.09583333333333333981, 0.1000000000000000056, 0.1041666666666666713, 0.1083333333333333370, 0.1125000000000000028, 0.1166666666666666685, 0.1208333333333333343, 0.1250000000000000000, 0.1291666666666666796, 0.1333333333333333315, 0.1375000000000000111, 0.1416666666666666630, 0.1458333333333333426, 0.1499999999999999944, 0.1541666666666666741, 0.1583333333333333259, 0.1625000000000000056, 0.1666666666666666574, 0.1708333333333333370, 0.1749999999999999889, 0.1791666666666666685, 0.1833333333333333204, 0.1875000000000000000, 0.1916666666666666796, 0.1958333333333333315, 0.2000000000000000111, 0.2041666666666666630, 0.2083333333333333426, 0.2124999999999999944, 0.2166666666666666741, 0.2208333333333333259, 0.2250000000000000056, 0.2291666666666666574, 0.2333333333333333370, 0.2374999999999999889, 0.2416666666666666685, 0.2458333333333333204, 0.2500000000000000000, 0.2541666666666666519, 0.2583333333333333592, 0.2625000000000000111, 0.2666666666666666630, 0.2708333333333333148, 0.2750000000000000222, 0.2791666666666666741, 0.2833333333333333259, 0.2874999999999999778, 0.2916666666666666852, 0.2958333333333333370, 0.2999999999999999889, 0.3041666666666666408, 0.3083333333333333481, 0.3125000000000000000, 0.3166666666666666519, 0.3208333333333333592, 0.3250000000000000111, 0.3291666666666666630, 0.3333333333333333148, 0.3375000000000000222, 0.3416666666666666741, 0.3458333333333333259, 0.3499999999999999778, 0.3541666666666666852, 0.3583333333333333370, 0.3624999999999999889, 0.3666666666666666408, 0.3708333333333333481, 0.3750000000000000000, 0.3791666666666666519, 0.3833333333333333592, 0.3875000000000000111, 0.3916666666666666630, 0.3958333333333333148, 0.4000000000000000222, 0.4041666666666666741, 0.4083333333333333259, 0.4124999999999999778, 0.4166666666666666852, 0.4208333333333333370, 0.4249999999999999889, 0.4291666666666666408, 0.4333333333333333481, 0.4375000000000000000, 0.4416666666666666519, 0.4458333333333333592, 0.4500000000000000111, 0.4541666666666666630, 0.4583333333333333148, 0.4625000000000000222, 0.4666666666666666741, 0.4708333333333333259, 0.4749999999999999778, 0.4791666666666666852, 0.4833333333333333370, 0.4874999999999999889, 0.4916666666666666408, 0.4958333333333333481, 0.5000000000000000000, 0.5041666666666666519, 0.5083333333333333037, 0.5124999999999999556, 0.5166666666666667185, 0.5208333333333333703, 0.5250000000000000222, 0.5291666666666666741, 0.5333333333333333259, 0.5374999999999999778, 0.5416666666666666297, 0.5458333333333332815, 0.5500000000000000444, 0.5541666666666666963, 0.5583333333333333481, 0.5625000000000000000, 0.5666666666666666519, 0.5708333333333333037, 0.5749999999999999556, 0.5791666666666667185, 0.5833333333333333703, 0.5875000000000000222, 0.5916666666666666741, 0.5958333333333333259, 0.5999999999999999778, 0.6041666666666666297, 0.6083333333333332815, 0.6125000000000000444, 0.6166666666666666963, 0.6208333333333333481, 0.6250000000000000000, 0.6291666666666666519, 0.6333333333333333037, 0.6374999999999999556, 0.6416666666666667185, 0.6458333333333333703, 0.6500000000000000222, 0.6541666666666666741, 0.6583333333333333259, 0.6624999999999999778, 0.6666666666666666297, 0.6708333333333332815, 0.6750000000000000444, 0.6791666666666666963, 0.6833333333333333481, 0.6875000000000000000, 0.6916666666666666519, 0.6958333333333333037, 0.6999999999999999556, 0.7041666666666667185, 0.7083333333333333703, 0.7125000000000000222, 0.7166666666666666741, 0.7208333333333333259, 0.7249999999999999778, 0.7291666666666666297, 0.7333333333333332815, 0.7375000000000000444, 0.7416666666666666963, 0.7458333333333333481, 0.7500000000000000000, 0.7541666666666666519, 0.7583333333333333037, 0.7624999999999999556, 0.7666666666666667185, 0.7708333333333333703, 0.7750000000000000222, 0.7791666666666666741, 0.7833333333333333259, 0.7874999999999999778, 0.7916666666666666297, 0.7958333333333332815, 0.8000000000000000444, 0.8041666666666666963, 0.8083333333333333481, 0.8125000000000000000, 0.8166666666666666519, 0.8208333333333333037, 0.8249999999999999556, 0.8291666666666667185, 0.8333333333333333703, 0.8375000000000000222, 0.8416666666666666741, 0.8458333333333333259, 0.8499999999999999778, 0.8541666666666666297, 0.8583333333333332815, 0.8625000000000000444, 0.8666666666666666963, 0.8708333333333333481, 0.8750000000000000000, 0.8791666666666666519, 0.8833333333333333037, 0.8874999999999999556, 0.8916666666666667185, 0.8958333333333333703, 0.9000000000000000222, 0.9041666666666666741, 0.9083333333333333259, 0.9124999999999999778, 0.9166666666666666297, 0.9208333333333332815, 0.9250000000000000444, 0.9291666666666666963, 0.9333333333333333481, 0.9375000000000000000, 0.9416666666666666519, 0.9458333333333333037, 0.9499999999999999556, 0.9541666666666667185, 0.9583333333333333703, 0.9625000000000000222, 0.9666666666666666741, 0.9708333333333333259, 0.9749999999999999778, 0.9791666666666666297, 0.9833333333333332815, 0.9875000000000000444 ),
 .UNSPECIFIED. ) 
 GEOMETRIC_REPRESENTATION_ITEM ( )  RATIONAL_B_SPLINE_SURFACE ( (
 ( 1.000000000000000000, 0.9659258262890683122, 1.000000000000000000, 0.9659258262890683122, 1.000000000000000000, 0.9659258262890683122, 1.000000000000000000, 0.9659258262890683122, 1.000000000000000000, 0.9659258262890683122, 1.000000000000000000, 0.9659258262890683122, 1.000000000000000000, 0.9659258262890683122, 1.000000000000000000, 0.9659258262890683122, 1.000000000000000000, 0.9659258262890683122, 1.000000000000000000, 0.9659258262890683122, 1.000000000000000000, 0.9659258262890683122, 1.000000000000000000, 0.9659258262890683122, 1.000000000000000000, 0.9659258262890683122, 1.000000000000000000, 0.9659258262890683122, 1.000000000000000000, 0.9659258262890683122, 1.000000000000000000, 0.9659258262890683122, 1.000000000000000000, 0.9659258262890683122, 1.000000000000000000, 0.9659258262890683122, 1.000000000000000000, 0.9659258262890683122, 1.000000000000000000, 0.9659258262890683122, 1.000000000000000000, 0.9659258262890683122, 1.000000000000000000, 0.9659258262890683122, 1.000000000000000000, 0.9659258262890683122, 1.000000000000000000, 0.9659258262890683122, 1.000000000000000000, 0.9659258262890683122, 1.000000000000000000, 0.9659258262890683122, 1.000000000000000000, 0.9659258262890683122, 1.000000000000000000, 0.9659258262890683122, 1.000000000000000000, 0.9659258262890683122, 1.000000000000000000, 0.9659258262890683122, 1.000000000000000000, 0.9659258262890683122, 1.000000000000000000, 0.9659258262890683122, 1.000000000000000000, 0.9659258262890683122, 1.000000000000000000, 0.9659258262890683122, 1.000000000000000000, 0.9659258262890683122, 1.000000000000000000, 0.9659258262890683122, 1.000000000000000000, 0.9659258262890683122, 1.000000000000000000, 0.9659258262890683122, 1.000000000000000000, 0.9659258262890683122, 1.000000000000000000, 0.9659258262890683122, 1.000000000000000000, 0.9659258262890683122, 1.000000000000000000, 0.9659258262890683122, 1.000000000000000000, 0.9659258262890683122, 1.000000000000000000, 0.9659258262890683122, 1.000000000000000000, 0.9659258262890683122, 1.000000000000000000, 0.9659258262890683122, 1.000000000000000000, 0.9659258262890683122, 1.000000000000000000, 0.9659258262890683122, 1.000000000000000000, 0.9659258262890683122, 1.000000000000000000, 0.9659258262890683122, 1.000000000000000000, 0.9659258262890683122, 1.000000000000000000, 0.9659258262890683122, 1.000000000000000000, 0.9659258262890683122, 1.000000000000000000, 0.9659258262890683122, 1.000000000000000000, 0.9659258262890683122, 1.000000000000000000, 0.9659258262890683122, 1.000000000000000000, 0.9659258262890683122, 1.000000000000000000, 0.9659258262890683122, 1.000000000000000000, 0.9659258262890683122, 1.000000000000000000, 0.9659258262890683122, 1.000000000000000000, 0.9659258262890683122, 1.000000000000000000, 0.9659258262890683122, 1.000000000000000000, 0.9659258262890683122, 1.000000000000000000, 0.9659258262890683122, 1.000000000000000000, 0.9659258262890683122, 1.000000000000000000, 0.9659258262890683122, 1.000000000000000000, 0.9659258262890683122, 1.000000000000000000, 0.9659258262890683122, 1.000000000000000000, 0.9659258262890683122, 1.000000000000000000, 0.9659258262890683122, 1.000000000000000000, 0.9659258262890683122, 1.000000000000000000, 0.9659258262890683122, 1.000000000000000000, 0.9659258262890683122, 1.000000000000000000, 0.9659258262890683122, 1.000000000000000000, 0.9659258262890683122, 1.000000000000000000, 0.9659258262890683122, 1.000000000000000000, 0.9659258262890683122, 1.000000000000000000, 0.9659258262890683122, 1.000000000000000000, 0.9659258262890683122, 1.000000000000000000, 0.9659258262890683122, 1.000000000000000000, 0.9659258262890683122, 1.000000000000000000, 0.9659258262890683122, 1.000000000000000000, 0.9659258262890683122, 1.000000000000000000, 0.9659258262890683122, 1.000000000000000000, 0.9659258262890683122, 1.000000000000000000, 0.9659258262890683122, 1.000000000000000000, 0.9659258262890683122, 1.000000000000000000, 0.9659258262890683122, 1.000000000000000000, 0.9659258262890683122, 1.000000000000000000, 0.9659258262890683122, 1.000000000000000000, 0.9659258262890683122, 1.000000000000000000, 0.9659258262890683122, 1.000000000000000000, 0.9659258262890683122, 1.000000000000000000, 0.9659258262890683122, 1.000000000000000000, 0.9659258262890683122, 1.000000000000000000, 0.9659258262890683122, 1.000000000000000000, 0.9659258262890683122, 1.000000000000000000, 0.9659258262890683122, 1.000000000000000000, 0.9659258262890683122, 1.000000000000000000, 0.9659258262890683122, 1.000000000000000000, 0.9659258262890683122, 1.000000000000000000, 0.9659258262890683122, 1.000000000000000000, 0.9659258262890683122, 1.000000000000000000, 0.9659258262890683122, 1.000000000000000000, 0.9659258262890683122, 1.000000000000000000, 0.9659258262890683122, 1.000000000000000000, 0.9659258262890683122, 1.000000000000000000, 0.9659258262890683122, 1.000000000000000000, 0.9659258262890683122, 1.000000000000000000, 0.9659258262890683122, 1.000000000000000000, 0.9659258262890683122, 1.000000000000000000, 0.9659258262890683122, 1.000000000000000000, 0.9659258262890683122, 1.000000000000000000, 0.9659258262890683122, 1.000000000000000000, 0.9659258262890683122, 1.000000000000000000, 0.9659258262890683122, 1.000000000000000000, 0.9659258262890683122, 1.000000000000000000, 0.9659258262890683122, 1.000000000000000000, 0.9659258262890683122, 1.000000000000000000, 0.9659258262890683122, 1.000000000000000000, 0.9659258262890683122, 1.000000000000000000, 0.9659258262890683122, 1.000000000000000000, 0.9659258262890683122, 1.000000000000000000, 0.9659258262890683122, 1.000000000000000000, 0.9659258262890683122, 1.000000000000000000, 0.9659258262890683122, 1.000000000000000000, 0.9659258262890683122, 1.000000000000000000, 0.9659258262890683122, 1.000000000000000000, 0.9659258262890683122, 1.000000000000000000, 0.9659258262890683122, 1.000000000000000000, 0.9659258262890683122, 1.000000000000000000, 0.9659258262890683122, 1.000000000000000000, 0.9659258262890683122, 1.000000000000000000, 0.9659258262890683122, 1.000000000000000000, 0.9659258262890683122, 1.000000000000000000, 0.9659258262890683122, 1.000000000000000000, 0.9659258262890683122, 1.000000000000000000, 0.9659258262890683122, 1.000000000000000000, 0.9659258262890683122, 1.000000000000000000, 0.9659258262890683122, 1.000000000000000000, 0.9659258262890683122, 1.000000000000000000, 0.9659258262890683122, 1.000000000000000000, 0.9659258262890683122, 1.000000000000000000, 0.9659258262890683122, 1.000000000000000000, 0.9659258262890683122, 1.000000000000000000, 0.9659258262890683122, 1.000000000000000000, 0.9659258262890683122, 1.000000000000000000, 0.9659258262890683122, 1.000000000000000000, 0.9659258262890683122, 1.000000000000000000, 0.9659258262890683122, 1.000000000000000000, 0.9659258262890683122, 1.000000000000000000, 0.9659258262890683122, 1.000000000000000000, 0.9659258262890683122, 1.000000000000000000, 0.9659258262890683122, 1.000000000000000000, 0.9659258262890683122, 1.000000000000000000, 0.9659258262890683122, 1.000000000000000000, 0.9659258262890683122, 1.000000000000000000, 0.9659258262890683122, 1.000000000000000000, 0.9659258262890683122, 1.000000000000000000, 0.9659258262890683122, 1.000000000000000000, 0.9659258262890683122, 1.000000000000000000, 0.9659258262890683122, 1.000000000000000000, 0.9659258262890683122, 1.000000000000000000, 0.9659258262890683122, 1.000000000000000000, 0.9659258262890683122, 1.000000000000000000, 0.9659258262890683122, 1.000000000000000000, 0.9659258262890683122, 1.000000000000000000, 0.9659258262890683122, 1.000000000000000000, 0.9659258262890683122, 1.000000000000000000, 0.9659258262890683122, 1.000000000000000000, 0.9659258262890683122, 1.000000000000000000, 0.9659258262890683122, 1.000000000000000000, 0.9659258262890683122, 1.000000000000000000, 0.9659258262890683122, 1.000000000000000000, 0.9659258262890683122, 1.000000000000000000, 0.9659258262890683122, 1.000000000000000000, 0.9659258262890683122, 1.000000000000000000, 0.9659258262890683122, 1.000000000000000000, 0.9659258262890683122, 1.000000000000000000, 0.9659258262890683122, 1.000000000000000000, 0.9659258262890683122, 1.000000000000000000, 0.9659258262890683122, 1.000000000000000000, 0.9659258262890683122, 1.000000000000000000, 0.9659258262890683122, 1.000000000000000000, 0.9659258262890683122, 1.000000000000000000, 0.9659258262890683122, 1.000000000000000000, 0.9659258262890683122, 1.000000000000000000, 0.9659258262890683122, 1.000000000000000000, 0.9659258262890683122, 1.000000000000000000, 0.9659258262890683122, 1.000000000000000000, 0.9659258262890683122, 1.000000000000000000, 0.9659258262890683122, 1.000000000000000000, 0.9659258262890683122, 1.000000000000000000, 0.9659258262890683122, 1.000000000000000000, 0.9659258262890683122, 1.000000000000000000, 0.9659258262890683122, 1.000000000000000000, 0.9659258262890683122, 1.000000000000000000, 0.9659258262890683122, 1.000000000000000000, 0.9659258262890683122, 1.000000000000000000, 0.9659258262890683122, 1.000000000000000000, 0.9659258262890683122, 1.000000000000000000, 0.9659258262890683122, 1.000000000000000000, 0.9659258262890683122, 1.000000000000000000, 0.9659258262890683122, 1.000000000000000000, 0.9659258262890683122, 1.000000000000000000, 0.9659258262890683122, 1.000000000000000000, 0.9659258262890683122, 1.000000000000000000, 0.9659258262890683122, 1.000000000000000000, 0.9659258262890683122, 1.000000000000000000, 0.9659258262890683122, 1.000000000000000000, 0.9659258262890683122, 1.000000000000000000, 0.9659258262890683122, 1.000000000000000000, 0.9659258262890683122, 1.000000000000000000, 0.9659258262890683122, 1.000000000000000000, 0.9659258262890683122, 1.000000000000000000, 0.9659258262890683122, 1.000000000000000000, 0.9659258262890683122, 1.000000000000000000, 0.9659258262890683122, 1.000000000000000000, 0.9659258262890683122, 1.000000000000000000, 0.9659258262890683122, 1.000000000000000000, 0.9659258262890683122, 1.000000000000000000, 0.9659258262890683122, 1.000000000000000000, 0.9659258262890683122, 1.000000000000000000, 0.9659258262890683122, 1.000000000000000000, 0.9659258262890683122, 1.000000000000000000, 0.9659258262890683122, 1.000000000000000000, 0.9659258262890683122, 1.000000000000000000, 0.9659258262890683122, 1.000000000000000000, 0.9659258262890683122, 1.000000000000000000, 0.9659258262890683122, 1.000000000000000000, 0.9659258262890683122, 1.000000000000000000, 0.9659258262890683122, 1.000000000000000000, 0.9659258262890683122, 1.000000000000000000, 0.9659258262890683122, 1.000000000000000000, 0.9659258262890683122, 1.000000000000000000, 0.9659258262890683122, 1.000000000000000000, 0.9659258262890683122, 1.000000000000000000),
 ( 1.000000000000000000, 0.9659258262890683122, 1.000000000000000000, 0.9659258262890683122, 1.000000000000000000, 0.9659258262890683122, 1.000000000000000000, 0.9659258262890683122, 1.000000000000000000, 0.9659258262890683122, 1.000000000000000000, 0.9659258262890683122, 1.000000000000000000, 0.9659258262890683122, 1.000000000000000000, 0.9659258262890683122, 1.000000000000000000, 0.9659258262890683122, 1.000000000000000000, 0.9659258262890683122, 1.000000000000000000, 0.9659258262890683122, 1.000000000000000000, 0.9659258262890683122, 1.000000000000000000, 0.9659258262890683122, 1.000000000000000000, 0.9659258262890683122, 1.000000000000000000, 0.9659258262890683122, 1.000000000000000000, 0.9659258262890683122, 1.000000000000000000, 0.9659258262890683122, 1.000000000000000000, 0.9659258262890683122, 1.000000000000000000, 0.9659258262890683122, 1.000000000000000000, 0.9659258262890683122, 1.000000000000000000, 0.9659258262890683122, 1.000000000000000000, 0.9659258262890683122, 1.000000000000000000, 0.9659258262890683122, 1.000000000000000000, 0.9659258262890683122, 1.000000000000000000, 0.9659258262890683122, 1.000000000000000000, 0.9659258262890683122, 1.000000000000000000, 0.9659258262890683122, 1.000000000000000000, 0.9659258262890683122, 1.000000000000000000, 0.9659258262890683122, 1.000000000000000000, 0.9659258262890683122, 1.000000000000000000, 0.9659258262890683122, 1.000000000000000000, 0.9659258262890683122, 1.000000000000000000, 0.9659258262890683122, 1.000000000000000000, 0.9659258262890683122, 1.000000000000000000, 0.9659258262890683122, 1.000000000000000000, 0.9659258262890683122, 1.000000000000000000, 0.9659258262890683122, 1.000000000000000000, 0.9659258262890683122, 1.000000000000000000, 0.9659258262890683122, 1.000000000000000000, 0.9659258262890683122, 1.000000000000000000, 0.9659258262890683122, 1.000000000000000000, 0.9659258262890683122, 1.000000000000000000, 0.9659258262890683122, 1.000000000000000000, 0.9659258262890683122, 1.000000000000000000, 0.9659258262890683122, 1.000000000000000000, 0.9659258262890683122, 1.000000000000000000, 0.9659258262890683122, 1.000000000000000000, 0.9659258262890683122, 1.000000000000000000, 0.9659258262890683122, 1.000000000000000000, 0.9659258262890683122, 1.000000000000000000, 0.9659258262890683122, 1.000000000000000000, 0.9659258262890683122, 1.000000000000000000, 0.9659258262890683122, 1.000000000000000000, 0.9659258262890683122, 1.000000000000000000, 0.9659258262890683122, 1.000000000000000000, 0.9659258262890683122, 1.000000000000000000, 0.9659258262890683122, 1.000000000000000000, 0.9659258262890683122, 1.000000000000000000, 0.9659258262890683122, 1.000000000000000000, 0.9659258262890683122, 1.000000000000000000, 0.9659258262890683122, 1.000000000000000000, 0.9659258262890683122, 1.000000000000000000, 0.9659258262890683122, 1.000000000000000000, 0.9659258262890683122, 1.000000000000000000, 0.9659258262890683122, 1.000000000000000000, 0.9659258262890683122, 1.000000000000000000, 0.9659258262890683122, 1.000000000000000000, 0.9659258262890683122, 1.000000000000000000, 0.9659258262890683122, 1.000000000000000000, 0.9659258262890683122, 1.000000000000000000, 0.9659258262890683122, 1.000000000000000000, 0.9659258262890683122, 1.000000000000000000, 0.9659258262890683122, 1.000000000000000000, 0.9659258262890683122, 1.000000000000000000, 0.9659258262890683122, 1.000000000000000000, 0.9659258262890683122, 1.000000000000000000, 0.9659258262890683122, 1.000000000000000000, 0.9659258262890683122, 1.000000000000000000, 0.9659258262890683122, 1.000000000000000000, 0.9659258262890683122, 1.000000000000000000, 0.9659258262890683122, 1.000000000000000000, 0.9659258262890683122, 1.000000000000000000, 0.9659258262890683122, 1.000000000000000000, 0.9659258262890683122, 1.000000000000000000, 0.9659258262890683122, 1.000000000000000000, 0.9659258262890683122, 1.000000000000000000, 0.9659258262890683122, 1.000000000000000000, 0.9659258262890683122, 1.000000000000000000, 0.9659258262890683122, 1.000000000000000000, 0.9659258262890683122, 1.000000000000000000, 0.9659258262890683122, 1.000000000000000000, 0.9659258262890683122, 1.000000000000000000, 0.9659258262890683122, 1.000000000000000000, 0.9659258262890683122, 1.000000000000000000, 0.9659258262890683122, 1.000000000000000000, 0.9659258262890683122, 1.000000000000000000, 0.9659258262890683122, 1.000000000000000000, 0.9659258262890683122, 1.000000000000000000, 0.9659258262890683122, 1.000000000000000000, 0.9659258262890683122, 1.000000000000000000, 0.9659258262890683122, 1.000000000000000000, 0.9659258262890683122, 1.000000000000000000, 0.9659258262890683122, 1.000000000000000000, 0.9659258262890683122, 1.000000000000000000, 0.9659258262890683122, 1.000000000000000000, 0.9659258262890683122, 1.000000000000000000, 0.9659258262890683122, 1.000000000000000000, 0.9659258262890683122, 1.000000000000000000, 0.9659258262890683122, 1.000000000000000000, 0.9659258262890683122, 1.000000000000000000, 0.9659258262890683122, 1.000000000000000000, 0.9659258262890683122, 1.000000000000000000, 0.9659258262890683122, 1.000000000000000000, 0.9659258262890683122, 1.000000000000000000, 0.9659258262890683122, 1.000000000000000000, 0.9659258262890683122, 1.000000000000000000, 0.9659258262890683122, 1.000000000000000000, 0.9659258262890683122, 1.000000000000000000, 0.9659258262890683122, 1.000000000000000000, 0.9659258262890683122, 1.000000000000000000, 0.9659258262890683122, 1.000000000000000000, 0.9659258262890683122, 1.000000000000000000, 0.9659258262890683122, 1.000000000000000000, 0.9659258262890683122, 1.000000000000000000, 0.9659258262890683122, 1.000000000000000000, 0.9659258262890683122, 1.000000000000000000, 0.9659258262890683122, 1.000000000000000000, 0.9659258262890683122, 1.000000000000000000, 0.9659258262890683122, 1.000000000000000000, 0.9659258262890683122, 1.000000000000000000, 0.9659258262890683122, 1.000000000000000000, 0.9659258262890683122, 1.000000000000000000, 0.9659258262890683122, 1.000000000000000000, 0.9659258262890683122, 1.000000000000000000, 0.9659258262890683122, 1.000000000000000000, 0.9659258262890683122, 1.000000000000000000, 0.9659258262890683122, 1.000000000000000000, 0.9659258262890683122, 1.000000000000000000, 0.9659258262890683122, 1.000000000000000000, 0.9659258262890683122, 1.000000000000000000, 0.9659258262890683122, 1.000000000000000000, 0.9659258262890683122, 1.000000000000000000, 0.9659258262890683122, 1.000000000000000000, 0.9659258262890683122, 1.000000000000000000, 0.9659258262890683122, 1.000000000000000000, 0.9659258262890683122, 1.000000000000000000, 0.9659258262890683122, 1.000000000000000000, 0.9659258262890683122, 1.000000000000000000, 0.9659258262890683122, 1.000000000000000000, 0.9659258262890683122, 1.000000000000000000, 0.9659258262890683122, 1.000000000000000000, 0.9659258262890683122, 1.000000000000000000, 0.9659258262890683122, 1.000000000000000000, 0.9659258262890683122, 1.000000000000000000, 0.9659258262890683122, 1.000000000000000000, 0.9659258262890683122, 1.000000000000000000, 0.9659258262890683122, 1.000000000000000000, 0.9659258262890683122, 1.000000000000000000, 0.9659258262890683122, 1.000000000000000000, 0.9659258262890683122, 1.000000000000000000, 0.9659258262890683122, 1.000000000000000000, 0.9659258262890683122, 1.000000000000000000, 0.9659258262890683122, 1.000000000000000000, 0.9659258262890683122, 1.000000000000000000, 0.9659258262890683122, 1.000000000000000000, 0.9659258262890683122, 1.000000000000000000, 0.9659258262890683122, 1.000000000000000000, 0.9659258262890683122, 1.000000000000000000, 0.9659258262890683122, 1.000000000000000000, 0.9659258262890683122, 1.000000000000000000, 0.9659258262890683122, 1.000000000000000000, 0.9659258262890683122, 1.000000000000000000, 0.9659258262890683122, 1.000000000000000000, 0.9659258262890683122, 1.000000000000000000, 0.9659258262890683122, 1.000000000000000000, 0.9659258262890683122, 1.000000000000000000, 0.9659258262890683122, 1.000000000000000000, 0.9659258262890683122, 1.000000000000000000, 0.9659258262890683122, 1.000000000000000000, 0.9659258262890683122, 1.000000000000000000, 0.9659258262890683122, 1.000000000000000000, 0.9659258262890683122, 1.000000000000000000, 0.9659258262890683122, 1.000000000000000000, 0.9659258262890683122, 1.000000000000000000, 0.9659258262890683122, 1.000000000000000000, 0.9659258262890683122, 1.000000000000000000, 0.9659258262890683122, 1.000000000000000000, 0.9659258262890683122, 1.000000000000000000, 0.9659258262890683122, 1.000000000000000000, 0.9659258262890683122, 1.000000000000000000, 0.9659258262890683122, 1.000000000000000000, 0.9659258262890683122, 1.000000000000000000, 0.9659258262890683122, 1.000000000000000000, 0.9659258262890683122, 1.000000000000000000, 0.9659258262890683122, 1.000000000000000000, 0.9659258262890683122, 1.000000000000000000, 0.9659258262890683122, 1.000000000000000000, 0.9659258262890683122, 1.000000000000000000, 0.9659258262890683122, 1.000000000000000000, 0.9659258262890683122, 1.000000000000000000, 0.9659258262890683122, 1.000000000000000000, 0.9659258262890683122, 1.000000000000000000, 0.9659258262890683122, 1.000000000000000000, 0.9659258262890683122, 1.000000000000000000, 0.9659258262890683122, 1.000000000000000000, 0.9659258262890683122, 1.000000000000000000, 0.9659258262890683122, 1.000000000000000000, 0.9659258262890683122, 1.000000000000000000, 0.9659258262890683122, 1.000000000000000000, 0.9659258262890683122, 1.000000000000000000, 0.9659258262890683122, 1.000000000000000000, 0.9659258262890683122, 1.000000000000000000, 0.9659258262890683122, 1.000000000000000000, 0.9659258262890683122, 1.000000000000000000, 0.9659258262890683122, 1.000000000000000000, 0.9659258262890683122, 1.000000000000000000, 0.9659258262890683122, 1.000000000000000000, 0.9659258262890683122, 1.000000000000000000, 0.9659258262890683122, 1.000000000000000000, 0.9659258262890683122, 1.000000000000000000, 0.9659258262890683122, 1.000000000000000000, 0.9659258262890683122, 1.000000000000000000, 0.9659258262890683122, 1.000000000000000000, 0.9659258262890683122, 1.000000000000000000, 0.9659258262890683122, 1.000000000000000000, 0.9659258262890683122, 1.000000000000000000, 0.9659258262890683122, 1.000000000000000000, 0.9659258262890683122, 1.000000000000000000, 0.9659258262890683122, 1.000000000000000000, 0.9659258262890683122, 1.000000000000000000, 0.9659258262890683122, 1.000000000000000000, 0.9659258262890683122, 1.000000000000000000, 0.9659258262890683122, 1.000000000000000000, 0.9659258262890683122, 1.000000000000000000, 0.9659258262890683122, 1.000000000000000000, 0.9659258262890683122, 1.000000000000000000, 0.9659258262890683122, 1.000000000000000000) ) ) 
 REPRESENTATION_ITEM ( '' )  SURFACE ( )  );
#51472=CARTESIAN_POINT ( 'NONE',  ( 0.3460692066303959757, -0.1998031496062991907, -0.2624671916010499206 ) ) ;
#51473=CARTESIAN_POINT ( 'NONE',  ( -0.3460692066303960313, 0.1998031496062989965, -2.622703412073490892 ) ) ;
#51478=CARTESIAN_POINT ( 'NONE',  ( -9.787531504996567848E-17, 0.3996062992125986035, -2.047244094488188892 ) ) ;
#51479=CARTESIAN_POINT ( 'NONE',  ( -0.3420746716998661618, 0.1974969037888702206, -1.916010498687664043 ) ) ;
#51480=CARTESIAN_POINT ( 'NONE',  ( -0.3917322834645671215, 0.1049643490035301469, -0.3398950131233596239 ) ) ;
#51482=CARTESIAN_POINT ( 'NONE',  ( 4.797336870675656522E-17, -0.3917322834645670104, -1.015748031496062964 ) ) ;
#51485=CARTESIAN_POINT ( 'NONE',  ( 0.3420746716998660508, 0.1974969037888705814, -2.570209973753280863 ) ) ;
#51489=CARTESIAN_POINT ( 'NONE',  ( -0.4724409448818898682, -8.678599364036362592E-17, -2.716535433070865757 ) ) ;
#51490=CARTESIAN_POINT ( 'NONE',  ( -0.1070741851644056997, 0.3996062992125986035, -2.211286089238845065 ) ) ;
#51491=CARTESIAN_POINT ( 'NONE',  ( -0.1049643490035302301, -0.3917322834645671770, -0.6988382134196345907 ) ) ;
#51497=CARTESIAN_POINT ( 'NONE',  ( 0.2867679344610365999, -0.2867679344610365444, -0.1830708661417323746 ) ) ;
#51506=CARTESIAN_POINT ( 'NONE',  ( -0.3392501089628017219, -0.1958661417322836718, -0.7670603674540683592 ) ) ;
#51507=CARTESIAN_POINT ( 'NONE',  ( -0.2867679344610364334, -0.2867679344610367109, -1.311023622047244430 ) ) ;
#51508=CARTESIAN_POINT ( 'NONE',  ( -0.3917322834645669549, -0.1049643490035306603, -2.872703412073490448 ) ) ;
#51510=CARTESIAN_POINT ( 'NONE',  ( -0.1998031496062991907, -0.3460692066303959757, -0.2230971128608923992 ) ) ;
#51514=CARTESIAN_POINT ( 'NONE',  ( -0.3460692066303958092, -0.1998031496062994683, -1.627296587926509330 ) ) ;
#51519=CARTESIAN_POINT ( 'NONE',  ( -0.3917322834645671215, 0.1049643490035301469, -0.9048556430446195176 ) ) ;
#51529=CARTESIAN_POINT ( 'NONE',  ( 0.3458507752293908943, -0.3458507752293908943, -1.988188976377952777 ) ) ;
#51540=CARTESIAN_POINT ( 'NONE',  ( -0.2867679344610364334, -0.2867679344610368219, -0.6115292406486071419 ) ) ;
#51543=CARTESIAN_POINT ( 'NONE',  ( 0.3917322834645670104, -0.1049643490035303273, -0.9835958005249345604 ) ) ;
#51548=CARTESIAN_POINT ( 'NONE',  ( -0.2867679344610365999, 0.2867679344610364889, -2.688976377952755570 ) ) ;
#51552=CARTESIAN_POINT ( 'NONE',  ( 0.4724409448818897572, -0.1265901696524988906, -1.133202099737532720 ) ) ;
#51565=CARTESIAN_POINT ( 'NONE',  ( -0.1070741851644051862, -0.3996062992125986590, -2.511154855643044748 ) ) ;
#51569=CARTESIAN_POINT ( 'NONE',  ( -0.3996062992125984925, -0.1070741851644056858, -1.382545931758530022 ) ) ;
#51573=CARTESIAN_POINT ( 'NONE',  ( -0.4724409448818898682, -8.678599364036362592E-17, -0.03937007874015747977 ) ) ;
#51575=CARTESIAN_POINT ( 'NONE',  ( 0.3996062992125985480, 2.446882876249141654E-17, -0.8248031496062991907 ) ) ;
#51576=CARTESIAN_POINT ( 'NONE',  ( -0.1070741851644056997, 0.3996062992125986035, -0.7939632545931758489 ) ) ;
#51578=CARTESIAN_POINT ( 'NONE',  ( -0.2891555358219911054, 0.2891555358219909388, -0.4921259842519685179 ) ) ;
#51584=CARTESIAN_POINT ( 'NONE',  ( 0.3949938075777408852, 0.1058382717557500435, -1.146325459317585338 ) ) ;
#51586=( BOUNDED_CURVE ( )  B_SPLINE_CURVE ( 2, ( #36849, #4451, #24623, #67610, #30937, #50290, #18330, #81073, #54959, #75168, #48645, #49881, #9941 ),
 .UNSPECIFIED., .F., .F. ) 
 B_SPLINE_CURVE_WITH_KNOTS ( ( 3, 2, 2, 2, 2, 2, 3 ),
 ( 0.3125000000000000000, 0.3166666666666666519, 0.3208333333333333592, 0.3250000000000000111, 0.3291666666666666630, 0.3333333333333333148, 0.3375000000000000222 ),
 .UNSPECIFIED. ) 
 CURVE ( )  GEOMETRIC_REPRESENTATION_ITEM ( )  RATIONAL_B_SPLINE_CURVE ( ( 1.000000000000000000, 0.9659258262890683122, 1.000000000000000000, 0.9659258262890683122, 1.000000000000000000, 0.9659258262890683122, 1.000000000000000000, 0.9659258262890683122, 1.000000000000000000, 0.9659258262890683122, 1.000000000000000000, 0.9659258262890683122, 1.000000000000000000 ) ) 
 REPRESENTATION_ITEM ( '' )  );
#51590=CARTESIAN_POINT ( 'NONE',  ( 0.1265901696524990294, -0.4724409448818896462, -1.502624671916010346 ) ) ;
#51593=ORIENTED_EDGE ( 'NONE', *, *, #81282, .F. ) ;
#51598=CARTESIAN_POINT ( 'NONE',  ( 0.3392501089628018329, 0.1958661417322835052, -1.943550238023935561 ) ) ;
#51604=CARTESIAN_POINT ( 'NONE',  ( -0.3392501089628019995, 0.1958661417322832277, -1.593175853018372612 ) ) ;
#51607=CARTESIAN_POINT ( 'NONE',  ( 0.1058382717557500713, -0.3949938075777409408, -1.817585301837270739 ) ) ;
#51609=DIRECTION ( 'NONE',  ( 0.000000000000000000, 0.000000000000000000, 1.000000000000000000 ) ) ;
#51612=CARTESIAN_POINT ( 'NONE',  ( 0.1998031496062994405, -0.3460692066303958092, -0.09186351706036746667 ) ) ;
#51619=CARTESIAN_POINT ( 'NONE',  ( 0.3917322834645669549, 0.1049643490035304660, -0.3667979002624672802 ) ) ;
#51627=CARTESIAN_POINT ( 'NONE',  ( -0.3996062992125986590, 0.1070741851644051723, -1.999343832020997525 ) ) ;
#51632=CARTESIAN_POINT ( 'NONE',  ( -0.2362204724409447953, -0.4091458600556404646, -0.8530183727034120755 ) ) ;
#51634=CARTESIAN_POINT ( 'NONE',  ( -0.1958661417322836718, 0.3392501089628017219, -0.1627296587926508609 ) ) ;
#51635=CARTESIAN_POINT ( 'NONE',  ( 0.3917322834645670104, 2.398668435337828261E-17, -2.092519685039370358 ) ) ;
#51639=CARTESIAN_POINT ( 'NONE',  ( 0.2362204724409451007, -0.4091458600556402980, -2.688320209973753538 ) ) ;
#51644=CARTESIAN_POINT ( 'NONE',  ( 0.3420746716998660508, -0.1974969037888704149, -2.543963254593176071 ) ) ;
#51652=CARTESIAN_POINT ( 'NONE',  ( -0.3917322834645669549, -0.1049643490035306603, -1.297900262467191590 ) ) ;
#51656=CARTESIAN_POINT ( 'NONE',  ( 0.3458507752293908943, 0.3458507752293908943, 0.1003937007874015769 ) ) ;
#51669=CARTESIAN_POINT ( 'NONE',  ( 0.2925321140481932369, -0.2925321140481931814, -0.9625984251968502381 ) ) ;
#51670=CARTESIAN_POINT ( 'NONE',  ( -0.3917322834645669549, -0.1049643490035306603, -2.492782152230970993 ) ) ;
#51681=CARTESIAN_POINT ( 'NONE',  ( 0.3392501089628018329, 0.1958661417322835607, -2.017735851214910170 ) ) ;
#51683=ADVANCED_FACE ( 'NONE', ( #57562 ), #46066, .T. ) ;
#51688=CARTESIAN_POINT ( 'NONE',  ( -0.1049643490035302024, -0.3917322834645671215, -1.889107611548556109 ) ) ;
#51693=CARTESIAN_POINT ( 'NONE',  ( 0.1070741851644054637, -0.3996062992125984925, -2.681758530183727451 ) ) ;
#51695=CARTESIAN_POINT ( 'NONE',  ( -0.2925321140481930704, -0.2925321140481933480, -1.318897637795275690 ) ) ;
#51698=CARTESIAN_POINT ( 'NONE',  ( 4.797336870675656522E-17, -0.3917322834645670659, -0.07547863336714100146 ) ) ;
#51709=EDGE_CURVE ( 'NONE', #83292, #49627, #8491, .T. ) ;
#51712=CARTESIAN_POINT ( 'NONE',  ( 0.2867679344610365999, 0.2867679344610365999, -0.1299212598425196485 ) ) ;
#51715=CARTESIAN_POINT ( 'NONE',  ( 0.1974969037888706369, -0.3420746716998659953, -0.5643044619422573627 ) ) ;
#51716=VERTEX_POINT ( 'NONE', #19507 ) ;
#51723=CARTESIAN_POINT ( 'NONE',  ( -0.1049643490035307158, 0.3917322834645670104, -1.578103305283151681 ) ) ;
#51729=CARTESIAN_POINT ( 'NONE',  ( -0.3460692066303960868, 0.1998031496062990242, -1.128608923884514503 ) ) ;
#51731=CARTESIAN_POINT ( 'NONE',  ( -0.1998031496062991630, -0.3460692066303959202, -0.7723097112860892732 ) ) ;
#51732=CARTESIAN_POINT ( 'NONE',  ( -0.1998031496062991630, -0.3460692066303959202, -0.2998687664041995160 ) ) ;
#51734=CARTESIAN_POINT ( 'NONE',  ( -0.2925321140481932924, 0.2925321140481931814, -2.854330708661417138 ) ) ;
#51736=CARTESIAN_POINT ( 'NONE',  ( -0.3917322834645671215, 0.1049643490035301469, -2.007217847769029007 ) ) ;
#51742=CARTESIAN_POINT ( 'NONE',  ( 5.785732909357575061E-17, -0.4724409448818898682, -1.572834645669291431 ) ) ;
#51745=CARTESIAN_POINT ( 'NONE',  ( -0.3420746716998662729, 0.1974969037888702206, -1.362860892388451539 ) ) ;
#51755=CARTESIAN_POINT ( 'NONE',  ( -9.787531504996566615E-17, 0.3996062992125985480, -1.966535433070866201 ) ) ;
#51757=CARTESIAN_POINT ( 'NONE',  ( 0.3917322834645669549, 2.398668435337827645E-17, -1.930426878443882943 ) ) ;
#51767=CARTESIAN_POINT ( 'NONE',  ( -0.1265901696524993347, 0.4724409448818896462, -2.368766404199475151 ) ) ;
#51770=CARTESIAN_POINT ( 'NONE',  ( -0.3996062992125986590, 0.1070741851644051723, 0.2053805774278214813 ) ) ;
#51772=CARTESIAN_POINT ( 'NONE',  ( 0.2867679344610365999, -0.2867679344610365444, -1.285433070866141669 ) ) ;
#51776=CARTESIAN_POINT ( 'NONE',  ( -0.3983403474834782965, -0.03178304480584832892, -1.220472440944881942 ) ) ;
#51793=CARTESIAN_POINT ( 'NONE',  ( -0.1958661417322836718, 0.3392501089628017219, -2.524934383202099397 ) ) ;
#51796=CARTESIAN_POINT ( 'NONE',  ( -0.1265901696524993347, 0.4724409448818895907, -0.6364829396325458744 ) ) ;
#51797=CARTESIAN_POINT ( 'NONE',  ( 0.3996062992125986035, 2.446882876249141962E-17, 0.03937007874015746589 ) ) ;
#51800=CARTESIAN_POINT ( 'NONE',  ( 0.1958661417322834775, 0.3392501089628018884, -1.711286089238845287 ) ) ;
#51804=CARTESIAN_POINT ( 'NONE',  ( 0.09156050430091122738, 0.3808816823641256732, -2.755905511811024056 ) ) ;
#51811=CARTESIAN_POINT ( 'NONE',  ( 0.1049643490035304522, -0.3917322834645668994, -1.267697219651231499 ) ) ;
#51818=CARTESIAN_POINT ( 'NONE',  ( 0.1049643490035304799, -0.3917322834645670104, -2.601725352527246127 ) ) ;
#51827=CARTESIAN_POINT ( 'NONE',  ( 0.1958661417322836440, -0.3392501089628017219, -1.908792650918635259 ) ) ;
#51844=CARTESIAN_POINT ( 'NONE',  ( -0.4091458600556405756, 0.2362204724409446288, -0.4179790026246719137 ) ) ;
#51847=CARTESIAN_POINT ( 'NONE',  ( 0.1974969037888706092, -0.3420746716998660508, -0.3261154855643044748 ) ) ;
#51852=CARTESIAN_POINT ( 'NONE',  ( -9.674558042662122972E-17, 0.3949938075777409963, -0.07677165354330710290 ) ) ;
#51859=CARTESIAN_POINT ( 'NONE',  ( 0.2925321140481932369, 0.2925321140481932369, -0.8444881889763780070 ) ) ;
#51861=CARTESIAN_POINT ( 'NONE',  ( -9.594673741351313045E-17, 0.3917322834645670104, -0.7795275590551180578 ) ) ;
#51865=CARTESIAN_POINT ( 'NONE',  ( 0.3458507752293908943, -0.3458507752293908943, -0.4901574803149605919 ) ) ;
#51878=CARTESIAN_POINT ( 'NONE',  ( 0.1265901696524989462, 0.4724409448818897572, -2.432414698162729039 ) ) ;
#51896=CARTESIAN_POINT ( 'NONE',  ( 0.3996062992125986035, -0.1070741851644053111, -0.2690288713910761187 ) ) ;
#51900=CARTESIAN_POINT ( 'NONE',  ( -0.3996062992125986035, -7.340648628747425578E-17, -2.716535433070865757 ) ) ;
#51901=CARTESIAN_POINT ( 'NONE',  ( -0.3949938075777409408, -0.1058382717557502933, -2.093175853018372834 ) ) ;
#51902=CARTESIAN_POINT ( 'NONE',  ( 0.1049643490035304938, -0.3917322834645669549, -0.3923884514435695414 ) ) ;
#51904=CARTESIAN_POINT ( 'NONE',  ( 0.1958661417322834775, 0.3392501089628018884, -1.081364829396325389 ) ) ;
#51906=CARTESIAN_POINT ( 'NONE',  ( -0.3917322834645671215, 0.1049643490035301469, -0.9698162729658791337 ) ) ;
#51908=CARTESIAN_POINT ( 'NONE',  ( -0.1958661417322834497, -0.3392501089628018884, 0.1693106543645162554 ) ) ;
#51914=CARTESIAN_POINT ( 'NONE',  ( -0.3460692066303958092, -0.1998031496062994683, -2.414698162729658648 ) ) ;
#51915=CARTESIAN_POINT ( 'NONE',  ( -0.3917322834645671770, 0.1049643490035302024, -1.289389394521996968 ) ) ;
#51923=CARTESIAN_POINT ( 'NONE',  ( -0.2867679344610365999, 0.2867679344610364889, -0.5767716535433071723 ) ) ;
#51931=CARTESIAN_POINT ( 'NONE',  ( 0.1265901696524989184, 0.4724409448818898127, -0.5426509186351704539 ) ) ;
#51932=CARTESIAN_POINT ( 'NONE',  ( 0.3917322834645669549, 0.1049643490035304660, -2.006561679790026531 ) ) ;
#51934=EDGE_LOOP ( 'NONE', ( #9934, #80737, #16994, #32370 ) ) ;
#51935=CARTESIAN_POINT ( 'NONE',  ( 0.1998031496062992740, 0.3460692066303959757, -0.1443569553805774397 ) ) ;
#51942=CARTESIAN_POINT ( 'NONE',  ( 0.3392501089628018329, 0.1958661417322835607, -0.6883202099737534274 ) ) ;
#51945=CARTESIAN_POINT ( 'NONE',  ( -0.3941128856533543945, -0.02500110684012597437, -1.929133858266767865 ) ) ;
#51948=ORIENTED_EDGE ( 'NONE', *, *, #14046, .F. ) ;
#51957=CARTESIAN_POINT ( 'NONE',  ( -0.2362204724409447953, -0.4091458600556404646, -2.504593175853018661 ) ) ;
#51961=CARTESIAN_POINT ( 'NONE',  ( 0.1958661417322834497, 0.3392501089628018329, -0.8543113928795783574 ) ) ;
#51969=CARTESIAN_POINT ( 'NONE',  ( -0.1958661417322836995, 0.3392501089628017219, -0.009861835466878533449 ) ) ;
#51974=CARTESIAN_POINT ( 'NONE',  ( 0.3458507752293908943, -0.3458507752293908943, -1.120078740157480324 ) ) ;
#51983=CARTESIAN_POINT ( 'NONE',  ( 0.000000000000000000, 0.000000000000000000, -1.220472440944881942 ) ) ;
#51988=VERTEX_POINT ( 'NONE', #2242 ) ;
#51989=CARTESIAN_POINT ( 'NONE',  ( -0.2925321140481932369, 0.2925321140481931259, -2.458661417322834719 ) ) ;
#51993=CARTESIAN_POINT ( 'NONE',  ( -0.3460692066303957537, -0.1998031496062994405, -1.861548556430446366 ) ) ;
#51999=CARTESIAN_POINT ( 'NONE',  ( 0.3996062992125985480, 2.446882876249141654E-17, -0.9822834645669291653 ) ) ;
#52000=CARTESIAN_POINT ( 'NONE',  ( 4.893765752498283924E-17, -0.3996062992125986035, -1.181102362204724310 ) ) ;
#52001=CARTESIAN_POINT ( 'NONE',  ( 0.2891555358219910499, 0.2891555358219910499, -0.6102362204724410821 ) ) ;
#52007=CARTESIAN_POINT ( 'NONE',  ( 0.1974969037888706092, -0.3420746716998660508, -1.585958005249344493 ) ) ;
#52012=CARTESIAN_POINT ( 'NONE',  ( -0.2362204724409451284, 0.4091458600556402425, -1.430446194225721834 ) ) ;
#52013=CARTESIAN_POINT ( 'NONE',  ( 0.3330030935778962586, -0.2065800153021633556, -2.755905511811022723 ) ) ;
#52020=CARTESIAN_POINT ( 'NONE',  ( 0.3917322834645668994, -0.1049643490035303134, -2.081345513614486276 ) ) ;
#52027=CARTESIAN_POINT ( 'NONE',  ( -0.3392501089628017219, -0.1958661417322836718, -1.461942257217847763 ) ) ;
#52030=CARTESIAN_POINT ( 'NONE',  ( 0.2891555358219910499, -0.2891555358219909944, -1.830708661417323135 ) ) ;
#52037=CARTESIAN_POINT ( 'NONE',  ( 0.2925321140481932369, 0.2925321140481932369, -0.6102362204724409711 ) ) ;
#52044=CARTESIAN_POINT ( 'NONE',  ( 0.1049643490035304938, -0.3917322834645669549, -0.4849081364829396779 ) ) ;
#52051=CARTESIAN_POINT ( 'NONE',  ( 0.3460692066303959202, -0.1998031496062991630, -1.914041994750656395 ) ) ;
#52055=CARTESIAN_POINT ( 'NONE',  ( -0.4724409448818898682, -8.678599364036362592E-17, -0.6692913385826770867 ) ) ;
#52057=CARTESIAN_POINT ( 'NONE',  ( -0.3917322834645669549, -0.1049643490035306603, -0.3530183727034120755 ) ) ;
#52058=CARTESIAN_POINT ( 'NONE',  ( -0.2867679344610364334, -0.2867679344610367109, -2.033464566929133799 ) ) ;
#52062=CARTESIAN_POINT ( 'NONE',  ( -0.3458507752293909498, 0.3458507752293907833, -2.616141732283464805 ) ) ;
#52066=CARTESIAN_POINT ( 'NONE',  ( 0.3949938075777408852, 0.1058382717557500435, -2.721128608923885306 ) ) ;
#52073=CARTESIAN_POINT ( 'NONE',  ( -0.3917322834645671215, 0.1049643490035301469, -1.599737532808399143 ) ) ;
#52076=CARTESIAN_POINT ( 'NONE',  ( 0.4091458600556403535, 0.2362204724409449896, 0.1069553805774278027 ) ) ;
#52088=CARTESIAN_POINT ( 'NONE',  ( -0.1070741851644056997, 0.3996062992125984925, -1.028215223097112663 ) ) ;
#52089=( BOUNDED_CURVE ( )  B_SPLINE_CURVE ( 2, ( #21043, #34505, #41637, #53839, #10076, #29007, #27766, #42047, #9250, #22285, #53431, #53005, #34084 ),
 .UNSPECIFIED., .F., .F. ) 
 B_SPLINE_CURVE_WITH_KNOTS ( ( 3, 2, 2, 2, 2, 2, 3 ),
 ( 0.7875000000000000888, 0.7916666666666667407, 0.7958333333333333925, 0.8000000000000000444, 0.8041666666666666963, 0.8083333333333333481, 0.8125000000000000000 ),
 .UNSPECIFIED. ) 
 CURVE ( )  GEOMETRIC_REPRESENTATION_ITEM ( )  RATIONAL_B_SPLINE_CURVE ( ( 0.9999999999999991118, 0.9659258262890692004, 1.000000000000000000, 0.9659258262890683122, 1.000000000000000000, 0.9659258262890683122, 1.000000000000000000, 0.9659258262890683122, 1.000000000000000000, 0.9659258262890683122, 1.000000000000000000, 0.9659258262890683122, 1.000000000000000000 ) ) 
 REPRESENTATION_ITEM ( '' )  );
#52090=CARTESIAN_POINT ( 'NONE',  ( -0.3392501089628017219, -0.1958661417322836718, -2.656824146981627166 ) ) ;
#52101=CARTESIAN_POINT ( 'NONE',  ( -0.3917322834645670659, -7.196005306013484475E-17, -2.555793593997062629 ) ) ;
#52108=CARTESIAN_POINT ( 'NONE',  ( -0.1049643490035307020, 0.3917322834645669549, -1.823490813648294129 ) ) ;
#52116=CARTESIAN_POINT ( 'NONE',  ( -0.1998031496062991907, -0.3460692066303959757, -1.325459317585301777 ) ) ;
#52118=CARTESIAN_POINT ( 'NONE',  ( -0.3917322834645671770, 0.1049643490035302024, 0.1279334401236726371 ) ) ;
#52131=CARTESIAN_POINT ( 'NONE',  ( -0.3392501089628019995, 0.1958661417322832277, -0.3333333333333333148 ) ) ;
#52134=CARTESIAN_POINT ( 'NONE',  ( -0.1974969037888706647, 0.3420746716998658843, -0.4855643044619423754 ) ) ;
#52138=CARTESIAN_POINT ( 'NONE',  ( -0.4724409448818899238, 0.1265901696524986964, -0.1902887139107611314 ) ) ;
#52149=CARTESIAN_POINT ( 'NONE',  ( -9.787531504996567848E-17, 0.3996062992125986035, -1.417322834645669216 ) ) ;
#52151=CARTESIAN_POINT ( 'NONE',  ( -0.1998031496062994405, 0.3460692066303957537, -0.7198162729658792447 ) ) ;
#52152=CARTESIAN_POINT ( 'NONE',  ( -9.787531504996566615E-17, 0.3996062992125985480, 0.08070866141732281618 ) ) ;
#52155=CARTESIAN_POINT ( 'NONE',  ( 0.3460692066303959757, -0.1998031496062991907, -2.624671916010498762 ) ) ;
#52156=CARTESIAN_POINT ( 'NONE',  ( -0.3392501089628019995, 0.1958661417322832277, -2.000656167979002920 ) ) ;
#52163=CARTESIAN_POINT ( 'NONE',  ( -1.157146581871515012E-16, 0.4724409448818898682, -1.651574803149606474 ) ) ;
#52166=CARTESIAN_POINT ( 'NONE',  ( -0.1058382717557497660, -0.3949938075777411073, -1.408792650918635259 ) ) ;
#52169=EDGE_CURVE ( 'NONE', #13953, #71224, #79692, .T. ) ;
#52177=CARTESIAN_POINT ( 'NONE',  ( -0.3996062992125984925, -0.1070741851644056858, -2.169947506561679340 ) ) ;
#52179=CARTESIAN_POINT ( 'NONE',  ( 0.3917322834645668994, -0.1049643490035303134, -2.081345513614486276 ) ) ;
#52192=CARTESIAN_POINT ( 'NONE',  ( 0.3996062992125985480, 2.446882876249141654E-17, -0.03740157480314962313 ) ) ;
#52194=CARTESIAN_POINT ( 'NONE',  ( -0.3917322834645669549, -0.1049643490035306603, -1.390419947506561504 ) ) ;
#52203=CARTESIAN_POINT ( 'NONE',  ( 5.785732909357575061E-17, -0.4724409448818898682, -2.598425196850393970 ) ) ;
#52216=CARTESIAN_POINT ( 'NONE',  ( -0.3392501089628019995, 0.1958661417322832277, -2.380577427821522374 ) ) ;
#52219=CARTESIAN_POINT ( 'NONE',  ( 0.1265901696524990294, -0.4724409448818896462, -0.5577427821522309426 ) ) ;
#52220=CARTESIAN_POINT ( 'NONE',  ( -0.3996062992125986035, -7.340648628747425578E-17, -0.1968503937007874405 ) ) ;
#52223=CARTESIAN_POINT ( 'NONE',  ( 4.797336870675656522E-17, -0.3917322834645670104, -1.645669291338582640 ) ) ;
#52234=CARTESIAN_POINT ( 'NONE',  ( 4.797336870675655290E-17, -0.3917322834645669549, -1.261135539861205412 ) ) ;
#52240=CARTESIAN_POINT ( 'NONE',  ( 0.2867679344610366554, -0.2867679344610365999, -2.614848712107298745 ) ) ;
#52248=CARTESIAN_POINT ( 'NONE',  ( 0.3917322834645670104, -0.1049643490035303411, -1.928477690288713742 ) ) ;
#52257=DIRECTION ( 'NONE',  ( 0.000000000000000000, 0.000000000000000000, 1.000000000000000000 ) ) ;
#52263=CARTESIAN_POINT ( 'NONE',  ( 5.785732909357575061E-17, -0.4724409448818898682, -0.3129921259842520231 ) ) ;
#52267=CARTESIAN_POINT ( 'NONE',  ( -0.3420746716998660508, -0.1974969037888706924, 0.02821522309711286050 ) ) ;
#52273=CARTESIAN_POINT ( 'NONE',  ( 0.1058382717557500852, -0.3949938075777408852, -0.1620734908136483021 ) ) ;
#52280=CARTESIAN_POINT ( 'NONE',  ( 4.893765752498283308E-17, -0.3996062992125985480, -1.100393700787401619 ) ) ;
#52282=CARTESIAN_POINT ( 'NONE',  ( 0.1958661417322834775, 0.3392501089628018884, -0.7664041994750655507 ) ) ;
#52297=CARTESIAN_POINT ( 'NONE',  ( 4.893765752498283308E-17, -0.3996062992125985480, 0.1594488188976377896 ) ) ;
#52313=CARTESIAN_POINT ( 'NONE',  ( -0.1070741851644051862, -0.3996062992125986590, -0.5446194225721784354 ) ) ;
#52314=CARTESIAN_POINT ( 'NONE',  ( 0.4724409448818897017, 0.1265901696524990294, -1.146325459317585116 ) ) ;
#52319=CARTESIAN_POINT ( 'NONE',  ( -0.3996062992125986035, -0.1070741851644056997, -2.565616797900262647 ) ) ;
#52320=CARTESIAN_POINT ( 'NONE',  ( 0.3949938075777411073, -0.1058382717557499464, -2.001312335958005395 ) ) ;
#52321=CARTESIAN_POINT ( 'NONE',  ( -0.2867679344610364334, -0.2867679344610367109, -0.6811023622047243098 ) ) ;
#52323=CARTESIAN_POINT ( 'NONE',  ( 0.2867679344610366554, 0.2867679344610366554, -1.074803149606299080 ) ) ;
#52325=CARTESIAN_POINT ( 'NONE',  ( -0.3392501089628019995, 0.1958661417322832277, -0.9632545931758529356 ) ) ;
#52327=CARTESIAN_POINT ( 'NONE',  ( -0.3949938075777409963, -7.255918531996591613E-17, -2.793307086614173151 ) ) ;
#52333=CARTESIAN_POINT ( 'NONE',  ( -0.3460692066303960868, 0.1998031496062990242, -2.388451443569553856 ) ) ;
#52334=CARTESIAN_POINT ( 'NONE',  ( 0.2867679344610366554, 0.2867679344610366554, -1.236895956201786717 ) ) ;
#52340=CARTESIAN_POINT ( 'NONE',  ( 0.1958661417322836440, -0.3392501089628017219, -0.4914698162729659869 ) ) ;
#52348=CARTESIAN_POINT ( 'NONE',  ( -0.1002886991216605655, -0.3788256970794443568, -1.929133858267718882 ) ) ;
#52349=CARTESIAN_POINT ( 'NONE',  ( -0.3917322834645669549, -0.1049643490035306603, -2.085301837270341352 ) ) ;
#52351=CARTESIAN_POINT ( 'NONE',  ( -0.2925321140481932924, 0.2925321140481931814, -0.1771653543307087075 ) ) ;
#52358=CARTESIAN_POINT ( 'NONE',  ( -0.3917322834645669549, -0.1049643490035306603, -0.7604986876640419391 ) ) ;
#52362=CARTESIAN_POINT ( 'NONE',  ( -0.3917864676224234177, -0.04037479286093467734, -1.929133858266767865 ) ) ;
#52377=CARTESIAN_POINT ( 'NONE',  ( -0.3917322834645668994, -0.1049643490035306742, -0.7558861960291846094 ) ) ;
#52380=CARTESIAN_POINT ( 'NONE',  ( -0.4724409448818899238, 0.1265901696524986964, -0.8202099737532806412 ) ) ;
#52386=CARTESIAN_POINT ( 'NONE',  ( -0.2867679344610367109, 0.2867679344610365444, -0.1739038302175346939 ) ) ;
#52389=CARTESIAN_POINT ( 'NONE',  ( -0.1265901696524993347, 0.4724409448818895907, -1.343175853018372834 ) ) ;
#52398=CARTESIAN_POINT ( 'NONE',  ( 0.3458507752293908943, 0.3458507752293908943, -2.104330708661417138 ) ) ;
#52404=CARTESIAN_POINT ( 'NONE',  ( 0.1070741851644053388, 0.3996062992125986035, -2.589895013123359568 ) ) ;
#52408=CARTESIAN_POINT ( 'NONE',  ( -9.787531504996566615E-17, 0.3996062992125985480, -1.809055118110236560 ) ) ;
#52414=CARTESIAN_POINT ( 'NONE',  ( 0.1070741851644054637, -0.3996062992125984925, -1.106955380577427706 ) ) ;
#52415=CARTESIAN_POINT ( 'NONE',  ( -0.2925321140481930704, -0.2925321140481933480, -1.161417322834645383 ) ) ;
#52416=CARTESIAN_POINT ( 'NONE',  ( 0.1058382717557499880, 0.3949938075777411073, -0.7808398950131234528 ) ) ;
#52422=CARTESIAN_POINT ( 'NONE',  ( -0.1058382717557503072, 0.3949938075777408852, -1.658136482939632339 ) ) ;
#52427=CARTESIAN_POINT ( 'NONE',  ( 0.1265901696524989462, 0.4724409448818897572, -2.040682414698162361 ) ) ;
#52435=CARTESIAN_POINT ( 'NONE',  ( 0.1958661417322836162, -0.3392501089628018329, -2.376621104165667298 ) ) ;
#52436=CARTESIAN_POINT ( 'NONE',  ( 0.1998031496062992463, 0.3460692066303959202, -2.740813648293963567 ) ) ;
#52441=CARTESIAN_POINT ( 'NONE',  ( -0.3917322834645669549, -7.196005306013483243E-17, -2.639088295766717884 ) ) ;
#52444=CARTESIAN_POINT ( 'NONE',  ( -0.3917322834645670104, -7.196005306013484475E-17, -2.078740157480314821 ) ) ;
#52447=CARTESIAN_POINT ( 'NONE',  ( 0.1974969037888706369, -0.3420746716998659953, -1.981627296587926690 ) ) ;
#52452=CARTESIAN_POINT ( 'NONE',  ( 0.1070741851644054915, -0.3996062992125986035, -0.4002624671916010235 ) ) ;
#52459=ADVANCED_FACE ( 'NONE', ( #35053, #63195 ), #11453, .F. ) ;
#52462=CARTESIAN_POINT ( 'NONE',  ( -9.594673741351313045E-17, 0.3917322834645670104, -0.5570866141732284671 ) ) ;
#52469=CARTESIAN_POINT ( 'NONE',  ( -0.2925321140481930149, -0.2925321140481933480, -1.868110236220472453 ) ) ;
#52472=CARTESIAN_POINT ( 'NONE',  ( 0.000000000000000000, 0.000000000000000000, 0.000000000000000000 ) ) ;
#52474=CARTESIAN_POINT ( 'NONE',  ( 0.3458507752293908943, 0.3458507752293908943, -1.082677165354330562 ) ) ;
#52476=CARTESIAN_POINT ( 'NONE',  ( 0.1049643490035304938, -0.3917322834645669549, -0.2349081364829396223 ) ) ;
#52477=CARTESIAN_POINT ( 'NONE',  ( -0.3917322834645671215, 0.1049643490035301469, -2.637139107611548461 ) ) ;
#52481=CARTESIAN_POINT ( 'NONE',  ( 0.1070741851644053388, 0.3996062992125986035, -0.2276902887139107545 ) ) ;
#52486=CARTESIAN_POINT ( 'NONE',  ( 0.3949938075777409963, 2.418639510665530743E-17, -2.557086614173228689 ) ) ;
#52493=CARTESIAN_POINT ( 'NONE',  ( 4.797336870675656522E-17, -0.3917322834645670104, -1.803149606299212726 ) ) ;
#52496=CARTESIAN_POINT ( 'NONE',  ( 0.4091458600556404646, -0.2362204724409448231, -0.02427821522309711946 ) ) ;
#52510=CARTESIAN_POINT ( 'NONE',  ( 0.3460692066303958092, 0.1998031496062993018, -1.152887139107611425 ) ) ;
#52511=CARTESIAN_POINT ( 'NONE',  ( -0.1958661417322836718, 0.3392501089628017219, -2.617454068241469756 ) ) ;
#52520=CARTESIAN_POINT ( 'NONE',  ( -0.2925321140481932924, 0.2925321140481931814, -0.01968503937007875029 ) ) ;
#52521=CARTESIAN_POINT ( 'NONE',  ( -0.3917322834645671770, 0.1049643490035302024, -2.391751599246406457 ) ) ;
#52529=CARTESIAN_POINT ( 'NONE',  ( -0.3917322834645671215, 0.1049643490035301469, -2.322178477690288734 ) ) ;
#52536=CARTESIAN_POINT ( 'NONE',  ( -0.1998031496062991907, -0.3460692066303959757, -1.482939632545931863 ) ) ;
#52538=CARTESIAN_POINT ( 'NONE',  ( -0.3392501089628019995, 0.1958661417322831999, 0.1344951199136988906 ) ) ;
#52549=CARTESIAN_POINT ( 'NONE',  ( -0.3392501089628019995, 0.1958661417322832277, -0.6482939632545930975 ) ) ;
#52552=CARTESIAN_POINT ( 'NONE',  ( 0.2891555358219910499, -0.2891555358219909944, -0.5708661417322835607 ) ) ;
#52567=STYLED_ITEM ( 'NONE', ( #58361 ), #31714 ) ;
#52568=CARTESIAN_POINT ( 'NONE',  ( 0.3996062992125986035, 0.1070741851644054776, -1.227034120734908029 ) ) ;
#52570=CARTESIAN_POINT ( 'NONE',  ( -0.3996062992125986590, 0.1070741851644051723, -0.8969816272965877024 ) ) ;
#52571=CARTESIAN_POINT ( 'NONE',  ( 0.1070741851644053388, 0.3996062992125986035, 0.08727034120734902811 ) ) ;
#52573=CARTESIAN_POINT ( 'NONE',  ( -0.1070741851644056997, 0.3996062992125986035, -2.841207349081364963 ) ) ;
#52574=CARTESIAN_POINT ( 'NONE',  ( 0.2867679344610365999, 0.2867679344610365999, -2.112204724409449064 ) ) ;
#52580=CARTESIAN_POINT ( 'NONE',  ( 0.3458507752293908943, -0.3458507752293908943, -1.907480314960629197 ) ) ;
#52583=CARTESIAN_POINT ( 'NONE',  ( -0.1974969037888704149, -0.3420746716998661063, -1.402230971128609172 ) ) ;
#52589=EDGE_CURVE ( 'NONE', #14913, #39936, #69192, .T. ) ;
#52595=CARTESIAN_POINT ( 'NONE',  ( 0.1070741851644054776, -0.3996062992125984925, -2.366797900262467280 ) ) ;
#52597=CARTESIAN_POINT ( 'NONE',  ( 0.2867679344610365999, 0.2867679344610365999, -2.265072547735221153 ) ) ;
#52611=CARTESIAN_POINT ( 'NONE',  ( -0.1998031496062994405, 0.3460692066303957537, -0.08989501312335958227 ) ) ;
#52613=CARTESIAN_POINT ( 'NONE',  ( -0.2867679344610365999, 0.2867679344610364889, -1.521653543307086354 ) ) ;
#52636=CARTESIAN_POINT ( 'NONE',  ( -0.3917322834645669549, -0.1049643490035306603, -2.557742782152230721 ) ) ;
#52639=CARTESIAN_POINT ( 'NONE',  ( -0.4724409448818895907, -0.1265901696524993070, -0.8333333333333332593 ) ) ;
#52640=CARTESIAN_POINT ( 'NONE',  ( -0.3460692066303960868, 0.1998031496062990242, 0.1312335958005249048 ) ) ;
#52643=CARTESIAN_POINT ( 'NONE',  ( 0.1958661417322834775, 0.3392501089628018884, -1.868766404199474929 ) ) ;
#52653=CARTESIAN_POINT ( 'NONE',  ( 0.3917322834645668994, -0.1049643490035303134, -1.136463623850706650 ) ) ;
#52659=CARTESIAN_POINT ( 'NONE',  ( 0.1049643490035303967, 0.3917322834645670659, -2.667342150427508773 ) ) ;
#52667=CARTESIAN_POINT ( 'NONE',  ( -9.594673741351313045E-17, 0.3917322834645670104, -1.659448818897637734 ) ) ;
#52671=CARTESIAN_POINT ( 'NONE',  ( -0.03757601356356682354, 0.4709442531824372113, -2.755905511811023612 ) ) ;
#52681=CARTESIAN_POINT ( 'NONE',  ( -0.2362204724409447953, -0.4091458600556404646, -0.1423884514435695414 ) ) ;
#52684=CARTESIAN_POINT ( 'NONE',  ( -0.3949938075777408852, -0.1058382717557502933, -0.1227034120734908501 ) ) ;
#52689=CARTESIAN_POINT ( 'NONE',  ( -0.1974969037888704149, -0.3420746716998661063, -0.1423884514435695414 ) ) ;
#52697=CARTESIAN_POINT ( 'NONE',  ( -0.3996062992125984925, -0.1070741851644056858, -0.7526246719160103460 ) ) ;
#52699=CARTESIAN_POINT ( 'NONE',  ( -0.3392501089628017219, -0.1958661417322836718, -0.5170603674540682482 ) ) ;
#52711=CARTESIAN_POINT ( 'NONE',  ( -0.3893108287682406909, 0.05073257145186435557, -1.220472440944881276 ) ) ;
#52714=CARTESIAN_POINT ( 'NONE',  ( -1.157146581871515012E-16, 0.4724409448818898682, -2.753937007874015741 ) ) ;
#52731=CARTESIAN_POINT ( 'NONE',  ( -0.3996062992125986590, 0.1070741851644051862, -0.9776902887139107268 ) ) ;
#52737=CARTESIAN_POINT ( 'NONE',  ( -0.3460692066303958092, -0.1998031496062994683, -2.572178477690288734 ) ) ;
#52738=CARTESIAN_POINT ( 'NONE',  ( 0.3420746716998660508, -0.1974969037888703871, -1.837270341207348556 ) ) ;
#52740=CARTESIAN_POINT ( 'NONE',  ( 4.797336870675656522E-17, -0.3917322834645670104, -0.5433070866141732624 ) ) ;
#52744=CARTESIAN_POINT ( 'NONE',  ( -0.1958661417322836718, 0.3392501089628017219, -1.265091863517060489 ) ) ;
#52747=CARTESIAN_POINT ( 'NONE',  ( 0.3392501089628018329, -0.1958661417322834497, -0.02753973933627114692 ) ) ;
#52752=CARTESIAN_POINT ( 'NONE',  ( 0.1265901696524989184, 0.4724409448818898127, -0.07020997375328084933 ) ) ;
#52753=CARTESIAN_POINT ( 'NONE',  ( 0.1998031496062994405, -0.3460692066303958092, -2.769028871391076230 ) ) ;
#52754=CARTESIAN_POINT ( 'NONE',  ( 0.3917322834645670659, -0.1049643490035303273, -1.210649237041681703 ) ) ;
#52760=CARTESIAN_POINT ( 'NONE',  ( -0.3392501089628017219, -0.1958661417322836718, -0.6095800524934383846 ) ) ;
#52768=CARTESIAN_POINT ( 'NONE',  ( 0.09865214182602936865, -0.3796925558542994517, -1.929133858267717549 ) ) ;
#52770=CARTESIAN_POINT ( 'NONE',  ( -0.1049643490035307020, 0.3917322834645669549, -1.888451443569553412 ) ) ;
#52772=CARTESIAN_POINT ( 'NONE',  ( -0.3996062992125986035, -7.340648628747425578E-17, -0.5118110236220472231 ) ) ;
#52773=ORIENTED_EDGE ( 'NONE', *, *, #81291, .F. ) ;
#52778=CARTESIAN_POINT ( 'NONE',  ( -0.3458507752293906723, -0.3458507752293910609, -1.161417322834645605 ) ) ;
#52779=CARTESIAN_POINT ( 'NONE',  ( -0.1049643490035307020, 0.3917322834645669549, -0.7211286089238846397 ) ) ;
#52794=ORIENTED_EDGE ( 'NONE', *, *, #82467, .F. ) ;
#52799=CARTESIAN_POINT ( 'NONE',  ( -0.1958661417322834497, -0.3392501089628018884, -0.6180909204386334510 ) ) ;
#52808=CARTESIAN_POINT ( 'NONE',  ( -0.1049643490035307158, 0.3917322834645670104, -0.1607804706374822146 ) ) ;
#52810=CARTESIAN_POINT ( 'NONE',  ( 5.785732909357575061E-17, -0.4724409448818898682, -0.2362204724409449064 ) ) ;
#52811=CARTESIAN_POINT ( 'NONE',  ( -0.2362204724409447953, -0.4091458600556404646, -1.559711286089238591 ) ) ;
#52826=CARTESIAN_POINT ( 'NONE',  ( -0.2925321140481930149, -0.2925321140481933480, -2.655511811023622215 ) ) ;
#52831=CARTESIAN_POINT ( 'NONE',  ( -0.3996062992125986590, 0.1070741851644051723, -1.999343832020997525 ) ) ;
#52836=CARTESIAN_POINT ( 'NONE',  ( 4.893765752498283308E-17, -0.3996062992125985480, -1.100393700787401619 ) ) ;
#52838=CARTESIAN_POINT ( 'NONE',  ( -0.1998031496062991907, -0.3460692066303959757, -1.482939632545931863 ) ) ;
#52839=CARTESIAN_POINT ( 'NONE',  ( -0.3949938075777411628, 0.1058382717557497937, -0.6627296587926508886 ) ) ;
#52845=CARTESIAN_POINT ( 'NONE',  ( 4.837279021331061486E-17, -0.3949938075777409963, -1.572834645669291875 ) ) ;
#52850=CARTESIAN_POINT ( 'NONE',  ( -0.3458507752293906723, -0.3458507752293910609, -1.948818897637795144 ) ) ;
#52851=CARTESIAN_POINT ( 'NONE',  ( 0.1614515132151791432, -0.3594585737333411690, -2.755905511811025388 ) ) ;
#52858=CARTESIAN_POINT ( 'NONE',  ( -0.3917322834645668994, -0.1049643490035306742, -2.330689345635483356 ) ) ;
#52864=CARTESIAN_POINT ( 'NONE',  ( 0.2867679344610365999, -0.2867679344610365999, -2.855623728837584085 ) ) ;
#52866=CARTESIAN_POINT ( 'NONE',  ( -9.594673741351313045E-17, 0.3917322834645670104, -1.881889763779527769 ) ) ;
#52868=ORIENTED_EDGE ( 'NONE', *, *, #23484, .T. ) ;
#52869=CARTESIAN_POINT ( 'NONE',  ( 0.3949938075777409408, 0.1058382717557500574, -2.171916010498687655 ) ) ;
#52874=CARTESIAN_POINT ( 'NONE',  ( 0.3996062992125986590, -0.1070741851644053111, -0.7414698162729659314 ) ) ;
#52881=CARTESIAN_POINT ( 'NONE',  ( -0.1958661417322836718, 0.3392501089628017219, -0.5702099737532808632 ) ) ;
#52886=VERTEX_POINT ( 'NONE', #80830 ) ;
#52891=CARTESIAN_POINT ( 'NONE',  ( 0.4724409448818897572, -0.1265901696524988906, -1.213910761154855189 ) ) ;
#52893=CARTESIAN_POINT ( 'NONE',  ( 0.2867679344610365999, -0.2867679344610365444, -0.2480314960629920740 ) ) ;
#52894=CARTESIAN_POINT ( 'NONE',  ( 0.1049643490035303689, 0.3917322834645670104, -2.282808398950130879 ) ) ;
#52897=CARTESIAN_POINT ( 'NONE',  ( -0.1998031496062994405, 0.3460692066303957537, -0.2473753280839895152 ) ) ;
#52902=CARTESIAN_POINT ( 'NONE',  ( 0.2891555358219910499, -0.2891555358219909944, -2.852362204724409267 ) ) ;
#52904=CARTESIAN_POINT ( 'NONE',  ( -0.1049643490035307020, 0.3917322834645669549, -0.09120734908136493568 ) ) ;
#52909=CARTESIAN_POINT ( 'NONE',  ( 0.1958661417322834775, 0.3392501089628018884, -1.711286089238845287 ) ) ;
#52912=CARTESIAN_POINT ( 'NONE',  ( -0.4724409448818898682, -8.678599364036362592E-17, -0.2736220472440945017 ) ) ;
#52926=CARTESIAN_POINT ( 'NONE',  ( 0.3996062992125984925, 0.1070741851644054637, -1.146325459317585116 ) ) ;
#52927=EDGE_CURVE ( 'NONE', #5969, #55042, #77293, .T. ) ;
#52928=CARTESIAN_POINT ( 'NONE',  ( 0.3392501089628018329, 0.1958661417322835607, -2.735564304461941987 ) ) ;
#52937=CARTESIAN_POINT ( 'NONE',  ( 0.3996062992125986035, 0.1070741851644054776, -0.1246719160104987068 ) ) ;
#52938=CARTESIAN_POINT ( 'NONE',  ( 0.1049643490035303967, 0.3917322834645670659, -2.667342150427508773 ) ) ;
#52943=CARTESIAN_POINT ( 'NONE',  ( 0.3392501089628018329, 0.1958661417322835607, -2.578083989501311901 ) ) ;
#52948=CARTESIAN_POINT ( 'NONE',  ( -0.3996062992125986035, -7.340648628747425578E-17, -2.086614173228346303 ) ) ;
#52950=CARTESIAN_POINT ( 'NONE',  ( -0.1070741851644051862, -0.3996062992125987146, -1.646981627296587591 ) ) ;
#52952=CARTESIAN_POINT ( 'NONE',  ( -0.3917322834645670659, -7.196005306013484475E-17, -0.1935888695876134269 ) ) ;
#52965=CARTESIAN_POINT ( 'NONE',  ( 0.1958661417322834775, 0.3392501089628018884, -0.7664041994750655507 ) ) ;
#52968=CARTESIAN_POINT ( 'NONE',  ( -0.3949938075777409963, -7.255918531996591613E-17, -0.6692913385826770867 ) ) ;
#52979=DIRECTION ( 'NONE',  ( 0.000000000000000000, 0.000000000000000000, 1.000000000000000000 ) ) ;
#52980=CARTESIAN_POINT ( 'NONE',  ( -0.1265901696524986964, -0.4724409448818899238, -2.749343832020996636 ) ) ;
#52984=CARTESIAN_POINT ( 'NONE',  ( 0.1070741851644053527, 0.3996062992125986590, -1.095800524934382958 ) ) ;
#52986=CARTESIAN_POINT ( 'NONE',  ( 0.2925321140481932369, 0.2925321140481932369, -0.6870078740157479213 ) ) ;
#52987=CARTESIAN_POINT ( 'NONE',  ( -9.787531504996566615E-17, 0.3996062992125985480, -0.7066929133858268486 ) ) ;
#52989=CARTESIAN_POINT ( 'NONE',  ( 0.3460692066303959757, -0.1998031496062991907, -2.939632545931758489 ) ) ;
#52990=CARTESIAN_POINT ( 'NONE',  ( -9.594673741351313045E-17, 0.3917322834645670104, -2.131889763779527769 ) ) ;
#52996=CARTESIAN_POINT ( 'NONE',  ( -0.1265901696524986964, -0.4724409448818899238, -1.723753280839894986 ) ) ;
#52999=CARTESIAN_POINT ( 'NONE',  ( 0.3949938075777408852, 0.1058382717557500435, -1.303805774278215424 ) ) ;
#53005=CARTESIAN_POINT ( 'NONE',  ( -0.4724409448818899238, 0.1265901696524986964, -2.314304461942256808 ) ) ;
#53009=CARTESIAN_POINT ( 'NONE',  ( 0.3996062992125984925, 0.1070741851644054637, -2.721128608923884418 ) ) ;
#53010=( BOUNDED_CURVE ( )  B_SPLINE_CURVE ( 1, ( #78798, #52671 ),
 .UNSPECIFIED., .F., .F. ) 
 B_SPLINE_CURVE_WITH_KNOTS ( ( 2, 2 ),
 ( 0.000000000000000000, 0.001849999999999999648 ),
 .UNSPECIFIED. ) 
 CURVE ( )  GEOMETRIC_REPRESENTATION_ITEM ( )  RATIONAL_B_SPLINE_CURVE ( ( 0.9911642120908024101, 0.9911642120908024101 ) ) 
 REPRESENTATION_ITEM ( '' )  );
#53011=CARTESIAN_POINT ( 'NONE',  ( -0.1958661417322834497, -0.3392501089628018884, -1.877933440123672471 ) ) ;
#53026=CARTESIAN_POINT ( 'NONE',  ( -0.1958661417322836718, 0.3392501089628017219, -1.515091863517060489 ) ) ;
#53036=CARTESIAN_POINT ( 'NONE',  ( 0.2925321140481932369, -0.2925321140481931814, -0.8051181102362205966 ) ) ;
#53049=CARTESIAN_POINT ( 'NONE',  ( -9.594673741351313045E-17, 0.3917322834645670104, -2.511811023622047223 ) ) ;
#53052=CARTESIAN_POINT ( 'NONE',  ( -0.1070741851644056997, 0.3996062992125986035, -0.6364829396325458744 ) ) ;
#53055=CARTESIAN_POINT ( 'NONE',  ( -0.2867679344610364334, -0.2867679344610367109, -1.940944881889763884 ) ) ;
#53062=FACE_OUTER_BOUND ( 'NONE', #64869, .T. ) ;
#53067=CARTESIAN_POINT ( 'NONE',  ( 0.1958661417322834497, 0.3392501089628018329, -1.011791707840208332 ) ) ;
#53073=CARTESIAN_POINT ( 'NONE',  ( -9.594673741351313045E-17, 0.3917322834645670659, -2.673903830217533972 ) ) ;
#53081=CARTESIAN_POINT ( 'NONE',  ( -0.3917322834645671215, 0.1049643490035301469, -2.007217847769029007 ) ) ;
#53084=PRODUCT_DEFINITION_FORMATION_WITH_SPECIFIED_SOURCE ( 'ANY', '', #72209, .NOT_KNOWN. ) ;
#53090=CARTESIAN_POINT ( 'NONE',  ( -0.3996062992125987146, 0.1070741851644051862, -1.922572178477689908 ) ) ;
#53092=EDGE_CURVE ( 'NONE', #29367, #55042, #25200, .T. ) ;
#53097=CARTESIAN_POINT ( 'NONE',  ( -0.2362204724409447953, -0.4091458600556404646, -0.6148293963254594097 ) ) ;
#53101=CARTESIAN_POINT ( 'NONE',  ( -0.2891555358219909388, -0.2891555358219912164, -0.1358267716535433156 ) ) ;
#53106=CARTESIAN_POINT ( 'NONE',  ( 0.3949938075777409408, -0.1058382717557499186, -0.5032808398950131545 ) ) ;
#53113=CARTESIAN_POINT ( 'NONE',  ( 0.1998031496062992463, 0.3460692066303959202, -1.166010498687663821 ) ) ;
#53115=CARTESIAN_POINT ( 'NONE',  ( -0.2867679344610364334, -0.2867679344610367109, -0.8385826771653541734 ) ) ;
#53129=CARTESIAN_POINT ( 'NONE',  ( 0.4091458600556403535, 0.2362204724409449896, -2.727690288713910949 ) ) ;
#53145=CARTESIAN_POINT ( 'NONE',  ( -0.2925321140481932369, 0.2925321140481931814, -0.9645669291338581086 ) ) ;
#53150=CARTESIAN_POINT ( 'NONE',  ( -0.2925321140481932924, 0.2925321140481931814, -2.696850393700787052 ) ) ;
#53151=CARTESIAN_POINT ( 'NONE',  ( 0.3949938075777409963, 2.418639510665530435E-17, -1.850393700787401396 ) ) ;
#53152=CARTESIAN_POINT ( 'NONE',  ( -0.3917322834645670104, -7.196005306013484475E-17, -0.5039370078740157410 ) ) ;
#53155=CARTESIAN_POINT ( 'NONE',  ( -0.2867679344610364334, -0.2867679344610367109, -1.153543307086613900 ) ) ;
#53158=CARTESIAN_POINT ( 'NONE',  ( 0.1958661417322836162, -0.3392501089628018329, -0.01441637975621864153 ) ) ;
#53165=CARTESIAN_POINT ( 'NONE',  ( 0.3996062992125986035, 0.1070741851644054776, -2.486876640419947382 ) ) ;
#53166=CARTESIAN_POINT ( 'NONE',  ( -0.2867679344610365444, -0.2867679344610367664, -1.000675483760841811 ) ) ;
#53171=CARTESIAN_POINT ( 'NONE',  ( -0.3392501089628019995, 0.1958661417322832277, -0.4258530183727035068 ) ) ;
#53179=CARTESIAN_POINT ( 'NONE',  ( -0.3401783215940975547, -0.1988659768061105948, -1.929133858267717105 ) ) ;
#53180=CARTESIAN_POINT ( 'NONE',  ( 0.1049643490035304938, -0.3917322834645669549, -1.809711286089239035 ) ) ;
#53182=CARTESIAN_POINT ( 'NONE',  ( -0.1998031496062991907, -0.3460692066303959757, -0.3805774278215223183 ) ) ;
#53189=CARTESIAN_POINT ( 'NONE',  ( 0.4091458600556404646, -0.2362204724409448231, -0.02427821522309711946 ) ) ;
#53191=CARTESIAN_POINT ( 'NONE',  ( 0.1049643490035304938, -0.3917322834645669549, -1.272309711286089273 ) ) ;
#53196=ORIENTED_EDGE ( 'NONE', *, *, #65648, .F. ) ;
#53213=CARTESIAN_POINT ( 'NONE',  ( -0.3392501089628019439, 0.1958661417322832554, -1.208642101540995606 ) ) ;
#53223=CARTESIAN_POINT ( 'NONE',  ( -0.1958661417322833942, -0.3392501089628018884, -0.2198355887477184134 ) ) ;
#53225=CARTESIAN_POINT ( 'NONE',  ( -0.4724409448818898682, -8.678599364036362592E-17, -0.5885826771653542844 ) ) ;
#53226=CARTESIAN_POINT ( 'NONE',  ( -0.3458507752293909498, 0.3458507752293907833, -1.828740157480315265 ) ) ;
#53242=CARTESIAN_POINT ( 'NONE',  ( 0.1998031496062992463, 0.3460692066303959202, -2.740813648293963567 ) ) ;
#53248=CARTESIAN_POINT ( 'NONE',  ( -0.3996062992125986590, 0.1070741851644051723, -1.684383202099737575 ) ) ;
#53251=AXIS2_PLACEMENT_3D ( 'NONE', #57851, #13682, #65022 ) ;
#53255=CARTESIAN_POINT ( 'NONE',  ( -0.1998031496062991630, -0.3460692066303959202, -0.9297900262467192478 ) ) ;
#53256=CARTESIAN_POINT ( 'NONE',  ( 0.3460692066303959202, 0.1998031496062993295, -1.548556430446194287 ) ) ;
#53258=CARTESIAN_POINT ( 'NONE',  ( -0.2891555358219911054, 0.2891555358219909388, -0.8070866141732284671 ) ) ;
#53263=CARTESIAN_POINT ( 'NONE',  ( 0.1058382717557499880, 0.3949938075777409408, -1.645013123359580831 ) ) ;
#53268=CARTESIAN_POINT ( 'NONE',  ( 0.2362204724409449064, 0.4091458600556404646, -2.034120734908136718 ) ) ;
#53269=CARTESIAN_POINT ( 'NONE',  ( 0.3859888145977959928, 0.06766049032611561043, -2.755905511811024056 ) ) ;
#53277=CARTESIAN_POINT ( 'NONE',  ( -0.3392501089628018329, -0.1958661417322836440, -2.337251025425510331 ) ) ;
#53283=CARTESIAN_POINT ( 'NONE',  ( 0.3917322834645670104, 2.398668435337828261E-17, 0.1122047244094487306 ) ) ;
#53285=CARTESIAN_POINT ( 'NONE',  ( 0.3917322834645670104, -0.1049643490035303411, -1.678477690288713964 ) ) ;
#53288=CARTESIAN_POINT ( 'NONE',  ( -0.2891555358219908833, -0.2891555358219912164, -2.263779527559055094 ) ) ;
#53293=CARTESIAN_POINT ( 'NONE',  ( -0.3996062992125987146, 0.1070741851644051862, -0.5052493438320209140 ) ) ;
#53297=SURFACE_STYLE_USAGE ( .BOTH. , #45311 ) ;
#53298=CARTESIAN_POINT ( 'NONE',  ( -0.3917322834645671215, 0.1049643490035301469, 0.1975065616797899160 ) ) ;
#53300=CARTESIAN_POINT ( 'NONE',  ( 0.3917322834645669549, 0.1049643490035304660, -0.6817585301837268963 ) ) ;
#53311=CARTESIAN_POINT ( 'NONE',  ( -0.4724409448818895907, -0.1265901696524993070, -1.148293963254592986 ) ) ;
#53313=CARTESIAN_POINT ( 'NONE',  ( -0.3392501089628017219, -0.1958661417322836718, -0.5170603674540682482 ) ) ;
#53315=CARTESIAN_POINT ( 'NONE',  ( 0.2867679344610366554, 0.2867679344610366554, -2.584645669291338876 ) ) ;
#53320=CARTESIAN_POINT ( 'NONE',  ( 0.3996062992125986035, -0.1070741851644052972, -0.1883202099737532609 ) ) ;
#53326=CARTESIAN_POINT ( 'NONE',  ( 0.1958661417322834497, 0.3392501089628018329, 0.09057049688420130973 ) ) ;
#53328=CARTESIAN_POINT ( 'NONE',  ( -0.3917322834645669549, -0.1049643490035306603, -0.1305774278215224016 ) ) ;
#53333=CARTESIAN_POINT ( 'NONE',  ( 0.1049643490035303689, 0.3917322834645670104, -1.717847769028871596 ) ) ;
#53338=CARTESIAN_POINT ( 'NONE',  ( 0.4724409448818898682, 2.892866454678787531E-17, -0.3523622047244094335 ) ) ;
#53351=CARTESIAN_POINT ( 'NONE',  ( 4.893765752498283308E-17, -0.3996062992125985480, -1.415354330708661346 ) ) ;
#53352=CARTESIAN_POINT ( 'NONE',  ( -0.3917322834645670104, -7.196005306013484475E-17, -2.486220472440944906 ) ) ;
#53359=CARTESIAN_POINT ( 'NONE',  ( 0.03178304480586199854, -0.3983403474834772418, -9.560572922657961637E-16 ) ) ;
#53361=CARTESIAN_POINT ( 'NONE',  ( -0.3460692066303960868, 0.1998031496062990242, -0.02624671916010499692 ) ) ;
#53362=CARTESIAN_POINT ( 'NONE',  ( -0.3392501089628019995, 0.1958661417322831999, -2.700150549377639653 ) ) ;
#53367=CARTESIAN_POINT ( 'NONE',  ( 0.2867679344610365999, -0.2867679344610365444, -2.545275590551181022 ) ) ;
#53377=CARTESIAN_POINT ( 'NONE',  ( 0.3392501089628018329, 0.1958661417322835607, -0.2854523866479808936 ) ) ;
#53391=CARTESIAN_POINT ( 'NONE',  ( -0.1958661417322836718, 0.3392501089628017219, -0.7926509186351704539 ) ) ;
#53394=CARTESIAN_POINT ( 'NONE',  ( 0.1058382717557500713, -0.3949938075777409408, -1.030183727034120755 ) ) ;
#53410=CARTESIAN_POINT ( 'NONE',  ( 0.3996062992125986035, 0.1070741851644054776, -1.541994750656167978 ) ) ;
#53411=CARTESIAN_POINT ( 'NONE',  ( 0.3460692066303958092, 0.1998031496062993018, -1.152887139107611425 ) ) ;
#53412=CARTESIAN_POINT ( 'NONE',  ( 0.2925321140481932369, 0.2925321140481932369, -0.3720472440944882497 ) ) ;
#53414=CARTESIAN_POINT ( 'NONE',  ( 0.3458507752293908943, 0.3458507752293908943, 0.01968503937007874335 ) ) ;
#53415=CARTESIAN_POINT ( 'NONE',  ( -0.3392501089628017219, -0.1958661417322836718, -2.184383202099737797 ) ) ;
#53421=CARTESIAN_POINT ( 'NONE',  ( 0.2362204724409451007, -0.4091458600556402980, -1.900918635170603554 ) ) ;
#53425=CARTESIAN_POINT ( 'NONE',  ( -0.3949938075777409963, -7.255918531996591613E-17, -1.218503937007874072 ) ) ;
#53431=CARTESIAN_POINT ( 'NONE',  ( -0.4091458600556405756, 0.2362204724409446288, -2.307742782152230721 ) ) ;
#53435=CARTESIAN_POINT ( 'NONE',  ( -0.3460692066303960313, 0.1998031496062989965, -2.622703412073490892 ) ) ;
#53436=CARTESIAN_POINT ( 'NONE',  ( -9.594673741351310580E-17, 0.3917322834645669549, -1.969796957184039909 ) ) ;
#53448=CARTESIAN_POINT ( 'NONE',  ( -0.2925321140481932369, 0.2925321140481931259, -0.4114173228346455491 ) ) ;
#53450=CARTESIAN_POINT ( 'NONE',  ( -0.3392501089628017219, -0.1958661417322836718, -1.239501312335958172 ) ) ;
#53459=CARTESIAN_POINT ( 'NONE',  ( 0.1070741851644053388, 0.3996062992125986035, -0.8576115485564304031 ) ) ;
#53471=CARTESIAN_POINT ( 'NONE',  ( -0.3392501089628017219, -0.1958661417322836718, -2.721784776902886893 ) ) ;
#53474=CARTESIAN_POINT ( 'NONE',  ( 0.3996062992125986035, 0.1070741851644054776, -0.4396325459317584339 ) ) ;
#53477=CARTESIAN_POINT ( 'NONE',  ( 0.2867679344610365999, 0.2867679344610365999, -2.334645669291338432 ) ) ;
#53484=CARTESIAN_POINT ( 'NONE',  ( 5.785732909357575061E-17, -0.4724409448818898682, -2.045275590551181022 ) ) ;
#53488=CARTESIAN_POINT ( 'NONE',  ( 0.2867679344610365999, 0.2867679344610365999, -1.635151287892701255 ) ) ;
#53495=CARTESIAN_POINT ( 'NONE',  ( -0.1958661417322833942, -0.3392501089628018884, -2.739520628117797063 ) ) ;
#53505=CARTESIAN_POINT ( 'NONE',  ( -0.3392501089628017219, -0.1958661417322836718, -1.869422572178477848 ) ) ;
#53514=CARTESIAN_POINT ( 'NONE',  ( -9.787531504996567848E-17, 0.3996062992125986035, -2.047244094488188892 ) ) ;
#53516=EDGE_CURVE ( 'NONE', #63931, #37370, #5442, .T. ) ;
#53520=CARTESIAN_POINT ( 'NONE',  ( 0.4091458600556404646, -0.2362204724409448231, -0.8116797900262466836 ) ) ;
#53523=CARTESIAN_POINT ( 'NONE',  ( 0.1974969037888706092, -0.3420746716998660508, -0.1686351706036745279 ) ) ;
#53528=CARTESIAN_POINT ( 'NONE',  ( 0.3420746716998660508, -0.1974969037888704149, -0.6541994750656167090 ) ) ;
#53532=CARTESIAN_POINT ( 'NONE',  ( 5.785732909357575061E-17, -0.4724409448818898682, -0.1555118110236220763 ) ) ;
#53535=CARTESIAN_POINT ( 'NONE',  ( -0.1998031496062994405, 0.3460692066303957537, -1.507217847769029007 ) ) ;
#53537=CARTESIAN_POINT ( 'NONE',  ( 0.2867679344610365999, -0.2867679344610365444, -0.8779527559055116948 ) ) ;
#53539=CARTESIAN_POINT ( 'NONE',  ( -0.4724409448818898682, -8.678599364036362592E-17, -2.320866141732283783 ) ) ;
#53550=CARTESIAN_POINT ( 'NONE',  ( -0.2362204724409451284, 0.4091458600556402425, -2.767060367454068359 ) ) ;
#53566=CARTESIAN_POINT ( 'NONE',  ( 0.1070741851644054915, -0.3996062992125985480, -0.7152230971128609172 ) ) ;
#53570=CARTESIAN_POINT ( 'NONE',  ( 0.3460692066303959757, -0.1998031496062991907, -2.467191601049868677 ) ) ;
#53571=CARTESIAN_POINT ( 'NONE',  ( -0.3949938075777411628, 0.1058382717557497937, -2.395013123359580387 ) ) ;
#53573=CARTESIAN_POINT ( 'NONE',  ( -0.2867679344610364334, -0.2867679344610367109, -0.9960629921259842590 ) ) ;
#53576=CARTESIAN_POINT ( 'NONE',  ( -0.3392501089628017219, -0.1958661417322836718, -1.146981627296587813 ) ) ;
#53578=CARTESIAN_POINT ( 'NONE',  ( 0.3392501089628018329, -0.1958661417322834497, 0.1299405756243587895 ) ) ;
#53584=CARTESIAN_POINT ( 'NONE',  ( -0.3460692066303960868, 0.1998031496062990242, -2.545931758530183497 ) ) ;
#53585=CARTESIAN_POINT ( 'NONE',  ( 0.1958661417322834775, 0.3392501089628018884, -1.400937950952442668 ) ) ;
#53591=CARTESIAN_POINT ( 'NONE',  ( 0.2867679344610365999, -0.2867679344610365444, -0.6555118110236222151 ) ) ;
#53599=CARTESIAN_POINT ( 'NONE',  ( -0.2881610400570164265, -0.2661962643049016197, -1.929133858267716883 ) ) ;
#53600=CARTESIAN_POINT ( 'NONE',  ( -9.594673741351313045E-17, 0.3917322834645670104, -2.354330708661417138 ) ) ;
#53602=CARTESIAN_POINT ( 'NONE',  ( 0.1070741851644054915, -0.3996062992125986035, -0.4002624671916010235 ) ) ;
#53608=CARTESIAN_POINT ( 'NONE',  ( 0.03757601356357168076, -0.4709442531824368783, -4.620136098463503353E-16 ) ) ;
#53610=CARTESIAN_POINT ( 'NONE',  ( 4.797336870675656522E-17, -0.3917322834645670104, -1.423228346456693050 ) ) ;
#53611=CARTESIAN_POINT ( 'NONE',  ( -0.3986795681650724954, -0.0008564280373882149269, -1.929133858267715551 ) ) ;
#53619=CARTESIAN_POINT ( 'NONE',  ( 0.3460692066303959202, -0.1998031496062991630, -2.071522309711286258 ) ) ;
#53629=CARTESIAN_POINT ( 'NONE',  ( -0.1958661417322836440, 0.3392501089628016664, -1.352999056921573295 ) ) ;
#53632=CARTESIAN_POINT ( 'NONE',  ( -0.3917322834645669549, -0.1049643490035306603, -1.075459317585301777 ) ) ;
#53639=CARTESIAN_POINT ( 'NONE',  ( -0.1958661417322833942, -0.3392501089628018884, -0.06235527378708850127 ) ) ;
#53642=CARTESIAN_POINT ( 'NONE',  ( -0.2362204724409447953, -0.4091458600556404646, -0.2230971128608923715 ) ) ;
#53643=CARTESIAN_POINT ( 'NONE',  ( -0.4724409448818895907, -0.1265901696524993070, -1.540026246719159886 ) ) ;
#53658=CARTESIAN_POINT ( 'NONE',  ( -0.1974969037888704149, -0.3420746716998661063, 0.1725721784776902690 ) ) ;
#53664=CARTESIAN_POINT ( 'NONE',  ( -0.3460692066303960313, 0.1998031496062989965, -1.677821522309711488 ) ) ;
#53669=CARTESIAN_POINT ( 'NONE',  ( -0.3996062992125985480, -7.340648628747423112E-17, -0.9035433070866141225 ) ) ;
#53670=CARTESIAN_POINT ( 'NONE',  ( 0.1998031496062992740, 0.3460692066303959757, -1.246719160104986734 ) ) ;
#53671=CARTESIAN_POINT ( 'NONE',  ( 4.837279021331060870E-17, -0.3949938075777409963, -1.023622047244094446 ) ) ;
#53672=CARTESIAN_POINT ( 'NONE',  ( 0.3392501089628018884, -0.1958661417322834220, -0.2545931758530183275 ) ) ;
#53676=CARTESIAN_POINT ( 'NONE',  ( -0.1974969037888704149, -0.3420746716998661063, -1.874671916010499428 ) ) ;
#53680=CARTESIAN_POINT ( 'NONE',  ( 0.4724409448818897572, -0.1265901696524988906, -2.001312335958005395 ) ) ;
#53681=CARTESIAN_POINT ( 'NONE',  ( 0.3496712940256230251, 0.1778467755331661626, -2.755905511811022279 ) ) ;
#53683=VERTEX_POINT ( 'NONE', #25611 ) ;
#53688=CARTESIAN_POINT ( 'NONE',  ( -0.3917322834645669549, -7.196005306013483243E-17, -2.481607980806087799 ) ) ;
#53695=CARTESIAN_POINT ( 'NONE',  ( -0.1049643490035302024, -0.3917322834645671215, 0.1581364829396324501 ) ) ;
#53697=CARTESIAN_POINT ( 'NONE',  ( -0.1958661417322834220, -0.3392501089628018884, -1.790026246719160330 ) ) ;
#53700=CARTESIAN_POINT ( 'NONE',  ( 0.1058382717557500713, -0.3949938075777409408, -2.447506561679789971 ) ) ;
#53705=CARTESIAN_POINT ( 'NONE',  ( -0.3996062992125986035, -0.1070741851644056997, -0.6758530183727035068 ) ) ;
#53711=CARTESIAN_POINT ( 'NONE',  ( -0.3917322834645670104, -7.196005306013484475E-17, 0.1909448818897636901 ) ) ;
#53717=CARTESIAN_POINT ( 'NONE',  ( -0.3917322834645671215, 0.1049643490035301469, 0.1325459317585302166 ) ) ;
#53722=CARTESIAN_POINT ( 'NONE',  ( -0.1265901696524993347, 0.4724409448818895907, -1.108923884514435798 ) ) ;
#53725=CARTESIAN_POINT ( 'NONE',  ( 0.3917322834645669549, 0.1049643490035304660, -0.5892388451443569819 ) ) ;
#53726=CARTESIAN_POINT ( 'NONE',  ( 4.797336870675656522E-17, -0.3917322834645670104, -2.368110236220472675 ) ) ;
#53729=CARTESIAN_POINT ( 'NONE',  ( -9.787531504996566615E-17, 0.3996062992125985480, -0.07677165354330711677 ) ) ;
#53734=CARTESIAN_POINT ( 'NONE',  ( 0.2867679344610365999, 0.2867679344610365999, -0.06034813828640239741 ) ) ;
#53741=CARTESIAN_POINT ( 'NONE',  ( 0.1958661417322834775, 0.3392501089628018884, -2.026246719160105236 ) ) ;
#53745=CARTESIAN_POINT ( 'NONE',  ( 0.4724409448818898682, 2.892866454678787531E-17, -0.5098425196850393526 ) ) ;
#53757=CARTESIAN_POINT ( 'NONE',  ( -9.787531504996566615E-17, 0.3996062992125985480, -1.494094488188976388 ) ) ;
#53766=CARTESIAN_POINT ( 'NONE',  ( -0.3996062992125986035, -7.340648628747425578E-17, -0.03937007874015749365 ) ) ;
#53767=CARTESIAN_POINT ( 'NONE',  ( -0.3392501089628017219, -0.1958661417322836995, -2.568916953577114359 ) ) ;
#53773=CARTESIAN_POINT ( 'NONE',  ( 0.3392501089628018884, -0.1958661417322834220, -2.551837270341207109 ) ) ;
#53778=CARTESIAN_POINT ( 'NONE',  ( -9.787531504996567848E-17, 0.3996062992125986035, -2.047244094488188892 ) ) ;
#53780=ADVANCED_FACE ( 'NONE', ( #77395 ), #13010, .T. ) ;
#53782=CARTESIAN_POINT ( 'NONE',  ( -0.2867679344610365444, -0.2867679344610367664, -0.2132739089576921876 ) ) ;
#53796=CARTESIAN_POINT ( 'NONE',  ( -0.2867679344610364334, -0.2867679344610367109, -0.6811023622047243098 ) ) ;
#53799=CARTESIAN_POINT ( 'NONE',  ( -0.3949938075777409408, -0.1058382717557502933, -1.148293963254593431 ) ) ;
#53815=CARTESIAN_POINT ( 'NONE',  ( 0.3460692066303959757, -0.1998031496062991907, -1.522309711286089273 ) ) ;
#53818=CARTESIAN_POINT ( 'NONE',  ( 0.3460692066303958092, 0.1998031496062993018, -0.9954068241469815614 ) ) ;
#53819=CARTESIAN_POINT ( 'NONE',  ( -0.3996062992125984925, -0.1070741851644056858, -0.4376640419947506744 ) ) ;
#53821=CARTESIAN_POINT ( 'NONE',  ( 0.1070741851644054915, -0.3996062992125986035, -2.919947506561679784 ) ) ;
#53822=( BOUNDED_CURVE ( )  B_SPLINE_CURVE ( 2, ( #80641, #75144, #17489, #54934, #67584, #47787, #9916, #43120, #68817 ),
 .UNSPECIFIED., .F., .F. ) 
 B_SPLINE_CURVE_WITH_KNOTS ( ( 3, 2, 2, 2, 3 ),
 ( 0.9375000000000000000, 0.9416666666666666519, 0.9458333333333333037, 0.9499999999999999556, 0.9506378855240343873 ),
 .UNSPECIFIED. ) 
 CURVE ( )  GEOMETRIC_REPRESENTATION_ITEM ( )  RATIONAL_B_SPLINE_CURVE ( ( 1.000000000000000000, 0.9659258262890683122, 1.000000000000000000, 0.9659258262890683122, 1.000000000000000000, 0.9659258262890683122, 1.000000000000000000, 0.9947834986831269877, 0.9911642120908010778 ) ) 
 REPRESENTATION_ITEM ( '' )  );
#53823=CARTESIAN_POINT ( 'NONE',  ( 0.3392501089628018884, -0.1958661417322834220, -2.394356955380577467 ) ) ;
#53829=CARTESIAN_POINT ( 'NONE',  ( 0.1265901696524989462, 0.4724409448818897572, -1.959973753280839892 ) ) ;
#53832=CARTESIAN_POINT ( 'NONE',  ( 0.1058382717557500852, -0.3949938075777408852, -1.736876640419947826 ) ) ;
#53839=CARTESIAN_POINT ( 'NONE',  ( 0.3458507752293908943, 0.3458507752293908943, -2.261811023622047223 ) ) ;
#53843=CARTESIAN_POINT ( 'NONE',  ( -0.1070741851644051862, -0.3996062992125986590, -2.511154855643044748 ) ) ;
#53844=CARTESIAN_POINT ( 'NONE',  ( -0.3917322834645668994, -0.1049643490035306742, -2.330689345635483356 ) ) ;
#53857=CARTESIAN_POINT ( 'NONE',  ( 0.2925321140481932369, 0.2925321140481932369, -0.2145669291338583029 ) ) ;
#53859=CARTESIAN_POINT ( 'NONE',  ( -0.3917322834645670104, -7.196005306013484475E-17, -2.013779527559055094 ) ) ;
#53868=CARTESIAN_POINT ( 'NONE',  ( -0.3996062992125985480, -7.340648628747423112E-17, -0.9035433070866141225 ) ) ;
#53874=CARTESIAN_POINT ( 'NONE',  ( 0.3941128856533801517, 0.02500110683994734295, -1.220472440943932924 ) ) ;
#53876=CARTESIAN_POINT ( 'NONE',  ( 0.4724409448818881474, -0.1265901696525019160, -2.158792650918635037 ) ) ;
#53884=CARTESIAN_POINT ( 'NONE',  ( -0.3460692066303960868, 0.1998031496062990242, -0.3412073490813647969 ) ) ;
#53885=VERTEX_POINT ( 'NONE', #32351 ) ;
#53887=CARTESIAN_POINT ( 'NONE',  ( -0.3392501089628017219, -0.1958661417322836718, -2.249343832020997525 ) ) ;
#53894=CARTESIAN_POINT ( 'NONE',  ( -0.4091458600556402980, -0.2362204724409451284, -2.019028871391076230 ) ) ;
#53899=CARTESIAN_POINT ( 'NONE',  ( 0.3917322834645668994, -0.1049643490035303134, -1.766384883693226771 ) ) ;
#53904=ORIENTED_EDGE ( 'NONE', *, *, #76928, .T. ) ;
#53905=CARTESIAN_POINT ( 'NONE',  ( 0.1958661417322834775, 0.3392501089628018884, -2.818260785598111884 ) ) ;
#53915=CARTESIAN_POINT ( 'NONE',  ( -0.1958661417322834220, -0.3392501089628018884, -2.197506561679789971 ) ) ;
#53923=CARTESIAN_POINT ( 'NONE',  ( -0.3460692066303960313, 0.1998031496062989965, 0.2119422572178477626 ) ) ;
#53925=CARTESIAN_POINT ( 'NONE',  ( 0.3996062992125986035, 2.446882876249141962E-17, -2.007874015748031482 ) ) ;
#53931=CARTESIAN_POINT ( 'NONE',  ( 0.2362204724409449064, 0.4091458600556404646, -0.8510498687664042050 ) ) ;
#53934=CARTESIAN_POINT ( 'NONE',  ( 0.2891555358219910499, -0.2891555358219909944, -0.6476377952755905110 ) ) ;
#53939=CARTESIAN_POINT ( 'NONE',  ( 0.1058382717557499880, 0.3949938075777409408, -0.3851706036745406458 ) ) ;
#53943=CARTESIAN_POINT ( 'NONE',  ( 0.1265901696524990572, -0.4724409448818897017, -0.1620734908136483021 ) ) ;
#53946=CARTESIAN_POINT ( 'NONE',  ( 0.2925321140481932369, 0.2925321140481932369, -1.316929133858267820 ) ) ;
#53948=CARTESIAN_POINT ( 'NONE',  ( -0.1958661417322834220, -0.3392501089628018884, -1.002624671916010568 ) ) ;
#53950=CARTESIAN_POINT ( 'NONE',  ( -0.3859888145977992124, -0.06766049032609708358, -3.091116300196750268E-17 ) ) ;
#53961=CARTESIAN_POINT ( 'NONE',  ( 0.2362204724409451007, -0.4091458600556402980, -2.688320209973753538 ) ) ;
#53968=CARTESIAN_POINT ( 'NONE',  ( -0.4091458600556405756, 0.2362204724409446288, -2.073490813648294129 ) ) ;
#53979=CARTESIAN_POINT ( 'NONE',  ( -0.3996062992125986035, -7.340648628747425578E-17, -0.6692913385826770867 ) ) ;
#53983=CARTESIAN_POINT ( 'NONE',  ( -0.2362204724409447953, -0.4091458600556404646, 0.09186351706036745279 ) ) ;
#53984=CARTESIAN_POINT ( 'NONE',  ( -0.1058382717557503211, 0.3949938075777409408, -2.368766404199475595 ) ) ;
#53987=CARTESIAN_POINT ( 'NONE',  ( -0.2867679344610365999, 0.2867679344610364889, -0.9566929133858265155 ) ) ;
#53994=CARTESIAN_POINT ( 'NONE',  ( 0.3917322834645668994, 0.1049643490035304522, -0.3621854086276097839 ) ) ;
#54001=CARTESIAN_POINT ( 'NONE',  ( 0.2867679344610366554, 0.2867679344610366554, -1.709336901083676086 ) ) ;
#54007=CARTESIAN_POINT ( 'NONE',  ( -0.3392501089628017219, -0.1958661417322836718, -1.082020997375328086 ) ) ;
#54017=CARTESIAN_POINT ( 'NONE',  ( 0.3392501089628018329, 0.1958661417322835607, -2.170603674540682260 ) ) ;
#54025=CARTESIAN_POINT ( 'NONE',  ( 0.1049643490035304938, -0.3917322834645669549, -1.114829396325459410 ) ) ;
#54026=CARTESIAN_POINT ( 'NONE',  ( -0.3460692066303957537, -0.1998031496062994405, -2.176509186351706315 ) ) ;
#54036=CARTESIAN_POINT ( 'NONE',  ( 0.2867679344610365999, 0.2867679344610365999, 0.02755905511811028441 ) ) ;
#54043=CARTESIAN_POINT ( 'NONE',  ( 0.1049643490035304522, -0.3917322834645668994, -1.110216904690602080 ) ) ;
#54052=CARTESIAN_POINT ( 'NONE',  ( 0.2867679344610366554, -0.2867679344610365999, -0.5676046176191095194 ) ) ;
#54055=CARTESIAN_POINT ( 'NONE',  ( 0.1265901696524989462, 0.4724409448818897572, -1.487532808398950301 ) ) ;
#54073=CARTESIAN_POINT ( 'NONE',  ( 0.3460692066303959202, -0.1998031496062991630, -2.701443569553806157 ) ) ;
#54078=CARTESIAN_POINT ( 'NONE',  ( 0.1070741851644053388, 0.3996062992125986035, -2.274934383202099397 ) ) ;
#54084=CARTESIAN_POINT ( 'NONE',  ( 0.1998031496062994405, -0.3460692066303958092, -1.981627296587926690 ) ) ;
#54085=CARTESIAN_POINT ( 'NONE',  ( 0.1058382717557500713, -0.3949938075777409408, -1.187664041994750619 ) ) ;
#54086=CARTESIAN_POINT ( 'NONE',  ( 0.3996062992125986590, -0.1070741851644053111, -2.631233595800525293 ) ) ;
#54088=CARTESIAN_POINT ( 'NONE',  ( -0.2867679344610364334, -0.2867679344610367109, -0.2086614173228345526 ) ) ;
#54092=CARTESIAN_POINT ( 'NONE',  ( 0.2891555358219910499, -0.2891555358219909944, -2.222440944881889813 ) ) ;
#54096=CARTESIAN_POINT ( 'NONE',  ( 0.2362204724409451007, -0.4091458600556402980, -2.139107611548556331 ) ) ;
#54104=CARTESIAN_POINT ( 'NONE',  ( 4.797336870675655290E-17, -0.3917322834645669549, -2.206017429624985038 ) ) ;
#54112=CARTESIAN_POINT ( 'NONE',  ( 0.3392501089628018329, 0.1958661417322835607, 0.09908136482939623735 ) ) ;
#54114=CARTESIAN_POINT ( 'NONE',  ( 0.1049643490035304938, -0.3917322834645669549, -1.967191601049868899 ) ) ;
#54117=CARTESIAN_POINT ( 'NONE',  ( 0.2891555358219910499, 0.2891555358219910499, -2.500000000000000444 ) ) ;
#54122=CARTESIAN_POINT ( 'NONE',  ( -0.1070741851644056997, 0.3996062992125986035, -1.108923884514435798 ) ) ;
#54127=CARTESIAN_POINT ( 'NONE',  ( -0.1958661417322834220, -0.3392501089628018884, 0.1646981627296586759 ) ) ;
#54134=ORIENTED_EDGE ( 'NONE', *, *, #46355, .T. ) ;
#54138=CARTESIAN_POINT ( 'NONE',  ( -0.4091458600556402980, -0.2362204724409451284, -1.469816272965879245 ) ) ;
#54141=CARTESIAN_POINT ( 'NONE',  ( -0.3917322834645671215, 0.1049643490035301469, -0.6548556430446192955 ) ) ;
#54142=CARTESIAN_POINT ( 'NONE',  ( -0.3917322834645670104, -7.196005306013484475E-17, -2.328740157480315265 ) ) ;
#54145=CARTESIAN_POINT ( 'NONE',  ( -0.1070741851644056997, 0.3996062992125984925, -0.08333333333333337034 ) ) ;
#54150=CARTESIAN_POINT ( 'NONE',  ( -0.3917322834645668994, -0.1049643490035306742, -0.1259649361866648498 ) ) ;
#54152=CARTESIAN_POINT ( 'NONE',  ( -9.594673741351313045E-17, 0.3917322834645670104, -0.3996062992125985480 ) ) ;
#54157=CARTESIAN_POINT ( 'NONE',  ( -0.1958661417322834220, -0.3392501089628018884, -1.790026246719160330 ) ) ;
#54161=CARTESIAN_POINT ( 'NONE',  ( 5.785732909357575061E-17, -0.4724409448818898682, -0.1555118110236220763 ) ) ;
#54164=LINE ( 'NONE', #41139, #64002 ) ;
#54172=CARTESIAN_POINT ( 'NONE',  ( 0.2925321140481932369, -0.2925321140481931814, -1.435039370078740051 ) ) ;
#54181=CARTESIAN_POINT ( 'NONE',  ( -0.1070741851644057135, 0.3996062992125984925, -0.2408136482939632061 ) ) ;
#54182=CARTESIAN_POINT ( 'NONE',  ( 0.3996062992125986035, 2.446882876249141962E-17, 0.03937007874015747283 ) ) ;
#54183=CARTESIAN_POINT ( 'NONE',  ( 0.1958661417322836718, -0.3392501089628017219, -2.923247662238532385 ) ) ;
#54184=CARTESIAN_POINT ( 'NONE',  ( 0.03175677952934891773, -0.3980111619244106613, -1.112674926538824158E-15 ) ) ;
#54186=CARTESIAN_POINT ( 'NONE',  ( 0.2017716535433070613, 0.2017716535433070613, 0.000000000000000000 ) ) ;
#54188=CARTESIAN_POINT ( 'NONE',  ( 0.1958661417322836440, -0.3392501089628017219, -2.538713910761154491 ) ) ;
#54193=CARTESIAN_POINT ( 'NONE',  ( 0.1265901696524990294, -0.4724409448818896462, -0.8727034120734907807 ) ) ;
#54194=CARTESIAN_POINT ( 'NONE',  ( 0.2925321140481932369, -0.2925321140481931814, -1.988188976377952777 ) ) ;
#54197=CARTESIAN_POINT ( 'NONE',  ( -0.3392501089628017219, -0.1958661417322836995, -0.2067122291676659340 ) ) ;
#54212=CARTESIAN_POINT ( 'NONE',  ( 0.2867679344610365999, -0.2867679344610365444, -0.7204724409448818312 ) ) ;
#54215=CARTESIAN_POINT ( 'NONE',  ( -0.1058382717557497937, -0.3949938075777411628, -1.017060367454068359 ) ) ;
#54225=CARTESIAN_POINT ( 'NONE',  ( 0.1265901696524989184, 0.4724409448818898127, -0.3851706036745407014 ) ) ;
#54232=CARTESIAN_POINT ( 'NONE',  ( -0.1998031496062991907, -0.3460692066303959757, -1.797900262467191590 ) ) ;
#54235=CARTESIAN_POINT ( 'NONE',  ( 0.3460692066303959202, -0.1998031496062991630, -1.126640419947506633 ) ) ;
#54236=CARTESIAN_POINT ( 'NONE',  ( 0.3996062992125986035, -0.1070741851644052972, -0.5032808398950130435 ) ) ;
#54239=CARTESIAN_POINT ( 'NONE',  ( -0.1265901696524993347, 0.4724409448818895907, -0.006561679790026246628 ) ) ;
#54240=CARTESIAN_POINT ( 'NONE',  ( 0.1049643490035303689, 0.3917322834645670104, -2.440288713910760521 ) ) ;
#54246=CARTESIAN_POINT ( 'NONE',  ( 0.4724409448818898682, 2.892866454678787531E-17, -1.769685039370078927 ) ) ;
#54250=CARTESIAN_POINT ( 'NONE',  ( -0.3420746716998660508, -0.1974969037888706924, -1.861548556430446588 ) ) ;
#54259=CARTESIAN_POINT ( 'NONE',  ( -0.3996062992125984925, -0.1070741851644056858, -2.484908136482939955 ) ) ;
#54260=CARTESIAN_POINT ( 'NONE',  ( 0.3917322834645668994, 0.1049643490035304522, -2.566909818076428706 ) ) ;
#54270=CARTESIAN_POINT ( 'NONE',  ( 0.4091458600556404646, -0.2362204724409448231, -0.8923884514435694859 ) ) ;
#54274=CARTESIAN_POINT ( 'NONE',  ( 0.3996062992125985480, 2.446882876249141654E-17, -0.5098425196850393526 ) ) ;
#54276=CARTESIAN_POINT ( 'NONE',  ( 0.3392501089628018884, -0.1958661417322834220, -1.921916010498687877 ) ) ;
#54285=CARTESIAN_POINT ( 'NONE',  ( -0.1070741851644056997, 0.3996062992125984925, -1.028215223097112663 ) ) ;
#54298=CARTESIAN_POINT ( 'NONE',  ( -0.3392501089628019995, 0.1958661417322832277, -2.695538057742782101 ) ) ;
#54301=CARTESIAN_POINT ( 'NONE',  ( -0.1070741851644051862, -0.3996062992125987146, -0.3871391076115485719 ) ) ;
#54306=CARTESIAN_POINT ( 'NONE',  ( -0.1049643490035302024, -0.3917322834645671215, -2.269028871391075786 ) ) ;
#54313=CARTESIAN_POINT ( 'NONE',  ( 0.3458507752293908943, -0.3458507752293908943, -2.064960629921259283 ) ) ;
#54316=CARTESIAN_POINT ( 'NONE',  ( -0.2867679344610366554, 0.2867679344610365444, -1.517041051672229024 ) ) ;
#54320=EDGE_CURVE ( 'NONE', #59512, #21899, #21649, .T. ) ;
#54324=CARTESIAN_POINT ( 'NONE',  ( 0.1058382717557500713, -0.3949938075777409408, 0.07217847769028866434 ) ) ;
#54332=CARTESIAN_POINT ( 'NONE',  ( 4.797336870675656522E-17, -0.3917322834645670659, -1.335321153052180243 ) ) ;
#54334=CARTESIAN_POINT ( 'NONE',  ( 0.1958661417322836440, -0.3392501089628017219, -2.381233595800524849 ) ) ;
#54341=CARTESIAN_POINT ( 'NONE',  ( -9.787531504996566615E-17, 0.3996062992125985480, 0.2381889763779527491 ) ) ;
#54343=CARTESIAN_POINT ( 'NONE',  ( -0.1070741851644051862, -0.3996062992125987146, -1.804461942257217677 ) ) ;
#54348=CARTESIAN_POINT ( 'NONE',  ( -0.2362204724409447953, -0.4091458600556404646, -0.4573490813648293796 ) ) ;
#54351=CARTESIAN_POINT ( 'NONE',  ( 0.3949938075777408852, 0.1058382717557500435, -0.6738845144356955252 ) ) ;
#54357=CARTESIAN_POINT ( 'NONE',  ( 0.3420746716998660508, -0.1974969037888704149, -0.3392388451443569819 ) ) ;
#54364=CARTESIAN_POINT ( 'NONE',  ( 0.3996062992125986035, -0.1070741851644052972, -1.448162729658792669 ) ) ;
#54366=CARTESIAN_POINT ( 'NONE',  ( -0.1958661417322834220, -0.3392501089628018884, -1.160104986876640210 ) ) ;
#54368=CARTESIAN_POINT ( 'NONE',  ( -0.3874523867751280548, 0.05870088567680999819, 1.458593243026437152E-17 ) ) ;
#54382=CARTESIAN_POINT ( 'NONE',  ( 0.1265901696524990572, -0.4724409448818897017, -0.3195538057742782212 ) ) ;
#54395=CARTESIAN_POINT ( 'NONE',  ( 0.3996062992125986035, -0.1070741851644053111, -0.5839895013123358458 ) ) ;
#54399=CARTESIAN_POINT ( 'NONE',  ( 0.1265901696524989462, 0.4724409448818897572, 0.006561679790026246628 ) ) ;
#54400=CARTESIAN_POINT ( 'NONE',  ( 4.837279021331060870E-17, -0.3949938075777409963, -2.283464566929133799 ) ) ;
#54403=CARTESIAN_POINT ( 'NONE',  ( -0.3392501089628017219, -0.1958661417322836718, -0.8320209973753279753 ) ) ;
#54411=CARTESIAN_POINT ( 'NONE',  ( 0.3917322834645668994, -0.1049643490035303134, -0.1915817340869272467 ) ) ;
#54418=CARTESIAN_POINT ( 'NONE',  ( -0.3392501089628019995, 0.1958661417322831999, -1.440308029692600522 ) ) ;
#54425=CARTESIAN_POINT ( 'NONE',  ( 0.2867679344610365999, 0.2867679344610365999, -1.167322834645669438 ) ) ;
#54434=CARTESIAN_POINT ( 'NONE',  ( 0.1049643490035304938, -0.3917322834645669549, -2.439632545931758045 ) ) ;
#54443=CARTESIAN_POINT ( 'NONE',  ( -0.4724409448818898682, 5.785732909357575061E-17, -2.755905511811024056 ) ) ;
#54444=CARTESIAN_POINT ( 'NONE',  ( -0.1049643490035302024, -0.3917322834645671215, -1.259186351706037099 ) ) ;
#54445=CARTESIAN_POINT ( 'NONE',  ( -0.1070741851644056997, 0.3996062992125984925, -2.288057742782152015 ) ) ;
#54454=CARTESIAN_POINT ( 'NONE',  ( 0.2925321140481931814, 0.2925321140481931814, -2.104330708661417582 ) ) ;
#54456=CARTESIAN_POINT ( 'NONE',  ( -0.1049643490035302024, -0.3917322834645671215, 0.09317585301837272294 ) ) ;
#54464=CARTESIAN_POINT ( 'NONE',  ( -0.1049643490035301746, -0.3917322834645670659, -1.254573860071179103 ) ) ;
#54473=CARTESIAN_POINT ( 'NONE',  ( 4.797336870675656522E-17, -0.3917322834645670659, -0.5479195782490308142 ) ) ;
#54476=CARTESIAN_POINT ( 'NONE',  ( 0.1265901696524989462, 0.4724409448818897572, -1.802493438320209584 ) ) ;
#54490=CARTESIAN_POINT ( 'NONE',  ( 0.03178304480586199854, -0.3983403474834772418, -9.560572922657961637E-16 ) ) ;
#54497=CARTESIAN_POINT ( 'NONE',  ( 0.3996062992125984925, 0.1070741851644054637, -2.406167979002624246 ) ) ;
#54501=CARTESIAN_POINT ( 'NONE',  ( -0.3996062992125986035, -0.1070741851644056997, -1.935695538057742526 ) ) ;
#54502=CARTESIAN_POINT ( 'NONE',  ( -0.1058382717557497937, -0.3949938075777411628, -1.174540682414698223 ) ) ;
#54503=CARTESIAN_POINT ( 'NONE',  ( 0.3460692066303959757, -0.1998031496062991907, -2.624671916010498762 ) ) ;
#54505=CARTESIAN_POINT ( 'NONE',  ( 0.3392501089628018329, 0.1958661417322835607, -0.2808398950131232863 ) ) ;
#54509=CARTESIAN_POINT ( 'NONE',  ( 0.1058382717557499880, 0.3949938075777409408, -1.959973753280839670 ) ) ;
#54513=CARTESIAN_POINT ( 'NONE',  ( 0.4724409448818897572, -0.1265901696524988906, -2.631233595800525293 ) ) ;
#54514=CARTESIAN_POINT ( 'NONE',  ( -0.2925321140481932924, 0.2925321140481931814, -1.909448818897637512 ) ) ;
#54522=CARTESIAN_POINT ( 'NONE',  ( 0.3917322834645668994, -0.1049643490035303134, -2.711266773457006174 ) ) ;
#54529=CARTESIAN_POINT ( 'NONE',  ( -0.3917322834645669549, -0.1049643490035306603, 0.02690288713910752097 ) ) ;
#54531=CARTESIAN_POINT ( 'NONE',  ( -0.1958661417322834220, -0.3392501089628018884, -2.104986876640420057 ) ) ;
#54534=CARTESIAN_POINT ( 'NONE',  ( 0.3949938075777409963, 2.418639510665530435E-17, -2.480314960629921295 ) ) ;
#54535=VERTEX_POINT ( 'NONE', #30029 ) ;
#54539=CARTESIAN_POINT ( 'NONE',  ( 4.893765752498283924E-17, -0.3996062992125986035, -0.8661417322834645827 ) ) ;
#54540=DIRECTION ( 'NONE',  ( 0.000000000000000000, 0.000000000000000000, 1.000000000000000000 ) ) ;
#54544=CARTESIAN_POINT ( 'NONE',  ( 0.3392501089628018884, -0.1958661417322834220, 0.1253280839895012100 ) ) ;
#54550=CARTESIAN_POINT ( 'NONE',  ( -0.3917322834645669549, -0.1049643490035306603, 0.1194225721784776956 ) ) ;
#54555=CARTESIAN_POINT ( 'NONE',  ( -1.157146581871515012E-16, 0.4724409448818898682, -1.889763779527559251 ) ) ;
#54557=EDGE_CURVE ( 'NONE', #24503, #17964, #67109, .T. ) ;
#54558=CARTESIAN_POINT ( 'NONE',  ( 0.2867679344610365999, -0.2867679344610365444, -0.7204724409448818312 ) ) ;
#54567=CARTESIAN_POINT ( 'NONE',  ( -0.2867679344610366554, 0.2867679344610365444, 0.05776209793407005577 ) ) ;
#54570=CARTESIAN_POINT ( 'NONE',  ( 0.3392501089628018884, -0.1958661417322834220, -0.5045931758530184386 ) ) ;
#54576=CARTESIAN_POINT ( 'NONE',  ( 0.1958661417322836440, -0.3392501089628017219, -2.446194225721784576 ) ) ;
#54581=CARTESIAN_POINT ( 'NONE',  ( 0.1265901696524990294, -0.4724409448818896462, -0.1620734908136483021 ) ) ;
#54590=CARTESIAN_POINT ( 'NONE',  ( 0.3458507752293908943, 0.3458507752293908943, -1.946850393700787274 ) ) ;
#54592=CARTESIAN_POINT ( 'NONE',  ( 0.3996062992125986035, -0.1070741851644052972, -1.763123359580051952 ) ) ;
#54602=CARTESIAN_POINT ( 'NONE',  ( 0.3996062992125985480, 2.446882876249141654E-17, -0.03740157480314963701 ) ) ;
#54603=CARTESIAN_POINT ( 'NONE',  ( 0.2925321140481932369, -0.2925321140481932369, -0.5708661417322833387 ) ) ;
#54604=CARTESIAN_POINT ( 'NONE',  ( 0.2867679344610366554, -0.2867679344610365999, -2.929809342028559360 ) ) ;
#54607=DIRECTION ( 'NONE',  ( 0.000000000000000000, 0.000000000000000000, 1.000000000000000000 ) ) ;
#54609=CARTESIAN_POINT ( 'NONE',  ( -0.3949938075777408852, -0.1058382717557502933, -1.067585301837270739 ) ) ;
#54614=CARTESIAN_POINT ( 'NONE',  ( -1.157146581871515012E-16, 0.4724409448818898682, -1.102362204724409489 ) ) ;
#54615=CARTESIAN_POINT ( 'NONE',  ( -0.3996062992125986590, 0.1070741851644051862, -2.237532808398950301 ) ) ;
#54618=CARTESIAN_POINT ( 'NONE',  ( -0.1049643490035302301, -0.3917322834645671770, -0.5413578984590045051 ) ) ;
#54629=CARTESIAN_POINT ( 'NONE',  ( -0.2867679344610364334, -0.2867679344610367109, -0.9960629921259842590 ) ) ;
#54632=CARTESIAN_POINT ( 'NONE',  ( 0.1974969037888704704, 0.3420746716998660508, -1.089238845144357093 ) ) ;
#54645=CARTESIAN_POINT ( 'NONE',  ( 0.4724409448818898682, 2.892866454678787531E-17, -0.3523622047244094335 ) ) ;
#54651=CARTESIAN_POINT ( 'NONE',  ( -0.1070741851644056997, 0.3996062992125986035, -1.581364829396325389 ) ) ;
#54654=CARTESIAN_POINT ( 'NONE',  ( 0.3996062992125986035, -0.1070741851644052972, -0.9757217847769029673 ) ) ;
#54657=CARTESIAN_POINT ( 'NONE',  ( 0.3458507752293908943, -0.3458507752293908943, -0.2559055118110235560 ) ) ;
#54658=CARTESIAN_POINT ( 'NONE',  ( -0.3392501089628017219, -0.1958661417322836718, -2.656824146981627166 ) ) ;
#54664=CARTESIAN_POINT ( 'NONE',  ( -0.1265901696524986964, -0.4724409448818899238, -2.353674540682414218 ) ) ;
#54667=CARTESIAN_POINT ( 'NONE',  ( 0.2891555358219910499, 0.2891555358219910499, -1.789370078740157632 ) ) ;
#54678=CARTESIAN_POINT ( 'NONE',  ( -0.2867679344610366554, 0.2867679344610365444, -2.304442626475378564 ) ) ;
#54693=CARTESIAN_POINT ( 'NONE',  ( 0.1998031496062994128, -0.3460692066303957537, -0.1686351706036745557 ) ) ;
#54697=CARTESIAN_POINT ( 'NONE',  ( -0.1049643490035307020, 0.3917322834645669549, -1.980971128608924214 ) ) ;
#54708=CARTESIAN_POINT ( 'NONE',  ( -0.3460692066303957537, -0.1998031496062994405, -1.074146981627296604 ) ) ;
#54711=ORIENTED_EDGE ( 'NONE', *, *, #18760, .T. ) ;
#54716=CARTESIAN_POINT ( 'NONE',  ( 0.1049643490035304938, -0.3917322834645669549, -1.744750656167979308 ) ) ;
#54717=CARTESIAN_POINT ( 'NONE',  ( 0.2417350488526480157, 0.3089825338611894012, -1.220472440944881942 ) ) ;
#54722=CARTESIAN_POINT ( 'NONE',  ( 0.1998031496062992463, 0.3460692066303959202, -2.268372703412073754 ) ) ;
#54725=CARTESIAN_POINT ( 'NONE',  ( 0.3460692066303959757, -0.1998031496062991907, -0.4199475065616797842 ) ) ;
#54728=CARTESIAN_POINT ( 'NONE',  ( -0.2867679344610364334, -0.2867679344610367109, -2.255905511811023612 ) ) ;
#54738=CARTESIAN_POINT ( 'NONE',  ( 0.3392501089628018329, 0.1958661417322835052, -1.471109293142045304 ) ) ;
#54744=CARTESIAN_POINT ( 'NONE',  ( -0.3917322834645671770, 0.1049643490035302024, -2.864192544128295825 ) ) ;
#54752=CARTESIAN_POINT ( 'NONE',  ( -0.1049643490035302301, -0.3917322834645671770, -1.171279158301524292 ) ) ;
#54754=CARTESIAN_POINT ( 'NONE',  ( -0.1049643490035307020, 0.3917322834645669549, -2.295931758530183497 ) ) ;
#54760=CARTESIAN_POINT ( 'NONE',  ( 0.3460692066303958092, 0.1998031496062993018, -0.05052493438320210251 ) ) ;
#54762=CARTESIAN_POINT ( 'NONE',  ( 0.1070741851644054915, -0.3996062992125986035, -1.817585301837270517 ) ) ;
#54769=CARTESIAN_POINT ( 'NONE',  ( 0.2362204724409449064, 0.4091458600556404646, -0.6935695538057742304 ) ) ;
#54772=CARTESIAN_POINT ( 'NONE',  ( -0.3420746716998662729, 0.1974969037888702206, -0.7329396325459319739 ) ) ;
#54777=CARTESIAN_POINT ( 'NONE',  ( 0.3949938075777409408, -0.1058382717557499186, -0.3458005249343832910 ) ) ;
#54785=CARTESIAN_POINT ( 'NONE',  ( 0.1070741851644053388, 0.3996062992125986035, -1.487532808398950301 ) ) ;
#54787=CARTESIAN_POINT ( 'NONE',  ( 0.1049643490035304938, -0.3917322834645669549, -1.179790026246718915 ) ) ;
#54811=( BOUNDED_CURVE ( )  B_SPLINE_CURVE ( 2, ( #41608, #16787, #67297, #60963, #62205, #4542, #42424, #16370, #73619, #79522, #21837, #47500, #73193 ),
 .UNSPECIFIED., .F., .F. ) 
 B_SPLINE_CURVE_WITH_KNOTS ( ( 3, 2, 2, 2, 2, 2, 3 ),
 ( 0.3624999999999999889, 0.3666666666666666408, 0.3708333333333333481, 0.3750000000000000000, 0.3791666666666666519, 0.3833333333333333592, 0.3875000000000000111 ),
 .UNSPECIFIED. ) 
 CURVE ( )  GEOMETRIC_REPRESENTATION_ITEM ( )  RATIONAL_B_SPLINE_CURVE ( ( 1.000000000000000000, 0.9659258262890683122, 1.000000000000000000, 0.9659258262890683122, 1.000000000000000000, 0.9659258262890683122, 1.000000000000000000, 0.9659258262890683122, 1.000000000000000000, 0.9659258262890683122, 1.000000000000000000, 0.9659258262890683122, 1.000000000000000000 ) ) 
 REPRESENTATION_ITEM ( '' )  );
#54813=FACE_OUTER_BOUND ( 'NONE', #72622, .T. ) ;
#54815=CARTESIAN_POINT ( 'NONE',  ( 0.3996062992125986035, -0.1070741851644053111, -1.056430446194225770 ) ) ;
#54820=CARTESIAN_POINT ( 'NONE',  ( 0.3458507752293908943, -0.3458507752293908943, 0.05905511811023620578 ) ) ;
#54821=CARTESIAN_POINT ( 'NONE',  ( 0.1058382717557499880, 0.3949938075777411073, -2.513123359580052174 ) ) ;
#54824=CARTESIAN_POINT ( 'NONE',  ( 0.3392501089628018329, 0.1958661417322835607, -0.7532808398950130435 ) ) ;
#54826=CARTESIAN_POINT ( 'NONE',  ( -0.1265901696524986964, -0.4724409448818899238, -2.276902887139107268 ) ) ;
#54832=CARTESIAN_POINT ( 'NONE',  ( -0.2867679344610366554, 0.2867679344610365444, -0.09971821702655986330 ) ) ;
#54839=CARTESIAN_POINT ( 'NONE',  ( 0.3917322834645670659, 2.398668435337828261E-17, -1.532171546752967739 ) ) ;
#54843=ADVANCED_FACE ( 'NONE', ( #48973 ), #17580, .T. ) ;
#54846=CARTESIAN_POINT ( 'NONE',  ( -0.1049643490035302024, -0.3917322834645671215, -1.101706036745407014 ) ) ;
#54855=CARTESIAN_POINT ( 'NONE',  ( 0.1049643490035303689, 0.3917322834645670104, -2.505249343832020248 ) ) ;
#54862=CARTESIAN_POINT ( 'NONE',  ( -0.2867679344610364334, -0.2867679344610367109, -0.9311023622047245318 ) ) ;
#54865=CARTESIAN_POINT ( 'NONE',  ( -0.1958661417322834220, -0.3392501089628018884, -1.252624671916010568 ) ) ;
#54866=CARTESIAN_POINT ( 'NONE',  ( -9.787531504996566615E-17, 0.3996062992125985480, -2.596456692913385655 ) ) ;
#54875=CARTESIAN_POINT ( 'NONE',  ( -0.3460692066303957537, -0.1998031496062994405, -2.176509186351706315 ) ) ;
#54877=CARTESIAN_POINT ( 'NONE',  ( -0.1958661417322836718, 0.3392501089628017219, 0.1522309711286089495 ) ) ;
#54885=CARTESIAN_POINT ( 'NONE',  ( -0.3917322834645668994, -0.1049643490035306742, -1.070846825950444448 ) ) ;
#54893=CARTESIAN_POINT ( 'NONE',  ( -0.1958661417322836995, 0.3392501089628017219, -0.4823027803487682785 ) ) ;
#54895=CARTESIAN_POINT ( 'NONE',  ( 0.4091458600556403535, 0.2362204724409449896, -2.097769028871391050 ) ) ;
#54905=CARTESIAN_POINT ( 'NONE',  ( -0.4724409448818917001, 0.1265901696524956710, -2.156824146981627610 ) ) ;
#54914=CARTESIAN_POINT ( 'NONE',  ( -0.3996062992125986035, -7.340648628747425578E-17, -0.03937007874015750059 ) ) ;
#54915=CARTESIAN_POINT ( 'NONE',  ( -0.2925321140481930149, -0.2925321140481933480, -2.025590551181102317 ) ) ;
#54920=CARTESIAN_POINT ( 'NONE',  ( -0.2925321140481930704, -0.2925321140481933480, -1.948818897637795144 ) ) ;
#54921=CARTESIAN_POINT ( 'NONE',  ( 0.3420746716998659953, 0.1974969037888705536, -1.233595800524934338 ) ) ;
#54922=CARTESIAN_POINT ( 'NONE',  ( -0.2925321140481930704, -0.2925321140481933480, -2.263779527559055094 ) ) ;
#54924=CARTESIAN_POINT ( 'NONE',  ( 0.3917322834645669549, 0.1049643490035304660, -0.1167979002624671414 ) ) ;
#54928=CARTESIAN_POINT ( 'NONE',  ( -0.3949938075777408852, -0.1058382717557502933, -2.169947506561679784 ) ) ;
#54932=CARTESIAN_POINT ( 'NONE',  ( 0.4091458600556403535, 0.2362204724409449896, -2.650918635170603554 ) ) ;
#54933=CARTESIAN_POINT ( 'NONE',  ( 0.1070741851644053527, 0.3996062992125986590, -1.725721784776903078 ) ) ;
#54934=CARTESIAN_POINT ( 'NONE',  ( 0.3458507752293908943, 0.3458507752293908943, -2.734251968503936592 ) ) ;
#54941=CARTESIAN_POINT ( 'NONE',  ( -0.1049643490035302024, -0.3917322834645671215, 0.1581364829396324501 ) ) ;
#54942=CARTESIAN_POINT ( 'NONE',  ( 0.4709442531824356015, 0.03757601356358734185, -1.929133858267717549 ) ) ;
#54944=CARTESIAN_POINT ( 'NONE',  ( 0.1265901696524990572, -0.4724409448818897017, -2.447506561679789527 ) ) ;
#54948=CARTESIAN_POINT ( 'NONE',  ( 0.1958661417322836440, -0.3392501089628017219, -0.1765091863517061210 ) ) ;
#54950=CARTESIAN_POINT ( 'NONE',  ( -0.1049643490035302024, -0.3917322834645671215, -2.426509186351705427 ) ) ;
#54953=CARTESIAN_POINT ( 'NONE',  ( -0.3949938075777409408, -0.1058382717557502933, -2.723097112860892732 ) ) ;
#54957=CARTESIAN_POINT ( 'NONE',  ( 0.3996062992125986035, 0.1070741851644054776, -0.9120734908136483021 ) ) ;
#54959=CARTESIAN_POINT ( 'NONE',  ( 0.2362204724409451007, -0.4091458600556402980, -0.7985564304461942875 ) ) ;
#54962=CARTESIAN_POINT ( 'NONE',  ( -0.2867679344610364334, -0.2867679344610367109, 0.01377952755905502598 ) ) ;
#54968=CARTESIAN_POINT ( 'NONE',  ( 0.3917322834645670104, 2.398668435337828261E-17, 0.04724409448818902429 ) ) ;
#54971=CARTESIAN_POINT ( 'NONE',  ( 0.000000000000000000, 0.000000000000000000, -2.755905511811024056 ) ) ;
#54972=CARTESIAN_POINT ( 'NONE',  ( -0.3458507752293906723, -0.3458507752293910609, -1.633858267716534973 ) ) ;
#54974=CARTESIAN_POINT ( 'NONE',  ( -0.1049643490035307020, 0.3917322834645669549, -0.7860892388451442558 ) ) ;
#54975=CARTESIAN_POINT ( 'NONE',  ( 0.09156050430091122738, 0.3808816823641256732, -2.755905511811024056 ) ) ;
#54982=CARTESIAN_POINT ( 'NONE',  ( 0.1958661417322836162, -0.3392501089628018329, -0.01441637975621864153 ) ) ;
#54984=CARTESIAN_POINT ( 'NONE',  ( -0.3392501089628017219, -0.1958661417322836718, -0.2946194225721785465 ) ) ;
#54989=CARTESIAN_POINT ( 'NONE',  ( 0.3917322834645670104, 2.398668435337828261E-17, -2.472440944881889813 ) ) ;
#54992=CARTESIAN_POINT ( 'NONE',  ( -0.3458507752293909498, 0.3458507752293907833, -0.8838582677165351953 ) ) ;
#55003=CARTESIAN_POINT ( 'NONE',  ( -0.3996062992125986590, 0.1070741851644051723, -1.841863517060367439 ) ) ;
#55010=CARTESIAN_POINT ( 'NONE',  ( 0.3460692066303958092, 0.1998031496062993018, -0.2080052493438320771 ) ) ;
#55011=CARTESIAN_POINT ( 'NONE',  ( 0.1070741851644054915, -0.3996062992125986035, -0.4002624671916010235 ) ) ;
#55012=CARTESIAN_POINT ( 'NONE',  ( -0.3392501089628019995, 0.1958661417322831999, -2.857630864338269738 ) ) ;
#55018=CARTESIAN_POINT ( 'NONE',  ( 0.1058382717557499880, 0.3949938075777409408, -0.8576115485564304031 ) ) ;
#55024=CARTESIAN_POINT ( 'NONE',  ( 0.3458507752293908943, 0.3458507752293908943, -1.082677165354330562 ) ) ;
#55025=CARTESIAN_POINT ( 'NONE',  ( -0.2925321140481930704, -0.2925321140481933480, -2.421259842519684735 ) ) ;
#55028=CARTESIAN_POINT ( 'NONE',  ( 0.1049643490035303967, 0.3917322834645670659, -0.6200980559393196589 ) ) ;
#55040=CARTESIAN_POINT ( 'NONE',  ( 0.2867679344610365999, -0.2867679344610365444, -0.8779527559055116948 ) ) ;
#55042=VERTEX_POINT ( 'NONE', #22447 ) ;
#55043=CARTESIAN_POINT ( 'NONE',  ( 0.3949938075777409963, 2.418639510665530435E-17, -0.9055118110236219930 ) ) ;
#55058=CARTESIAN_POINT ( 'NONE',  ( -0.3996062992125986035, -7.340648628747425578E-17, -1.771653543307086576 ) ) ;
#55059=CARTESIAN_POINT ( 'NONE',  ( -0.4724409448818898682, -8.678599364036362592E-17, -0.3543307086614173040 ) ) ;
#55061=CARTESIAN_POINT ( 'NONE',  ( -9.787531504996566615E-17, 0.3996062992125985480, -1.336614173228346303 ) ) ;
#55065=CARTESIAN_POINT ( 'NONE',  ( -0.1265901696524986964, -0.4724409448818899238, -0.3871391076115485719 ) ) ;
#55066=CARTESIAN_POINT ( 'NONE',  ( 0.3392501089628018329, 0.1958661417322835607, -2.735564304461941987 ) ) ;
#55072=CARTESIAN_POINT ( 'NONE',  ( 0.3458507752293908943, 0.3458507752293908943, -2.419291338582676865 ) ) ;
#55074=CARTESIAN_POINT ( 'NONE',  ( -0.1974969037888706924, 0.3420746716998658843, -1.822178477690288512 ) ) ;
#55080=CARTESIAN_POINT ( 'NONE',  ( 5.785732909357575061E-17, -0.4724409448818898682, -2.202755905511811108 ) ) ;
#55084=CARTESIAN_POINT ( 'NONE',  ( -0.2867679344610364334, -0.2867679344610368219, -2.343812705215535974 ) ) ;
#55097=B_SPLINE_CURVE_WITH_KNOTS ( 'NONE', 1,
 ( #49199, #4585 ),
 .UNSPECIFIED., .F., .F.,
 ( 2, 2 ),
 ( 0.000000000000000000, 0.001849999999999997480 ),
 .UNSPECIFIED. ) ;
#55099=CARTESIAN_POINT ( 'NONE',  ( 0.1070741851644053388, 0.3996062992125986035, -0.3851706036745406458 ) ) ;
#55101=CARTESIAN_POINT ( 'NONE',  ( -0.1049643490035302024, -0.3917322834645671215, -1.731627296587926468 ) ) ;
#55110=CARTESIAN_POINT ( 'NONE',  ( 0.3996062992125985480, 2.446882876249141654E-17, -1.454724409448818978 ) ) ;
#55112=CARTESIAN_POINT ( 'NONE',  ( 0.4724409448818898682, 2.892866454678787531E-17, -2.557086614173228689 ) ) ;
#55117=CARTESIAN_POINT ( 'NONE',  ( -0.3917322834645670104, -7.196005306013484475E-17, -1.541338582677165503 ) ) ;
#55118=CARTESIAN_POINT ( 'NONE',  ( -0.4091458600556402980, -0.2362204724409451284, -2.099737532808398921 ) ) ;
#55122=CARTESIAN_POINT ( 'NONE',  ( 0.1070741851644054637, -0.3996062992125984925, -2.524278215223096478 ) ) ;
#55124=CARTESIAN_POINT ( 'NONE',  ( 0.3996062992125986035, 0.1070741851644054776, -0.9120734908136483021 ) ) ;
#55125=ORIENTED_EDGE ( 'NONE', *, *, #30797, .T. ) ;
#55127=CARTESIAN_POINT ( 'NONE',  ( -9.594673741351313045E-17, 0.3917322834645670104, -2.354330708661417138 ) ) ;
#55137=CARTESIAN_POINT ( 'NONE',  ( 0.2867679344610365999, 0.2867679344610365999, -1.477670972932071614 ) ) ;
#55141=CARTESIAN_POINT ( 'NONE',  ( -0.3392501089628017219, -0.1958661417322836718, -2.656824146981627166 ) ) ;
#55144=CARTESIAN_POINT ( 'NONE',  ( -0.3392501089628019995, 0.1958661417322831999, -2.700150549377639653 ) ) ;
#55152=CARTESIAN_POINT ( 'NONE',  ( -0.3392501089628019995, 0.1958661417322831999, -1.440308029692600522 ) ) ;
#55154=CARTESIAN_POINT ( 'NONE',  ( 0.3917322834645669549, 0.1049643490035304660, -2.414041994750655729 ) ) ;
#55159=EDGE_CURVE ( 'NONE', #47997, #12829, #31071, .T. ) ;
#55160=CARTESIAN_POINT ( 'NONE',  ( -0.2925321140481930704, -0.2925321140481933480, -0.5314960629921260393 ) ) ;
#55162=CARTESIAN_POINT ( 'NONE',  ( -0.3460692066303960313, 0.1998031496062989965, 0.05446194225721784354 ) ) ;
#55164=CARTESIAN_POINT ( 'NONE',  ( 0.2925321140481932369, 0.2925321140481932369, -2.185039370078739829 ) ) ;
#55165=B_SPLINE_CURVE_WITH_KNOTS ( 'NONE', 1,
 ( #33011, #76398 ),
 .UNSPECIFIED., .F., .F.,
 ( 2, 2 ),
 ( 0.000000000000000000, 0.001849999999999997480 ),
 .UNSPECIFIED. ) ;
#55170=CARTESIAN_POINT ( 'NONE',  ( -0.2362204724409451284, 0.4091458600556402425, -0.8772965879265091083 ) ) ;
#55173=CARTESIAN_POINT ( 'NONE',  ( 4.837279021331061486E-17, -0.3949938075777409963, -0.4704724409448818867 ) ) ;
#55187=CARTESIAN_POINT ( 'NONE',  ( 0.3996062992125986035, -0.1070741851644052972, -1.920603674540682260 ) ) ;
#55190=CARTESIAN_POINT ( 'NONE',  ( 0.3917322834645670104, 2.398668435337828261E-17, -1.212598425196850238 ) ) ;
#55211=CARTESIAN_POINT ( 'NONE',  ( -0.1049643490035307158, 0.3917322834645670104, -2.208024565125671135 ) ) ;
#55222=CARTESIAN_POINT ( 'NONE',  ( -0.1070741851644056997, 0.3996062992125986035, -2.841207349081364963 ) ) ;
#55223=CARTESIAN_POINT ( 'NONE',  ( 0.3949938075777409408, 0.1058382717557500574, -2.329396325459317740 ) ) ;
#55226=CARTESIAN_POINT ( 'NONE',  ( -0.1958661417322836718, 0.3392501089628017219, -1.107611548556430403 ) ) ;
#55228=CARTESIAN_POINT ( 'NONE',  ( -0.2362204724409451284, 0.4091458600556402425, -2.375328083989501238 ) ) ;
#55235=CARTESIAN_POINT ( 'NONE',  ( -0.3917322834645669549, -7.196005306013483243E-17, -0.4343638863178984622 ) ) ;
#55236=ADVANCED_FACE ( 'NONE', ( #81361 ), #12297, .F. ) ;
#55241=DIRECTION ( 'NONE',  ( 1.000000000000000000, -0.000000000000000000, 0.000000000000000000 ) ) ;
#55242=CARTESIAN_POINT ( 'NONE',  ( 0.3460692066303959757, -0.1998031496062991907, -2.939632545931758489 ) ) ;
#55243=CARTESIAN_POINT ( 'NONE',  ( 0.3917322834645670659, -0.1049643490035303273, -1.683090181923571294 ) ) ;
#55249=CARTESIAN_POINT ( 'NONE',  ( 0.3392501089628018884, -0.1958661417322834220, -0.9770341207349081403 ) ) ;
#55258=CARTESIAN_POINT ( 'NONE',  ( 0.3917322834645669549, 0.1049643490035304660, -2.164041994750655729 ) ) ;
#55265=CARTESIAN_POINT ( 'NONE',  ( 0.3917322834645670104, 2.398668435337828261E-17, -0.6751968503937009203 ) ) ;
#55266=CARTESIAN_POINT ( 'NONE',  ( 0.2362204724409451007, -0.4091458600556402980, -0.01115485564304462100 ) ) ;
#55268=CARTESIAN_POINT ( 'NONE',  ( 0.3460692066303958092, 0.1998031496062993018, -2.570209973753280863 ) ) ;
#55287=CARTESIAN_POINT ( 'NONE',  ( 0.1958661417322834497, 0.3392501089628018329, -1.641712967682728008 ) ) ;
#55297=CARTESIAN_POINT ( 'NONE',  ( -0.1958661417322836995, 0.3392501089628017219, -0.6397830953093982531 ) ) ;
#55301=CARTESIAN_POINT ( 'NONE',  ( -0.4724409448818895907, -0.1265901696524993070, -2.169947506561679340 ) ) ;
#55323=CARTESIAN_POINT ( 'NONE',  ( 0.1998031496062994128, -0.3460692066303957537, -2.373359580052493367 ) ) ;
#55328=CARTESIAN_POINT ( 'NONE',  ( -9.787531504996567848E-17, 0.3996062992125986035, -1.732283464566929165 ) ) ;
#55329=CARTESIAN_POINT ( 'NONE',  ( 0.3420746716998659953, 0.1974969037888705536, -1.076115485564304475 ) ) ;
#55330=CARTESIAN_POINT ( 'NONE',  ( 0.1070741851644053527, 0.3996062992125986590, -2.513123359580052174 ) ) ;
#55332=CARTESIAN_POINT ( 'NONE',  ( 0.3917322834645669549, 0.1049643490035304660, -0.7467191601049868455 ) ) ;
#55336=CARTESIAN_POINT ( 'NONE',  ( 0.2891555358219910499, 0.2891555358219910499, -2.104330708661417138 ) ) ;
#55341=CARTESIAN_POINT ( 'NONE',  ( 0.2362204724409449064, 0.4091458600556404646, -2.349081364829396446 ) ) ;
#55342=CARTESIAN_POINT ( 'NONE',  ( 0.1070741851644053527, 0.3996062992125986590, -1.568241469816272993 ) ) ;
#55349=CARTESIAN_POINT ( 'NONE',  ( 0.1049643490035303689, 0.3917322834645670104, 0.07939632545931750440 ) ) ;
#55350=CARTESIAN_POINT ( 'NONE',  ( -0.3983403474834782965, -0.03178304480584832892, -1.220472440944881942 ) ) ;
#55356=CARTESIAN_POINT ( 'NONE',  ( 0.3917322834645670104, 2.398668435337828261E-17, -0.3602362204724410266 ) ) ;
#55358=CARTESIAN_POINT ( 'NONE',  ( 0.1049643490035303689, 0.3917322834645670104, -2.190288713910760521 ) ) ;
#55362=CARTESIAN_POINT ( 'NONE',  ( 0.1974969037888706369, -0.3420746716998659953, -2.769028871391075786 ) ) ;
#55366=CARTESIAN_POINT ( 'NONE',  ( 0.3996062992125986035, 0.1070741851644054776, -1.069553805774278166 ) ) ;
#55369=DIRECTION ( 'NONE',  ( -1.000000000000000000, 0.000000000000000000, 0.000000000000000000 ) ) ;
#55370=CARTESIAN_POINT ( 'NONE',  ( 0.0008564280371968460877, -0.3986795681651700840, -2.755905511811023612 ) ) ;
#55371=CARTESIAN_POINT ( 'NONE',  ( -0.2867679344610365999, 0.2867679344610364889, -0.2618110236220473341 ) ) ;
#55377=CARTESIAN_POINT ( 'NONE',  ( -9.594673741351313045E-17, 0.3917322834645670104, -0.3070866141732283006 ) ) ;
#55378=ORIENTED_EDGE ( 'NONE', *, *, #38275, .F. ) ;
#55381=CARTESIAN_POINT ( 'NONE',  ( -0.4724409448818899238, 0.1265901696524986686, -1.607611548556430403 ) ) ;
#55383=CARTESIAN_POINT ( 'NONE',  ( -0.2867679344610364334, -0.2867679344610367109, -2.663385826771653253 ) ) ;
#55390=CARTESIAN_POINT ( 'NONE',  ( -0.3917322834645670659, 0.1049643490035301607, -0.5852825214885022387 ) ) ;
#55392=CARTESIAN_POINT ( 'NONE',  ( -0.1958661417322834220, -0.3392501089628018884, -0.6227034120734910028 ) ) ;
#55398=CARTESIAN_POINT ( 'NONE',  ( -9.594673741351313045E-17, 0.3917322834645670104, -2.511811023622047223 ) ) ;
#55401=CARTESIAN_POINT ( 'NONE',  ( 0.4724409448818897572, -0.1265901696524988906, -0.8182414698162727706 ) ) ;
#55409=CARTESIAN_POINT ( 'NONE',  ( 0.000000000000000000, 0.000000000000000000, -2.755905511811024056 ) ) ;
#55413=CARTESIAN_POINT ( 'NONE',  ( 0.2925321140481932369, 0.2925321140481932369, -1.789370078740157410 ) ) ;
#55421=CARTESIAN_POINT ( 'NONE',  ( 0.1070741851644054637, -0.3996062992125984925, -0.1620734908136483299 ) ) ;
#55422=CARTESIAN_POINT ( 'NONE',  ( 0.3996062992125986590, -0.1070741851644053111, -0.4265091863517060933 ) ) ;
#55423=CARTESIAN_POINT ( 'NONE',  ( -0.2867679344610367109, 0.2867679344610365444, -2.851069184548242763 ) ) ;
#55428=CARTESIAN_POINT ( 'NONE',  ( -0.3949938075777411073, 0.1058382717557497660, -1.054461942257217899 ) ) ;
#55433=CARTESIAN_POINT ( 'NONE',  ( 0.2362204724409449064, 0.4091458600556404646, -1.246719160104986734 ) ) ;
#55434=CARTESIAN_POINT ( 'NONE',  ( 4.893765752498283924E-17, -0.3996062992125986035, -2.125984251968504157 ) ) ;
#55437=CARTESIAN_POINT ( 'NONE',  ( -9.594673741351313045E-17, 0.3917322834645670659, -0.6266597357293457460 ) ) ;
#55448=CARTESIAN_POINT ( 'NONE',  ( -9.594673741351313045E-17, 0.3917322834645670104, -1.094488188976378007 ) ) ;
#55451=CARTESIAN_POINT ( 'NONE',  ( -0.3949938075777411628, 0.1058382717557497937, -1.292650918635170676 ) ) ;
#55452=ORIENTED_EDGE ( 'NONE', *, *, #44019, .T. ) ;
#55462=CARTESIAN_POINT ( 'NONE',  ( -9.594673741351313045E-17, 0.3917322834645670104, -0.08464566929133868212 ) ) ;
#55467=CARTESIAN_POINT ( 'NONE',  ( 0.1998031496062994405, -0.3460692066303958092, -2.139107611548556331 ) ) ;
#55469=ORIENTED_EDGE ( 'NONE', *, *, #61540, .F. ) ;
#55470=CARTESIAN_POINT ( 'NONE',  ( -0.3996062992125985480, -7.340648628747423112E-17, -1.533464566929133799 ) ) ;
#55474=CARTESIAN_POINT ( 'NONE',  ( 5.785732909357575061E-17, -0.4724409448818898682, -0.3937007874015748254 ) ) ;
#55476=CARTESIAN_POINT ( 'NONE',  ( 0.2867679344610365999, 0.2867679344610365999, -2.584645669291338876 ) ) ;
#55483=CARTESIAN_POINT ( 'NONE',  ( -0.3458507752293909498, 0.3458507752293907833, -2.458661417322834719 ) ) ;
#55485=CARTESIAN_POINT ( 'NONE',  ( -0.3420746716998662729, 0.1974969037888702206, -1.992782152230971882 ) ) ;
#55496=CARTESIAN_POINT ( 'NONE',  ( 0.1958661417322834497, 0.3392501089628018329, -2.429114542485877770 ) ) ;
#55509=CARTESIAN_POINT ( 'NONE',  ( -0.1998031496062994405, 0.3460692066303957537, -0.7198162729658792447 ) ) ;
#55510=CARTESIAN_POINT ( 'NONE',  ( 0.2867679344610365999, -0.2867679344610365444, -1.915354330708661124 ) ) ;
#55519=CARTESIAN_POINT ( 'NONE',  ( -0.3996062992125985480, -7.340648628747423112E-17, -1.533464566929134021 ) ) ;
#55526=CARTESIAN_POINT ( 'NONE',  ( -0.1049643490035307020, 0.3917322834645669549, -1.508530183727033736 ) ) ;
#55527=CARTESIAN_POINT ( 'NONE',  ( 0.2362204724409451007, -0.4091458600556402980, -2.139107611548556331 ) ) ;
#55530=DIRECTION ( 'NONE',  ( 0.000000000000000000, 0.000000000000000000, 1.000000000000000000 ) ) ;
#55531=CARTESIAN_POINT ( 'NONE',  ( 0.3996062992125985480, -0.1070741851644052972, -2.235564304461942431 ) ) ;
#55533=CARTESIAN_POINT ( 'NONE',  ( -0.1998031496062994683, 0.3460692066303958092, -0.8005249343832020470 ) ) ;
#55536=CARTESIAN_POINT ( 'NONE',  ( -0.2867679344610365999, 0.2867679344610364889, -2.846456692913385655 ) ) ;
#55544=FACE_OUTER_BOUND ( 'NONE', #74101, .T. ) ;
#55547=CARTESIAN_POINT ( 'NONE',  ( -0.3917322834645670659, 0.1049643490035301607, -1.845125041173541369 ) ) ;
#55550=CARTESIAN_POINT ( 'NONE',  ( -0.3917322834645671215, 0.1049643490035301469, 0.1325459317585302443 ) ) ;
#55553=CARTESIAN_POINT ( 'NONE',  ( -0.2891555358219908833, -0.2891555358219912164, -0.05905511811023628904 ) ) ;
#55562=CARTESIAN_POINT ( 'NONE',  ( -0.2867679344610367109, 0.2867679344610365444, -1.276266034941944127 ) ) ;
#55564=CARTESIAN_POINT ( 'NONE',  ( 0.2867679344610365999, 0.2867679344610365999, -2.112204724409449064 ) ) ;
#55569=CARTESIAN_POINT ( 'NONE',  ( -0.3996062992125986035, -7.340648628747425578E-17, -0.3543307086614173040 ) ) ;
#55571=CARTESIAN_POINT ( 'NONE',  ( 0.1070741851644054776, -0.3996062992125984925, -0.004593175853018378711 ) ) ;
#55573=CARTESIAN_POINT ( 'NONE',  ( 0.2925321140481932369, 0.2925321140481932369, -2.342519685039369914 ) ) ;
#55578=CARTESIAN_POINT ( 'NONE',  ( -0.1265901696524986964, -0.4724409448818899238, -1.093832020997375087 ) ) ;
#55581=CARTESIAN_POINT ( 'NONE',  ( -0.1974969037888706924, 0.3420746716998658843, -0.7198162729658792447 ) ) ;
#55594=CARTESIAN_POINT ( 'NONE',  ( -0.3460692066303957537, -0.1998031496062994405, -1.546587926509186639 ) ) ;
#55597=CARTESIAN_POINT ( 'NONE',  ( 0.3917322834645669549, 0.1049643490035304660, -1.691601049868766360 ) ) ;
#55599=CARTESIAN_POINT ( 'NONE',  ( -0.3876764156950357476, -0.05722014593895402568, 1.721458645558463398E-17 ) ) ;
#55621=CARTESIAN_POINT ( 'NONE',  ( -0.3917322834645671770, 0.1049643490035302024, -2.234271284285776371 ) ) ;
#55628=CARTESIAN_POINT ( 'NONE',  ( -0.3460692066303960868, 0.1998031496062990242, -1.128608923884514503 ) ) ;
#55629=CARTESIAN_POINT ( 'NONE',  ( 0.3917322834645670104, -0.1049643490035303273, -2.150918635170603554 ) ) ;
#55632=CARTESIAN_POINT ( 'NONE',  ( -0.3996062992125987146, 0.1070741851644051862, -2.867454068241469756 ) ) ;
#55633=CARTESIAN_POINT ( 'NONE',  ( 0.1058382717557499880, 0.3949938075777411073, -2.828083989501312345 ) ) ;
#55636=CARTESIAN_POINT ( 'NONE',  ( 0.2867679344610365999, -0.2867679344610365444, -1.192913385826771755 ) ) ;
#55638=CARTESIAN_POINT ( 'NONE',  ( -0.4724409448818898682, -8.678599364036362592E-17, -2.401574803149606474 ) ) ;
#55644=CARTESIAN_POINT ( 'NONE',  ( -0.1958661417322834497, -0.3392501089628018884, -0.3031302905173735573 ) ) ;
#55651=DIRECTION ( 'NONE',  ( 0.000000000000000000, 0.000000000000000000, 1.000000000000000000 ) ) ;
#55652=CARTESIAN_POINT ( 'NONE',  ( -0.1049643490035302301, -0.3917322834645671770, -1.801200418144043969 ) ) ;
#55658=CARTESIAN_POINT ( 'NONE',  ( -0.1958661417322834220, -0.3392501089628018884, -0.7801837270341208663 ) ) ;
#55669=CARTESIAN_POINT ( 'NONE',  ( -0.1049643490035302024, -0.3917322834645671215, -2.898950131233595684 ) ) ;
#55676=CARTESIAN_POINT ( 'NONE',  ( 0.3917322834645669549, 0.1049643490035304660, -0.8392388451443569819 ) ) ;
#55679=VECTOR ( 'NONE', #75744, 39.37007874015748143 ) ;
#55680=CARTESIAN_POINT ( 'NONE',  ( 4.893765752498283308E-17, -0.3996062992125985480, -2.517716535433071279 ) ) ;
#55690=CARTESIAN_POINT ( 'NONE',  ( -9.787531504996566615E-17, 0.3996062992125985480, -0.5492125984251968740 ) ) ;
#55692=DIRECTION ( 'NONE',  ( 0.000000000000000000, 1.000000000000000000, 0.000000000000000000 ) ) ;
#55699=CARTESIAN_POINT ( 'NONE',  ( 0.3392501089628018329, -0.1958661417322834497, -1.602342888942570154 ) ) ;
#55708=CARTESIAN_POINT ( 'NONE',  ( 0.3392501089628018884, -0.1958661417322833942, -0.4166859824485057984 ) ) ;
#55712=CARTESIAN_POINT ( 'NONE',  ( 5.785732909357575061E-17, -0.4724409448818898682, -2.202755905511811108 ) ) ;
#55735=CARTESIAN_POINT ( 'NONE',  ( 0.2925321140481932369, 0.2925321140481932369, -2.419291338582676865 ) ) ;
#55740=CARTESIAN_POINT ( 'NONE',  ( -0.1070741851644056997, 0.3996062992125986035, -1.738845144356955696 ) ) ;
#55741=CARTESIAN_POINT ( 'NONE',  ( 0.3420746716998660508, -0.1974969037888703871, -1.679790026246719359 ) ) ;
#55744=CARTESIAN_POINT ( 'NONE',  ( 0.1958661417322836440, -0.3392501089628017219, -0.5564304461942257696 ) ) ;
#55748=CARTESIAN_POINT ( 'NONE',  ( -0.3949938075777409963, -7.255918531996591613E-17, -2.163385826771653697 ) ) ;
#55752=CARTESIAN_POINT ( 'NONE',  ( -0.2362204724409447953, -0.4091458600556404646, -2.270341207349081181 ) ) ;
#55753=CARTESIAN_POINT ( 'NONE',  ( -0.1070741851644056997, 0.3996062992125986035, -1.581364829396325389 ) ) ;
#55761=CARTESIAN_POINT ( 'NONE',  ( 0.3392501089628018329, 0.1958661417322835052, -2.730951812827084435 ) ) ;
#55767=CARTESIAN_POINT ( 'NONE',  ( -0.2867679344610364334, -0.2867679344610367109, -0.1437007874015748810 ) ) ;
#55769=CARTESIAN_POINT ( 'NONE',  ( 0.2867679344610365999, 0.2867679344610365999, -2.492125984251968518 ) ) ;
#55771=ORIENTED_EDGE ( 'NONE', *, *, #61540, .T. ) ;
#55772=CARTESIAN_POINT ( 'NONE',  ( -0.1058382717557497937, -0.3949938075777411628, -2.906824146981628054 ) ) ;
#55776=CARTESIAN_POINT ( 'NONE',  ( 0.3460692066303959757, -0.1998031496062991907, -1.207349081364829324 ) ) ;
#55781=CARTESIAN_POINT ( 'NONE',  ( -0.2867679344610364334, -0.2867679344610367109, -0.4586614173228347746 ) ) ;
#55789=CARTESIAN_POINT ( 'NONE',  ( -0.1049643490035302024, -0.3917322834645671215, -0.2217847769028870319 ) ) ;
#55793=CARTESIAN_POINT ( 'NONE',  ( -0.1265901696524993347, 0.4724409448818895907, -1.581364829396325389 ) ) ;
#55802=CARTESIAN_POINT ( 'NONE',  ( -9.594673741351310580E-17, 0.3917322834645669549, -0.3949938075777409963 ) ) ;
#55804=CARTESIAN_POINT ( 'NONE',  ( 0.3917322834645670104, -0.1049643490035303273, -0.5111548556430446366 ) ) ;
#55809=CARTESIAN_POINT ( 'NONE',  ( 0.3917322834645669549, 0.1049643490035304660, -2.164041994750655729 ) ) ;
#55813=CARTESIAN_POINT ( 'NONE',  ( -0.4724409448818895907, -0.1265901696524993070, -0.9101049868766404316 ) ) ;
#55824=CARTESIAN_POINT ( 'NONE',  ( 0.1070741851644053388, 0.3996062992125986035, -1.802493438320209584 ) ) ;
#55825=EDGE_CURVE ( 'NONE', #18415, #21240, #22574, .T. ) ;
#55833=CARTESIAN_POINT ( 'NONE',  ( 0.1070741851644053527, 0.3996062992125985480, -0.3851706036745407014 ) ) ;
#55834=CARTESIAN_POINT ( 'NONE',  ( -0.3996062992125986035, -0.1070741851644056997, -0.3608923884514435576 ) ) ;
#55835=CARTESIAN_POINT ( 'NONE',  ( 0.3420746716998659953, 0.1974969037888705536, 0.02624671916010492753 ) ) ;
#55839=CARTESIAN_POINT ( 'NONE',  ( 0.4091458600556404646, -0.2362204724409448231, -2.386482939632545985 ) ) ;
#55840=CARTESIAN_POINT ( 'NONE',  ( -0.1058382717557503072, 0.3949938075777408852, -0.7132545931758530466 ) ) ;
#55845=CARTESIAN_POINT ( 'NONE',  ( 5.785732909357575061E-17, -0.4724409448818898682, -1.338582677165354173 ) ) ;
#55846=CARTESIAN_POINT ( 'NONE',  ( 0.3460692066303959202, 0.1998031496062993295, -2.493438320209973469 ) ) ;
#55850=CARTESIAN_POINT ( 'NONE',  ( -0.3392501089628019995, 0.1958661417322831999, -0.6529064548894508713 ) ) ;
#55861=CARTESIAN_POINT ( 'NONE',  ( -0.3917322834645670104, -7.196005306013484475E-17, -0.9763779527559053317 ) ) ;
#55864=CARTESIAN_POINT ( 'NONE',  ( -0.3420746716998659953, -0.1974969037888706647, -1.469816272965879245 ) ) ;
#55872=EDGE_CURVE ( 'NONE', #24385, #50887, #2394, .T. ) ;
#55876=CARTESIAN_POINT ( 'NONE',  ( -0.3392501089628017219, -0.1958661417322836718, -0.1371391076115486551 ) ) ;
#55883=CARTESIAN_POINT ( 'NONE',  ( -0.1998031496062991907, -0.3460692066303959757, -2.112860892388451539 ) ) ;
#55886=CARTESIAN_POINT ( 'NONE',  ( -0.3996062992125986590, 0.1070741851644051723, -1.526902887139107490 ) ) ;
#55890=CARTESIAN_POINT ( 'NONE',  ( 0.1265901696524989462, 0.4724409448818897572, -0.4658792650918635592 ) ) ;
#55891=LINE ( 'NONE', #63050, #81535 ) ;
#55892=CARTESIAN_POINT ( 'NONE',  ( -9.594673741351313045E-17, 0.3917322834645670104, 0.1653543307086614844 ) ) ;
#55900=CARTESIAN_POINT ( 'NONE',  ( 0.3458507752293908943, -0.3458507752293908943, -2.222440944881889813 ) ) ;
#55902=CARTESIAN_POINT ( 'NONE',  ( 4.837279021331061486E-17, -0.3949938075777409963, -2.202755905511811108 ) ) ;
#55914=FACE_OUTER_BOUND ( 'NONE', #64752, .T. ) ;
#55923=CARTESIAN_POINT ( 'NONE',  ( -0.3460692066303960313, 0.1998031496062989965, -0.7329396325459317518 ) ) ;
#55924=CARTESIAN_POINT ( 'NONE',  ( 4.797336870675656522E-17, -0.3917322834645670104, -2.210629921259842590 ) ) ;
#55935=ORIENTED_EDGE ( 'NONE', *, *, #27502, .T. ) ;
#55940=CARTESIAN_POINT ( 'NONE',  ( -0.1958661417322836718, 0.3392501089628017219, -1.515091863517060489 ) ) ;
#55947=CARTESIAN_POINT ( 'NONE',  ( 0.3996062992125984925, 0.1070741851644054499, -2.563648293963254776 ) ) ;
#55948=AXIS2_PLACEMENT_3D ( 'NONE', #13269, #72171, #78914 ) ;
#55950=CARTESIAN_POINT ( 'NONE',  ( -9.787531504996567848E-17, 0.3996062992125986035, -0.9448818897637796255 ) ) ;
#55953=CARTESIAN_POINT ( 'NONE',  ( -0.1958661417322836718, 0.3392501089628017219, -2.682414698162729483 ) ) ;
#55963=CARTESIAN_POINT ( 'NONE',  ( 0.2867679344610365999, -0.2867679344610365999, -1.910741839073804016 ) ) ;
#55966=CARTESIAN_POINT ( 'NONE',  ( -9.594673741351313045E-17, 0.3917322834645670104, 0.1653543307086614844 ) ) ;
#55969=CARTESIAN_POINT ( 'NONE',  ( 0.3420746716998660508, -0.1974969037888703871, -0.1049868766404199877 ) ) ;
#55979=CARTESIAN_POINT ( 'NONE',  ( 0.1958661417322834775, 0.3392501089628018884, -1.243457635991812582 ) ) ;
#55981=CARTESIAN_POINT ( 'NONE',  ( -0.1049643490035307020, 0.3917322834645669549, -2.768372703412072866 ) ) ;
#55986=CARTESIAN_POINT ( 'NONE',  ( -0.3996062992125987146, 0.1070741851644051862, -0.9776902887139107268 ) ) ;
#55988=CARTESIAN_POINT ( 'NONE',  ( 0.3460692066303959202, -0.1998031496062991630, -0.3392388451443569819 ) ) ;
#55990=CARTESIAN_POINT ( 'NONE',  ( -0.1998031496062994683, 0.3460692066303958092, -2.375328083989501238 ) ) ;
#55994=CARTESIAN_POINT ( 'NONE',  ( 0.2362204724409449064, 0.4091458600556404646, -1.008530183727034180 ) ) ;
#55998=CARTESIAN_POINT ( 'NONE',  ( 0.3949938075777409963, 2.418639510665530743E-17, -0.8248031496062994128 ) ) ;
#56000=CARTESIAN_POINT ( 'NONE',  ( 0.4724409448818898127, -0.1265901696524988629, -1.133202099737532720 ) ) ;
#56010=CARTESIAN_POINT ( 'NONE',  ( 0.3996062992125984925, 0.1070741851644054637, -1.776246719160104570 ) ) ;
#56012=AXIS2_PLACEMENT_3D ( 'NONE', #63259, #12341, #124 ) ;
#56013=CARTESIAN_POINT ( 'NONE',  ( -0.1958661417322834220, -0.3392501089628018884, -1.475065616797900381 ) ) ;
#56028=CARTESIAN_POINT ( 'NONE',  ( -0.2867679344610365999, 0.2867679344610364889, -1.049212598425196763 ) ) ;
#56042=CARTESIAN_POINT ( 'NONE',  ( -0.4724409448818891466, -0.1265901696525000564, -0.5183727034120735322 ) ) ;
#56046=CARTESIAN_POINT ( 'NONE',  ( 0.1958661417322836440, -0.3392501089628017219, -1.973753280839895208 ) ) ;
#56049=CARTESIAN_POINT ( 'NONE',  ( -0.4724409448818899238, 0.1265901696524986686, -0.1902887139107611314 ) ) ;
#56050=CARTESIAN_POINT ( 'NONE',  ( 0.3420746716998660508, -0.1974969037888703871, -2.939632545931758489 ) ) ;
#56053=CARTESIAN_POINT ( 'NONE',  ( -0.3917322834645671215, 0.1049643490035301469, -1.284776902887139194 ) ) ;
#56055=CARTESIAN_POINT ( 'NONE',  ( -0.3458507752293909498, 0.3458507752293907833, -2.539370078740157410 ) ) ;
#56061=CARTESIAN_POINT ( 'NONE',  ( 0.3392501089628018329, 0.1958661417322835052, -0.6837077183388958757 ) ) ;
#56071=CARTESIAN_POINT ( 'NONE',  ( -0.3917322834645670659, -7.196005306013484475E-17, -2.240832964075802458 ) ) ;
#56079=CARTESIAN_POINT ( 'NONE',  ( -0.1958661417322836718, 0.3392501089628017219, -1.515091863517060489 ) ) ;
#56089=CARTESIAN_POINT ( 'NONE',  ( 0.3392501089628018884, -0.1958661417322834220, -2.616797900262466836 ) ) ;
#56096=CARTESIAN_POINT ( 'NONE',  ( 4.797336870675656522E-17, -0.3917322834645670104, -0.7933070866141732624 ) ) ;
#56097=CARTESIAN_POINT ( 'NONE',  ( -0.1265901696524986964, -0.4724409448818899238, 0.1660104986876640432 ) ) ;
#56099=CARTESIAN_POINT ( 'NONE',  ( 0.3996062992125984925, 0.1070741851644054637, -2.563648293963254776 ) ) ;
#56108=CARTESIAN_POINT ( 'NONE',  ( -0.2925321140481930149, -0.2925321140481933480, -0.6082677165354329896 ) ) ;
#56110=CARTESIAN_POINT ( 'NONE',  ( -0.2867679344610364334, -0.2867679344610367109, -0.05118110236220468900 ) ) ;
#56117=CARTESIAN_POINT ( 'NONE',  ( -0.3392501089628018329, -0.1958661417322836440, -1.549849450622360791 ) ) ;
#56126=CARTESIAN_POINT ( 'NONE',  ( 0.1958661417322834775, 0.3392501089628018884, -0.9284970060705530770 ) ) ;
#56131=CARTESIAN_POINT ( 'NONE',  ( 0.4724409448818898682, 2.892866454678787531E-17, -1.927165354330708569 ) ) ;
#56145=DIMENSIONAL_EXPONENTS ( 1.000000000000000000, 0.000000000000000000, 0.000000000000000000, 0.000000000000000000, 0.000000000000000000, 0.000000000000000000, 0.000000000000000000 ) ;
#56153=CARTESIAN_POINT ( 'NONE',  ( 0.1998031496062994128, -0.3460692066303957537, -2.688320209973753538 ) ) ;
#56158=CARTESIAN_POINT ( 'NONE',  ( -0.3996062992125986035, -7.340648628747425578E-17, -2.401574803149606474 ) ) ;
#56159=CARTESIAN_POINT ( 'NONE',  ( 0.1058382717557499880, 0.3949938075777411073, -1.568241469816272993 ) ) ;
#56160=CARTESIAN_POINT ( 'NONE',  ( 0.3460692066303959757, -0.1998031496062991907, -2.782152230971128848 ) ) ;
#56162=CARTESIAN_POINT ( 'NONE',  ( -0.3917322834645669549, -0.1049643490035306603, -0.6679790026246718027 ) ) ;
#56166=CARTESIAN_POINT ( 'NONE',  ( -0.1058382717557497660, -0.3949938075777411073, -2.668635170603674833 ) ) ;
#56170=CARTESIAN_POINT ( 'NONE',  ( -0.2362204724409447953, -0.4091458600556404646, -2.585301837270341352 ) ) ;
#56171=CARTESIAN_POINT ( 'NONE',  ( 4.893765752498283924E-17, -0.3996062992125986035, -2.283464566929133799 ) ) ;
#56178=CARTESIAN_POINT ( 'NONE',  ( -0.1049643490035301746, -0.3917322834645670659, -2.671896694716848764 ) ) ;
#56185=CARTESIAN_POINT ( 'NONE',  ( -9.594673741351313045E-17, 0.3917322834645670104, -0.5570866141732284671 ) ) ;
#56187=CARTESIAN_POINT ( 'NONE',  ( -0.2867679344610365999, 0.2867679344610364889, -1.586614173228346747 ) ) ;
#56188=CARTESIAN_POINT ( 'NONE',  ( -0.3392501089628017219, -0.1958661417322836718, -2.249343832020997525 ) ) ;
#56191=CARTESIAN_POINT ( 'NONE',  ( 0.1974969037888706369, -0.3420746716998659953, -2.611548556430445700 ) ) ;
#56196=CARTESIAN_POINT ( 'NONE',  ( -0.1070741851644051862, -0.3996062992125987146, -1.646981627296587591 ) ) ;
#56199=DIRECTION ( 'NONE',  ( 1.000000000000000000, 0.000000000000000000, 0.000000000000000000 ) ) ;
#56201=CARTESIAN_POINT ( 'NONE',  ( -0.1958661417322834220, -0.3392501089628018884, -0.3077427821522311091 ) ) ;
#56206=CARTESIAN_POINT ( 'NONE',  ( 0.3392501089628018884, -0.1958661417322834220, -0.09711286089238840846 ) ) ;
#56211=CARTESIAN_POINT ( 'NONE',  ( 0.2362204724409451007, -0.4091458600556402980, -1.509186351706036655 ) ) ;
#56214=( BOUNDED_CURVE ( )  B_SPLINE_CURVE ( 2, ( #78637, #46619, #28922, #54590, #9167, #72314, #60499, #80300, #28099, #22614, #14661, #48274, #15488 ),
 .UNSPECIFIED., .F., .F. ) 
 B_SPLINE_CURVE_WITH_KNOTS ( ( 3, 2, 2, 2, 2, 2, 3 ),
 ( 0.6881378855240347647, 0.6916666666666666519, 0.6958333333333333037, 0.6999999999999999556, 0.7041666666666666075, 0.7083333333333332593, 0.7124999999999999112 ),
 .UNSPECIFIED. ) 
 CURVE ( )  GEOMETRIC_REPRESENTATION_ITEM ( )  RATIONAL_B_SPLINE_CURVE ( ( 0.9911642120907970810, 0.9711423276059441001, 1.000000000000000000, 0.9659258262890683122, 1.000000000000000000, 0.9659258262890683122, 1.000000000000000000, 0.9659258262890683122, 1.000000000000000000, 0.9659258262890683122, 1.000000000000000000, 0.9659258262890692004, 0.9999999999999991118 ) ) 
 REPRESENTATION_ITEM ( '' )  );
#56225=CARTESIAN_POINT ( 'NONE',  ( -0.1049643490035301746, -0.3917322834645670659, -0.4671722852680298410 ) ) ;
#56227=CARTESIAN_POINT ( 'NONE',  ( -0.2867679344610366554, 0.2867679344610365444, -1.049212598425196985 ) ) ;
#56232=CARTESIAN_POINT ( 'NONE',  ( 0.3917322834645670104, 2.398668435337828261E-17, -2.314960629921259727 ) ) ;
#56236=CARTESIAN_POINT ( 'NONE',  ( 0.4724409448818898682, 2.892866454678787531E-17, -0.6673228346456693272 ) ) ;
#56247=CARTESIAN_POINT ( 'NONE',  ( -0.3996062992125985480, -7.340648628747423112E-17, -2.005905511811023612 ) ) ;
#56255=CARTESIAN_POINT ( 'NONE',  ( 0.1070741851644054637, -0.3996062992125984925, -0.6345144356955381149 ) ) ;
#56256=CARTESIAN_POINT ( 'NONE',  ( -0.3996062992125986035, -7.340648628747425578E-17, -0.5118110236220472231 ) ) ;
#56257=CARTESIAN_POINT ( 'NONE',  ( 0.1058382717557500713, -0.3949938075777409408, -0.08530183727034125474 ) ) ;
#56262=CARTESIAN_POINT ( 'NONE',  ( 0.1265901696524990572, -0.4724409448818897017, -2.366797900262467280 ) ) ;
#56263=CARTESIAN_POINT ( 'NONE',  ( -0.1974969037888706924, 0.3420746716998658843, -0.7198162729658792447 ) ) ;
#56268=CARTESIAN_POINT ( 'NONE',  ( -0.3458507752293906723, -0.3458507752293910609, -1.318897637795275690 ) ) ;
#56269=CARTESIAN_POINT ( 'NONE',  ( 0.3460692066303959757, -0.1998031496062991907, -2.152230971128608950 ) ) ;
#56272=CARTESIAN_POINT ( 'NONE',  ( -0.1958661417322833942, -0.3392501089628018884, -0.6922765336296082817 ) ) ;
#56284=CARTESIAN_POINT ( 'NONE',  ( -0.3392501089628019995, 0.1958661417322832277, -0.9632545931758529356 ) ) ;
#56287=CARTESIAN_POINT ( 'NONE',  ( -9.674558042662121740E-17, 0.3949938075777409963, -1.417322834645669216 ) ) ;
#56292=CARTESIAN_POINT ( 'NONE',  ( 0.3996062992125986590, -0.1070741851644053111, 0.04593175853018371946 ) ) ;
#56299=CARTESIAN_POINT ( 'NONE',  ( -0.1049643490035302024, -0.3917322834645671215, 0.1581364829396324501 ) ) ;
#56305=CARTESIAN_POINT ( 'NONE',  ( -0.3996062992125986035, -0.1070741851644056997, -1.935695538057742526 ) ) ;
#56308=CARTESIAN_POINT ( 'NONE',  ( -0.1070741851644056997, 0.3996062992125984925, -1.658136482939632117 ) ) ;
#56312=CARTESIAN_POINT ( 'NONE',  ( -0.4724409448818895907, -0.1265901696524993070, -0.3608923884514435576 ) ) ;
#56314=CARTESIAN_POINT ( 'NONE',  ( -0.3917322834645670104, -7.196005306013484475E-17, 0.1259842519685039908 ) ) ;
#56320=CARTESIAN_POINT ( 'NONE',  ( 0.4091458600556404646, -0.2362204724409448231, -2.543963254593176071 ) ) ;
#56322=CARTESIAN_POINT ( 'NONE',  ( -0.2891555358219911054, 0.2891555358219909388, -2.301181102362205078 ) ) ;
#56328=CARTESIAN_POINT ( 'NONE',  ( -0.3458507752293906723, -0.3458507752293910609, -2.183070866141731958 ) ) ;
#56333=DIRECTION ( 'NONE',  ( -0.000000000000000000, -0.000000000000000000, 1.000000000000000000 ) ) ;
#56343=CARTESIAN_POINT ( 'NONE',  ( -0.1070741851644051862, -0.3996062992125986590, -0.7788713910761155823 ) ) ;
#56344=CARTESIAN_POINT ( 'NONE',  ( 0.2867679344610365999, 0.2867679344610365999, -2.112204724409449064 ) ) ;
#56362=CARTESIAN_POINT ( 'NONE',  ( -0.1958661417322836718, 0.3392501089628017219, -1.357611548556430625 ) ) ;
#56363=CARTESIAN_POINT ( 'NONE',  ( -0.09865214182458049985, 0.3796925558546804247, -1.220472440944881498 ) ) ;
#56366=CARTESIAN_POINT ( 'NONE',  ( 0.3458507752293908943, 0.3458507752293908943, -0.4527559055118110520 ) ) ;
#56367=CARTESIAN_POINT ( 'NONE',  ( 0.2925321140481931814, -0.2925321140481931259, -2.537401574803149984 ) ) ;
#56369=CARTESIAN_POINT ( 'NONE',  ( 0.3996062992125986035, 2.446882876249141962E-17, -0.7480314960629921295 ) ) ;
#56372=CARTESIAN_POINT ( 'NONE',  ( 0.3392501089628018884, -0.1958661417322834220, -2.616797900262466836 ) ) ;
#56373=ORIENTED_EDGE ( 'NONE', *, *, #6822, .T. ) ;
#56384=CARTESIAN_POINT ( 'NONE',  ( -0.1049643490035302024, -0.3917322834645671215, -2.676509186351705871 ) ) ;
#56387=CARTESIAN_POINT ( 'NONE',  ( -0.1058382717557503211, 0.3949938075777409408, -0.3215223097112862027 ) ) ;
#56395=CARTESIAN_POINT ( 'NONE',  ( 0.3917322834645670659, 2.398668435337828261E-17, -1.689651861713597603 ) ) ;
#56397=CARTESIAN_POINT ( 'NONE',  ( -9.594673741351313045E-17, 0.3917322834645670104, -2.446850393700787496 ) ) ;
#56402=CARTESIAN_POINT ( 'NONE',  ( -0.3460692066303960868, 0.1998031496062990242, -0.9711286089238845287 ) ) ;
#56404=CARTESIAN_POINT ( 'NONE',  ( -0.3460692066303957537, -0.1998031496062994405, -0.1292650918635170620 ) ) ;
#56406=CARTESIAN_POINT ( 'NONE',  ( 0.1070741851644053527, 0.3996062992125986590, -2.198162729658792447 ) ) ;
#56407=CARTESIAN_POINT ( 'NONE',  ( -0.1049643490035307020, 0.3917322834645669549, -1.823490813648294129 ) ) ;
#56411=CARTESIAN_POINT ( 'NONE',  ( 0.3458507752293908943, -0.3458507752293908943, -0.9625984251968502381 ) ) ;
#56414=CARTESIAN_POINT ( 'NONE',  ( 0.3949938075777409408, -0.1058382717557499186, -0.9757217847769031893 ) ) ;
#56425=CARTESIAN_POINT ( 'NONE',  ( -0.3996062992125985480, -7.340648628747423112E-17, -1.690944881889763884 ) ) ;
#56438=CARTESIAN_POINT ( 'NONE',  ( 0.1958661417322834775, 0.3392501089628018884, -1.016404199475065662 ) ) ;
#56457=CARTESIAN_POINT ( 'NONE',  ( 0.3996062992125986035, 2.446882876249141962E-17, -1.062992125984252079 ) ) ;
#56459=CARTESIAN_POINT ( 'NONE',  ( -0.2867679344610364334, -0.2867679344610367109, -1.940944881889763884 ) ) ;
#56462=CARTESIAN_POINT ( 'NONE',  ( -0.1265901696524986964, -0.4724409448818899238, -0.3871391076115485719 ) ) ;
#56463=CARTESIAN_POINT ( 'NONE',  ( 0.3949938075777411073, -0.1058382717557499464, -2.788713910761155379 ) ) ;
#56466=CARTESIAN_POINT ( 'NONE',  ( -0.3917322834645670104, -7.196005306013484475E-17, -1.448818897637795367 ) ) ;
#56469=CARTESIAN_POINT ( 'NONE',  ( 0.1265901696524989462, 0.4724409448818897572, -2.355643044619422533 ) ) ;
#56474=CARTESIAN_POINT ( 'NONE',  ( 0.1958661417322834497, 0.3392501089628018329, -0.5393507629583185192 ) ) ;
#56481=CARTESIAN_POINT ( 'NONE',  ( 0.1049643490035304799, -0.3917322834645670104, -2.129284407645356314 ) ) ;
#56483=VERTEX_POINT ( 'NONE', #4861 ) ;
#56489=CARTESIAN_POINT ( 'NONE',  ( 0.3917322834645670104, -0.1049643490035303411, -1.456036745406824151 ) ) ;
#56498=CARTESIAN_POINT ( 'NONE',  ( -0.1958661417322834220, -0.3392501089628018884, -2.577427821522309426 ) ) ;
#56505=CARTESIAN_POINT ( 'NONE',  ( 0.3392501089628018884, -0.1958661417322834220, -1.291994750656167978 ) ) ;
#56508=CARTESIAN_POINT ( 'NONE',  ( -0.1058382717557497660, -0.3949938075777411073, 0.1660104986876640432 ) ) ;
#56517=CARTESIAN_POINT ( 'NONE',  ( -0.3460692066303960313, 0.1998031496062989965, -0.4179790026246719137 ) ) ;
#56520=CARTESIAN_POINT ( 'NONE',  ( -0.3917322834645671215, 0.1049643490035301469, -0.1824146981627296216 ) ) ;
#56536=CARTESIAN_POINT ( 'NONE',  ( -0.3917322834645670659, -7.196005306013484475E-17, -0.9809904443907629945 ) ) ;
#56538=ADVANCED_FACE ( 'NONE', ( #42740 ), #30535, .T. ) ;
#56541=CARTESIAN_POINT ( 'NONE',  ( 0.2362204724409449064, 0.4091458600556404646, -1.953412073490813805 ) ) ;
#56561=CARTESIAN_POINT ( 'NONE',  ( 4.893765752498283308E-17, -0.3996062992125985480, -2.517716535433071279 ) ) ;
#56566=CARTESIAN_POINT ( 'NONE',  ( -0.2925321140481932924, 0.2925321140481931814, -2.224409448818897239 ) ) ;
#56567=CARTESIAN_POINT ( 'NONE',  ( 0.1974969037888706369, -0.3420746716998659953, -1.666666666666666741 ) ) ;
#56570=CARTESIAN_POINT ( 'NONE',  ( -0.3392501089628019995, 0.1958661417322832277, -0.4908136482939632339 ) ) ;
#56574=CARTESIAN_POINT ( 'NONE',  ( -9.674558042662122972E-17, 0.3949938075777409963, -2.438976377952756014 ) ) ;
#56578=CARTESIAN_POINT ( 'NONE',  ( 0.1265901696524989462, 0.4724409448818897572, -2.828083989501312345 ) ) ;
#56579=CARTESIAN_POINT ( 'NONE',  ( -0.3996062992125987146, 0.1070741851644051862, -2.080052493438320216 ) ) ;
#56585=CARTESIAN_POINT ( 'NONE',  ( -0.3917322834645670104, -7.196005306013484475E-17, -0.2814960629921260393 ) ) ;
#56593=CARTESIAN_POINT ( 'NONE',  ( 0.1049643490035304938, -0.3917322834645669549, -0.6423884514435697080 ) ) ;
#56594=CARTESIAN_POINT ( 'NONE',  ( -0.2867679344610365999, 0.2867679344610364889, -1.429133858267716661 ) ) ;
#56595=CARTESIAN_POINT ( 'NONE',  ( 0.1049643490035303689, 0.3917322834645670104, -2.505249343832020248 ) ) ;
#56598=CARTESIAN_POINT ( 'NONE',  ( -0.1058382717557503211, 0.3949938075777409408, -2.683727034120735766 ) ) ;
#56602=CARTESIAN_POINT ( 'NONE',  ( 0.2925321140481932369, 0.2925321140481932369, -1.397637795275590067 ) ) ;
#56607=CARTESIAN_POINT ( 'NONE',  ( 0.1958661417322836440, -0.3392501089628017219, -0.3339895013123360679 ) ) ;
#56613=VERTEX_POINT ( 'NONE', #81900 ) ;
#56617=CARTESIAN_POINT ( 'NONE',  ( -0.4724409448818898682, -8.678599364036362592E-17, -1.929133858267716439 ) ) ;
#56623=CARTESIAN_POINT ( 'NONE',  ( 0.3458507752293908943, -0.3458507752293908943, -2.303149606299212060 ) ) ;
#56627=CARTESIAN_POINT ( 'NONE',  ( -0.3392501089628019439, 0.1958661417322832554, -0.2637602117772160915 ) ) ;
#56629=CARTESIAN_POINT ( 'NONE',  ( 0.2867679344610366554, 0.2867679344610366554, -0.8523622047244096001 ) ) ;
#56634=CARTESIAN_POINT ( 'NONE',  ( 0.2867679344610365999, -0.2867679344610365444, -2.767716535433069946 ) ) ;
#56637=CARTESIAN_POINT ( 'NONE',  ( -0.2362204724409451284, 0.4091458600556402425, -0.7198162729658792447 ) ) ;
#56650=CARTESIAN_POINT ( 'NONE',  ( -0.1070741851644056997, 0.3996062992125984925, -1.815616797900262425 ) ) ;
#56658=CARTESIAN_POINT ( 'NONE',  ( -0.3460692066303960313, 0.1998031496062989965, -0.7329396325459317518 ) ) ;
#56659=CARTESIAN_POINT ( 'NONE',  ( -0.1070741851644056997, 0.3996062992125986035, -1.108923884514435798 ) ) ;
#56660=CARTESIAN_POINT ( 'NONE',  ( 0.3949938075777409963, 2.418639510665530435E-17, -0.2755905511811024278 ) ) ;
#56667=CARTESIAN_POINT ( 'NONE',  ( 0.1974969037888704704, 0.3420746716998660508, -1.480971128608923548 ) ) ;
#56672=CARTESIAN_POINT ( 'NONE',  ( -0.3458507752293906723, -0.3458507752293910609, -1.791338582677165059 ) ) ;
#56680=DIMENSIONAL_EXPONENTS ( 1.000000000000000000, 0.000000000000000000, 0.000000000000000000, 0.000000000000000000, 0.000000000000000000, 0.000000000000000000, 0.000000000000000000 ) ;
#56688=CARTESIAN_POINT ( 'NONE',  ( 0.3917322834645670104, 2.398668435337828261E-17, -1.370078740157480324 ) ) ;
#56691=CARTESIAN_POINT ( 'NONE',  ( 0.3949938075777411073, -0.1058382717557499464, -1.371391076115485719 ) ) ;
#56692=ORIENTED_EDGE ( 'NONE', *, *, #59375, .T. ) ;
#56696=CARTESIAN_POINT ( 'NONE',  ( -0.2925321140481930704, -0.2925321140481933480, -0.05905511811023621965 ) ) ;
#56703=CARTESIAN_POINT ( 'NONE',  ( 0.3392501089628018884, -0.1958661417322834220, 0.1253280839895012100 ) ) ;
#56709=CARTESIAN_POINT ( 'NONE',  ( 0.3996062992125986035, 0.1070741851644054776, -2.014435695538057569 ) ) ;
#56712=CARTESIAN_POINT ( 'NONE',  ( -9.787531504996566615E-17, 0.3996062992125985480, -1.651574803149606474 ) ) ;
#56718=CARTESIAN_POINT ( 'NONE',  ( -0.4724409448818899238, 0.1265901696524986686, -0.9776902887139107268 ) ) ;
#56720=CARTESIAN_POINT ( 'NONE',  ( -0.1958661417322834220, -0.3392501089628018884, 0.09973753280839900426 ) ) ;
#56726=CARTESIAN_POINT ( 'NONE',  ( 0.4091458600556404646, -0.2362204724409448231, -2.858923884514435798 ) ) ;
#56728=CARTESIAN_POINT ( 'NONE',  ( 0.3949938075777408852, 0.1058382717557500435, -2.248687664041995049 ) ) ;
#56749=CARTESIAN_POINT ( 'NONE',  ( -0.3460692066303960313, 0.1998031496062989965, -0.8904199475065617264 ) ) ;
#56750=CARTESIAN_POINT ( 'NONE',  ( -0.2867679344610365999, 0.2867679344610364889, -2.309055118110235671 ) ) ;
#56766=CARTESIAN_POINT ( 'NONE',  ( -0.3917322834645671215, 0.1049643490035301469, -2.007217847769029007 ) ) ;
#56767=CARTESIAN_POINT ( 'NONE',  ( 0.2155943732411896574, 0.3272402980636398007, -1.220472440944881942 ) ) ;
#56771=CARTESIAN_POINT ( 'NONE',  ( -0.1998031496062991630, -0.3460692066303959202, -2.662073490813648746 ) ) ;
#56773=CARTESIAN_POINT ( 'NONE',  ( -0.1998031496062994683, 0.3460692066303958092, -1.115485564304461885 ) ) ;
#56775=CARTESIAN_POINT ( 'NONE',  ( 4.797336870675656522E-17, -0.3917322834645670104, -2.748031496062991685 ) ) ;
#56788=CARTESIAN_POINT ( 'NONE',  ( -0.3917322834645670104, -7.196005306013484475E-17, 0.1259842519685039908 ) ) ;
#56791=CARTESIAN_POINT ( 'NONE',  ( -9.674558042662121740E-17, 0.3949938075777409963, -0.3149606299212598937 ) ) ;
#56798=CARTESIAN_POINT ( 'NONE',  ( -0.3917322834645670104, -0.1049643490035307020, -1.617473384023309091 ) ) ;
#56801=CARTESIAN_POINT ( 'NONE',  ( -0.3392501089628017219, -0.1958661417322836718, -2.499343832020997080 ) ) ;
#56806=CARTESIAN_POINT ( 'NONE',  ( 0.3996062992125986035, 0.1070741851644054776, -0.9120734908136483021 ) ) ;
#56808=CARTESIAN_POINT ( 'NONE',  ( -9.787531504996566615E-17, 0.3996062992125985480, -0.2342519685039370358 ) ) ;
#56810=CARTESIAN_POINT ( 'NONE',  ( 4.893765752498283924E-17, -0.3996062992125986035, -2.283464566929133799 ) ) ;
#56811=CARTESIAN_POINT ( 'NONE',  ( -0.1958661417322834220, -0.3392501089628018884, -1.567585301837270295 ) ) ;
#56815=CARTESIAN_POINT ( 'NONE',  ( -0.4724409448818899238, 0.1265901696524986686, -1.211942257217847541 ) ) ;
#56819=CARTESIAN_POINT ( 'NONE',  ( -0.3949938075777409963, -7.255918531996591613E-17, -0.9035433070866141225 ) ) ;
#56821=CARTESIAN_POINT ( 'NONE',  ( 0.4091458600556404646, -0.2362204724409448231, -1.126640419947506633 ) ) ;
#56830=CARTESIAN_POINT ( 'NONE',  ( -0.3996062992125986590, 0.1070741851644051723, -1.841863517060367661 ) ) ;
#56845=CARTESIAN_POINT ( 'NONE',  ( -0.1049643490035307020, 0.3917322834645669549, -1.193569553805774452 ) ) ;
#56867=DIRECTION ( 'NONE',  ( 1.000000000000000000, 0.000000000000000000, -0.000000000000000000 ) ) ;
#56870=( BOUNDED_CURVE ( )  B_SPLINE_CURVE ( 1, ( #51776, #26115 ),
 .UNSPECIFIED., .F., .F. ) 
 B_SPLINE_CURVE_WITH_KNOTS ( ( 2, 2 ),
 ( 1.748223473168675632E-18, 0.001849999999999997913 ),
 .UNSPECIFIED. ) 
 CURVE ( )  GEOMETRIC_REPRESENTATION_ITEM ( )  RATIONAL_B_SPLINE_CURVE ( ( 0.9911642120908021880, 0.9911642120908021880 ) ) 
 REPRESENTATION_ITEM ( '' )  );
#56871=CARTESIAN_POINT ( 'NONE',  ( -0.4724409448818898682, -8.678599364036362592E-17, -0.3543307086614173040 ) ) ;
#56872=CARTESIAN_POINT ( 'NONE',  ( -9.787531504996567848E-17, 0.3996062992125986035, 0.1574803149606298913 ) ) ;
#56875=VECTOR ( 'NONE', #47760, 39.37007874015748143 ) ;
#56876=CARTESIAN_POINT ( 'NONE',  ( 0.3917322834645670104, 2.398668435337828261E-17, -1.370078740157480324 ) ) ;
#56878=CARTESIAN_POINT ( 'NONE',  ( 0.05073257145186254452, 0.3893108287682404689, -2.755905511811024944 ) ) ;
#56885=CARTESIAN_POINT ( 'NONE',  ( -0.3392501089628019439, 0.1958661417322832554, -0.8936814716197357678 ) ) ;
#56892=CARTESIAN_POINT ( 'NONE',  ( 0.3917322834645670659, -0.1049643490035303273, -1.840570496884201379 ) ) ;
#56894=EDGE_LOOP ( 'NONE', ( #21504, #24284, #35247 ) ) ;
#56899=CARTESIAN_POINT ( 'NONE',  ( 0.1958661417322836440, -0.3392501089628017219, -1.593832020997375531 ) ) ;
#56904=CARTESIAN_POINT ( 'NONE',  ( -0.0003067303408297487139, 0.3990339831394625336, 7.618016766297074103E-18 ) ) ;
#56908=CARTESIAN_POINT ( 'NONE',  ( -0.3917322834645669549, -0.1049643490035306603, -2.715223097112861250 ) ) ;
#56915=CARTESIAN_POINT ( 'NONE',  ( -9.594673741351313045E-17, 0.3917322834645670104, -1.029527559055118280 ) ) ;
#56919=CARTESIAN_POINT ( 'NONE',  ( -0.1998031496062991630, -0.3460692066303959202, -2.662073490813648746 ) ) ;
#56929=CARTESIAN_POINT ( 'NONE',  ( -0.3996062992125984925, -0.1070741851644056858, -0.2801837270341207553 ) ) ;
#56931=CARTESIAN_POINT ( 'NONE',  ( -0.3392501089628017219, -0.1958661417322836718, -0.3595800524934382736 ) ) ;
#56945=CARTESIAN_POINT ( 'NONE',  ( 0.1049643490035304799, -0.3917322834645670104, -0.8694418879603171835 ) ) ;
#56949=CARTESIAN_POINT ( 'NONE',  ( -0.1265901696524986964, -0.4724409448818899238, -2.511154855643044748 ) ) ;
#56967=CARTESIAN_POINT ( 'NONE',  ( -9.787531504996567848E-17, 0.3996062992125986035, -0.4724409448818898127 ) ) ;
#56968=CARTESIAN_POINT ( 'NONE',  ( -0.1070741851644056997, 0.3996062992125984925, -2.603018372703412631 ) ) ;
#56973=CARTESIAN_POINT ( 'NONE',  ( -0.1998031496062994683, 0.3460692066303958092, -2.375328083989501238 ) ) ;
#56974=CARTESIAN_POINT ( 'NONE',  ( -0.3420746716998661618, 0.1974969037888702206, -1.601049868766404094 ) ) ;
#56975=CARTESIAN_POINT ( 'NONE',  ( -0.3996062992125986035, -0.1070741851644056997, -2.880577427821522374 ) ) ;
#56978=CARTESIAN_POINT ( 'NONE',  ( -0.1049643490035307020, 0.3917322834645669549, -0.6286089238845143923 ) ) ;
#56981=CARTESIAN_POINT ( 'NONE',  ( 0.1058382717557500852, -0.3949938075777408852, -2.681758530183727451 ) ) ;
#56985=CARTESIAN_POINT ( 'NONE',  ( -0.4724409448818898682, -8.678599364036362592E-17, -2.874015748031495843 ) ) ;
#56986=CARTESIAN_POINT ( 'NONE',  ( -0.2925321140481930704, -0.2925321140481933480, -2.106299212598425452 ) ) ;
#56993=CARTESIAN_POINT ( 'NONE',  ( 0.1958661417322836440, -0.3392501089628017219, -0.1765091863517061210 ) ) ;
#57000=CARTESIAN_POINT ( 'NONE',  ( -0.3917322834645670104, -7.196005306013484475E-17, -0.4389763779527560139 ) ) ;
#57001=CARTESIAN_POINT ( 'NONE',  ( 0.1049643490035303689, 0.3917322834645670104, -1.402887139107611647 ) ) ;
#57002=( BOUNDED_CURVE ( )  B_SPLINE_CURVE ( 2, ( #44348, #70039, #57402, #76776, #83093, #52752, #47270, #19953, #78876, #71714, #39298, #14069, #1846 ),
 .UNSPECIFIED., .F., .F. ) 
 B_SPLINE_CURVE_WITH_KNOTS ( ( 3, 2, 2, 2, 2, 2, 3 ),
 ( 0.08750000000000000833, 0.09166666666666667407, 0.09583333333333335369, 0.1000000000000000056, 0.1041666666666666713, 0.1083333333333333370, 0.1125000000000000028 ),
 .UNSPECIFIED. ) 
 CURVE ( )  GEOMETRIC_REPRESENTATION_ITEM ( )  RATIONAL_B_SPLINE_CURVE ( ( 0.9999999999999998890, 0.9659258262890684232, 1.000000000000000000, 0.9659258262890683122, 1.000000000000000000, 0.9659258262890683122, 1.000000000000000000, 0.9659258262890683122, 1.000000000000000000, 0.9659258262890683122, 1.000000000000000000, 0.9659258262890683122, 1.000000000000000000 ) ) 
 REPRESENTATION_ITEM ( '' )  );
#57003=CARTESIAN_POINT ( 'NONE',  ( -0.1049643490035302024, -0.3917322834645671215, -2.583989501312335513 ) ) ;
#57005=CARTESIAN_POINT ( 'NONE',  ( -0.3460692066303960868, 0.1998031496062990242, 0.1312335958005249048 ) ) ;
#57009=CARTESIAN_POINT ( 'NONE',  ( -9.787531504996567848E-17, 0.3996062992125986035, -1.574803149606299302 ) ) ;
#57011=CARTESIAN_POINT ( 'NONE',  ( 0.4091458600556403535, 0.2362204724409449896, -2.412729658792650778 ) ) ;
#57014=CARTESIAN_POINT ( 'NONE',  ( -0.3917322834645671215, 0.1049643490035301469, -0.4324146981627298159 ) ) ;
#57025=CARTESIAN_POINT ( 'NONE',  ( -0.4724409448818899238, 0.1265901696524986686, -2.237532808398950301 ) ) ;
#57035=CARTESIAN_POINT ( 'NONE',  ( -0.3917322834645670659, 0.1049643490035301607, -0.2703218915672423450 ) ) ;
#57037=CARTESIAN_POINT ( 'NONE',  ( -0.3917322834645670104, -7.196005306013484475E-17, -0.7539370078740157410 ) ) ;
#57043=CARTESIAN_POINT ( 'NONE',  ( 0.3917322834645670104, -0.1049643490035303411, -2.938320209973753538 ) ) ;
#57046=CARTESIAN_POINT ( 'NONE',  ( -0.4091458600556402980, -0.2362204724409451284, -1.389107611548556553 ) ) ;
#57059=CARTESIAN_POINT ( 'NONE',  ( 0.1070741851644054776, -0.3996062992125984925, -2.524278215223096478 ) ) ;
#57062=CARTESIAN_POINT ( 'NONE',  ( 0.2925321140481932369, -0.2925321140481931814, -1.277559055118110187 ) ) ;
#57066=CARTESIAN_POINT ( 'NONE',  ( 0.4724409448818899238, -0.1265901696524985298, -0.1115485564304462274 ) ) ;
#57068=CARTESIAN_POINT ( 'NONE',  ( -0.1998031496062991630, -0.3460692066303959202, -0.7723097112860892732 ) ) ;
#57069=CARTESIAN_POINT ( 'NONE',  ( 0.3460692066303959757, -0.1998031496062991907, -1.049868766404199460 ) ) ;
#57070=CARTESIAN_POINT ( 'NONE',  ( 0.3949938075777411073, -0.1058382717557499464, -0.4265091863517062043 ) ) ;
#57076=CARTESIAN_POINT ( 'NONE',  ( -0.2891555358219909388, -0.2891555358219912164, -1.238188976377952999 ) ) ;
#57081=CARTESIAN_POINT ( 'NONE',  ( -0.3458507752293906723, -0.3458507752293910609, -1.476377952755905554 ) ) ;
#57095=CARTESIAN_POINT ( 'NONE',  ( -0.3917322834645669549, -0.1049643490035306603, -1.455380577427821676 ) ) ;
#57097=ORIENTED_EDGE ( 'NONE', *, *, #17054, .T. ) ;
#57098=CARTESIAN_POINT ( 'NONE',  ( 0.1058382717557499880, 0.3949938075777411073, -1.253280839895013488 ) ) ;
#57103=CARTESIAN_POINT ( 'NONE',  ( 0.3996062992125986590, -0.1070741851644053111, -0.2690288713910760632 ) ) ;
#57111=CARTESIAN_POINT ( 'NONE',  ( -9.594673741351313045E-17, 0.3917322834645670104, 0.07283464566929125084 ) ) ;
#57118=ORIENTED_EDGE ( 'NONE', *, *, #59835, .T. ) ;
#57119=CARTESIAN_POINT ( 'NONE',  ( -0.3996062992125985480, -7.340648628747423112E-17, -1.375984251968503713 ) ) ;
#57124=CARTESIAN_POINT ( 'NONE',  ( -0.4091458600556402980, -0.2362204724409451284, -0.8398950131233595684 ) ) ;
#57126=CARTESIAN_POINT ( 'NONE',  ( 0.3392501089628018884, -0.1958661417322834220, 0.06036745406824151755 ) ) ;
#57128=CARTESIAN_POINT ( 'NONE',  ( 0.3392501089628018329, 0.1958661417322835607, -1.948162729658792891 ) ) ;
#57132=CARTESIAN_POINT ( 'NONE',  ( -0.4724409448818895907, -0.1265901696524993070, -2.642388451443570041 ) ) ;
#57135=CARTESIAN_POINT ( 'NONE',  ( 0.3949938075777409408, -0.1058382717557499186, -2.393044619422572072 ) ) ;
#57156=CARTESIAN_POINT ( 'NONE',  ( 4.893765752498283308E-17, -0.3996062992125985480, -0.7854330708661416693 ) ) ;
#57157=CARTESIAN_POINT ( 'NONE',  ( 0.3392501089628018329, 0.1958661417322835607, -2.420603674540682260 ) ) ;
#57167=CARTESIAN_POINT ( 'NONE',  ( -0.1265901696524986964, -0.4724409448818899238, -0.7020997375328084100 ) ) ;
#57168=CARTESIAN_POINT ( 'NONE',  ( -0.2867679344610365444, -0.2867679344610367664, -2.260518003445880719 ) ) ;
#57174=CARTESIAN_POINT ( 'NONE',  ( 0.2867679344610365999, -0.2867679344610365444, -1.915354330708661124 ) ) ;
#57181=CARTESIAN_POINT ( 'NONE',  ( 0.2925321140481932369, -0.2925321140481932369, -1.515748031496062742 ) ) ;
#57183=CARTESIAN_POINT ( 'NONE',  ( -0.3917322834645670659, -7.196005306013484475E-17, 0.1213717603336463974 ) ) ;
#57195=CARTESIAN_POINT ( 'NONE',  ( -0.1049643490035307020, 0.3917322834645669549, -0.3136482939632545541 ) ) ;
#57197=ORIENTED_EDGE ( 'NONE', *, *, #67875, .T. ) ;
#57198=CARTESIAN_POINT ( 'NONE',  ( 0.1974969037888706369, -0.3420746716998659953, -0.2493438320209974690 ) ) ;
#57202=CARTESIAN_POINT ( 'NONE',  ( -0.4724409448818898682, -8.678599364036362592E-17, -2.716535433070865757 ) ) ;
#57206=CARTESIAN_POINT ( 'NONE',  ( 0.1049643490035303967, 0.3917322834645670659, -1.564979945703099062 ) ) ;
#57208=CARTESIAN_POINT ( 'NONE',  ( -0.1049643490035307020, 0.3917322834645669549, -2.453412073490813139 ) ) ;
#57212=CARTESIAN_POINT ( 'NONE',  ( 0.3460692066303959757, -0.1998031496062991907, -0.7349081364829396223 ) ) ;
#57214=CARTESIAN_POINT ( 'NONE',  ( -0.1998031496062994405, 0.3460692066303957537, -0.4048556430446194621 ) ) ;
#57215=CARTESIAN_POINT ( 'NONE',  ( -0.1070741851644051862, -0.3996062992125986590, -0.1489501312335958227 ) ) ;
#57217=CARTESIAN_POINT ( 'NONE',  ( -0.3460692066303960868, 0.1998031496062990242, -2.545931758530183497 ) ) ;
#57218=CARTESIAN_POINT ( 'NONE',  ( -0.2867679344610365999, 0.2867679344610364889, -1.836614173228346747 ) ) ;
#57224=CARTESIAN_POINT ( 'NONE',  ( -1.157146581871515012E-16, 0.4724409448818898682, -1.336614173228346303 ) ) ;
#57227=CARTESIAN_POINT ( 'NONE',  ( -0.1058382717557503072, 0.3949938075777408852, -0.8707349081364829102 ) ) ;
#57236=CARTESIAN_POINT ( 'NONE',  ( 4.893765752498283308E-17, -0.3996062992125985480, -2.202755905511811108 ) ) ;
#57253=CARTESIAN_POINT ( 'NONE',  ( -0.2867679344610364334, -0.2867679344610367109, -0.9311023622047245318 ) ) ;
#57276=CARTESIAN_POINT ( 'NONE',  ( 4.797336870675656522E-17, -0.3917322834645670104, -2.118110236220472675 ) ) ;
#57280=CARTESIAN_POINT ( 'NONE',  ( -0.4724409448818895907, -0.1265901696524993070, -0.2034120734908136108 ) ) ;
#57281=CARTESIAN_POINT ( 'NONE',  ( -0.3420746716998659953, -0.1974969037888706647, -2.729658792650918819 ) ) ;
#57282=ORIENTED_EDGE ( 'NONE', *, *, #64580, .F. ) ;
#57284=CARTESIAN_POINT ( 'NONE',  ( 0.1958661417322834775, 0.3392501089628018884, -1.396325459317585338 ) ) ;
#57292=CARTESIAN_POINT ( 'NONE',  ( 0.3917322834645669549, 2.398668435337827645E-17, -0.6705843587588433685 ) ) ;
#57299=CARTESIAN_POINT ( 'NONE',  ( 0.1958661417322836718, -0.3392501089628017219, -2.135846087435382401 ) ) ;
#57306=CARTESIAN_POINT ( 'NONE',  ( 0.2867679344610365999, -0.2867679344610365444, -1.285433070866141669 ) ) ;
#57316=CARTESIAN_POINT ( 'NONE',  ( -0.2867679344610364334, -0.2867679344610367109, -2.885826771653543066 ) ) ;
#57325=FACE_OUTER_BOUND ( 'NONE', #34687, .T. ) ;
#57326=CARTESIAN_POINT ( 'NONE',  ( 0.1049643490035303689, 0.3917322834645670104, -1.180446194225722056 ) ) ;
#57327=CARTESIAN_POINT ( 'NONE',  ( 0.4724409448818896462, 0.1265901696524990294, -0.2014435695538057958 ) ) ;
#57330=CARTESIAN_POINT ( 'NONE',  ( 4.893765752498283308E-17, -0.3996062992125985480, -2.675196850393700920 ) ) ;
#57340=CARTESIAN_POINT ( 'NONE',  ( -0.1998031496062991630, -0.3460692066303959202, -0.2998687664041995160 ) ) ;
#57342=CARTESIAN_POINT ( 'NONE',  ( -0.1958661417322834220, -0.3392501089628018884, -0.2152230971128608339 ) ) ;
#57355=CARTESIAN_POINT ( 'NONE',  ( -0.1049643490035307158, 0.3917322834645670104, -0.7907017304800020296 ) ) ;
#57360=CARTESIAN_POINT ( 'NONE',  ( -0.1265901696524993347, 0.4724409448818895907, -2.445538057742782101 ) ) ;
#57381=CARTESIAN_POINT ( 'NONE',  ( -0.1070741851644051862, -0.3996062992125986590, -0.2296587926509186528 ) ) ;
#57382=CARTESIAN_POINT ( 'NONE',  ( 4.893765752498283308E-17, -0.3996062992125985480, -2.832677165354331006 ) ) ;
#57390=CARTESIAN_POINT ( 'NONE',  ( 0.1070741851644054915, -0.3996062992125986035, -2.290026246719159442 ) ) ;
#57391=CARTESIAN_POINT ( 'NONE',  ( -0.1974969037888706647, 0.3420746716998658843, -1.430446194225722056 ) ) ;
#57392=CARTESIAN_POINT ( 'NONE',  ( -0.1070741851644051862, -0.3996062992125987146, -2.749343832020996636 ) ) ;
#57394=CARTESIAN_POINT ( 'NONE',  ( 0.1049643490035303689, 0.3917322834645670104, -1.087926509186351476 ) ) ;
#57398=CARTESIAN_POINT ( 'NONE',  ( 0.3420746716998660508, -0.1974969037888704149, -2.701443569553805713 ) ) ;
#57402=CARTESIAN_POINT ( 'NONE',  ( 0.4091458600556403535, 0.2362204724409449896, -0.05052493438320210251 ) ) ;
#57403=CARTESIAN_POINT ( 'NONE',  ( 0.1070741851644054915, -0.3996062992125986035, -2.290026246719159442 ) ) ;
#57409=CARTESIAN_POINT ( 'NONE',  ( -0.3392501089628019995, 0.1958661417322832277, 0.04658792650918625738 ) ) ;
#57417=CARTESIAN_POINT ( 'NONE',  ( 0.1958661417322834775, 0.3392501089628018884, -0.7014435695538058235 ) ) ;
#57418=CARTESIAN_POINT ( 'NONE',  ( -0.3392501089628019995, 0.1958661417322832277, -1.593175853018372612 ) ) ;
#57419=CARTESIAN_POINT ( 'NONE',  ( 0.3917322834645669549, 0.1049643490035304660, -2.636482939632545985 ) ) ;
#57421=CARTESIAN_POINT ( 'NONE',  ( -0.3460692066303958092, -0.1998031496062994683, 0.1049868766404199322 ) ) ;
#57425=CARTESIAN_POINT ( 'NONE',  ( -0.3996062992125987146, 0.1070741851644051862, -1.607611548556430403 ) ) ;
#57427=CARTESIAN_POINT ( 'NONE',  ( 0.2362204724409449064, 0.4091458600556404646, -2.425853018372703396 ) ) ;
#57430=CARTESIAN_POINT ( 'NONE',  ( -0.1049643490035302024, -0.3917322834645671215, -0.9442257217847768169 ) ) ;
#57439=CARTESIAN_POINT ( 'NONE',  ( -0.1265901696524986964, -0.4724409448818899238, -1.961942257217847763 ) ) ;
#57445=VERTEX_POINT ( 'NONE', #1870 ) ;
#57450=CARTESIAN_POINT ( 'NONE',  ( 0.1049643490035304522, -0.3917322834645668994, -0.6377759598087122672 ) ) ;
#57452=CARTESIAN_POINT ( 'NONE',  ( -0.1958661417322836718, 0.3392501089628017219, -0.7276902887139108378 ) ) ;
#57457=CARTESIAN_POINT ( 'NONE',  ( -0.1049643490035302024, -0.3917322834645671215, -2.898950131233595684 ) ) ;
#57460=CARTESIAN_POINT ( 'NONE',  ( 5.785732909357575061E-17, -0.4724409448818898682, -1.100393700787401619 ) ) ;
#57472=CARTESIAN_POINT ( 'NONE',  ( -0.3996062992125985480, -7.340648628747423112E-17, -2.320866141732283783 ) ) ;
#57476=CARTESIAN_POINT ( 'NONE',  ( -0.1998031496062994405, 0.3460692066303957537, -1.349737532808399143 ) ) ;
#57482=CARTESIAN_POINT ( 'NONE',  ( -0.3996062992125984925, -0.1070741851644056719, -0.5951443569553805935 ) ) ;
#57484=CARTESIAN_POINT ( 'NONE',  ( 0.3996062992125986035, 0.1070741851644054776, -0.7545931758530182165 ) ) ;
#57485=CARTESIAN_POINT ( 'NONE',  ( -0.1974969037888706647, 0.3420746716998658843, -0.1706036745406825095 ) ) ;
#57491=CARTESIAN_POINT ( 'NONE',  ( -0.3949938075777411073, 0.1058382717557497660, -1.369422572178477848 ) ) ;
#57497=CARTESIAN_POINT ( 'NONE',  ( 0.4724409448818897572, -0.1265901696524988906, -1.686351706036745446 ) ) ;
#57499=CARTESIAN_POINT ( 'NONE',  ( 0.4724409448818898682, 0.000000000000000000, -2.755905511811024056 ) ) ;
#57501=ORIENTED_EDGE ( 'NONE', *, *, #1376, .T. ) ;
#57506=CARTESIAN_POINT ( 'NONE',  ( -0.3917322834645668994, -0.1049643490035306742, -2.173209030674854159 ) ) ;
#57513=CARTESIAN_POINT ( 'NONE',  ( -0.1049643490035307020, 0.3917322834645669549, -1.573490813648293907 ) ) ;
#57516=CARTESIAN_POINT ( 'NONE',  ( 0.2891555358219910499, 0.2891555358219910499, -2.027559055118110631 ) ) ;
#57521=CARTESIAN_POINT ( 'NONE',  ( -0.1998031496062991907, -0.3460692066303959757, -0.06561679790026248016 ) ) ;
#57529=CARTESIAN_POINT ( 'NONE',  ( -0.3917322834645670104, -7.196005306013484475E-17, -0.2814960629921260393 ) ) ;
#57535=EDGE_LOOP ( 'NONE', ( #18629, #65867, #57501, #6823 ) ) ;
#57536=CARTESIAN_POINT ( 'NONE',  ( -0.3996062992125985480, -7.340648628747423112E-17, -2.163385826771653697 ) ) ;
#57541=CARTESIAN_POINT ( 'NONE',  ( 0.2362204724409451007, -0.4091458600556402980, -0.7217847769028871152 ) ) ;
#57543=CARTESIAN_POINT ( 'NONE',  ( -0.3392501089628019995, 0.1958661417322832277, 0.1391076115485564701 ) ) ;
#57544=CARTESIAN_POINT ( 'NONE',  ( -0.3917322834645669549, -0.1049643490035306603, -2.020341207349081181 ) ) ;
#57548=CARTESIAN_POINT ( 'NONE',  ( -0.1265901696524986964, -0.4724409448818899238, -2.826115485564304475 ) ) ;
#57552=CARTESIAN_POINT ( 'NONE',  ( 0.2891555358219910499, 0.2891555358219910499, -2.104330708661417138 ) ) ;
#57559=CARTESIAN_POINT ( 'NONE',  ( -9.594673741351313045E-17, 0.3917322834645670104, -1.566929133858267820 ) ) ;
#57562=FACE_OUTER_BOUND ( 'NONE', #28954, .T. ) ;
#57574=CARTESIAN_POINT ( 'NONE',  ( -0.1070741851644056997, 0.3996062992125984925, -1.343175853018372834 ) ) ;
#57576=CARTESIAN_POINT ( 'NONE',  ( -0.1958661417322834220, -0.3392501089628018884, -2.354986876640420057 ) ) ;
#57587=EDGE_CURVE ( 'NONE', #69925, #81066, #39691, .T. ) ;
#57588=CARTESIAN_POINT ( 'NONE',  ( 4.797336870675656522E-17, -0.3917322834645670659, -1.965242412894699919 ) ) ;
#57594=CARTESIAN_POINT ( 'NONE',  ( -0.3392501089628019995, 0.1958661417322832277, -2.000656167979002920 ) ) ;
#57595=CARTESIAN_POINT ( 'NONE',  ( 0.05870088567680617486, 0.3874523867751286099, -1.220472440944882164 ) ) ;
#57598=DIRECTION ( 'NONE',  ( 0.000000000000000000, 0.000000000000000000, 1.000000000000000000 ) ) ;
#57601=CARTESIAN_POINT ( 'NONE',  ( 0.2925321140481932369, 0.2925321140481932369, -1.240157480314960647 ) ) ;
#57603=CARTESIAN_POINT ( 'NONE',  ( -0.3392501089628019995, 0.1958661417322832277, -2.853018372703412187 ) ) ;
#57617=CARTESIAN_POINT ( 'NONE',  ( 0.3917322834645669549, 0.1049643490035304660, -0.2742782152230970327 ) ) ;
#57620=CARTESIAN_POINT ( 'NONE',  ( 0.3949938075777409963, 2.418639510665530435E-17, -0.4330708661417323468 ) ) ;
#57627=CARTESIAN_POINT ( 'NONE',  ( -0.3392501089628017219, -0.1958661417322836995, -1.624035063813334956 ) ) ;
#57629=CARTESIAN_POINT ( 'NONE',  ( -0.2867679344610364334, -0.2867679344610367109, -2.663385826771653253 ) ) ;
#57633=CARTESIAN_POINT ( 'NONE',  ( 0.3460692066303959757, -0.1998031496062991907, -1.049868766404199460 ) ) ;
#57635=CARTESIAN_POINT ( 'NONE',  ( -0.1070741851644056997, 0.3996062992125984925, -0.8707349081364830212 ) ) ;
#57636=CARTESIAN_POINT ( 'NONE',  ( -9.787531504996566615E-17, 0.3996062992125985480, -0.2342519685039370358 ) ) ;
#57638=CARTESIAN_POINT ( 'NONE',  ( 4.893765752498283924E-17, -0.3996062992125986035, -2.913385826771653697 ) ) ;
#57639=CARTESIAN_POINT ( 'NONE',  ( -0.1049643490035302024, -0.3917322834645671215, -1.889107611548556109 ) ) ;
#57645=CARTESIAN_POINT ( 'NONE',  ( 0.3458507752293908943, -0.3458507752293908943, -1.592519685039370358 ) ) ;
#57648=CARTESIAN_POINT ( 'NONE',  ( -0.1974969037888704149, -0.3420746716998661063, -1.087270341207349000 ) ) ;
#57658=CARTESIAN_POINT ( 'NONE',  ( 0.2925321140481932369, -0.2925321140481931814, -2.222440944881889813 ) ) ;
#57660=CARTESIAN_POINT ( 'NONE',  ( -0.3917322834645669549, -7.196005306013483243E-17, -1.851686720963567456 ) ) ;
#57672=CARTESIAN_POINT ( 'NONE',  ( 0.1998031496062994128, -0.3460692066303957537, -0.01115485564304462100 ) ) ;
#57674=CARTESIAN_POINT ( 'NONE',  ( 0.2867679344610365999, -0.2867679344610365444, -0.9704724409448820532 ) ) ;
#57694=CARTESIAN_POINT ( 'NONE',  ( 4.797336870675656522E-17, -0.3917322834645670104, -2.590551181102362044 ) ) ;
#57697=CARTESIAN_POINT ( 'NONE',  ( -0.3458507752293906723, -0.3458507752293910609, -0.3740157480314960092 ) ) ;
#57698=CARTESIAN_POINT ( 'NONE',  ( -0.3996062992125986035, -7.340648628747425578E-17, -0.03937007874015750059 ) ) ;
#57701=CARTESIAN_POINT ( 'NONE',  ( -0.1049643490035307020, 0.3917322834645669549, -1.730971128608923992 ) ) ;
#57703=CARTESIAN_POINT ( 'NONE',  ( -0.4724409448818895907, -0.1265901696524993070, -2.880577427821522374 ) ) ;
#57711=CARTESIAN_POINT ( 'NONE',  ( 0.1049643490035303689, 0.3917322834645668994, -0.8608730726696044444 ) ) ;
#57718=CARTESIAN_POINT ( 'NONE',  ( 0.3917322834645670659, 2.398668435337828261E-17, -1.847132176674227688 ) ) ;
#57726=CARTESIAN_POINT ( 'NONE',  ( -0.3917322834645669549, -0.1049643490035306603, -1.390419947506561504 ) ) ;
#57741=CARTESIAN_POINT ( 'NONE',  ( 0.3996062992125986035, 2.446882876249141962E-17, -1.220472440944881942 ) ) ;
#57742=CARTESIAN_POINT ( 'NONE',  ( -0.1049643490035307020, 0.3917322834645669549, -1.193569553805774452 ) ) ;
#57743=CARTESIAN_POINT ( 'NONE',  ( 0.1265901696524989462, 0.4724409448818897572, -0.3851706036745406458 ) ) ;
#57746=CARTESIAN_POINT ( 'NONE',  ( -0.2891555358219911054, 0.2891555358219909388, 0.2185039370078739884 ) ) ;
#57751=CARTESIAN_POINT ( 'NONE',  ( 0.3949938075777409963, 2.418639510665530743E-17, 0.1200787401574803376 ) ) ;
#57758=CARTESIAN_POINT ( 'NONE',  ( -0.3460692066303957537, -0.1998031496062994405, -0.9166666666666666297 ) ) ;
#57760=CARTESIAN_POINT ( 'NONE',  ( 0.1958661417322834775, 0.3392501089628018884, -0.2939632545931757934 ) ) ;
#57776=CARTESIAN_POINT ( 'NONE',  ( 0.2362204724409449064, 0.4091458600556404646, -2.583333333333333481 ) ) ;
#57792=CARTESIAN_POINT ( 'NONE',  ( -0.3996062992125986035, -7.340648628747425578E-17, -0.1968503937007874405 ) ) ;
#57793=CARTESIAN_POINT ( 'NONE',  ( -0.2925321140481930149, -0.2925321140481933480, -2.498031496062992574 ) ) ;
#57798=CARTESIAN_POINT ( 'NONE',  ( -0.3996062992125987146, 0.1070741851644051862, -2.080052493438320216 ) ) ;
#57799=CARTESIAN_POINT ( 'NONE',  ( 0.1058382717557499880, 0.3949938075777411073, -2.040682414698163250 ) ) ;
#57800=CARTESIAN_POINT ( 'NONE',  ( -0.2867679344610365999, 0.2867679344610364889, -0.4842519685039369248 ) ) ;
#57802=CARTESIAN_POINT ( 'NONE',  ( -0.2867679344610364334, -0.2867679344610367109, -0.9960629921259841479 ) ) ;
#57806=CARTESIAN_POINT ( 'NONE',  ( -0.1974969037888704149, -0.3420746716998661063, -2.662073490813648746 ) ) ;
#57810=CARTESIAN_POINT ( 'NONE',  ( 0.1265901696524990294, -0.4724409448818896462, -2.762467191601049255 ) ) ;
#57811=CARTESIAN_POINT ( 'NONE',  ( 0.3460692066303959202, 0.1998031496062993295, -2.178477690288713742 ) ) ;
#57812=CARTESIAN_POINT ( 'NONE',  ( 0.1958661417322834775, 0.3392501089628018884, -0.6135363761492932388 ) ) ;
#57818=CARTESIAN_POINT ( 'NONE',  ( 4.797336870675656522E-17, -0.3917322834645670104, -0.3208661417322835607 ) ) ;
#57826=CARTESIAN_POINT ( 'NONE',  ( -0.3917322834645671215, 0.1049643490035301469, -0.7473753280839893209 ) ) ;
#57827=CARTESIAN_POINT ( 'NONE',  ( -0.3917322834645670104, -7.196005306013484475E-17, -1.448818897637795367 ) ) ;
#57828=CARTESIAN_POINT ( 'NONE',  ( 4.797336870675656522E-17, -0.3917322834645670104, -2.590551181102362044 ) ) ;
#57829=ORIENTED_EDGE ( 'NONE', *, *, #71814, .F. ) ;
#57830=CARTESIAN_POINT ( 'NONE',  ( 0.1070741851644053527, 0.3996062992125986590, -0.1509186351706036655 ) ) ;
#57834=CARTESIAN_POINT ( 'NONE',  ( 0.1070741851644054915, -0.3996062992125986035, -1.345144356955380704 ) ) ;
#57839=CARTESIAN_POINT ( 'NONE',  ( -0.1049643490035307020, 0.3917322834645669549, -1.036089238845144589 ) ) ;
#57846=VERTEX_POINT ( 'NONE', #62010 ) ;
#57849=CARTESIAN_POINT ( 'NONE',  ( -0.3458507752293909498, 0.3458507752293907833, -2.066929133858267154 ) ) ;
#57851=CARTESIAN_POINT ( 'NONE',  ( 0.2017716535433070613, 0.2017716535433070613, -0.3937007874015748254 ) ) ;
#57856=CARTESIAN_POINT ( 'NONE',  ( -0.4724409448818896462, -0.1265901696524993070, -2.484908136482939955 ) ) ;
#57861=CARTESIAN_POINT ( 'NONE',  ( 0.2867679344610365999, 0.2867679344610365999, -0.6902693981289222958 ) ) ;
#57863=CARTESIAN_POINT ( 'NONE',  ( -0.1049643490035301885, -0.3917322834645671215, -0.9442257217847769279 ) ) ;
#57870=CARTESIAN_POINT ( 'NONE',  ( -0.3917322834645670104, -7.196005306013484475E-17, -2.866141732283464361 ) ) ;
#57873=CARTESIAN_POINT ( 'NONE',  ( 0.1265901696524990294, -0.4724409448818896462, -1.264435695538057569 ) ) ;
#57886=CARTESIAN_POINT ( 'NONE',  ( -0.1070741851644056997, 0.3996062992125984925, -2.445538057742782101 ) ) ;
#57890=CARTESIAN_POINT ( 'NONE',  ( -0.3996062992125986590, 0.1070741851644051723, -1.211942257217847541 ) ) ;
#57896=CARTESIAN_POINT ( 'NONE',  ( -0.3996062992125986035, 0.1070741851644051584, -0.7395013123359578389 ) ) ;
#57897=CARTESIAN_POINT ( 'NONE',  ( -0.2925321140481930704, -0.2925321140481933480, -0.8464566929133857665 ) ) ;
#57898=ADVANCED_FACE ( 'NONE', ( #80977 ), #17108, .T. ) ;
#57899=CARTESIAN_POINT ( 'NONE',  ( -9.674558042662121740E-17, 0.3949938075777409963, -0.1574803149606300023 ) ) ;
#57906=CARTESIAN_POINT ( 'NONE',  ( -0.3949938075777408852, -0.1058382717557502933, -1.382545931758530688 ) ) ;
#57912=CARTESIAN_POINT ( 'NONE',  ( -0.4724409448818895907, -0.1265901696524993070, -1.620734908136482799 ) ) ;
#57913=LINE ( 'NONE', #57499, #38470 ) ;
#57920=CARTESIAN_POINT ( 'NONE',  ( 0.3917322834645668994, 0.1049643490035304522, -1.779508243273278945 ) ) ;
#57921=CARTESIAN_POINT ( 'NONE',  ( -0.1998031496062991630, -0.3460692066303959202, -2.819553805774277944 ) ) ;
#57926=CARTESIAN_POINT ( 'NONE',  ( 0.1049643490035303689, 0.3917322834645670104, -1.560367454068241511 ) ) ;
#57929=CARTESIAN_POINT ( 'NONE',  ( 0.2891555358219910499, -0.2891555358219909944, -1.988188976377952777 ) ) ;
#57934=CARTESIAN_POINT ( 'NONE',  ( 0.1070741851644053527, 0.3996062992125986590, -0.3083989501312335846 ) ) ;
#57940=CARTESIAN_POINT ( 'NONE',  ( 0.3392501089628018329, 0.1958661417322835607, -0.5308398950131234528 ) ) ;
#57947=CARTESIAN_POINT ( 'NONE',  ( 0.1070741851644054776, -0.3996062992125984925, -2.051837270341206665 ) ) ;
#57952=CARTESIAN_POINT ( 'NONE',  ( -0.2362204724409451284, 0.4091458600556402425, -0.6430446194225721834 ) ) ;
#57954=CARTESIAN_POINT ( 'NONE',  ( 0.1049643490035304938, -0.3917322834645669549, -0.3923884514435695414 ) ) ;
#57955=CARTESIAN_POINT ( 'NONE',  ( 0.000000000000000000, 0.000000000000000000, 0.000000000000000000 ) ) ;
#57959=CARTESIAN_POINT ( 'NONE',  ( -0.2362204724409447953, -0.4091458600556404646, -2.819553805774277944 ) ) ;
#57964=CARTESIAN_POINT ( 'NONE',  ( 0.3420746716998660508, 0.1974969037888705814, -2.727690288713910949 ) ) ;
#57974=CARTESIAN_POINT ( 'NONE',  ( -0.2867679344610364334, -0.2867679344610367109, -1.468503937007874294 ) ) ;
#57989=CARTESIAN_POINT ( 'NONE',  ( -0.3996062992125985480, -7.340648628747423112E-17, -1.061023622047243986 ) ) ;
#57991=CARTESIAN_POINT ( 'NONE',  ( -0.3392501089628019995, 0.1958661417322832277, -2.473097112860892288 ) ) ;
#58001=CARTESIAN_POINT ( 'NONE',  ( -0.3460692066303960868, 0.1998031496062990242, 0.1312335958005249048 ) ) ;
#58002=CARTESIAN_POINT ( 'NONE',  ( 0.3917322834645670659, -0.1049643490035303273, -1.998050811844831243 ) ) ;
#58008=CARTESIAN_POINT ( 'NONE',  ( -0.3392501089628017219, -0.1958661417322836718, -2.184383202099737797 ) ) ;
#58015=CARTESIAN_POINT ( 'NONE',  ( 0.2925321140481932369, 0.2925321140481932369, -1.397637795275590067 ) ) ;
#58017=CARTESIAN_POINT ( 'NONE',  ( -0.3917322834645671215, 0.1049643490035301469, -2.859580052493438274 ) ) ;
#58020=PRODUCT_DEFINITION_SHAPE ( 'NONE', 'NONE',  #38279 ) ;
#58032=CARTESIAN_POINT ( 'NONE',  ( 0.1958661417322836440, -0.3392501089628017219, -0.2414698162729658204 ) ) ;
#58034=EDGE_LOOP ( 'NONE', ( #17916, #51151, #74936, #57197 ) ) ;
#58035=CARTESIAN_POINT ( 'NONE',  ( 4.837279021331060870E-17, -0.3949938075777409963, -0.5511811023622048555 ) ) ;
#58042=CARTESIAN_POINT ( 'NONE',  ( 0.3917322834645670659, -0.1049643490035303273, -1.525609866962941430 ) ) ;
#58048=CARTESIAN_POINT ( 'NONE',  ( 4.893765752498283924E-17, -0.3996062992125986035, -1.181102362204724310 ) ) ;
#58050=CARTESIAN_POINT ( 'NONE',  ( -0.3996062992125985480, -7.340648628747423112E-17, -0.5885826771653542844 ) ) ;
#58051=CARTESIAN_POINT ( 'NONE',  ( 4.893765752498283308E-17, -0.3996062992125985480, -0.1555118110236220763 ) ) ;
#58053=CARTESIAN_POINT ( 'NONE',  ( 0.3996062992125986035, 2.446882876249141962E-17, -2.637795275590551380 ) ) ;
#58054=CARTESIAN_POINT ( 'NONE',  ( -0.1958661417322836718, 0.3392501089628017219, -2.145013123359580387 ) ) ;
#58060=CARTESIAN_POINT ( 'NONE',  ( -0.1265901696524986964, -0.4724409448818899238, -1.566272965879265344 ) ) ;
#58063=CARTESIAN_POINT ( 'NONE',  ( 4.837279021331061486E-17, -0.3949938075777409963, -1.257874015748031260 ) ) ;
#58074=CARTESIAN_POINT ( 'NONE',  ( 0.1998031496062992463, 0.3460692066303959202, -2.268372703412073754 ) ) ;
#58076=CARTESIAN_POINT ( 'NONE',  ( -0.1049643490035301746, -0.3917322834645670659, -1.569534489992439497 ) ) ;
#58084=CARTESIAN_POINT ( 'NONE',  ( 0.2362204724409449064, 0.4091458600556404646, -2.349081364829396446 ) ) ;
#58088=CARTESIAN_POINT ( 'NONE',  ( -0.3460692066303960313, 0.1998031496062989965, 0.05446194225721784354 ) ) ;
#58090=CARTESIAN_POINT ( 'NONE',  ( -0.3917322834645669549, -0.1049643490035306603, -1.232939632545931863 ) ) ;
#58110=CARTESIAN_POINT ( 'NONE',  ( 0.2867679344610366554, -0.2867679344610365444, -2.452755905511810663 ) ) ;
#58113=CARTESIAN_POINT ( 'NONE',  ( 0.3458507752293908943, 0.3458507752293908943, -0.7677165354330709457 ) ) ;
#58114=CARTESIAN_POINT ( 'NONE',  ( -0.3996062992125987146, 0.1070741851644051862, 0.1246719160104986790 ) ) ;
#58117=CARTESIAN_POINT ( 'NONE',  ( 0.1049643490035303689, 0.3917322834645670104, -1.717847769028871596 ) ) ;
#58121=CARTESIAN_POINT ( 'NONE',  ( 0.4091458600556404646, -0.2362204724409448231, -2.782152230971128848 ) ) ;
#58128=CARTESIAN_POINT ( 'NONE',  ( -0.2867679344610364334, -0.2867679344610368219, -1.241450500491126707 ) ) ;
#58135=CARTESIAN_POINT ( 'NONE',  ( -0.2867679344610365444, -0.2867679344610367664, -2.575478633367141779 ) ) ;
#58144=CARTESIAN_POINT ( 'NONE',  ( -0.1049643490035302024, -0.3917322834645671215, -1.731627296587926468 ) ) ;
#58160=CARTESIAN_POINT ( 'NONE',  ( 0.3458507752293908943, -0.3458507752293908943, -0.4133858267716534196 ) ) ;
#58161=CARTESIAN_POINT ( 'NONE',  ( -0.2362204724409451284, 0.4091458600556402425, -0.4048556430446194621 ) ) ;
#58164=CARTESIAN_POINT ( 'NONE',  ( -0.1058382717557503072, 0.3949938075777408852, 0.2316272965879264401 ) ) ;
#58169=CARTESIAN_POINT ( 'NONE',  ( 0.3420746716998660508, -0.1974969037888704149, 0.1332020997375328031 ) ) ;
#58176=CARTESIAN_POINT ( 'NONE',  ( -0.3460692066303957537, -0.1998031496062994405, -0.7591863517060367661 ) ) ;
#58178=CARTESIAN_POINT ( 'NONE',  ( -0.1049643490035307020, 0.3917322834645669549, -0.7860892388451442558 ) ) ;
#58195=CARTESIAN_POINT ( 'NONE',  ( -0.3458507752293906723, -0.3458507752293910609, -2.655511811023622215 ) ) ;
#58213=CARTESIAN_POINT ( 'NONE',  ( -0.3996062992125985480, -0.1070741851644057135, -0.2034120734908136663 ) ) ;
#58214=CARTESIAN_POINT ( 'NONE',  ( 0.4724409448818898682, 2.892866454678787531E-17, -1.139763779527559029 ) ) ;
#58218=CARTESIAN_POINT ( 'NONE',  ( 4.893765752498283924E-17, -0.3996062992125986035, -2.598425196850393970 ) ) ;
#58219=CARTESIAN_POINT ( 'NONE',  ( -0.3949938075777411628, 0.1058382717557497937, -2.080052493438320216 ) ) ;
#58220=CARTESIAN_POINT ( 'NONE',  ( 0.1958661417322834775, 0.3392501089628018884, -0.6089238845144356871 ) ) ;
#58222=CARTESIAN_POINT ( 'NONE',  ( -0.3917322834645670104, -7.196005306013484475E-17, -0.8188976377952754682 ) ) ;
#58224=CARTESIAN_POINT ( 'NONE',  ( 0.3917322834645670104, 2.398668435337828261E-17, -1.055118110236220375 ) ) ;
#58226=CARTESIAN_POINT ( 'NONE',  ( 0.3420746716998660508, -0.1974969037888704149, -2.858923884514436242 ) ) ;
#58231=CARTESIAN_POINT ( 'NONE',  ( 0.4724409448818897572, -0.1265901696524988906, -2.788713910761154047 ) ) ;
#58232=CARTESIAN_POINT ( 'NONE',  ( -0.2925321140481932924, 0.2925321140481931814, -2.539370078740157410 ) ) ;
#58233=CARTESIAN_POINT ( 'NONE',  ( -0.3917322834645670659, -7.196005306013484475E-17, -1.295951074312022833 ) ) ;
#58240=CARTESIAN_POINT ( 'NONE',  ( -0.2867679344610365999, 0.2867679344610364889, -0.1043307086614174151 ) ) ;
#58249=CARTESIAN_POINT ( 'NONE',  ( -0.1308238996047441649, -0.3698506310986687806, -1.929133858267718660 ) ) ;
#58250=CARTESIAN_POINT ( 'NONE',  ( -0.1049643490035302024, -0.3917322834645671215, -1.954068241469816503 ) ) ;
#58251=CARTESIAN_POINT ( 'NONE',  ( -0.3392501089628017219, -0.1958661417322836718, -2.879265091863516979 ) ) ;
#58253=CARTESIAN_POINT ( 'NONE',  ( 0.3460692066303959757, -0.1998031496062991907, -0.1049868766404199599 ) ) ;
#58259=CARTESIAN_POINT ( 'NONE',  ( 0.3959418824714268648, 0.02190130575838933683, -1.929133858267716661 ) ) ;
#58260=CARTESIAN_POINT ( 'NONE',  ( 0.2867679344610365999, -0.2867679344610365444, -0.6555118110236222151 ) ) ;
#58280=CARTESIAN_POINT ( 'NONE',  ( -0.3392501089628018329, -0.1958661417322836440, -0.6049675608585809439 ) ) ;
#58289=CARTESIAN_POINT ( 'NONE',  ( 0.3917322834645670104, 2.398668435337828261E-17, -2.629921259842519898 ) ) ;
#58293=CARTESIAN_POINT ( 'NONE',  ( -0.4091458600556405756, 0.2362204724409446288, -1.205380577427821454 ) ) ;
#58307=CARTESIAN_POINT ( 'NONE',  ( 0.3460692066303958092, 0.1998031496062993018, -2.570209973753280863 ) ) ;
#58312=CARTESIAN_POINT ( 'NONE',  ( 0.3996062992125985480, 2.446882876249141654E-17, -1.927165354330708791 ) ) ;
#58317=CARTESIAN_POINT ( 'NONE',  ( 0.4724409448818898682, 2.892866454678787531E-17, -0.1181102362204724532 ) ) ;
#58319=CARTESIAN_POINT ( 'NONE',  ( 0.1998031496062992463, 0.3460692066303959202, -1.166010498687663821 ) ) ;
#58320=CARTESIAN_POINT ( 'NONE',  ( 0.1070741851644054915, -0.3996062992125986035, -0.8727034120734907807 ) ) ;
#58322=CARTESIAN_POINT ( 'NONE',  ( 0.3420746716998660508, -0.1974969037888703871, -0.5774278215223097588 ) ) ;
#58328=CARTESIAN_POINT ( 'NONE',  ( 0.2891555358219910499, 0.2891555358219910499, -1.789370078740157632 ) ) ;
#58333=CARTESIAN_POINT ( 'NONE',  ( -0.2362204724409451284, 0.4091458600556402425, -1.745406824146981561 ) ) ;
#58341=CARTESIAN_POINT ( 'NONE',  ( -0.2867679344610364334, -0.2867679344610368219, -2.028852075294276691 ) ) ;
#58342=CARTESIAN_POINT ( 'NONE',  ( 4.893765752498283308E-17, -0.3996062992125985480, -2.832677165354331006 ) ) ;
#58349=CARTESIAN_POINT ( 'NONE',  ( -0.2867679344610364334, -0.2867679344610367109, -1.468503937007874294 ) ) ;
#58352=CARTESIAN_POINT ( 'NONE',  ( 0.3949938075777411073, -0.1058382717557499464, -1.686351706036745668 ) ) ;
#58357=CARTESIAN_POINT ( 'NONE',  ( -0.3996062992125987146, 0.1070741851644051862, -0.1902887139107611314 ) ) ;
#58361=PRESENTATION_STYLE_ASSIGNMENT (( #53297 ) ) ;
#58364=DIRECTION ( 'NONE',  ( 0.000000000000000000, 0.000000000000000000, 1.000000000000000000 ) ) ;
#58365=CARTESIAN_POINT ( 'NONE',  ( 4.797336870675656522E-17, -0.3917322834645670104, -0.1633858267716536417 ) ) ;
#58373=CARTESIAN_POINT ( 'NONE',  ( 0.1070741851644054776, -0.3996062992125984925, -2.209317585301837195 ) ) ;
#58378=CARTESIAN_POINT ( 'NONE',  ( -0.4724409448818895907, -0.1265901696524993070, -0.8333333333333332593 ) ) ;
#58381=CARTESIAN_POINT ( 'NONE',  ( 0.3392501089628018884, -0.1958661417322834220, -0.2545931758530183275 ) ) ;
#58382=CARTESIAN_POINT ( 'NONE',  ( -0.1958661417322836718, 0.3392501089628017219, -1.987532808398950079 ) ) ;
#58386=CARTESIAN_POINT ( 'NONE',  ( 0.1265901696524990294, -0.4724409448818896462, -2.839238845144356649 ) ) ;
#58392=CARTESIAN_POINT ( 'NONE',  ( -0.2891555358219911054, 0.2891555358219909388, -2.773622047244094446 ) ) ;
#58394=CARTESIAN_POINT ( 'NONE',  ( 0.1049643490035304799, -0.3917322834645669549, -0.1699475065616798675 ) ) ;
#58399=CARTESIAN_POINT ( 'NONE',  ( 0.3392501089628018884, -0.1958661417322834220, -1.514435695538058013 ) ) ;
#58403=CARTESIAN_POINT ( 'NONE',  ( 5.785732909357575061E-17, -0.4724409448818898682, 0.1594488188976377896 ) ) ;
#58416=CARTESIAN_POINT ( 'NONE',  ( 0.2925321140481932369, 0.2925321140481932369, -1.159448818897637734 ) ) ;
#58417=CARTESIAN_POINT ( 'NONE',  ( 0.3392501089628018884, -0.1958661417322834220, -2.709317585301837195 ) ) ;
#58426=CARTESIAN_POINT ( 'NONE',  ( -0.1998031496062994683, 0.3460692066303958092, 0.1443569553805774119 ) ) ;
#58427=CARTESIAN_POINT ( 'NONE',  ( -0.2867679344610367109, 0.2867679344610365444, -2.378628239666354283 ) ) ;
#58433=CARTESIAN_POINT ( 'NONE',  ( 0.3917322834645670104, -0.1049643490035303411, -2.085958005249344271 ) ) ;
#58441=CARTESIAN_POINT ( 'NONE',  ( 0.1070741851644053527, 0.3996062992125986590, -1.410761154855643129 ) ) ;
#58444=CARTESIAN_POINT ( 'NONE',  ( 0.3917322834645670104, 0.1049643490035304660, -0.1214103918973247487 ) ) ;
#58458=CARTESIAN_POINT ( 'NONE',  ( -0.2867679344610365999, 0.2867679344610364889, -0.01181102362204719709 ) ) ;
#58461=CARTESIAN_POINT ( 'NONE',  ( 0.3420746716998659953, 0.1974969037888705536, -0.7611548556430446366 ) ) ;
#58475=CARTESIAN_POINT ( 'NONE',  ( -0.2925321140481930704, -0.2925321140481933480, -1.318897637795275690 ) ) ;
#58477=CARTESIAN_POINT ( 'NONE',  ( 0.3996062992125985480, 2.446882876249141654E-17, -0.8248031496062991907 ) ) ;
#58478=CARTESIAN_POINT ( 'NONE',  ( 0.1998031496062994128, -0.3460692066303957537, -0.3261154855643044748 ) ) ;
#58480=CARTESIAN_POINT ( 'NONE',  ( 0.3460692066303959757, -0.1998031496062991907, -2.782152230971128848 ) ) ;
#58481=CARTESIAN_POINT ( 'NONE',  ( 0.1958661417322834775, 0.3392501089628018884, -1.961286089238845287 ) ) ;
#58487=CARTESIAN_POINT ( 'NONE',  ( -0.1265901696524993347, 0.4724409448818895907, -1.343175853018372834 ) ) ;
#58490=CARTESIAN_POINT ( 'NONE',  ( 0.1974969037888706092, -0.3420746716998660508, -1.270997375328083878 ) ) ;
#58492=CARTESIAN_POINT ( 'NONE',  ( -0.1958661417322833942, -0.3392501089628018884, -1.637158423393387796 ) ) ;
#58501=CARTESIAN_POINT ( 'NONE',  ( -0.2925321140481930149, -0.2925321140481933480, -2.025590551181102317 ) ) ;
#58503=CARTESIAN_POINT ( 'NONE',  ( -0.3917322834645670659, 0.1049643490035301607, -2.002605356134171455 ) ) ;
#58516=CARTESIAN_POINT ( 'NONE',  ( -0.1070741851644056997, 0.3996062992125984925, 0.2316272965879264956 ) ) ;
#58518=CARTESIAN_POINT ( 'NONE',  ( 0.3917322834645670104, -0.1049643490035303411, -1.298556430446194510 ) ) ;
#58539=CARTESIAN_POINT ( 'NONE',  ( 0.1958661417322834775, 0.3392501089628018884, -2.656167979002624691 ) ) ;
#58542=CARTESIAN_POINT ( 'NONE',  ( 0.2362204724409449064, 0.4091458600556404646, -0.6167979002624671692 ) ) ;
#58544=CARTESIAN_POINT ( 'NONE',  ( -0.3996062992125987146, 0.1070741851644051862, -0.1902887139107611592 ) ) ;
#58547=CARTESIAN_POINT ( 'NONE',  ( 0.3392501089628018884, -0.1958661417322834220, -1.671916010498687655 ) ) ;
#58551=CARTESIAN_POINT ( 'NONE',  ( -0.01930322177395173144, 0.3957358693849742926, -2.755905511811586273 ) ) ;
#58558=CARTESIAN_POINT ( 'NONE',  ( 0.1958661417322834497, 0.3392501089628018329, -1.326752337761467837 ) ) ;
#58563=ORIENTED_EDGE ( 'NONE', *, *, #10855, .F. ) ;
#58564=CARTESIAN_POINT ( 'NONE',  ( -0.1049643490035302301, -0.3917322834645671770, -2.588601992947193509 ) ) ;
#58567=AXIS2_PLACEMENT_3D ( 'NONE', #528, #83019, #25342 ) ;
#58573=CARTESIAN_POINT ( 'NONE',  ( 0.1049643490035304938, -0.3917322834645669549, -1.902230971128608727 ) ) ;
#58583=VERTEX_POINT ( 'NONE', #54942 ) ;
#58588=CARTESIAN_POINT ( 'NONE',  ( -0.4724409448818895907, -0.1265901696524993070, -0.1227034120734908362 ) ) ;
#58591=CARTESIAN_POINT ( 'NONE',  ( -0.3949938075777409963, -7.255918531996591613E-17, 0.04133858267716533641 ) ) ;
#58596=CARTESIAN_POINT ( 'NONE',  ( -0.2891555358219909388, -0.2891555358219912164, 0.02165354330708659999 ) ) ;
#58603=CARTESIAN_POINT ( 'NONE',  ( 0.3460692066303958092, 0.1998031496062993018, -0.9954068241469815614 ) ) ;
#58605=CARTESIAN_POINT ( 'NONE',  ( 0.3392501089628018329, 0.1958661417322835607, -0.5958005249343831800 ) ) ;
#58608=CARTESIAN_POINT ( 'NONE',  ( -0.4724409448818898682, -8.678599364036362592E-17, -0.4311023622047244208 ) ) ;
#58620=CARTESIAN_POINT ( 'NONE',  ( -0.4724409448818898682, -8.678599364036362592E-17, -2.320866141732283783 ) ) ;
#58638=CARTESIAN_POINT ( 'NONE',  ( -0.3996062992125985480, -0.1070741851644057135, -0.3608923884514435576 ) ) ;
#58643=CARTESIAN_POINT ( 'NONE',  ( 0.3996062992125986035, 0.1070741851644054776, -2.644356955380577912 ) ) ;
#58644=CARTESIAN_POINT ( 'NONE',  ( -0.1974969037888706647, 0.3420746716998658843, -2.060367454068241067 ) ) ;
#58645=CARTESIAN_POINT ( 'NONE',  ( 0.3917322834645669549, 0.1049643490035304660, -0.5892388451443569819 ) ) ;
#58648=CARTESIAN_POINT ( 'NONE',  ( 0.3392501089628018329, 0.1958661417322835607, -0.9107611548556429071 ) ) ;
#58650=CARTESIAN_POINT ( 'NONE',  ( 0.1958661417322834775, 0.3392501089628018884, -1.238845144356955252 ) ) ;
#58652=CARTESIAN_POINT ( 'NONE',  ( -0.1049643490035301746, -0.3917322834645670659, 0.005268659613860090553 ) ) ;
#58659=CARTESIAN_POINT ( 'NONE',  ( -0.3996062992125986035, -7.340648628747425578E-17, -2.716535433070865757 ) ) ;
#58660=CARTESIAN_POINT ( 'NONE',  ( 0.1049643490035303967, 0.3917322834645670659, -1.250019315781839113 ) ) ;
#58666=CARTESIAN_POINT ( 'NONE',  ( 0.1049643490035304938, -0.3917322834645669549, -0.4849081364829396779 ) ) ;
#58675=CARTESIAN_POINT ( 'NONE',  ( 0.3392501089628018329, 0.1958661417322835607, -2.013123359580052618 ) ) ;
#58677=CARTESIAN_POINT ( 'NONE',  ( -0.1998031496062991907, -0.3460692066303959757, -0.06561679790026248016 ) ) ;
#58681=CARTESIAN_POINT ( 'NONE',  ( 0.3458507752293908943, 0.3458507752293908943, -2.419291338582677309 ) ) ;
#58684=CARTESIAN_POINT ( 'NONE',  ( -0.2867679344610364334, -0.2867679344610367109, -0.9311023622047245318 ) ) ;
#58687=CARTESIAN_POINT ( 'NONE',  ( -0.3981765293560192709, -0.002049465651759719426, -1.929133858267716217 ) ) ;
#58704=CARTESIAN_POINT ( 'NONE',  ( -0.1958661417322834497, -0.3392501089628018884, -0.9330515503598931781 ) ) ;
#58708=CARTESIAN_POINT ( 'NONE',  ( -0.3458507752293909498, 0.3458507752293908388, -0.8070866141732283561 ) ) ;
#58714=CARTESIAN_POINT ( 'NONE',  ( 0.1958661417322834775, 0.3392501089628018884, 0.01638488369322645480 ) ) ;
#58719=CARTESIAN_POINT ( 'NONE',  ( -0.1265901696524986964, -0.4724409448818899238, -1.251312335958005173 ) ) ;
#58729=CARTESIAN_POINT ( 'NONE',  ( 0.4091458600556403535, 0.2362204724409449896, -2.097769028871391050 ) ) ;
#58736=CARTESIAN_POINT ( 'NONE',  ( 0.1070741851644054776, -0.3996062992125984925, -2.366797900262467280 ) ) ;
#58740=CARTESIAN_POINT ( 'NONE',  ( 0.2925321140481932369, 0.2925321140481932369, -1.946850393700787496 ) ) ;
#58746=CARTESIAN_POINT ( 'NONE',  ( 0.1998031496062994128, -0.3460692066303957537, -1.113517060367454015 ) ) ;
#58747=CARTESIAN_POINT ( 'NONE',  ( 0.1998031496062994405, -0.3460692066303958092, -1.351706036745406792 ) ) ;
#58748=CARTESIAN_POINT ( 'NONE',  ( -0.1058382717557497937, -0.3949938075777411628, -0.7020997375328085210 ) ) ;
#58754=CARTESIAN_POINT ( 'NONE',  ( 0.3949938075777409963, 2.418639510665530743E-17, -1.927165354330708569 ) ) ;
#58759=CARTESIAN_POINT ( 'NONE',  ( -0.4724409448818895907, -0.1265901696524993070, -1.935695538057742526 ) ) ;
#58760=CARTESIAN_POINT ( 'NONE',  ( 0.3698506310979001177, -0.1308238996069263915, -2.755905511811022723 ) ) ;
#58766=CARTESIAN_POINT ( 'NONE',  ( 4.797336870675655290E-17, -0.3917322834645669549, -2.363497744585615123 ) ) ;
#58767=CARTESIAN_POINT ( 'NONE',  ( -0.1998031496062994405, 0.3460692066303957537, -2.767060367454068359 ) ) ;
#58773=CARTESIAN_POINT ( 'NONE',  ( -0.2867679344610364334, -0.2867679344610368219, -2.816253650097426231 ) ) ;
#58777=CARTESIAN_POINT ( 'NONE',  ( -0.3392501089628017219, -0.1958661417322836718, -1.934383202099737575 ) ) ;
#58780=CARTESIAN_POINT ( 'NONE',  ( 0.3949938075777409963, 2.418639510665530435E-17, -1.850393700787401396 ) ) ;
#58787=CARTESIAN_POINT ( 'NONE',  ( 0.2925321140481932369, -0.2925321140481932369, -0.5708661417322833387 ) ) ;
#58795=CARTESIAN_POINT ( 'NONE',  ( 0.1958661417322834775, 0.3392501089628018884, -0.2290026246719160941 ) ) ;
#58800=VERTEX_POINT ( 'NONE', #55350 ) ;
#58802=CARTESIAN_POINT ( 'NONE',  ( 0.3996062992125985480, 2.446882876249141654E-17, -1.927165354330708569 ) ) ;
#58807=CARTESIAN_POINT ( 'NONE',  ( 0.1265901696524989462, 0.4724409448818897572, -1.253280839895013044 ) ) ;
#58810=CARTESIAN_POINT ( 'NONE',  ( -0.3392501089628019995, 0.1958661417322832277, -0.4908136482939632339 ) ) ;
#58811=DIRECTION ( 'NONE',  ( 0.000000000000000000, 0.000000000000000000, 1.000000000000000000 ) ) ;
#58815=CARTESIAN_POINT ( 'NONE',  ( -0.1998031496062991630, -0.3460692066303959202, -0.1423884514435695692 ) ) ;
#58820=CARTESIAN_POINT ( 'NONE',  ( -0.3949938075777409963, -7.255918531996591613E-17, -2.793307086614173151 ) ) ;
#58822=CARTESIAN_POINT ( 'NONE',  ( 0.3917322834645670104, -0.1049643490035303273, -0.1961942257217848540 ) ) ;
#58827=CARTESIAN_POINT ( 'NONE',  ( -0.2867679344610365999, 0.2867679344610364889, -1.744094488188976610 ) ) ;
#58830=CARTESIAN_POINT ( 'NONE',  ( 0.4724409448818897572, -0.1265901696524988906, -0.03083989501312336262 ) ) ;
#58834=CARTESIAN_POINT ( 'NONE',  ( 0.2362204724409449064, 0.4091458600556404646, -0.6935695538057742304 ) ) ;
#58843=CARTESIAN_POINT ( 'NONE',  ( -9.787531504996566615E-17, 0.3996062992125985480, -1.021653543307086576 ) ) ;
#58844=CARTESIAN_POINT ( 'NONE',  ( 0.2867679344610365999, -0.2867679344610365444, -2.545275590551181022 ) ) ;
#58854=CARTESIAN_POINT ( 'NONE',  ( -0.1998031496062991907, -0.3460692066303959757, 0.09186351706036742504 ) ) ;
#58855=CARTESIAN_POINT ( 'NONE',  ( 0.3917322834645670659, -0.1049643490035303273, -2.470491756726720833 ) ) ;
#58862=CARTESIAN_POINT ( 'NONE',  ( 0.1049643490035303689, 0.3917322834645670104, -2.440288713910760521 ) ) ;
#58869=CARTESIAN_POINT ( 'NONE',  ( -0.1998031496062991907, -0.3460692066303959757, -1.167979002624671914 ) ) ;
#58871=CARTESIAN_POINT ( 'NONE',  ( 0.1958661417322836718, -0.3392501089628017219, 0.06887832201343642435 ) ) ;
#58882=CARTESIAN_POINT ( 'NONE',  ( 0.3392501089628018884, -0.1958661417322834220, -0.2545931758530183275 ) ) ;
#58885=CARTESIAN_POINT ( 'NONE',  ( -0.1974969037888703871, -0.3420746716998661063, -0.5380577427821522374 ) ) ;
#58900=CARTESIAN_POINT ( 'NONE',  ( 0.1070741851644054915, -0.3996062992125986035, -1.187664041994750619 ) ) ;
#58902=CARTESIAN_POINT ( 'NONE',  ( 0.1998031496062992463, 0.3460692066303959202, -0.6935695538057742304 ) ) ;
#58903=CARTESIAN_POINT ( 'NONE',  ( 0.1070741851644054776, -0.3996062992125984925, -0.004593175853018396058 ) ) ;
#58905=CARTESIAN_POINT ( 'NONE',  ( -0.3460692066303960868, 0.1998031496062990242, -2.703412073490813583 ) ) ;
#58906=CARTESIAN_POINT ( 'NONE',  ( 0.1958661417322836440, -0.3392501089628017219, -2.223753280839895208 ) ) ;
#58913=CARTESIAN_POINT ( 'NONE',  ( 0.4091458600556404646, -0.2362204724409448231, -1.441601049868766582 ) ) ;
#58916=CARTESIAN_POINT ( 'NONE',  ( 0.1974969037888704704, 0.3420746716998660508, -1.480971128608923548 ) ) ;
#58926=CARTESIAN_POINT ( 'NONE',  ( -0.1998031496062991630, -0.3460692066303959202, -2.347112860892388575 ) ) ;
#58927=CARTESIAN_POINT ( 'NONE',  ( -0.3917322834645669549, -7.196005306013483243E-17, -2.166647350884827183 ) ) ;
#58932=EDGE_CURVE ( 'NONE', #21240, #400, #42722, .T. ) ;
#58941=CARTESIAN_POINT ( 'NONE',  ( -0.3460692066303960313, 0.1998031496062989965, 0.2119422572178477626 ) ) ;
#58943=CARTESIAN_POINT ( 'NONE',  ( 4.797336870675656522E-17, -0.3917322834645670104, -1.580708661417322913 ) ) ;
#58965=CARTESIAN_POINT ( 'NONE',  ( 4.797336870675656522E-17, -0.3917322834645670104, -2.275590551181102317 ) ) ;
#58968=CARTESIAN_POINT ( 'NONE',  ( -0.3458507752293906723, -0.3458507752293910609, -0.6889763779527556808 ) ) ;
#58969=CARTESIAN_POINT ( 'NONE',  ( -0.3460692066303958092, -0.1998031496062994683, -0.2099737532808399199 ) ) ;
#58973=CARTESIAN_POINT ( 'NONE',  ( 0.3392501089628018884, -0.1958661417322834220, -1.829396325459317518 ) ) ;
#58984=CARTESIAN_POINT ( 'NONE',  ( 0.2867679344610365999, -0.2867679344610365999, -1.123340264270654698 ) ) ;
#58990=CARTESIAN_POINT ( 'NONE',  ( -0.2867679344610367109, 0.2867679344610365444, -2.536108554626983480 ) ) ;
#58998=CARTESIAN_POINT ( 'NONE',  ( 0.3917322834645669549, 0.1049643490035304660, -1.784120734908136274 ) ) ;
#59013=CARTESIAN_POINT ( 'NONE',  ( 0.3458507752293908943, 0.3458507752293908943, -0.05708661417322836301 ) ) ;
#59016=CARTESIAN_POINT ( 'NONE',  ( -0.2891555358219911054, 0.2891555358219909388, 0.06102362204724409017 ) ) ;
#59021=CARTESIAN_POINT ( 'NONE',  ( 0.1974969037888704704, 0.3420746716998660508, -0.2211286089238845842 ) ) ;
#59028=CARTESIAN_POINT ( 'NONE',  ( -0.1998031496062994405, 0.3460692066303957537, -1.034776902887139194 ) ) ;
#59030=CARTESIAN_POINT ( 'NONE',  ( -0.1958661417322834220, -0.3392501089628018884, -0.8451443569553805935 ) ) ;
#59043=CARTESIAN_POINT ( 'NONE',  ( -0.3928700489057014855, 0.01966910102760518683, -1.220472440944881276 ) ) ;
#59045=CARTESIAN_POINT ( 'NONE',  ( 0.4724409448818898682, 2.892866454678787531E-17, -2.714566929133858331 ) ) ;
#59061=CARTESIAN_POINT ( 'NONE',  ( -9.787531504996567848E-17, 0.3996062992125986035, -0.9448818897637796255 ) ) ;
#59066=CARTESIAN_POINT ( 'NONE',  ( 0.1070741851644053527, 0.3996062992125986590, -2.828083989501312345 ) ) ;
#59067=CARTESIAN_POINT ( 'NONE',  ( -0.1974969037888703871, -0.3420746716998661063, -1.797900262467191590 ) ) ;
#59068=CARTESIAN_POINT ( 'NONE',  ( -0.3392501089628019995, 0.1958661417322832277, -0.3333333333333333148 ) ) ;
#59069=CARTESIAN_POINT ( 'NONE',  ( 0.3392501089628018329, 0.1958661417322835607, -1.068241469816272771 ) ) ;
#59071=CARTESIAN_POINT ( 'NONE',  ( 0.1958661417322834775, 0.3392501089628018884, -1.081364829396325389 ) ) ;
#59073=CARTESIAN_POINT ( 'NONE',  ( -0.2891555358219909388, -0.2891555358219912164, -2.812992125984251857 ) ) ;
#59079=CARTESIAN_POINT ( 'NONE',  ( -0.3996062992125986035, -7.340648628747425578E-17, -2.559055118110236560 ) ) ;
#59080=CARTESIAN_POINT ( 'NONE',  ( -0.1049643490035307158, 0.3917322834645670104, -1.263142675361891731 ) ) ;
#59086=CARTESIAN_POINT ( 'NONE',  ( -0.2867679344610364334, -0.2867679344610367109, -0.6161417322834646937 ) ) ;
#59094=CARTESIAN_POINT ( 'NONE',  ( -0.06912221444153182626, -0.3857315817376797962, -1.929133858267716661 ) ) ;
#59095=CARTESIAN_POINT ( 'NONE',  ( 0.2867679344610365999, -0.2867679344610365444, -2.137795275590551380 ) ) ;
#59097=CARTESIAN_POINT ( 'NONE',  ( 0.1070741851644054915, -0.3996062992125986035, -0.2427821522309711877 ) ) ;
#59098=VERTEX_POINT ( 'NONE', #30920 ) ;
#59104=CARTESIAN_POINT ( 'NONE',  ( 0.3917322834645670104, 2.398668435337828261E-17, -0.9901574803149607584 ) ) ;
#59124=CARTESIAN_POINT ( 'NONE',  ( 0.3392501089628018329, -0.1958661417322834497, -0.9724216291000506995 ) ) ;
#59127=CARTESIAN_POINT ( 'NONE',  ( -0.1958661417322836718, 0.3392501089628017219, -1.200131233595800540 ) ) ;
#59133=CARTESIAN_POINT ( 'NONE',  ( 0.3917322834645670659, 2.398668435337828261E-17, 0.04263160285333144478 ) ) ;
#59137=CARTESIAN_POINT ( 'NONE',  ( -0.3458507752293909498, 0.3458507752293907833, -1.513779527559054872 ) ) ;
#59147=CARTESIAN_POINT ( 'NONE',  ( 0.2362204724409449064, 0.4091458600556404646, -2.110892388451443225 ) ) ;
#59153=CARTESIAN_POINT ( 'NONE',  ( -0.3460692066303960313, 0.1998031496062989965, -2.780183727034120977 ) ) ;
#59157=CARTESIAN_POINT ( 'NONE',  ( 0.3996062992125984925, 0.1070741851644054637, -1.776246719160104570 ) ) ;
#59162=CARTESIAN_POINT ( 'NONE',  ( -0.2925321140481932369, 0.2925321140481930704, -0.8838582677165351953 ) ) ;
#59163=CARTESIAN_POINT ( 'NONE',  ( -0.3996062992125986035, -0.1070741851644056997, -1.463254593175853158 ) ) ;
#59164=CARTESIAN_POINT ( 'NONE',  ( -0.3949938075777411628, 0.1058382717557497937, -0.5052493438320211361 ) ) ;
#59169=CARTESIAN_POINT ( 'NONE',  ( 0.1058382717557499880, 0.3949938075777409408, -1.802493438320210251 ) ) ;
#59174=CARTESIAN_POINT ( 'NONE',  ( 0.2362204724409451007, -0.4091458600556402980, -1.981627296587926690 ) ) ;
#59182=CARTESIAN_POINT ( 'NONE',  ( 0.3392501089628018329, 0.1958661417322835052, -2.415991182905824708 ) ) ;
#59183=CARTESIAN_POINT ( 'NONE',  ( -0.2925321140481932369, 0.2925321140481931259, -2.773622047244094002 ) ) ;
#59188=CARTESIAN_POINT ( 'NONE',  ( 4.797336870675656522E-17, -0.3917322834645670104, 0.1515748031496061965 ) ) ;
#59190=CARTESIAN_POINT ( 'NONE',  ( 0.3917322834645670104, -0.1049643490035303411, -1.835958005249343827 ) ) ;
#59193=CARTESIAN_POINT ( 'NONE',  ( 0.1974969037888704704, 0.3420746716998660508, -1.876640419947506633 ) ) ;
#59198=CARTESIAN_POINT ( 'NONE',  ( -0.1998031496062994683, 0.3460692066303958092, -0.4855643044619422644 ) ) ;
#59205=CARTESIAN_POINT ( 'NONE',  ( -0.1049643490035302024, -0.3917322834645671215, -0.4717847769028871152 ) ) ;
#59215=CARTESIAN_POINT ( 'NONE',  ( 5.785732909357575061E-17, -0.4724409448818898682, -1.181102362204724310 ) ) ;
#59218=CARTESIAN_POINT ( 'NONE',  ( -0.3917322834645671215, 0.1049643490035301469, -0.3398950131233596239 ) ) ;
#59219=CARTESIAN_POINT ( 'NONE',  ( 0.3392501089628018329, 0.1958661417322835607, -2.420603674540682260 ) ) ;
#59222=CARTESIAN_POINT ( 'NONE',  ( 0.1998031496062994128, -0.3460692066303957537, -0.1686351706036745557 ) ) ;
#59227=CARTESIAN_POINT ( 'NONE',  ( 0.2891555358219910499, -0.2891555358219909944, -2.537401574803150428 ) ) ;
#59229=CARTESIAN_POINT ( 'NONE',  ( 0.1958661417322836440, -0.3392501089628017219, -0.01902887139107619849 ) ) ;
#59234=CARTESIAN_POINT ( 'NONE',  ( 0.3392501089628018329, 0.1958661417322835607, -1.855643044619422533 ) ) ;
#59249=EDGE_CURVE ( 'NONE', #51988, #29367, #75107, .T. ) ;
#59253=CARTESIAN_POINT ( 'NONE',  ( 0.1070741851644054776, -0.3996062992125984925, -1.106955380577427706 ) ) ;
#59254=CARTESIAN_POINT ( 'NONE',  ( -0.1049643490035307020, 0.3917322834645669549, -2.768372703412072866 ) ) ;
#59263=CARTESIAN_POINT ( 'NONE',  ( -0.2925321140481930704, -0.2925321140481933480, -0.2165354330708661734 ) ) ;
#59264=CARTESIAN_POINT ( 'NONE',  ( -0.1049643490035307158, 0.3917322834645670104, -2.680465510007561836 ) ) ;
#59269=CARTESIAN_POINT ( 'NONE',  ( -0.2867679344610364334, -0.2867679344610367109, -2.505905511811023612 ) ) ;
#59275=CARTESIAN_POINT ( 'NONE',  ( -0.1070741851644057135, 0.3996062992125985480, -2.053805774278214979 ) ) ;
#59277=CARTESIAN_POINT ( 'NONE',  ( -0.1998031496062994683, 0.3460692066303958092, -1.745406824146981561 ) ) ;
#59279=CARTESIAN_POINT ( 'NONE',  ( -0.2867679344610367109, 0.2867679344610365444, -0.4888644601387945876 ) ) ;
#59292=CARTESIAN_POINT ( 'NONE',  ( 0.3917322834645670104, -0.1049643490035303411, -0.7335958005249343383 ) ) ;
#59295=CARTESIAN_POINT ( 'NONE',  ( -0.2891555358219908833, -0.2891555358219912164, -0.6889763779527559029 ) ) ;
#59296=ORIENTED_EDGE ( 'NONE', *, *, #14203, .T. ) ;
#59306=CARTESIAN_POINT ( 'NONE',  ( 0.3392501089628018884, -0.1958661417322834220, -2.866797900262466836 ) ) ;
#59311=CARTESIAN_POINT ( 'NONE',  ( 0.3996062992125986590, -0.1070741851644053111, -1.213910761154855189 ) ) ;
#59313=CARTESIAN_POINT ( 'NONE',  ( 0.1070741851644054776, -0.3996062992125984925, -0.9494750656167976199 ) ) ;
#59314=CARTESIAN_POINT ( 'NONE',  ( 0.3996062992125985480, 2.446882876249141654E-17, -0.5098425196850393526 ) ) ;
#59316=CARTESIAN_POINT ( 'NONE',  ( -0.1265901696524993347, 0.4724409448818895907, 0.1509186351706036378 ) ) ;
#59317=CARTESIAN_POINT ( 'NONE',  ( -0.3917322834645669549, -0.1049643490035306603, -2.020341207349081181 ) ) ;
#59323=CARTESIAN_POINT ( 'NONE',  ( 0.4091458600556403535, 0.2362204724409449896, -1.782808398950131101 ) ) ;
#59326=CARTESIAN_POINT ( 'NONE',  ( -0.2891555358219909388, -0.2891555358219912164, -1.238188976377952999 ) ) ;
#59336=CARTESIAN_POINT ( 'NONE',  ( 0.3460692066303959202, -0.1998031496062991630, -2.701443569553806157 ) ) ;
#59337=CARTESIAN_POINT ( 'NONE',  ( 0.2867679344610365999, 0.2867679344610365999, -2.107592232774591068 ) ) ;
#59349=CARTESIAN_POINT ( 'NONE',  ( 4.893765752498283308E-17, -0.3996062992125985480, 0.1594488188976377896 ) ) ;
#59351=CARTESIAN_POINT ( 'NONE',  ( 0.1049643490035304938, -0.3917322834645669549, -1.429790026246719359 ) ) ;
#59373=CARTESIAN_POINT ( 'NONE',  ( -0.3917322834645671215, 0.1049643490035301469, -2.387139107611548461 ) ) ;
#59375=EDGE_CURVE ( 'NONE', #14913, #18027, #74090, .T. ) ;
#59377=CARTESIAN_POINT ( 'NONE',  ( 0.2925321140481932369, -0.2925321140481932369, 0.05905511811023619884 ) ) ;
#59380=CARTESIAN_POINT ( 'NONE',  ( 0.2867679344610365999, -0.2867679344610365444, -1.822834645669291653 ) ) ;
#59391=CARTESIAN_POINT ( 'NONE',  ( -0.1049643490035301746, -0.3917322834645670659, -1.097093545110549462 ) ) ;
#59397=CARTESIAN_POINT ( 'NONE',  ( -9.594673741351313045E-17, 0.3917322834645670659, -2.358943200296274689 ) ) ;
#59399=ORIENTED_EDGE ( 'NONE', *, *, #15762, .T. ) ;
#59403=EDGE_CURVE ( 'NONE', #56613, #70572, #1861, .T. ) ;
#59406=CARTESIAN_POINT ( 'NONE',  ( -9.594673741351313045E-17, 0.3917322834645670104, -1.974409448818897683 ) ) ;
#59415=CARTESIAN_POINT ( 'NONE',  ( 0.2925321140481932369, -0.2925321140481932369, -1.988188976377952777 ) ) ;
#59421=CARTESIAN_POINT ( 'NONE',  ( 0.3458507752293908943, -0.3458507752293908943, -0.6476377952755905110 ) ) ;
#59424=CARTESIAN_POINT ( 'NONE',  ( -0.3949938075777409963, -7.255918531996591613E-17, -0.2736220472440945017 ) ) ;
#59430=CARTESIAN_POINT ( 'NONE',  ( -0.1058382717557497660, -0.3949938075777411073, -0.3064304461942257696 ) ) ;
#59439=CARTESIAN_POINT ( 'NONE',  ( -0.3460692066303957537, -0.1998031496062994405, -1.074146981627296604 ) ) ;
#59441=CARTESIAN_POINT ( 'NONE',  ( -9.594673741351313045E-17, 0.3917322834645670104, -0.6220472440944880832 ) ) ;
#59458=CARTESIAN_POINT ( 'NONE',  ( -0.4091458600556402980, -0.2362204724409451284, -2.806430446194225770 ) ) ;
#59465=CARTESIAN_POINT ( 'NONE',  ( 0.2362204724409449064, 0.4091458600556404646, -2.034120734908136718 ) ) ;
#59474=CARTESIAN_POINT ( 'NONE',  ( 0.1998031496062992740, 0.3460692066303959757, -0.9317585301837270073 ) ) ;
#59479=CARTESIAN_POINT ( 'NONE',  ( 0.1070741851644053527, 0.3996062992125986590, -2.670603674540682260 ) ) ;
#59480=CARTESIAN_POINT ( 'NONE',  ( 0.2891555358219910499, -0.2891555358219909944, -1.830708661417323135 ) ) ;
#59482=CARTESIAN_POINT ( 'NONE',  ( 0.3917322834645670104, 2.398668435337828261E-17, -0.7401574803149605364 ) ) ;
#59485=CARTESIAN_POINT ( 'NONE',  ( 0.3392501089628018329, 0.1958661417322835607, -1.068241469816272771 ) ) ;
#59487=CARTESIAN_POINT ( 'NONE',  ( 0.1049643490035303689, 0.3917322834645668994, 0.08400881709417505616 ) ) ;
#59493=CARTESIAN_POINT ( 'NONE',  ( 0.3996062992125986035, 2.446882876249141962E-17, -2.795275590551181022 ) ) ;
#59494=CARTESIAN_POINT ( 'NONE',  ( -0.1049643490035307158, 0.3917322834645670104, -1.105662360401261868 ) ) ;
#59500=CARTESIAN_POINT ( 'NONE',  ( 0.1958661417322834775, 0.3392501089628018884, -0.3864829396325459854 ) ) ;
#59508=CARTESIAN_POINT ( 'NONE',  ( 0.3428707098289829891, -0.1906283239480039415, -1.929133858267717549 ) ) ;
#59509=CARTESIAN_POINT ( 'NONE',  ( 0.3392501089628018884, -0.1958661417322834220, -1.829396325459317518 ) ) ;
#59511=CARTESIAN_POINT ( 'NONE',  ( 0.1998031496062994405, -0.3460692066303958092, -0.2493438320209974135 ) ) ;
#59512=VERTEX_POINT ( 'NONE', #60755 ) ;
#59517=CARTESIAN_POINT ( 'NONE',  ( -0.1958661417322836718, 0.3392501089628017219, -1.200131233595800540 ) ) ;
#59519=CARTESIAN_POINT ( 'NONE',  ( -0.3992723400743253825, -6.536159750466813772E-18, -1.929133858267716661 ) ) ;
#59522=VERTEX_POINT ( 'NONE', #23689 ) ;
#59537=CARTESIAN_POINT ( 'NONE',  ( 0.2867679344610365999, -0.2867679344610365999, -1.123340264270654698 ) ) ;
#59538=AXIS2_PLACEMENT_3D ( 'NONE', #3162, #37510, #79784 ) ;
#59548=CARTESIAN_POINT ( 'NONE',  ( 0.1049643490035304799, -0.3917322834645670104, -0.2395206281177972019 ) ) ;
#59551=CARTESIAN_POINT ( 'NONE',  ( -0.4724409448818895907, -0.1265901696524993070, -1.697506561679789971 ) ) ;
#59565=ORIENTED_EDGE ( 'NONE', *, *, #64580, .T. ) ;
#59566=CARTESIAN_POINT ( 'NONE',  ( 0.3460692066303958092, 0.1998031496062993018, -2.727690288713910949 ) ) ;
#59571=CARTESIAN_POINT ( 'NONE',  ( 0.1070741851644053388, 0.3996062992125986035, -1.645013123359579943 ) ) ;
#59577=CARTESIAN_POINT ( 'NONE',  ( 0.3996062992125986590, -0.1070741851644053111, -1.528871391076114916 ) ) ;
#59578=CARTESIAN_POINT ( 'NONE',  ( 0.3949938075777411073, -0.1058382717557499464, -0.7414698162729659314 ) ) ;
#59584=CARTESIAN_POINT ( 'NONE',  ( -0.1974969037888704149, -0.3420746716998661063, -1.559711286089239035 ) ) ;
#59588=CARTESIAN_POINT ( 'NONE',  ( 0.4724409448818898682, 2.892866454678787531E-17, -2.007874015748031482 ) ) ;
#59589=CARTESIAN_POINT ( 'NONE',  ( 0.3913445824879516199, -0.02733964191756152462, -2.755905511811024056 ) ) ;
#59597=CARTESIAN_POINT ( 'NONE',  ( 0.2867679344610365999, 0.2867679344610365999, -2.422552862695851683 ) ) ;
#59603=CARTESIAN_POINT ( 'NONE',  ( 0.1049643490035303689, 0.3917322834645668994, -2.750636852197163584 ) ) ;
#59605=CARTESIAN_POINT ( 'NONE',  ( -0.3392501089628019995, 0.1958661417322832277, -1.750656167979002698 ) ) ;
#59608=CARTESIAN_POINT ( 'NONE',  ( -0.3949938075777411628, 0.1058382717557497937, -2.395013123359580387 ) ) ;
#59613=CARTESIAN_POINT ( 'NONE',  ( 4.893765752498283924E-17, -0.3996062992125986035, -0.7086614173228346081 ) ) ;
#59617=FILL_AREA_STYLE_COLOUR ( '', #78129 ) ;
#59618=CARTESIAN_POINT ( 'NONE',  ( -0.2867679344610364334, -0.2867679344610367109, -0.1437007874015748810 ) ) ;
#59620=CARTESIAN_POINT ( 'NONE',  ( 0.3392501089628018884, -0.1958661417322834220, -0.8195538057742782767 ) ) ;
#59625=CARTESIAN_POINT ( 'NONE',  ( 0.3917322834645669549, 0.1049643490035304660, 0.04068241469816277767 ) ) ;
#59630=CARTESIAN_POINT ( 'NONE',  ( 0.2362204724409451007, -0.4091458600556402980, -1.351706036745406792 ) ) ;
#59632=CARTESIAN_POINT ( 'NONE',  ( -0.2867679344610365999, 0.2867679344610364889, -0.1692913385826771144 ) ) ;
#59633=CARTESIAN_POINT ( 'NONE',  ( 0.1049643490035304799, -0.3917322834645669549, -2.532152230971127960 ) ) ;
#59636=CARTESIAN_POINT ( 'NONE',  ( -0.3996062992125984925, -0.1070741851644056858, -0.1227034120734908501 ) ) ;
#59641=CARTESIAN_POINT ( 'NONE',  ( -9.674558042662122972E-17, 0.3949938075777409963, -2.596456692913385655 ) ) ;
#59643=CARTESIAN_POINT ( 'NONE',  ( -0.2867679344610366554, 0.2867679344610365444, -0.1043307086614174151 ) ) ;
#59649=CARTESIAN_POINT ( 'NONE',  ( -0.3917322834645670104, -7.196005306013484475E-17, -2.078740157480314821 ) ) ;
#59653=CARTESIAN_POINT ( 'NONE',  ( 0.3458507752293908943, 0.3458507752293908943, -0.3720472440944882497 ) ) ;
#59667=CARTESIAN_POINT ( 'NONE',  ( 4.893765752498283308E-17, -0.3996062992125985480, -1.572834645669291431 ) ) ;
#59668=CARTESIAN_POINT ( 'NONE',  ( -0.1049643490035302024, -0.3917322834645671215, -2.833989501312335957 ) ) ;
#59676=CARTESIAN_POINT ( 'NONE',  ( 0.3996062992125986590, -0.1070741851644053111, 0.04593175853018371946 ) ) ;
#59677=CARTESIAN_POINT ( 'NONE',  ( 0.3392501089628018884, -0.1958661417322833942, -2.463930076936694746 ) ) ;
#59682=CARTESIAN_POINT ( 'NONE',  ( -0.1958661417322836718, 0.3392501089628017219, -2.302493438320210029 ) ) ;
#59691=CARTESIAN_POINT ( 'NONE',  ( -0.1049643490035302301, -0.3917322834645671770, -0.3838775834983745860 ) ) ;
#59705=CARTESIAN_POINT ( 'NONE',  ( -0.3917322834645670104, -7.196005306013484475E-17, -0.6614173228346454936 ) ) ;
#59707=VERTEX_POINT ( 'NONE', #80558 ) ;
#59708=CARTESIAN_POINT ( 'NONE',  ( -0.3420746716998661618, 0.1974969037888702206, -1.128608923884514503 ) ) ;
#59720=CARTESIAN_POINT ( 'NONE',  ( -0.2362204724409447953, -0.4091458600556404646, -2.742782152230971437 ) ) ;
#59725=CARTESIAN_POINT ( 'NONE',  ( -0.3996062992125986035, -0.1070741851644056997, -1.305774278215223072 ) ) ;
#59727=CARTESIAN_POINT ( 'NONE',  ( 4.893765752498283308E-17, -0.3996062992125985480, -1.257874015748031260 ) ) ;
#59728=CARTESIAN_POINT ( 'NONE',  ( -0.1070741851644056997, 0.3996062992125984925, -0.5557742782152230721 ) ) ;
#59730=CARTESIAN_POINT ( 'NONE',  ( -0.4724409448818898682, -8.678599364036362592E-17, -0.03937007874015747977 ) ) ;
#59731=( BOUNDED_CURVE ( )  B_SPLINE_CURVE ( 2, ( #27960, #48144, #72997, #48556, #73841, #9030, #3542, #61613, #74253, #40591, #34703, #9855, #15772, #79747, #22482, #23301, #16595, #66273, #2300, #59944, #28791, #16181, #53619, #10276, #60365, #48971, #2712, #54454, #28373, #8612, #34282, #22064, #67107, #73422, #9438, #35109, #35525, #61187, #54875, #80581, #75331, #23145, #17275, #74098, #36193, #3388, #29869, #55531, #61864, #43308, #74930, #69425, #54722, #80428, #37431, #4205, #22738, #42903, #29464, #82066, #67784, #49638, #68598, #62695, #81240, #23556, #61453, #49225, #75745, #10122, #10537, #11357, #69006, #30282, #3801, #10938, #74513, #48814, #16860, #36595, #17678, #37015, #42498, #35785, #81660, #24379, #5035, #62273, #4610, #29052, #30703, #55122, #80831, #56367, #50051, #68199, #18086, #55947, #16444, #43721, #23971, #11778, #48398, #42089, #19307, #12590, #38248, #64762, #800, #26463, #13847, #83289, #56771, #6262, #50867, #51693, #25612, #32352, #51275, #20152, #63104, #25201, #70235, #13425, #44959, #63926, #63516, #76158, #7101 ),
 .UNSPECIFIED., .F., .F. ) 
 B_SPLINE_CURVE_WITH_KNOTS ( ( 3, 2, 2, 2, 2, 2, 2, 2, 2, 2, 2, 2, 2, 2, 2, 2, 2, 2, 2, 2, 2, 2, 2, 2, 2, 2, 2, 2, 2, 2, 2, 2, 2, 2, 2, 2, 2, 2, 2, 2, 2, 2, 2, 2, 2, 2, 2, 2, 2, 2, 2, 2, 2, 2, 2, 2, 2, 2, 2, 2, 2, 2, 2, 2, 3 ),
 ( 0.6881378855240343206, 0.6916666666666666519, 0.6958333333333333037, 0.6999999999999999556, 0.7041666666666667185, 0.7083333333333333703, 0.7125000000000000222, 0.7166666666666666741, 0.7208333333333333259, 0.7249999999999999778, 0.7291666666666666297, 0.7333333333333332815, 0.7375000000000000444, 0.7416666666666666963, 0.7458333333333333481, 0.7500000000000000000, 0.7541666666666666519, 0.7583333333333333037, 0.7624999999999999556, 0.7666666666666667185, 0.7708333333333333703, 0.7750000000000000222, 0.7791666666666666741, 0.7833333333333333259, 0.7874999999999999778, 0.7916666666666666297, 0.7958333333333332815, 0.8000000000000000444, 0.8041666666666666963, 0.8083333333333333481, 0.8125000000000000000, 0.8166666666666666519, 0.8208333333333333037, 0.8249999999999999556, 0.8291666666666667185, 0.8333333333333333703, 0.8375000000000000222, 0.8416666666666666741, 0.8458333333333333259, 0.8499999999999999778, 0.8541666666666666297, 0.8583333333333332815, 0.8625000000000000444, 0.8666666666666666963, 0.8708333333333333481, 0.8750000000000000000, 0.8791666666666666519, 0.8833333333333333037, 0.8874999999999999556, 0.8916666666666667185, 0.8958333333333333703, 0.9000000000000000222, 0.9041666666666666741, 0.9083333333333333259, 0.9124999999999999778, 0.9166666666666666297, 0.9208333333333332815, 0.9250000000000000444, 0.9291666666666666963, 0.9333333333333333481, 0.9375000000000000000, 0.9416666666666666519, 0.9458333333333333037, 0.9499999999999999556, 0.9506378855240344983 ),
 .UNSPECIFIED. ) 
 CURVE ( )  GEOMETRIC_REPRESENTATION_ITEM ( )  RATIONAL_B_SPLINE_CURVE ( ( 0.9911642120908021880, 0.9711423276059405474, 1.000000000000000000, 0.9659258262890683122, 1.000000000000000000, 0.9659258262890683122, 1.000000000000000000, 0.9659258262890683122, 1.000000000000000000, 0.9659258262890683122, 1.000000000000000000, 0.9659258262890683122, 1.000000000000000000, 0.9659258262890683122, 1.000000000000000000, 0.9659258262890683122, 1.000000000000000000, 0.9659258262890683122, 1.000000000000000000, 0.9659258262890683122, 1.000000000000000000, 0.9659258262890683122, 1.000000000000000000, 0.9659258262890683122, 1.000000000000000000, 0.9659258262890683122, 1.000000000000000000, 0.9659258262890683122, 1.000000000000000000, 0.9659258262890683122, 1.000000000000000000, 0.9659258262890683122, 1.000000000000000000, 0.9659258262890683122, 1.000000000000000000, 0.9659258262890683122, 1.000000000000000000, 0.9659258262890683122, 1.000000000000000000, 0.9659258262890683122, 1.000000000000000000, 0.9659258262890683122, 1.000000000000000000, 0.9659258262890683122, 1.000000000000000000, 0.9659258262890683122, 1.000000000000000000, 0.9659258262890683122, 1.000000000000000000, 0.9659258262890683122, 1.000000000000000000, 0.9659258262890683122, 1.000000000000000000, 0.9659258262890683122, 1.000000000000000000, 0.9659258262890683122, 1.000000000000000000, 0.9659258262890683122, 1.000000000000000000, 0.9659258262890683122, 1.000000000000000000, 0.9659258262890683122, 1.000000000000000000, 0.9659258262890683122, 1.000000000000000000, 0.9659258262890683122, 1.000000000000000000, 0.9659258262890683122, 1.000000000000000000, 0.9659258262890683122, 1.000000000000000000, 0.9659258262890683122, 1.000000000000000000, 0.9659258262890683122, 1.000000000000000000, 0.9659258262890683122, 1.000000000000000000, 0.9659258262890683122, 1.000000000000000000, 0.9659258262890683122, 1.000000000000000000, 0.9659258262890683122, 1.000000000000000000, 0.9659258262890683122, 1.000000000000000000, 0.9659258262890683122, 1.000000000000000000, 0.9659258262890683122, 1.000000000000000000, 0.9659258262890683122, 1.000000000000000000, 0.9659258262890683122, 1.000000000000000000, 0.9659258262890683122, 1.000000000000000000, 0.9659258262890683122, 1.000000000000000000, 0.9659258262890683122, 1.000000000000000000, 0.9659258262890683122, 1.000000000000000000, 0.9659258262890683122, 1.000000000000000000, 0.9659258262890683122, 1.000000000000000000, 0.9659258262890683122, 1.000000000000000000, 0.9659258262890683122, 1.000000000000000000, 0.9659258262890683122, 1.000000000000000000, 0.9659258262890683122, 1.000000000000000000, 0.9659258262890683122, 1.000000000000000000, 0.9659258262890683122, 1.000000000000000000, 0.9659258262890683122, 1.000000000000000000, 0.9659258262890683122, 1.000000000000000000, 0.9659258262890683122, 1.000000000000000000, 0.9659258262890683122, 1.000000000000000000, 0.9659258262890683122, 1.000000000000000000, 0.9947834986831260995, 0.9911642120907998565 ) ) 
 REPRESENTATION_ITEM ( '' )  );
#59732=CARTESIAN_POINT ( 'NONE',  ( 0.1049643490035304938, -0.3917322834645669549, -2.217191601049868677 ) ) ;
#59738=CARTESIAN_POINT ( 'NONE',  ( 0.4091458600556404646, -0.2362204724409448231, -1.756561679790026309 ) ) ;
#59741=CARTESIAN_POINT ( 'NONE',  ( -0.3949938075777411073, 0.1058382717557497660, -1.211942257217847763 ) ) ;
#59751=CARTESIAN_POINT ( 'NONE',  ( 0.2925321140481932369, 0.2925321140481932369, -2.576771653543307394 ) ) ;
#59752=CARTESIAN_POINT ( 'NONE',  ( 0.3392501089628018329, -0.1958661417322834497, -2.074783833824459744 ) ) ;
#59765=CARTESIAN_POINT ( 'NONE',  ( -0.3460692066303957537, -0.1998031496062994405, -0.4442257217847768724 ) ) ;
#59767=CARTESIAN_POINT ( 'NONE',  ( -9.594673741351313045E-17, 0.3917322834645670104, -1.501968503937008093 ) ) ;
#59777=CARTESIAN_POINT ( 'NONE',  ( -0.1070741851644051862, -0.3996062992125986590, -0.7788713910761155823 ) ) ;
#59789=CARTESIAN_POINT ( 'NONE',  ( -0.2867679344610366554, 0.2867679344610365444, -2.688976377952755570 ) ) ;
#59793=CARTESIAN_POINT ( 'NONE',  ( 0.3460692066303959757, -0.1998031496062991907, -0.5774278215223097588 ) ) ;
#59794=ORIENTED_EDGE ( 'NONE', *, *, #21401, .T. ) ;
#59796=CARTESIAN_POINT ( 'NONE',  ( 0.3917322834645670104, 2.398668435337828261E-17, -2.157480314960630086 ) ) ;
#59803=CARTESIAN_POINT ( 'NONE',  ( -0.4724409448818898682, -8.678599364036362592E-17, -2.005905511811023612 ) ) ;
#59807=CARTESIAN_POINT ( 'NONE',  ( 0.2867679344610365999, -0.2867679344610365999, -1.438300894191914425 ) ) ;
#59813=CARTESIAN_POINT ( 'NONE',  ( 4.797336870675656522E-17, -0.3917322834645670659, -2.910124302658479767 ) ) ;
#59822=CARTESIAN_POINT ( 'NONE',  ( -0.3917322834645671215, 0.1049643490035301469, -1.849737532808399143 ) ) ;
#59827=DIRECTION ( 'NONE',  ( 0.000000000000000000, 0.000000000000000000, 1.000000000000000000 ) ) ;
#59831=DIRECTION ( 'NONE',  ( 0.000000000000000000, 0.000000000000000000, 1.000000000000000000 ) ) ;
#59833=CARTESIAN_POINT ( 'NONE',  ( -0.3996062992125986035, -0.1070741851644056997, -1.935695538057742526 ) ) ;
#59835=EDGE_CURVE ( 'NONE', #56483, #14101, #5278, .T. ) ;
#59839=CARTESIAN_POINT ( 'NONE',  ( 0.1265901696524989462, 0.4724409448818897572, -0.7001312335958002064 ) ) ;
#59843=CARTESIAN_POINT ( 'NONE',  ( -0.3949938075777411073, 0.1058382717557497660, -0.1095800524934383707 ) ) ;
#59848=CARTESIAN_POINT ( 'NONE',  ( 0.1974969037888704704, 0.3420746716998660508, -0.3786089238845145033 ) ) ;
#59855=CARTESIAN_POINT ( 'NONE',  ( 4.893765752498283308E-17, -0.3996062992125985480, -1.257874015748031482 ) ) ;
#59858=CARTESIAN_POINT ( 'NONE',  ( 0.1958661417322836440, -0.3392501089628017219, -0.8713910761154854967 ) ) ;
#59859=CARTESIAN_POINT ( 'NONE',  ( -0.2362204724409447953, -0.4091458600556404646, -0.4573490813648293796 ) ) ;
#59871=CARTESIAN_POINT ( 'NONE',  ( 5.785732909357575061E-17, -0.4724409448818898682, -2.832677165354331006 ) ) ;
#59887=CARTESIAN_POINT ( 'NONE',  ( 0.2925321140481932369, 0.2925321140481932369, -0.6102362204724408601 ) ) ;
#59893=CARTESIAN_POINT ( 'NONE',  ( 0.1998031496062994405, -0.3460692066303958092, -2.454068241469816058 ) ) ;
#59894=CARTESIAN_POINT ( 'NONE',  ( -0.3420746716998661618, 0.1974969037888702206, -2.388451443569553856 ) ) ;
#59896=CARTESIAN_POINT ( 'NONE',  ( -0.3392501089628019995, 0.1958661417322832277, -1.120734908136482799 ) ) ;
#59899=CARTESIAN_POINT ( 'NONE',  ( 0.1049643490035304938, -0.3917322834645669549, -1.022309711286088829 ) ) ;
#59901=CARTESIAN_POINT ( 'NONE',  ( 0.1974969037888706092, -0.3420746716998660508, -2.845800524934383624 ) ) ;
#59908=CARTESIAN_POINT ( 'NONE',  ( 0.1998031496062992740, 0.3460692066303959757, -2.506561679790026087 ) ) ;
#59909=CARTESIAN_POINT ( 'NONE',  ( 0.1049643490035304799, -0.3917322834645670104, -1.341882832842206774 ) ) ;
#59915=CARTESIAN_POINT ( 'NONE',  ( -0.1049643490035307020, 0.3917322834645669549, -0.5636482939632546652 ) ) ;
#59923=DIRECTION ( 'NONE',  ( 0.000000000000000000, 0.000000000000000000, 1.000000000000000000 ) ) ;
#59924=CARTESIAN_POINT ( 'NONE',  ( -9.594673741351313045E-17, 0.3917322834645670104, -2.039370078740157410 ) ) ;
#59926=CARTESIAN_POINT ( 'NONE',  ( 0.3996062992125986035, 2.446882876249141962E-17, -0.2755905511811024278 ) ) ;
#59930=AXIS2_PLACEMENT_3D ( 'NONE', #43556, #54540, #73928 ) ;
#59934=CARTESIAN_POINT ( 'NONE',  ( 0.3983403474834781299, 0.03178304480585100733, -1.929133858267716661 ) ) ;
#59935=CARTESIAN_POINT ( 'NONE',  ( 0.3392501089628018329, 0.1958661417322835607, -1.160761154855643129 ) ) ;
#59936=CARTESIAN_POINT ( 'NONE',  ( -0.3948464311378463432, -0.01987007963522063533, -1.929133858267717994 ) ) ;
#59944=CARTESIAN_POINT ( 'NONE',  ( 0.1070741851644054637, -0.3996062992125984925, -2.051837270341207109 ) ) ;
#59955=CARTESIAN_POINT ( 'NONE',  ( -0.1049643490035306742, 0.3917322834645668994, -1.346437377131546764 ) ) ;
#59958=CARTESIAN_POINT ( 'NONE',  ( 0.3392501089628018884, -0.1958661417322834220, -1.134514435695538115 ) ) ;
#59964=CARTESIAN_POINT ( 'NONE',  ( 0.1049643490035303967, 0.3917322834645670659, 0.009823203903200209905 ) ) ;
#59967=CARTESIAN_POINT ( 'NONE',  ( -0.1265901696524993347, 0.4724409448818895907, -1.658136482939632117 ) ) ;
#59984=CARTESIAN_POINT ( 'NONE',  ( -0.2891555358219909388, -0.2891555358219912164, 0.1791338582677165503 ) ) ;
#59990=CARTESIAN_POINT ( 'NONE',  ( -9.787531504996566615E-17, 0.3996062992125985480, -1.651574803149606474 ) ) ;
#59997=CARTESIAN_POINT ( 'NONE',  ( 0.1998031496062994128, -0.3460692066303957537, -0.9560367454068241511 ) ) ;
#59998=CARTESIAN_POINT ( 'NONE',  ( 0.2925321140481932369, 0.2925321140481932369, -1.240157480314960647 ) ) ;
#59999=CARTESIAN_POINT ( 'NONE',  ( -0.2891555358219908833, -0.2891555358219912164, -0.5314960629921261503 ) ) ;
#60001=CARTESIAN_POINT ( 'NONE',  ( -0.1958661417322836718, 0.3392501089628017219, -0.005249343832020950465 ) ) ;
#60005=CARTESIAN_POINT ( 'NONE',  ( 0.1974969037888704704, 0.3420746716998660508, -1.638451443569553634 ) ) ;
#60009=CARTESIAN_POINT ( 'NONE',  ( 0.3458507752293908943, -0.3458507752293908943, -2.145669291338581974 ) ) ;
#60010=CARTESIAN_POINT ( 'NONE',  ( 0.3857315817373125899, -0.06912221444358807032, -2.755905511811024056 ) ) ;
#60013=ORIENTED_EDGE ( 'NONE', *, *, #38729, .T. ) ;
#60018=CARTESIAN_POINT ( 'NONE',  ( 0.1958661417322834497, 0.3392501089628018329, -2.586594857446507412 ) ) ;
#60025=CARTESIAN_POINT ( 'NONE',  ( 0.1958661417322834497, 0.3392501089628018329, -2.744075172407137497 ) ) ;
#60027=CARTESIAN_POINT ( 'NONE',  ( -0.1049643490035307020, 0.3917322834645669549, -1.730971128608923992 ) ) ;
#60029=ORIENTED_EDGE ( 'NONE', *, *, #46673, .T. ) ;
#60030=CARTESIAN_POINT ( 'NONE',  ( -0.1058382717557503211, 0.3949938075777409408, -2.211286089238845065 ) ) ;
#60035=CARTESIAN_POINT ( 'NONE',  ( 0.3996062992125986590, -0.1070741851644053111, -0.5839895013123358458 ) ) ;
#60039=CARTESIAN_POINT ( 'NONE',  ( -8.478666411000228475E-17, -0.3992723400743185547, -2.755905511811022723 ) ) ;
#60040=CARTESIAN_POINT ( 'NONE',  ( 0.2867679344610365999, -0.2867679344610365444, 0.1318897637795274913 ) ) ;
#60046=CARTESIAN_POINT ( 'NONE',  ( 0.3917322834645670104, -0.1049643490035303411, 0.05380577427821527092 ) ) ;
#60051=CARTESIAN_POINT ( 'NONE',  ( 0.2362204724409451007, -0.4091458600556402980, -1.194225721784776928 ) ) ;
#60053=CARTESIAN_POINT ( 'NONE',  ( -0.1049643490035302024, -0.3917322834645671215, -0.6942257217847765949 ) ) ;
#60054=VECTOR ( 'NONE', #80491, 39.37007874015748143 ) ;
#60055=CARTESIAN_POINT ( 'NONE',  ( -9.594673741351313045E-17, 0.3917322834645670104, -2.289370078740157410 ) ) ;
#60060=CARTESIAN_POINT ( 'NONE',  ( 0.3996062992125985480, 2.446882876249141654E-17, -0.03740157480314963701 ) ) ;
#60065=CARTESIAN_POINT ( 'NONE',  ( -0.1958661417322836440, 0.3392501089628016664, 0.2218040926847262562 ) ) ;
#60072=CARTESIAN_POINT ( 'NONE',  ( -0.3917322834645669549, -0.1049643490035306603, -2.085301837270341352 ) ) ;
#60076=CARTESIAN_POINT ( 'NONE',  ( 0.4091458600556404646, -0.2362204724409448231, -0.4967191601049869010 ) ) ;
#60089=ORIENTED_EDGE ( 'NONE', *, *, #59835, .F. ) ;
#60090=CARTESIAN_POINT ( 'NONE',  ( -0.1070741851644051862, -0.3996062992125986590, -1.408792650918635259 ) ) ;
#60100=CARTESIAN_POINT ( 'NONE',  ( 0.3996062992125986035, 0.1070741851644054776, -0.2821522309711286258 ) ) ;
#60101=CARTESIAN_POINT ( 'NONE',  ( 0.1958661417322834775, 0.3392501089628018884, -2.660780470637482242 ) ) ;
#60107=CARTESIAN_POINT ( 'NONE',  ( 0.3917322834645669549, 0.1049643490035304660, -2.414041994750655729 ) ) ;
#60112=VECTOR ( 'NONE', #19789, 39.37007874015748143 ) ;
#60117=CARTESIAN_POINT ( 'NONE',  ( -9.594673741351313045E-17, 0.3917322834645670659, -0.4691794207687158269 ) ) ;
#60130=CARTESIAN_POINT ( 'NONE',  ( -0.1049643490035302024, -0.3917322834645671215, -0.5367454068241469534 ) ) ;
#60133=CARTESIAN_POINT ( 'NONE',  ( 0.1058382717557499880, 0.3949938075777411073, -1.095800524934383180 ) ) ;
#60134=VERTEX_POINT ( 'NONE', #37560 ) ;
#60149=CARTESIAN_POINT ( 'NONE',  ( -9.787531504996567848E-17, 0.3996062992125986035, -1.732283464566929165 ) ) ;
#60151=CARTESIAN_POINT ( 'NONE',  ( -0.1070741851644051862, -0.3996062992125986590, -1.093832020997375087 ) ) ;
#60152=CARTESIAN_POINT ( 'NONE',  ( 0.1070741851644054776, -0.3996062992125984925, -0.4770341207349080848 ) ) ;
#60154=CARTESIAN_POINT ( 'NONE',  ( 0.2925321140481932369, -0.2925321140481932369, -2.933070866141732402 ) ) ;
#60155=CARTESIAN_POINT ( 'NONE',  ( -0.3917322834645671215, 0.1049643490035301469, -2.322178477690288734 ) ) ;
#60161=CARTESIAN_POINT ( 'NONE',  ( -1.157146581871515012E-16, 0.4724409448818898682, -2.124015748031495843 ) ) ;
#60164=CARTESIAN_POINT ( 'NONE',  ( -0.2891555358219909388, -0.2891555358219912164, -2.025590551181102761 ) ) ;
#60172=CARTESIAN_POINT ( 'NONE',  ( -0.2925321140481932369, 0.2925321140481931259, -2.458661417322834719 ) ) ;
#60175=CARTESIAN_POINT ( 'NONE',  ( 0.3917322834645668994, -0.1049643490035303134, -2.238825828575116805 ) ) ;
#60189=CARTESIAN_POINT ( 'NONE',  ( -0.3996062992125986590, 0.1070741851644051723, -0.4245406824146981672 ) ) ;
#60191=CARTESIAN_POINT ( 'NONE',  ( -0.2867679344610365999, 0.2867679344610364889, -1.836614173228346747 ) ) ;
#60200=CARTESIAN_POINT ( 'NONE',  ( -0.3996062992125984925, -0.1070741851644056858, -0.7526246719160103460 ) ) ;
#60207=CARTESIAN_POINT ( 'NONE',  ( 0.3996062992125986035, 2.446882876249141962E-17, -1.220472440944881942 ) ) ;
#60209=CARTESIAN_POINT ( 'NONE',  ( -0.4724409448818914226, -0.1265901696524962816, -2.093175853018372834 ) ) ;
#60216=CARTESIAN_POINT ( 'NONE',  ( -0.3996062992125986035, -7.340648628747425578E-17, -0.3543307086614173040 ) ) ;
#60219=CARTESIAN_POINT ( 'NONE',  ( 4.797336870675656522E-17, -0.3917322834645670104, -2.118110236220472675 ) ) ;
#60226=CARTESIAN_POINT ( 'NONE',  ( -0.3458507752293906723, -0.3458507752293910609, -2.025590551181101873 ) ) ;
#60230=CARTESIAN_POINT ( 'NONE',  ( -0.1958661417322836440, 0.3392501089628016664, -1.510479371882202937 ) ) ;
#60234=( BOUNDED_CURVE ( )  B_SPLINE_CURVE ( 2, ( #6091, #19133, #57011, #58681, #57427, #622, #71321, #45208, #82707, #78062, #77644, #204, #51105 ),
 .UNSPECIFIED., .F., .F. ) 
 B_SPLINE_CURVE_WITH_KNOTS ( ( 3, 2, 2, 2, 2, 2, 3 ),
 ( 0.8375000000000000222, 0.8416666666666666741, 0.8458333333333333259, 0.8499999999999999778, 0.8541666666666666297, 0.8583333333333332815, 0.8625000000000000444 ),
 .UNSPECIFIED. ) 
 CURVE ( )  GEOMETRIC_REPRESENTATION_ITEM ( )  RATIONAL_B_SPLINE_CURVE ( ( 1.000000000000000000, 0.9659258262890683122, 1.000000000000000000, 0.9659258262890683122, 1.000000000000000000, 0.9659258262890683122, 1.000000000000000000, 0.9659258262890683122, 1.000000000000000000, 0.9659258262890683122, 1.000000000000000000, 0.9659258262890683122, 1.000000000000000000 ) ) 
 REPRESENTATION_ITEM ( '' )  );
#60238=CARTESIAN_POINT ( 'NONE',  ( 0.1958661417322836718, -0.3392501089628017219, -2.923247662238532385 ) ) ;
#60248=CARTESIAN_POINT ( 'NONE',  ( -0.3392501089628019995, 0.1958661417322832277, -2.158136482939632561 ) ) ;
#60253=CARTESIAN_POINT ( 'NONE',  ( 0.3917322834645670104, 2.398668435337828261E-17, -2.944881889763779181 ) ) ;
#60257=CARTESIAN_POINT ( 'NONE',  ( -0.1998031496062991907, -0.3460692066303959757, -1.955380577427821454 ) ) ;
#60263=CARTESIAN_POINT ( 'NONE',  ( 0.3458507752293908943, 0.3458507752293908943, -0.8444881889763780070 ) ) ;
#60266=CARTESIAN_POINT ( 'NONE',  ( 0.3420746716998660508, 0.1974969037888705814, -0.5229658792650918597 ) ) ;
#60271=CARTESIAN_POINT ( 'NONE',  ( -0.3949938075777411073, 0.1058382717557497660, -0.4245406824146981672 ) ) ;
#60278=CARTESIAN_POINT ( 'NONE',  ( 0.3996062992125984925, 0.1070741851644054637, -1.146325459317585116 ) ) ;
#60280=CARTESIAN_POINT ( 'NONE',  ( -0.3392501089628017219, -0.1958661417322836718, -0.9895013123359579499 ) ) ;
#60281=CARTESIAN_POINT ( 'NONE',  ( -0.4724409448818891466, -0.1265901696525000564, -0.4376640419947506744 ) ) ;
#60282=CARTESIAN_POINT ( 'NONE',  ( -0.3788256970788715927, 0.1002886991238273323, -1.587495037872346049E-17 ) ) ;
#60290=CARTESIAN_POINT ( 'NONE',  ( 0.2362204724409449064, 0.4091458600556404646, -0.2211286089238845010 ) ) ;
#60292=CARTESIAN_POINT ( 'NONE',  ( -0.1998031496062991630, -0.3460692066303959202, 0.1725721784776902690 ) ) ;
#60310=CARTESIAN_POINT ( 'NONE',  ( 0.1070741851644054915, -0.3996062992125985480, -0.8727034120734907807 ) ) ;
#60314=CARTESIAN_POINT ( 'NONE',  ( -0.3460692066303960868, 0.1998031496062990242, -2.860892388451443669 ) ) ;
#60315=CARTESIAN_POINT ( 'NONE',  ( 0.1974969037888704704, 0.3420746716998660508, -2.349081364829396446 ) ) ;
#60318=CARTESIAN_POINT ( 'NONE',  ( 0.3917322834645670104, -0.1049643490035303411, -0.8910761154855640909 ) ) ;
#60324=CARTESIAN_POINT ( 'NONE',  ( -0.1958661417322834497, -0.3392501089628018884, -0.4606106054780034764 ) ) ;
#60332=CARTESIAN_POINT ( 'NONE',  ( -0.3392501089628017219, -0.1958661417322836995, -1.466554748852705092 ) ) ;
#60338=CARTESIAN_POINT ( 'NONE',  ( 0.2867679344610365999, 0.2867679344610365999, -0.3799212598425197318 ) ) ;
#60348=CARTESIAN_POINT ( 'NONE',  ( -0.1049643490035302024, -0.3917322834645671215, -2.426509186351705427 ) ) ;
#60350=ORIENTED_EDGE ( 'NONE', *, *, #8023, .F. ) ;
#60356=CARTESIAN_POINT ( 'NONE',  ( -0.3392501089628017219, -0.1958661417322836718, -1.082020997375328086 ) ) ;
#60357=CARTESIAN_POINT ( 'NONE',  ( 0.3996062992125986035, -0.1070741851644052972, -1.920603674540682038 ) ) ;
#60365=CARTESIAN_POINT ( 'NONE',  ( 0.3996062992125985480, 2.446882876249141654E-17, -2.084645669291338876 ) ) ;
#60367=CARTESIAN_POINT ( 'NONE',  ( 0.3917322834645669549, 0.1049643490035304660, 0.04068241469816277767 ) ) ;
#60374=CARTESIAN_POINT ( 'NONE',  ( -0.1958661417322834497, -0.3392501089628018884, -1.090531865320523153 ) ) ;
#60383=CARTESIAN_POINT ( 'NONE',  ( 0.3917322834645670659, 2.398668435337828261E-17, -0.1148487121072984812 ) ) ;
#60386=CARTESIAN_POINT ( 'NONE',  ( 0.4724409448818897572, -0.1265901696524988906, -1.605643044619422977 ) ) ;
#60396=CARTESIAN_POINT ( 'NONE',  ( 0.4724409448818898682, 0.000000000000000000, -2.755905511811024056 ) ) ;
#60403=CARTESIAN_POINT ( 'NONE',  ( -0.3996062992125985480, -7.340648628747423112E-17, -2.635826771653543066 ) ) ;
#60408=CARTESIAN_POINT ( 'NONE',  ( -0.3460692066303957537, -0.1998031496062994405, -2.019028871391076230 ) ) ;
#60414=CARTESIAN_POINT ( 'NONE',  ( 4.893765752498283924E-17, -0.3996062992125986035, -1.968503937007873850 ) ) ;
#60415=CARTESIAN_POINT ( 'NONE',  ( -0.3420746716998659953, -0.1974969037888706647, -0.9973753280839895430 ) ) ;
#60416=CARTESIAN_POINT ( 'NONE',  ( -0.3996062992125986035, -7.340648628747425578E-17, -2.401574803149606474 ) ) ;
#60418=CARTESIAN_POINT ( 'NONE',  ( -0.3917322834645669549, -0.1049643490035306603, -0.1955380577427821009 ) ) ;
#60422=CARTESIAN_POINT ( 'NONE',  ( -9.674558042662122972E-17, 0.3949938075777409963, -2.124015748031495843 ) ) ;
#60426=CARTESIAN_POINT ( 'NONE',  ( -0.4724409448818895907, -0.1265901696524993070, -2.093175853018372834 ) ) ;
#60427=CARTESIAN_POINT ( 'NONE',  ( 0.1716039559346060062, 0.3527845929029486682, -2.755905511811024056 ) ) ;
#60428=EDGE_LOOP ( 'NONE', ( #16465, #75576, #1653, #75651, #48404, #60089, #21320, #40446, #75237, #81119, #35774, #73627, #18378, #24070, #45217, #19449, #62152, #75766, #63237, #77000 ) ) ;
#60434=CARTESIAN_POINT ( 'NONE',  ( 0.1958661417322836162, -0.3392501089628018329, -2.219140789205037656 ) ) ;
#60441=CARTESIAN_POINT ( 'NONE',  ( -0.1049643490035307020, 0.3917322834645669549, 0.2237532808398949025 ) ) ;
#60443=CARTESIAN_POINT ( 'NONE',  ( -0.1049643490035302024, -0.3917322834645671215, -1.796587926509185973 ) ) ;
#60446=CARTESIAN_POINT ( 'NONE',  ( 0.3949938075777411073, -0.1058382717557499464, -2.473753280839894764 ) ) ;
#60450=CARTESIAN_POINT ( 'NONE',  ( 0.1070741851644054915, -0.3996062992125986035, -0.5577427821522309426 ) ) ;
#60454=CARTESIAN_POINT ( 'NONE',  ( 0.0003067303408410983591, -0.3990339831394564274, -2.755905511811023612 ) ) ;
#60456=CARTESIAN_POINT ( 'NONE',  ( 0.1958661417322836440, -0.3392501089628017219, -0.1765091863517061210 ) ) ;
#60460=EDGE_CURVE ( 'NONE', #23246, #6583, #40484, .T. ) ;
#60467=CARTESIAN_POINT ( 'NONE',  ( -0.4091458600556405756, 0.2362204724409446288, -1.128608923884514503 ) ) ;
#60469=CARTESIAN_POINT ( 'NONE',  ( 0.3392501089628018329, 0.1958661417322835607, -0.7532808398950130435 ) ) ;
#60470=CARTESIAN_POINT ( 'NONE',  ( -0.1958661417322834220, -0.3392501089628018884, -2.512467191601049699 ) ) ;
#60473=CARTESIAN_POINT ( 'NONE',  ( 4.893765752498283308E-17, -0.3996062992125985480, 0.001968503937007844932 ) ) ;
#60478=CARTESIAN_POINT ( 'NONE',  ( -0.3392501089628019439, 0.1958661417322832554, -0.1062798968165861030 ) ) ;
#60480=CARTESIAN_POINT ( 'NONE',  ( -0.3917322834645669549, -0.1049643490035306603, -0.2880577427821522929 ) ) ;
#60486=CARTESIAN_POINT ( 'NONE',  ( 4.797336870675656522E-17, -0.3917322834645670104, -1.960629921259842368 ) ) ;
#60490=CARTESIAN_POINT ( 'NONE',  ( -1.157146581871515012E-16, 0.4724409448818898682, -0.2342519685039370358 ) ) ;
#60499=CARTESIAN_POINT ( 'NONE',  ( -1.157146581871515012E-16, 0.4724409448818898682, -1.966535433070865979 ) ) ;
#60503=CARTESIAN_POINT ( 'NONE',  ( -0.3996062992125984925, -0.1070741851644056858, -1.697506561679789971 ) ) ;
#60512=DIRECTION ( 'NONE',  ( 0.000000000000000000, 0.000000000000000000, 1.000000000000000000 ) ) ;
#60513=CARTESIAN_POINT ( 'NONE',  ( -0.1998031496062991907, -0.3460692066303959757, -0.2230971128608923715 ) ) ;
#60514=CARTESIAN_POINT ( 'NONE',  ( -0.2891555358219911054, 0.2891555358219909388, -0.01968503937007880233 ) ) ;
#60515=CARTESIAN_POINT ( 'NONE',  ( -0.05073257145186574335, -0.3893108287682404134, -1.862014699505666341E-17 ) ) ;
#60519=CARTESIAN_POINT ( 'NONE',  ( 0.1958661417322836440, -0.3392501089628017219, -2.381233595800524849 ) ) ;
#60524=CARTESIAN_POINT ( 'NONE',  ( -0.4724409448818898682, -8.678599364036362592E-17, -0.8267716535433070613 ) ) ;
#60528=CARTESIAN_POINT ( 'NONE',  ( 0.3917322834645670659, 2.398668435337828261E-17, -0.2723290270679284419 ) ) ;
#60541=CARTESIAN_POINT ( 'NONE',  ( -0.1958661417322834220, -0.3392501089628018884, -0.6876640419947506189 ) ) ;
#60544=CARTESIAN_POINT ( 'NONE',  ( -0.3949938075777409963, -7.255918531996591613E-17, -0.8267716535433070613 ) ) ;
#60545=EDGE_LOOP ( 'NONE', ( #66642, #47580, #29470, #524 ) ) ;
#60555=CARTESIAN_POINT ( 'NONE',  ( -0.4724409448818898682, -8.678599364036362592E-17, -0.4311023622047244208 ) ) ;
#60561=CARTESIAN_POINT ( 'NONE',  ( -0.1998031496062994683, 0.3460692066303958092, -1.745406824146981561 ) ) ;
#60564=CARTESIAN_POINT ( 'NONE',  ( 0.1070741851644053388, 0.3996062992125986035, -1.330052493438320216 ) ) ;
#60565=CARTESIAN_POINT ( 'NONE',  ( 4.893765752498283308E-17, -0.3996062992125985480, -0.4704724409448819422 ) ) ;
#60568=CARTESIAN_POINT ( 'NONE',  ( 0.2362204724409451007, -0.4091458600556402980, 0.06561679790026246628 ) ) ;
#60569=CARTESIAN_POINT ( 'NONE',  ( -0.3917322834645670104, -7.196005306013484475E-17, -2.643700787401574548 ) ) ;
#60575=CARTESIAN_POINT ( 'NONE',  ( 0.4091458600556403535, 0.2362204724409449896, -1.940288713910761187 ) ) ;
#60578=CARTESIAN_POINT ( 'NONE',  ( -0.1058382717557503072, 0.3949938075777408852, -1.815616797900262869 ) ) ;
#60588=CARTESIAN_POINT ( 'NONE',  ( -0.3996062992125986590, 0.1070741851644051723, -2.629265091863517423 ) ) ;
#60589=CARTESIAN_POINT ( 'NONE',  ( 0.3917322834645668994, -0.1049643490035303134, -2.553786458496376088 ) ) ;
#60602=CARTESIAN_POINT ( 'NONE',  ( 0.3996062992125986035, -0.1070741851644052972, -0.5032808398950130435 ) ) ;
#60604=CARTESIAN_POINT ( 'NONE',  ( 0.1049643490035303689, 0.3917322834645670104, -1.810367454068241511 ) ) ;
#60613=CARTESIAN_POINT ( 'NONE',  ( 0.1998031496062992463, 0.3460692066303959202, -0.8510498687664042050 ) ) ;
#60619=CARTESIAN_POINT ( 'NONE',  ( 0.3900885325447117635, 0.05060072268091646286, -1.220472440944882164 ) ) ;
#60627=CARTESIAN_POINT ( 'NONE',  ( -0.2925321140481930704, -0.2925321140481933480, -0.6889763779527556808 ) ) ;
#60630=CARTESIAN_POINT ( 'NONE',  ( -0.1958661417322834220, -0.3392501089628018884, -2.419947506561679784 ) ) ;
#60641=CARTESIAN_POINT ( 'NONE',  ( -0.2867679344610364334, -0.2867679344610368219, -1.556411130412386656 ) ) ;
#60647=CARTESIAN_POINT ( 'NONE',  ( -0.3949938075777409408, -0.1058382717557502933, 0.1115485564304461441 ) ) ;
#60657=CARTESIAN_POINT ( 'NONE',  ( -0.3917322834645669549, -0.1049643490035306603, -2.335301837270341352 ) ) ;
#60665=CARTESIAN_POINT ( 'NONE',  ( -0.2925321140481932369, 0.2925321140481931259, -0.09645669291338582196 ) ) ;
#60667=CARTESIAN_POINT ( 'NONE',  ( 0.1070741851644054915, -0.3996062992125986035, -1.660104986876640210 ) ) ;
#60672=CARTESIAN_POINT ( 'NONE',  ( -0.1265901696524986964, -0.4724409448818899238, -0.6213910761154856077 ) ) ;
#60675=CARTESIAN_POINT ( 'NONE',  ( -0.1058382717557497660, -0.3949938075777411073, -0.6213910761154856077 ) ) ;
#60680=CARTESIAN_POINT ( 'NONE',  ( 4.837279021331061486E-17, -0.3949938075777409963, -0.4704724409448818867 ) ) ;
#60687=CARTESIAN_POINT ( 'NONE',  ( -0.3996062992125984925, -0.1070741851644056858, -1.382545931758530022 ) ) ;
#60689=CARTESIAN_POINT ( 'NONE',  ( -0.3917322834645670104, -7.196005306013484475E-17, -1.133858267716535195 ) ) ;
#60691=CARTESIAN_POINT ( 'NONE',  ( -0.3622863298689263933, 0.1504864506494507925, -1.599317578742253179E-17 ) ) ;
#60718=CARTESIAN_POINT ( 'NONE',  ( -9.787531504996567848E-17, 0.3996062992125986035, -0.6299212598425196763 ) ) ;
#60722=CARTESIAN_POINT ( 'NONE',  ( -0.4091458600556405756, 0.2362204724409446288, 0.1312335958005249326 ) ) ;
#60723=CARTESIAN_POINT ( 'NONE',  ( 0.3420746716998659953, 0.1974969037888705536, -2.493438320209973469 ) ) ;
#60726=CARTESIAN_POINT ( 'NONE',  ( -0.1958661417322834220, -0.3392501089628018884, -1.160104986876640210 ) ) ;
#60733=CARTESIAN_POINT ( 'NONE',  ( -0.2867679344610364334, -0.2867679344610368219, -0.1390882957667173292 ) ) ;
#60740=CARTESIAN_POINT ( 'NONE',  ( -0.3392501089628019995, 0.1958661417322831999, -1.597788344653229720 ) ) ;
#60746=CARTESIAN_POINT ( 'NONE',  ( -0.3392501089628019995, 0.1958661417322832277, -0.8982939632545933195 ) ) ;
#60755=CARTESIAN_POINT ( 'NONE',  ( 0.4724409448818898682, 2.892866454678787531E-17, -0.3523622047244094335 ) ) ;
#60756=CARTESIAN_POINT ( 'NONE',  ( 0.3392501089628018329, 0.1958661417322835607, -2.485564304461941987 ) ) ;
#60757=ORIENTED_EDGE ( 'NONE', *, *, #5521, .T. ) ;
#60765=CARTESIAN_POINT ( 'NONE',  ( 0.2867679344610365999, 0.2867679344610365999, -1.167322834645669438 ) ) ;
#60766=CARTESIAN_POINT ( 'NONE',  ( -0.3996062992125985480, -7.340648628747423112E-17, -2.320866141732283783 ) ) ;
#60777=CARTESIAN_POINT ( 'NONE',  ( -0.2867679344610365999, 0.2867679344610364889, 0.1456692913385827237 ) ) ;
#60784=CARTESIAN_POINT ( 'NONE',  ( -0.3917322834645669549, -7.196005306013483243E-17, -1.064285146160418360 ) ) ;
#60793=CARTESIAN_POINT ( 'NONE',  ( 0.2867679344610366554, 0.2867679344610366554, -0.2920140664380071471 ) ) ;
#60795=CARTESIAN_POINT ( 'NONE',  ( 0.4091458600556403535, 0.2362204724409449896, -1.782808398950131101 ) ) ;
#60817=CARTESIAN_POINT ( 'NONE',  ( 0.3460692066303959202, -0.1998031496062991630, -2.071522309711286258 ) ) ;
#60823=CARTESIAN_POINT ( 'NONE',  ( -0.1070741851644051862, -0.3996062992125987146, -1.646981627296587591 ) ) ;
#60824=CARTESIAN_POINT ( 'NONE',  ( -0.3420746716998661618, 0.1974969037888702206, -0.9711286089238846397 ) ) ;
#60825=CARTESIAN_POINT ( 'NONE',  ( 0.1998031496062994405, -0.3460692066303958092, -2.611548556430446144 ) ) ;
#60827=CARTESIAN_POINT ( 'NONE',  ( -0.3917322834645671215, 0.1049643490035301469, -0.1824146981627296216 ) ) ;
#60831=CARTESIAN_POINT ( 'NONE',  ( -0.2891555358219909388, -0.2891555358219912164, -2.025590551181102761 ) ) ;
#60835=CARTESIAN_POINT ( 'NONE',  ( 0.3458507752293908943, -0.3458507752293908943, -2.618110236220472675 ) ) ;
#60836=CARTESIAN_POINT ( 'NONE',  ( -9.787531504996567848E-17, 0.3996062992125986035, -1.889763779527559251 ) ) ;
#60844=CARTESIAN_POINT ( 'NONE',  ( -0.1958661417322834497, -0.3392501089628018884, -2.665335014926823121 ) ) ;
#60851=CARTESIAN_POINT ( 'NONE',  ( -0.1958661417322834220, -0.3392501089628018884, -0.3077427821522311091 ) ) ;
#60853=CARTESIAN_POINT ( 'NONE',  ( 0.2867679344610365999, -0.2867679344610365444, -2.295275590551181022 ) ) ;
#60856=CARTESIAN_POINT ( 'NONE',  ( 0.2891555358219910499, 0.2891555358219910499, -2.342519685039370358 ) ) ;
#60860=CARTESIAN_POINT ( 'NONE',  ( -0.1998031496062994683, 0.3460692066303958092, -1.115485564304461885 ) ) ;
#60864=DIRECTION ( 'NONE',  ( 0.000000000000000000, 0.000000000000000000, 1.000000000000000000 ) ) ;
#60865=CARTESIAN_POINT ( 'NONE',  ( 0.3392501089628018884, -0.1958661417322834220, -0.03215223097112869521 ) ) ;
#60866=AXIS2_PLACEMENT_3D ( 'NONE', #54971, #67623, #47827 ) ;
#60876=CARTESIAN_POINT ( 'NONE',  ( 0.000000000000000000, 0.000000000000000000, 0.000000000000000000 ) ) ;
#60878=CARTESIAN_POINT ( 'NONE',  ( 0.3458507752293908943, 0.3458507752293908943, -1.870078740157480546 ) ) ;
#60881=CARTESIAN_POINT ( 'NONE',  ( 0.3917322834645670104, -0.1049643490035303411, -0.5761154855643042527 ) ) ;
#60882=CARTESIAN_POINT ( 'NONE',  ( 0.3917322834645670104, -0.1049643490035303273, -2.715879265091862838 ) ) ;
#60885=CARTESIAN_POINT ( 'NONE',  ( 0.2925321140481932369, 0.2925321140481932369, -0.6870078740157479213 ) ) ;
#60890=CARTESIAN_POINT ( 'NONE',  ( -0.1049643490035306742, 0.3917322834645668994, -0.08659485744650738392 ) ) ;
#60892=CARTESIAN_POINT ( 'NONE',  ( -0.2867679344610366554, 0.2867679344610365444, -0.2618110236220473341 ) ) ;
#60897=CARTESIAN_POINT ( 'NONE',  ( 0.3917322834645669549, 0.1049643490035304660, -2.321522309711285814 ) ) ;
#60901=CARTESIAN_POINT ( 'NONE',  ( 5.785732909357575061E-17, -0.4724409448818898682, -0.3129921259842520231 ) ) ;
#60902=ADVANCED_FACE ( 'NONE', ( #79635 ), #11192, .T. ) ;
#60912=CARTESIAN_POINT ( 'NONE',  ( -0.3460692066303960313, 0.1998031496062989965, -1.362860892388451539 ) ) ;
#60921=CARTESIAN_POINT ( 'NONE',  ( 0.1998031496062992463, 0.3460692066303959202, -0.2211286089238845565 ) ) ;
#60922=CARTESIAN_POINT ( 'NONE',  ( -0.1070741851644051862, -0.3996062992125987146, -0.5446194225721783244 ) ) ;
#60924=CARTESIAN_POINT ( 'NONE',  ( -0.1049643490035307158, 0.3917322834645670104, -2.837945824968191477 ) ) ;
#60929=CARTESIAN_POINT ( 'NONE',  ( -0.3949938075777411073, 0.1058382717557497660, -0.7395013123359579499 ) ) ;
#60934=CARTESIAN_POINT ( 'NONE',  ( 0.3458507752293908943, 0.3458507752293908943, -0.6102362204724409711 ) ) ;
#60935=CARTESIAN_POINT ( 'NONE',  ( 0.1070741851644054915, -0.3996062992125985480, -2.132545931758530244 ) ) ;
#60938=CARTESIAN_POINT ( 'NONE',  ( 0.3392501089628018884, -0.1958661417322833942, -0.2592056674878758793 ) ) ;
#60950=CARTESIAN_POINT ( 'NONE',  ( -0.1958661417322834220, -0.3392501089628018884, -0.5301837270341206443 ) ) ;
#60953=CARTESIAN_POINT ( 'NONE',  ( -9.674558042662121740E-17, 0.3949938075777409963, -1.102362204724409711 ) ) ;
#60957=CARTESIAN_POINT ( 'NONE',  ( 0.3996062992125986035, 0.1070741851644054776, 0.03280839895013121926 ) ) ;
#60963=CARTESIAN_POINT ( 'NONE',  ( -0.3458507752293906723, -0.3458507752293910609, -1.003937007874015741 ) ) ;
#60969=CARTESIAN_POINT ( 'NONE',  ( -0.3460692066303958092, -0.1998031496062994683, -1.627296587926509330 ) ) ;
#60970=CARTESIAN_POINT ( 'NONE',  ( 0.1208384647389237204, -0.3726288332213487653, -2.755905511811024056 ) ) ;
#60972=CARTESIAN_POINT ( 'NONE',  ( 0.1998031496062994128, -0.3460692066303957537, -0.9560367454068241511 ) ) ;
#60973=CARTESIAN_POINT ( 'NONE',  ( -9.787531504996566615E-17, 0.3996062992125985480, -0.3917322834645669549 ) ) ;
#60976=CARTESIAN_POINT ( 'NONE',  ( -0.4724409448818895907, -0.1265901696524993070, 0.1115485564304461719 ) ) ;
#60978=CARTESIAN_POINT ( 'NONE',  ( -0.1049643490035302024, -0.3917322834645671215, -2.361548556430446144 ) ) ;
#60984=CARTESIAN_POINT ( 'NONE',  ( -0.4724409448818899238, 0.1265901696524986686, -1.999343832020997525 ) ) ;
#60987=VECTOR ( 'NONE', #64786, 39.37007874015748143 ) ;
#60988=CARTESIAN_POINT ( 'NONE',  ( -0.3420746716998660508, -0.1974969037888706924, -1.704068241469815836 ) ) ;
#60999=CARTESIAN_POINT ( 'NONE',  ( -0.3917322834645670659, 0.1049643490035301607, -2.632526615976691353 ) ) ;
#61011=CARTESIAN_POINT ( 'NONE',  ( 0.1998031496062992463, 0.3460692066303959202, -0.2211286089238845010 ) ) ;
#61013=CARTESIAN_POINT ( 'NONE',  ( -0.1049643490035302024, -0.3917322834645671215, -1.889107611548556109 ) ) ;
#61023=CARTESIAN_POINT ( 'NONE',  ( 0.3996062992125984925, 0.1070741851644054637, -0.8313648293963252778 ) ) ;
#61025=CARTESIAN_POINT ( 'NONE',  ( -0.4724409448818898682, -8.678599364036362592E-17, -2.635826771653543066 ) ) ;
#61033=CARTESIAN_POINT ( 'NONE',  ( -0.1958661417322836718, 0.3392501089628017219, -1.672572178477690352 ) ) ;
#61034=CARTESIAN_POINT ( 'NONE',  ( 0.2881610400590569054, 0.2661962643026990483, -1.220472440944881942 ) ) ;
#61040=CARTESIAN_POINT ( 'NONE',  ( 0.3460692066303959202, 0.1998031496062993295, -0.4461942257217847430 ) ) ;
#61044=CARTESIAN_POINT ( 'NONE',  ( 0.3917322834645669549, 0.1049643490035304660, -2.164041994750655729 ) ) ;
#61054=CARTESIAN_POINT ( 'NONE',  ( 0.3392501089628018329, -0.1958661417322834497, -1.602342888942570154 ) ) ;
#61060=CARTESIAN_POINT ( 'NONE',  ( 0.1958661417322836718, -0.3392501089628017219, -2.765767347277902299 ) ) ;
#61068=CARTESIAN_POINT ( 'NONE',  ( 0.1049643490035303967, 0.3917322834645670659, -1.092539000821209250 ) ) ;
#61070=CARTESIAN_POINT ( 'NONE',  ( 0.1049643490035304938, -0.3917322834645669549, -2.374671916010498762 ) ) ;
#61077=CARTESIAN_POINT ( 'NONE',  ( -9.787531504996566615E-17, 0.3996062992125985480, 0.08070866141732283006 ) ) ;
#61079=CARTESIAN_POINT ( 'NONE',  ( -0.1998031496062991907, -0.3460692066303959757, -1.797900262467191590 ) ) ;
#61084=CARTESIAN_POINT ( 'NONE',  ( 5.785732909357575061E-17, -0.4724409448818898682, -0.4704724409448819422 ) ) ;
#61087=CARTESIAN_POINT ( 'NONE',  ( -0.3949938075777411073, 0.1058382717557497660, -0.5820209973753280863 ) ) ;
#61092=CARTESIAN_POINT ( 'NONE',  ( -0.3949938075777408852, -0.1058382717557502933, -0.2801837270341207553 ) ) ;
#61099=CARTESIAN_POINT ( 'NONE',  ( 0.1070741851644054776, -0.3996062992125984925, -1.264435695538057569 ) ) ;
#61101=CARTESIAN_POINT ( 'NONE',  ( 0.3392501089628018884, -0.1958661417322834220, -1.041994750656167756 ) ) ;
#61112=LINE ( 'NONE', #41351, #14189 ) ;
#61133=CARTESIAN_POINT ( 'NONE',  ( 0.3996062992125986035, 2.446882876249141962E-17, -2.952755905511811108 ) ) ;
#61134=CARTESIAN_POINT ( 'NONE',  ( -0.1974969037888706647, 0.3420746716998658843, -2.532808398950130879 ) ) ;
#61137=CARTESIAN_POINT ( 'NONE',  ( 0.3392501089628018329, 0.1958661417322835607, -0.9107611548556429071 ) ) ;
#61139=CARTESIAN_POINT ( 'NONE',  ( 0.3458507752293908943, 0.3458507752293908943, -2.500000000000000444 ) ) ;
#61145=CARTESIAN_POINT ( 'NONE',  ( -0.3392501089628019439, 0.1958661417322832554, -0.1062798968165861030 ) ) ;
#61151=CARTESIAN_POINT ( 'NONE',  ( -0.4091458600556405756, 0.2362204724409446288, -1.128608923884514503 ) ) ;
#61152=CARTESIAN_POINT ( 'NONE',  ( -0.3392501089628017219, -0.1958661417322836995, -1.781515378773965042 ) ) ;
#61159=CARTESIAN_POINT ( 'NONE',  ( 0.3917322834645670104, -0.1049643490035303411, -0.8261154855643043637 ) ) ;
#61167=CARTESIAN_POINT ( 'NONE',  ( -0.4091458600556402980, -0.2362204724409451284, -0.9166666666666666297 ) ) ;
#61168=CARTESIAN_POINT ( 'NONE',  ( 0.1958661417322834775, 0.3392501089628018884, -2.341207349081364963 ) ) ;
#61174=CARTESIAN_POINT ( 'NONE',  ( 0.4724409448818898682, 2.892866454678787531E-17, -2.165354330708661568 ) ) ;
#61175=CARTESIAN_POINT ( 'NONE',  ( -0.3917322834645671215, 0.1049643490035301469, -0.5898950131233595684 ) ) ;
#61178=CARTESIAN_POINT ( 'NONE',  ( 0.3392501089628018329, 0.1958661417322835607, -1.475721784776902856 ) ) ;
#61179=CARTESIAN_POINT ( 'NONE',  ( 0.2925321140481932369, 0.2925321140481932369, -2.576771653543307394 ) ) ;
#61187=CARTESIAN_POINT ( 'NONE',  ( -0.3996062992125984925, -0.1070741851644056719, -2.169947506561679784 ) ) ;
#61189=CARTESIAN_POINT ( 'NONE',  ( -0.1958661417322834220, -0.3392501089628018884, 0.09973753280839897650 ) ) ;
#61196=CARTESIAN_POINT ( 'NONE',  ( 4.797336870675655290E-17, -0.3917322834645669549, -1.418615854821835276 ) ) ;
#61204=CARTESIAN_POINT ( 'NONE',  ( -0.3917322834645670659, -7.196005306013484475E-17, -0.6660298144695031564 ) ) ;
#61208=CARTESIAN_POINT ( 'NONE',  ( 0.4091458600556403535, 0.2362204724409449896, -1.940288713910761187 ) ) ;
#61231=CARTESIAN_POINT ( 'NONE',  ( 0.3460692066303958092, 0.1998031496062993018, -2.097769028871391050 ) ) ;
#61236=CARTESIAN_POINT ( 'NONE',  ( 0.1998031496062994405, -0.3460692066303958092, -1.824146981627296604 ) ) ;
#61237=CARTESIAN_POINT ( 'NONE',  ( 0.1058382717557499880, 0.3949938075777411073, -1.253280839895013488 ) ) ;
#61239=CARTESIAN_POINT ( 'NONE',  ( -0.3996062992125986035, -0.1070741851644056997, -2.565616797900262647 ) ) ;
#61241=CARTESIAN_POINT ( 'NONE',  ( 0.1049643490035304799, -0.3917322834645669549, -0.3923884514435694859 ) ) ;
#61245=CARTESIAN_POINT ( 'NONE',  ( -9.674558042662122972E-17, 0.3949938075777409963, -2.281496062992126372 ) ) ;
#61249=CARTESIAN_POINT ( 'NONE',  ( 0.4724409448818898682, 2.892866454678787531E-17, -2.480314960629921295 ) ) ;
#61250=CARTESIAN_POINT ( 'NONE',  ( -0.3996062992125986035, -7.340648628747425578E-17, -1.929133858267716439 ) ) ;
#61257=CARTESIAN_POINT ( 'NONE',  ( -0.3392501089628019439, 0.1958661417322832554, -2.625964936186665266 ) ) ;
#61264=CARTESIAN_POINT ( 'NONE',  ( -0.3392501089628019995, 0.1958661417322832277, 0.04658792650918625738 ) ) ;
#61266=CARTESIAN_POINT ( 'NONE',  ( -0.3917322834645669549, -0.1049643490035306603, -2.242782152230970993 ) ) ;
#61269=CARTESIAN_POINT ( 'NONE',  ( -0.2891555358219908833, -0.2891555358219912164, -2.736220472440944462 ) ) ;
#61274=CARTESIAN_POINT ( 'NONE',  ( 0.3996062992125986590, -0.1070741851644053111, -0.8989501312335956840 ) ) ;
#61278=CARTESIAN_POINT ( 'NONE',  ( 0.01987007963503858304, -0.3948464311378711011, -2.755905511811022279 ) ) ;
#61279=CARTESIAN_POINT ( 'NONE',  ( 0.3917322834645669549, 0.1049643490035304660, -0.2093175853018373611 ) ) ;
#61286=CARTESIAN_POINT ( 'NONE',  ( 0.2867679344610365999, 0.2867679344610365999, 0.02755905511811028441 ) ) ;
#61290=CARTESIAN_POINT ( 'NONE',  ( 0.3458507752293908943, 0.3458507752293908943, -1.555118110236220597 ) ) ;
#61292=CARTESIAN_POINT ( 'NONE',  ( 0.3917322834645670104, 2.398668435337828261E-17, -0.5826771653543306728 ) ) ;
#61297=CARTESIAN_POINT ( 'NONE',  ( -0.4724409448818898682, -8.678599364036362592E-17, -1.929133858267716439 ) ) ;
#61300=CARTESIAN_POINT ( 'NONE',  ( -0.3917322834645668994, -0.1049643490035306742, 0.1889956937345949883 ) ) ;
#61302=CARTESIAN_POINT ( 'NONE',  ( -0.1049643490035307020, 0.3917322834645669549, -0.4061679790026246906 ) ) ;
#61308=CARTESIAN_POINT ( 'NONE',  ( -0.3917322834645671215, 0.1049643490035301469, -2.387139107611548905 ) ) ;
#61312=CARTESIAN_POINT ( 'NONE',  ( -0.2362204724409451284, 0.4091458600556402425, -0.8772965879265091083 ) ) ;
#61323=CARTESIAN_POINT ( 'NONE',  ( 0.2925321140481932369, 0.2925321140481932369, -1.631889763779527325 ) ) ;
#61332=CARTESIAN_POINT ( 'NONE',  ( -0.2925321140481932369, 0.2925321140481930704, -0.09645669291338584972 ) ) ;
#61333=CARTESIAN_POINT ( 'NONE',  ( 0.1998031496062994405, -0.3460692066303958092, -0.7217847769028871152 ) ) ;
#61334=CARTESIAN_POINT ( 'NONE',  ( 0.2867679344610366554, 0.2867679344610366554, -2.811699105808085797 ) ) ;
#61341=CARTESIAN_POINT ( 'NONE',  ( 0.1974969037888704704, 0.3420746716998660508, -0.6935695538057742304 ) ) ;
#61347=CARTESIAN_POINT ( 'NONE',  ( 0.3458507752293908943, 0.3458507752293908943, -1.240157480314960647 ) ) ;
#61348=CARTESIAN_POINT ( 'NONE',  ( -0.2925321140481932369, 0.2925321140481931814, -2.381889763779527769 ) ) ;
#61351=CARTESIAN_POINT ( 'NONE',  ( 0.3917322834645670104, 0.1049643490035304660, -0.5938513367792144226 ) ) ;
#61352=EDGE_LOOP ( 'NONE', ( #82587, #71016, #46332, #57829 ) ) ;
#61364=CARTESIAN_POINT ( 'NONE',  ( 0.3392501089628018884, -0.1958661417322834220, -1.199475065616797842 ) ) ;
#61367=CARTESIAN_POINT ( 'NONE',  ( -0.1058382717557503211, 0.3949938075777409408, -0.9514435695538059345 ) ) ;
#61386=CARTESIAN_POINT ( 'NONE',  ( 4.893765752498283924E-17, -0.3996062992125986035, -1.496062992125984259 ) ) ;
#61389=CARTESIAN_POINT ( 'NONE',  ( 0.1998031496062994128, -0.3460692066303957537, -1.113517060367454015 ) ) ;
#61393=CARTESIAN_POINT ( 'NONE',  ( 0.2362204724409451007, -0.4091458600556402980, -0.4068241469816273326 ) ) ;
#61394=CARTESIAN_POINT ( 'NONE',  ( 0.3917322834645669549, 0.1049643490035304660, -2.729002624671915900 ) ) ;
#61400=CARTESIAN_POINT ( 'NONE',  ( -0.3458507752293906723, -0.3458507752293910609, -2.340551181102362488 ) ) ;
#61402=CARTESIAN_POINT ( 'NONE',  ( 0.1058382717557499880, 0.3949938075777409408, -1.802493438320210251 ) ) ;
#61412=CARTESIAN_POINT ( 'NONE',  ( -0.3917322834645668994, -0.1049643490035306742, -2.488169660596113886 ) ) ;
#61427=CARTESIAN_POINT ( 'NONE',  ( -9.787531504996566615E-17, 0.3996062992125985480, -0.2342519685039370358 ) ) ;
#61430=CARTESIAN_POINT ( 'NONE',  ( 0.2867679344610365999, 0.2867679344610365999, -1.797244094488188892 ) ) ;
#61441=CARTESIAN_POINT ( 'NONE',  ( 0.1998031496062994128, -0.3460692066303957537, -0.9560367454068241511 ) ) ;
#61443=CARTESIAN_POINT ( 'NONE',  ( 0.4724409448818880919, 0.1265901696525020825, -2.563648293963254776 ) ) ;
#61448=CARTESIAN_POINT ( 'NONE',  ( 0.1049643490035304938, -0.3917322834645669549, -1.587270341207349222 ) ) ;
#61453=CARTESIAN_POINT ( 'NONE',  ( 4.893765752498283308E-17, -0.3996062992125985480, -2.360236220472441193 ) ) ;
#61456=CARTESIAN_POINT ( 'NONE',  ( 0.1070741851644054915, -0.3996062992125986035, -0.5577427821522309426 ) ) ;
#61459=CARTESIAN_POINT ( 'NONE',  ( -0.3392501089628019995, 0.1958661417322832277, -2.223097112860892288 ) ) ;
#61469=CARTESIAN_POINT ( 'NONE',  ( 0.1049643490035303689, 0.3917322834645668994, -1.648274647472754095 ) ) ;
#61473=CARTESIAN_POINT ( 'NONE',  ( 0.1958661417322836440, -0.3392501089628017219, 0.07349081364829400387 ) ) ;
#61476=CARTESIAN_POINT ( 'NONE',  ( 0.2867679344610366554, 0.2867679344610366554, -2.811699105808085797 ) ) ;
#61484=CARTESIAN_POINT ( 'NONE',  ( -9.594673741351313045E-17, 0.3917322834645670659, -1.256580995571865200 ) ) ;
#61487=CARTESIAN_POINT ( 'NONE',  ( -0.3917322834645670104, -7.196005306013484475E-17, -2.171259842519685179 ) ) ;
#61492=CARTESIAN_POINT ( 'NONE',  ( -9.787531504996567848E-17, 0.3996062992125986035, -0.3149606299212598381 ) ) ;
#61496=CARTESIAN_POINT ( 'NONE',  ( 0.3460692066303959202, 0.1998031496062993295, -2.493438320209973469 ) ) ;
#61502=CARTESIAN_POINT ( 'NONE',  ( -0.3458507752293909498, 0.3458507752293907833, -1.198818897637795367 ) ) ;
#61506=CARTESIAN_POINT ( 'NONE',  ( 0.1974969037888706092, -0.3420746716998660508, -0.6410761154855643129 ) ) ;
#61520=CARTESIAN_POINT ( 'NONE',  ( 0.2925321140481932369, -0.2925321140481931814, -1.120078740157480324 ) ) ;
#61522=CARTESIAN_POINT ( 'NONE',  ( 0.3392501089628018884, -0.1958661417322834220, -1.199475065616797842 ) ) ;
#61537=CARTESIAN_POINT ( 'NONE',  ( -0.2362204724409447953, -0.4091458600556404646, -0.2998687664041995160 ) ) ;
#61540=EDGE_CURVE ( 'NONE', #25753, #65725, #79173, .T. ) ;
#61545=CARTESIAN_POINT ( 'NONE',  ( 0.1958661417322834775, 0.3392501089628018884, -2.188339525755591986 ) ) ;
#61548=B_SPLINE_CURVE_WITH_KNOTS ( 'NONE', 3,
 ( #31237, #12311, #56904, #76292, #25746, #63644, #70369, #5983, #31654, #83009, #12724, #38383, #64060, #6399, #8499, #71216, #47192, #21533 ),
 .UNSPECIFIED., .F., .F.,
 ( 4, 2, 2, 2, 2, 2, 2, 2, 4 ),
 ( 0.000000000000000000, 2.503579457911093929E-05, 5.007158915822187858E-05, 0.0001001431783164417514, 0.0002002863566328814428, 0.0004005727132657608798, 0.0008011454265315193744, 0.001602290853063036364, 0.003204581706126070559 ),
 .UNSPECIFIED. ) ;
#61552=CARTESIAN_POINT ( 'NONE',  ( -0.2925321140481930704, -0.2925321140481933480, -1.003937007874015741 ) ) ;
#61557=CARTESIAN_POINT ( 'NONE',  ( -0.2362204724409447953, -0.4091458600556404646, -0.06561679790026246628 ) ) ;
#61558=CARTESIAN_POINT ( 'NONE',  ( -0.3420746716998659953, -0.1974969037888706647, -2.414698162729658648 ) ) ;
#61561=CARTESIAN_POINT ( 'NONE',  ( -0.1049643490035307020, 0.3917322834645669549, -1.101049868766403872 ) ) ;
#61563=CARTESIAN_POINT ( 'NONE',  ( 0.2362204724409449064, 0.4091458600556404646, -2.506561679790026087 ) ) ;
#61569=CARTESIAN_POINT ( 'NONE',  ( 0.3392501089628018329, 0.1958661417322835052, -0.2112667734570061184 ) ) ;
#61575=CARTESIAN_POINT ( 'NONE',  ( -0.4724409448818908119, 0.1265901696524971698, -1.135170603674540590 ) ) ;
#61576=CARTESIAN_POINT ( 'NONE',  ( -0.3917322834645670659, -7.196005306013484475E-17, -1.610911704233282560 ) ) ;
#61582=CARTESIAN_POINT ( 'NONE',  ( 0.1958661417322836440, -0.3392501089628017219, -0.9639107611548557442 ) ) ;
#61592=CARTESIAN_POINT ( 'NONE',  ( -0.1958661417322834220, -0.3392501089628018884, -2.419947506561679784 ) ) ;
#61599=CARTESIAN_POINT ( 'NONE',  ( -0.3392501089628017219, -0.1958661417322836718, -0.7670603674540683592 ) ) ;
#61600=CARTESIAN_POINT ( 'NONE',  ( 5.785732909357575061E-17, -0.4724409448818898682, 0.001968503937007862279 ) ) ;
#61603=CARTESIAN_POINT ( 'NONE',  ( -0.3996062992125986590, 0.1070741851644051723, -2.629265091863517423 ) ) ;
#61613=CARTESIAN_POINT ( 'NONE',  ( -0.1070741851644057135, 0.3996062992125984925, -1.973097112860892510 ) ) ;
#61615=CARTESIAN_POINT ( 'NONE',  ( -0.3392501089628019995, 0.1958661417322832277, -0.01837270341207344546 ) ) ;
#61622=CARTESIAN_POINT ( 'NONE',  ( -0.2867679344610366554, 0.2867679344610365444, -1.674521366632859110 ) ) ;
#61631=CARTESIAN_POINT ( 'NONE',  ( 0.2867679344610366554, 0.2867679344610366554, -0.4494943813986370107 ) ) ;
#61635=CARTESIAN_POINT ( 'NONE',  ( -0.1265901696524986964, -0.4724409448818899238, -2.038713910761154491 ) ) ;
#61646=CARTESIAN_POINT ( 'NONE',  ( -0.3458507752293909498, 0.3458507752293908388, -2.143700787401574104 ) ) ;
#61655=CARTESIAN_POINT ( 'NONE',  ( -0.2925321140481930704, -0.2925321140481933480, -0.05905511811023624047 ) ) ;
#61656=CARTESIAN_POINT ( 'NONE',  ( -9.787531504996566615E-17, 0.3996062992125985480, -2.124015748031496287 ) ) ;
#61661=CARTESIAN_POINT ( 'NONE',  ( 0.3460692066303959757, -0.1998031496062991907, -1.679790026246719137 ) ) ;
#61662=CARTESIAN_POINT ( 'NONE',  ( -0.2891555358219908833, -0.2891555358219912164, -1.003937007874015741 ) ) ;
#61663=CARTESIAN_POINT ( 'NONE',  ( -0.1998031496062991907, -0.3460692066303959757, -2.270341207349081181 ) ) ;
#61664=CARTESIAN_POINT ( 'NONE',  ( -0.2362204724409451284, 0.4091458600556402425, -0.6430446194225721834 ) ) ;
#61665=CARTESIAN_POINT ( 'NONE',  ( 0.1958661417322834775, 0.3392501089628018884, -0.1364829396325459021 ) ) ;
#61669=CARTESIAN_POINT ( 'NONE',  ( -0.3420746716998660508, -0.1974969037888706924, -2.333989501312335957 ) ) ;
#61673=CARTESIAN_POINT ( 'NONE',  ( 5.785732909357575061E-17, -0.4724409448818898682, -2.440944881889763884 ) ) ;
#61674=CARTESIAN_POINT ( 'NONE',  ( 0.2925321140481932369, 0.2925321140481932369, -1.555118110236220597 ) ) ;
#61676=EDGE_LOOP ( 'NONE', ( #13327, #12489, #21519, #36933 ) ) ;
#61681=CARTESIAN_POINT ( 'NONE',  ( 0.1958661417322834775, 0.3392501089628018884, 0.08595800524934374409 ) ) ;
#61688=CARTESIAN_POINT ( 'NONE',  ( 0.3917322834645670104, -0.1049643490035303411, -0.03871391076115493490 ) ) ;
#61691=CARTESIAN_POINT ( 'NONE',  ( 0.3392501089628018884, -0.1958661417322834220, -2.459317585301837195 ) ) ;
#61694=CARTESIAN_POINT ( 'NONE',  ( -0.3420746716998661618, 0.1974969037888702206, -2.860892388451444113 ) ) ;
#61696=CARTESIAN_POINT ( 'NONE',  ( -0.4709442531824371558, -0.03757601356356778805, -1.220472440944882164 ) ) ;
#61698=CARTESIAN_POINT ( 'NONE',  ( -0.1998031496062991907, -0.3460692066303959757, -1.010498687664042050 ) ) ;
#61702=CARTESIAN_POINT ( 'NONE',  ( 0.04037479286079570517, -0.3917864676224462328, -2.755905511810075481 ) ) ;
#61703=CARTESIAN_POINT ( 'NONE',  ( 0.2867679344610365999, 0.2867679344610365999, -0.3799212598425197318 ) ) ;
#61709=CARTESIAN_POINT ( 'NONE',  ( 0.3917322834645670104, 2.398668435337828261E-17, -0.2677165354330708347 ) ) ;
#61710=ORIENTED_EDGE ( 'NONE', *, *, #73965, .F. ) ;
#61713=CARTESIAN_POINT ( 'NONE',  ( -0.4091458600556405756, 0.2362204724409446288, -1.758530183727034180 ) ) ;
#61724=CARTESIAN_POINT ( 'NONE',  ( 0.3392501089628018329, -0.1958661417322834497, -0.1850200542969010764 ) ) ;
#61726=CARTESIAN_POINT ( 'NONE',  ( -0.3917322834645669549, -0.1049643490035306603, -0.6030183727034120755 ) ) ;
#61731=CARTESIAN_POINT ( 'NONE',  ( 0.3392501089628018329, 0.1958661417322835607, -2.328083989501312345 ) ) ;
#61734=CARTESIAN_POINT ( 'NONE',  ( 0.1265901696524990294, -0.4724409448818896462, -0.7919947506561679784 ) ) ;
#61742=CARTESIAN_POINT ( 'NONE',  ( 0.1265901696524989184, 0.4724409448818898127, -0.3083989501312335846 ) ) ;
#61745=CARTESIAN_POINT ( 'NONE',  ( -0.2925321140481930149, -0.2925321140481933480, -1.868110236220472453 ) ) ;
#61753=CARTESIAN_POINT ( 'NONE',  ( -0.3996062992125986035, 0.1070741851644051584, -0.4245406824146982228 ) ) ;
#61754=CARTESIAN_POINT ( 'NONE',  ( 0.2925321140481932369, 0.2925321140481932369, -0.4527559055118109965 ) ) ;
#61755=CARTESIAN_POINT ( 'NONE',  ( 0.1958661417322834775, 0.3392501089628018884, -2.818260785598111884 ) ) ;
#61761=CARTESIAN_POINT ( 'NONE',  ( 0.1058382717557499880, 0.3949938075777409408, -0.7001312335958006505 ) ) ;
#61766=CARTESIAN_POINT ( 'NONE',  ( 0.3458507752293908943, -0.3458507752293908943, -1.200787401574803015 ) ) ;
#61767=CARTESIAN_POINT ( 'NONE',  ( -0.2925321140481932369, 0.2925321140481931814, -2.224409448818897683 ) ) ;
#61770=CARTESIAN_POINT ( 'NONE',  ( -0.2867679344610365444, -0.2867679344610367664, -0.6857148538395820836 ) ) ;
#61771=ORIENTED_EDGE ( 'NONE', *, *, #48287, .T. ) ;
#61782=CARTESIAN_POINT ( 'NONE',  ( 0.3917322834645669549, 0.1049643490035304660, -0.9041994750656167090 ) ) ;
#61785=CARTESIAN_POINT ( 'NONE',  ( -0.1058382717557503211, 0.3949938075777409408, -1.266404199475065440 ) ) ;
#61801=CARTESIAN_POINT ( 'NONE',  ( 0.3996062992125986035, 2.446882876249141962E-17, -1.850393700787401619 ) ) ;
#61804=CARTESIAN_POINT ( 'NONE',  ( 4.893765752498283308E-17, -0.3996062992125985480, -1.415354330708661346 ) ) ;
#61808=CARTESIAN_POINT ( 'NONE',  ( -0.3458507752293906723, -0.3458507752293910609, -0.5314960629921260393 ) ) ;
#61810=CARTESIAN_POINT ( 'NONE',  ( 0.1049643490035304938, -0.3917322834645669549, -2.689632545931758489 ) ) ;
#61816=CARTESIAN_POINT ( 'NONE',  ( -0.4724409448818895907, -0.1265901696524993070, -2.169947506561679340 ) ) ;
#61818=CARTESIAN_POINT ( 'NONE',  ( 4.837279021331061486E-17, -0.3949938075777409963, -1.730314960629921295 ) ) ;
#61829=CARTESIAN_POINT ( 'NONE',  ( 4.797336870675655290E-17, -0.3917322834645669549, -2.363497744585615123 ) ) ;
#61842=CARTESIAN_POINT ( 'NONE',  ( 0.1998031496062992463, 0.3460692066303959202, -0.5360892388451443669 ) ) ;
#61843=CARTESIAN_POINT ( 'NONE',  ( -0.3917322834645670104, -7.196005306013484475E-17, -1.856299212598425230 ) ) ;
#61852=CARTESIAN_POINT ( 'NONE',  ( 0.1070741851644054776, -0.3996062992125984925, -1.264435695538057569 ) ) ;
#61859=CARTESIAN_POINT ( 'NONE',  ( -0.2867679344610364334, -0.2867679344610367109, -1.718503937007874072 ) ) ;
#61863=CARTESIAN_POINT ( 'NONE',  ( -0.4724409448818898682, -8.678599364036362592E-17, -0.5118110236220472231 ) ) ;
#61864=CARTESIAN_POINT ( 'NONE',  ( 0.3996062992125985480, 2.446882876249141654E-17, -2.242125984251968518 ) ) ;
#61866=CARTESIAN_POINT ( 'NONE',  ( -0.2925321140481932924, 0.2925321140481931814, -0.8070866141732284671 ) ) ;
#61869=CARTESIAN_POINT ( 'NONE',  ( -0.1049643490035302024, -0.3917322834645671215, -2.741469816272964710 ) ) ;
#61879=CARTESIAN_POINT ( 'NONE',  ( 0.3392501089628018329, -0.1958661417322834497, -2.074783833824459744 ) ) ;
#61882=CARTESIAN_POINT ( 'NONE',  ( -0.1049643490035302024, -0.3917322834645671215, -2.833989501312335957 ) ) ;
#61885=CARTESIAN_POINT ( 'NONE',  ( 0.1974969037888704704, 0.3420746716998660508, -0.1443569553805774675 ) ) ;
#61887=ORIENTED_EDGE ( 'NONE', *, *, #33217, .F. ) ;
#61893=CARTESIAN_POINT ( 'NONE',  ( 0.2867679344610366554, -0.2867679344610365999, -1.197525877461629307 ) ) ;
#61895=CARTESIAN_POINT ( 'NONE',  ( -9.594673741351313045E-17, 0.3917322834645670104, -2.131889763779527769 ) ) ;
#61900=CIRCLE ( 'NONE', #68634, 0.4724409448818898682 ) ;
#61901=CARTESIAN_POINT ( 'NONE',  ( 4.893765752498283924E-17, -0.3996062992125986035, -0.2362204724409449341 ) ) ;
#61903=CARTESIAN_POINT ( 'NONE',  ( 0.3996062992125985480, 2.446882876249141654E-17, 0.1200787401574803098 ) ) ;
#61905=CARTESIAN_POINT ( 'NONE',  ( -0.3996062992125986035, -0.1070741851644056997, -2.093175853018372834 ) ) ;
#61910=CARTESIAN_POINT ( 'NONE',  ( 0.2362204724409451007, -0.4091458600556402980, -1.113517060367454015 ) ) ;
#61913=CARTESIAN_POINT ( 'NONE',  ( 0.3420746716998660508, 0.1974969037888705814, -0.6804461942257220564 ) ) ;
#61919=DIRECTION ( 'NONE',  ( 1.000000000000000000, 0.000000000000000000, 0.000000000000000000 ) ) ;
#61927=CARTESIAN_POINT ( 'NONE',  ( 0.3996062992125985480, 2.446882876249141654E-17, -1.612204724409448842 ) ) ;
#61929=CARTESIAN_POINT ( 'NONE',  ( 4.797336870675656522E-17, -0.3917322834645670104, -1.645669291338582640 ) ) ;
#61931=CARTESIAN_POINT ( 'NONE',  ( -0.2432155562301253904, -0.3078094465263045976, 3.457013956890525812E-17 ) ) ;
#61945=EDGE_CURVE ( 'NONE', #15221, #54535, #11679, .T. ) ;
#61953=CARTESIAN_POINT ( 'NONE',  ( -0.3392501089628017219, -0.1958661417322836995, -1.938995693734595127 ) ) ;
#61960=CARTESIAN_POINT ( 'NONE',  ( 0.3460692066303959202, 0.1998031496062993295, -1.076115485564304475 ) ) ;
#61965=CARTESIAN_POINT ( 'NONE',  ( 0.4724409448818896462, 0.1265901696524990294, 0.03280839895013123314 ) ) ;
#61966=CARTESIAN_POINT ( 'NONE',  ( -0.1058382717557503211, 0.3949938075777409408, -2.683727034120735766 ) ) ;
#61969=CARTESIAN_POINT ( 'NONE',  ( -0.2867679344610365999, 0.2867679344610364889, -1.586614173228346747 ) ) ;
#61971=CARTESIAN_POINT ( 'NONE',  ( 0.1265901696524990294, -0.4724409448818896462, -2.604986876640420057 ) ) ;
#61972=CARTESIAN_POINT ( 'NONE',  ( 0.4091458600556403535, 0.2362204724409449896, -0.8379265091863516979 ) ) ;
#61979=CARTESIAN_POINT ( 'NONE',  ( -0.3392501089628018329, -0.1958661417322836440, -0.1325266159766911034 ) ) ;
#61984=FACE_OUTER_BOUND ( 'NONE', #71187, .T. ) ;
#61985=CARTESIAN_POINT ( 'NONE',  ( 0.3460692066303959202, 0.1998031496062993295, -2.808398950131233640 ) ) ;
#61986=CARTESIAN_POINT ( 'NONE',  ( 0.2867679344610366554, 0.2867679344610366554, -1.551856586123046888 ) ) ;
#61992=CARTESIAN_POINT ( 'NONE',  ( 0.1049643490035303689, 0.3917322834645670104, -1.180446194225722056 ) ) ;
#62001=ADVANCED_FACE ( 'NONE', ( #53062 ), #2576, .T. ) ;
#62003=CARTESIAN_POINT ( 'NONE',  ( -0.3392501089628019995, 0.1958661417322832277, -2.223097112860892288 ) ) ;
#62009=CARTESIAN_POINT ( 'NONE',  ( 0.1958661417322834775, 0.3392501089628018884, -0.7014435695538058235 ) ) ;
#62010=CARTESIAN_POINT ( 'NONE',  ( 0.09156050430091122738, 0.3808816823641256732, -2.755905511811024056 ) ) ;
#62012=CARTESIAN_POINT ( 'NONE',  ( -0.2925321140481930149, -0.2925321140481933480, -2.498031496062992574 ) ) ;
#62032=CARTESIAN_POINT ( 'NONE',  ( -0.1049643490035301746, -0.3917322834645670659, -1.727014804953068916 ) ) ;
#62041=CARTESIAN_POINT ( 'NONE',  ( -0.1958661417322836995, 0.3392501089628017219, -0.3248224653881383595 ) ) ;
#62045=CARTESIAN_POINT ( 'NONE',  ( 0.4724409448818896462, 0.1265901696524990294, -2.091207349081364519 ) ) ;
#62064=CARTESIAN_POINT ( 'NONE',  ( 0.1998031496062994405, -0.3460692066303958092, -0.09186351706036746667 ) ) ;
#62065=CARTESIAN_POINT ( 'NONE',  ( 0.3996062992125986035, -0.1070741851644052972, -2.393044619422572072 ) ) ;
#62071=CARTESIAN_POINT ( 'NONE',  ( 0.3996062992125986035, 2.446882876249141962E-17, -1.692913385826771533 ) ) ;
#62072=CARTESIAN_POINT ( 'NONE',  ( -0.3420746716998661618, 0.1974969037888702206, -1.128608923884514503 ) ) ;
#62073=CARTESIAN_POINT ( 'NONE',  ( 0.1998031496062994405, -0.3460692066303958092, -2.454068241469816058 ) ) ;
#62075=CARTESIAN_POINT ( 'NONE',  ( 0.3917322834645670104, 2.398668435337828261E-17, -0.4251968503937007537 ) ) ;
#62079=CARTESIAN_POINT ( 'NONE',  ( -0.3949938075777408852, -0.1058382717557502933, -2.012467191601050143 ) ) ;
#62082=CARTESIAN_POINT ( 'NONE',  ( -0.4091458600556405756, 0.2362204724409446288, -2.388451443569553856 ) ) ;
#62083=CARTESIAN_POINT ( 'NONE',  ( 0.1998031496062992740, 0.3460692066303959757, -1.561679790026246684 ) ) ;
#62090=CARTESIAN_POINT ( 'NONE',  ( -0.2867679344610364334, -0.2867679344610368219, -2.658773335136795701 ) ) ;
#62097=CARTESIAN_POINT ( 'NONE',  ( 0.1958661417322834775, 0.3392501089628018884, -0.07152230971128617498 ) ) ;
#62099=CARTESIAN_POINT ( 'NONE',  ( 0.3917322834645670104, -0.1049643490035303411, -2.308398950131233640 ) ) ;
#62102=CARTESIAN_POINT ( 'NONE',  ( -0.3949938075777409963, -7.255918531996591613E-17, -2.874015748031495843 ) ) ;
#62106=CARTESIAN_POINT ( 'NONE',  ( -0.3460692066303958092, -0.1998031496062994683, -0.8398950131233595684 ) ) ;
#62111=CARTESIAN_POINT ( 'NONE',  ( -0.3392501089628019995, 0.1958661417322832277, -0.4258530183727035068 ) ) ;
#62117=CARTESIAN_POINT ( 'NONE',  ( 0.3917322834645670104, 2.398668435337828261E-17, -0.1102362204724409156 ) ) ;
#62121=CARTESIAN_POINT ( 'NONE',  ( 0.3458507752293908943, 0.3458507752293908943, -1.712598425196850460 ) ) ;
#62131=CARTESIAN_POINT ( 'NONE',  ( 0.2867679344610365999, -0.2867679344610365999, -0.3359386894675047142 ) ) ;
#62133=CARTESIAN_POINT ( 'NONE',  ( 0.3917322834645670104, -0.1049643490035303273, -0.3536745406824148286 ) ) ;
#62139=CARTESIAN_POINT ( 'NONE',  ( 0.2867679344610365999, -0.2867679344610365444, -2.452755905511811108 ) ) ;
#62142=CARTESIAN_POINT ( 'NONE',  ( -0.1265901696524993347, 0.4724409448818895907, -0.7132545931758530466 ) ) ;
#62152=ORIENTED_EDGE ( 'NONE', *, *, #48287, .F. ) ;
#62154=CARTESIAN_POINT ( 'NONE',  ( -0.1998031496062994405, 0.3460692066303957537, -1.979658792650918597 ) ) ;
#62162=CARTESIAN_POINT ( 'NONE',  ( 0.1998031496062994128, -0.3460692066303957537, -0.1686351706036745557 ) ) ;
#62164=CARTESIAN_POINT ( 'NONE',  ( 0.1998031496062992740, 0.3460692066303959757, -0.6167979002624671692 ) ) ;
#62165=CARTESIAN_POINT ( 'NONE',  ( 0.3949938075777411073, -0.1058382717557499464, 0.04593175853018367782 ) ) ;
#62170=CARTESIAN_POINT ( 'NONE',  ( 0.2891555358219910499, 0.2891555358219910499, -0.8444881889763782290 ) ) ;
#62176=CARTESIAN_POINT ( 'NONE',  ( 0.4091458600556404646, -0.2362204724409448231, -1.207349081364829324 ) ) ;
#62177=CARTESIAN_POINT ( 'NONE',  ( 0.3460692066303959757, -0.1998031496062991907, -2.309711286089239035 ) ) ;
#62180=CARTESIAN_POINT ( 'NONE',  ( -0.3917322834645670659, -7.196005306013484475E-17, -0.9809904443907629945 ) ) ;
#62192=CARTESIAN_POINT ( 'NONE',  ( 0.2867679344610365999, 0.2867679344610365999, -1.074803149606299080 ) ) ;
#62195=CARTESIAN_POINT ( 'NONE',  ( -0.3949938075777409963, -7.255918531996591613E-17, -1.456692913385826627 ) ) ;
#62205=CARTESIAN_POINT ( 'NONE',  ( -0.2362204724409447953, -0.4091458600556404646, -1.010498687664042050 ) ) ;
#62206=CARTESIAN_POINT ( 'NONE',  ( -0.1049643490035307020, 0.3917322834645669549, 0.06627296587926499727 ) ) ;
#62212=CARTESIAN_POINT ( 'NONE',  ( 0.1998031496062992740, 0.3460692066303959757, -2.034120734908136718 ) ) ;
#62215=CARTESIAN_POINT ( 'NONE',  ( 0.2925321140481932369, -0.2925321140481931814, -1.435039370078740051 ) ) ;
#62216=CARTESIAN_POINT ( 'NONE',  ( -0.03087045868620141853, 0.3974833285012848716, -2.755905511811078679 ) ) ;
#62219=CARTESIAN_POINT ( 'NONE',  ( -0.3458507752293909498, 0.3458507752293907833, -0.3346456692913385988 ) ) ;
#62221=CARTESIAN_POINT ( 'NONE',  ( 4.797336870675656522E-17, -0.3917322834645670104, -2.840551181102362044 ) ) ;
#62227=CARTESIAN_POINT ( 'NONE',  ( -0.4724409448818895907, -0.1265901696524993070, -2.484908136482939955 ) ) ;
#62229=CARTESIAN_POINT ( 'NONE',  ( -9.674558042662122972E-17, 0.3949938075777409963, -2.438976377952756014 ) ) ;
#62251=CARTESIAN_POINT ( 'NONE',  ( -0.1998031496062994405, 0.3460692066303957537, -0.8772965879265091083 ) ) ;
#62253=CARTESIAN_POINT ( 'NONE',  ( 0.3917322834645669549, 0.1049643490035304660, -2.099081364829396446 ) ) ;
#62258=CARTESIAN_POINT ( 'NONE',  ( 4.893765752498283924E-17, -0.3996062992125986035, -2.755905511811023612 ) ) ;
#62268=CARTESIAN_POINT ( 'NONE',  ( 0.3917322834645669549, 0.1049643490035304660, -1.469160104986876769 ) ) ;
#62269=CARTESIAN_POINT ( 'NONE',  ( -0.2798680777847367684, 0.2749078412854674691, -1.220472440944882164 ) ) ;
#62272=CARTESIAN_POINT ( 'NONE',  ( 0.1265901696524989184, 0.4724409448818898127, -0.4658792650918635037 ) ) ;
#62273=CARTESIAN_POINT ( 'NONE',  ( -0.2925321140481930149, -0.2925321140481933480, -2.498031496062992574 ) ) ;
#62275=CARTESIAN_POINT ( 'NONE',  ( 0.1998031496062994405, -0.3460692066303958092, -0.7217847769028871152 ) ) ;
#62276=EDGE_LOOP ( 'NONE', ( #78479, #1041, #1228, #11798 ) ) ;
#62278=CARTESIAN_POINT ( 'NONE',  ( 0.2867679344610365999, -0.2867679344610365444, -2.610236220472441193 ) ) ;
#62289=CARTESIAN_POINT ( 'NONE',  ( 0.3392501089628018329, -0.1958661417322834497, -1.917303518863830103 ) ) ;
#62292=CARTESIAN_POINT ( 'NONE',  ( 0.3917322834645669549, 0.1049643490035304660, 0.04068241469816277767 ) ) ;
#62295=CARTESIAN_POINT ( 'NONE',  ( 0.1974969037888704704, 0.3420746716998660508, -0.3018372703412073865 ) ) ;
#62303=CARTESIAN_POINT ( 'NONE',  ( -0.1958661417322833942, -0.3392501089628018884, -1.164717478511497983 ) ) ;
#62305=CARTESIAN_POINT ( 'NONE',  ( 0.3917322834645670104, 2.398668435337828261E-17, -2.564960629921259727 ) ) ;
#62310=CARTESIAN_POINT ( 'NONE',  ( -0.2925321140481932924, 0.2925321140481931814, -0.9645669291338579976 ) ) ;
#62312=CARTESIAN_POINT ( 'NONE',  ( 0.3996062992125984925, 0.1070741851644054637, -0.3589238845144357426 ) ) ;
#62314=CARTESIAN_POINT ( 'NONE',  ( -0.2925321140481930704, -0.2925321140481933480, -2.421259842519684735 ) ) ;
#62318=CARTESIAN_POINT ( 'NONE',  ( 0.3458507752293908943, -0.3458507752293908943, -1.277559055118109965 ) ) ;
#62321=CARTESIAN_POINT ( 'NONE',  ( -0.1058382717557497660, -0.3949938075777411073, -0.9363517060367456679 ) ) ;
#62334=CARTESIAN_POINT ( 'NONE',  ( 0.2925321140481932369, -0.2925321140481931814, -1.750000000000000222 ) ) ;
#62336=CARTESIAN_POINT ( 'NONE',  ( 0.3917322834645670104, 2.398668435337828261E-17, -1.370078740157480324 ) ) ;
#62352=CARTESIAN_POINT ( 'NONE',  ( 0.3983403474834781299, 0.03178304480585100733, -1.929133858267716661 ) ) ;
#62366=CARTESIAN_POINT ( 'NONE',  ( 4.893765752498283924E-17, -0.3996062992125986035, -1.181102362204724310 ) ) ;
#62368=CARTESIAN_POINT ( 'NONE',  ( 0.1049643490035303689, 0.3917322834645670104, -2.032808398950130879 ) ) ;
#62371=CARTESIAN_POINT ( 'NONE',  ( -0.3458507752293906723, -0.3458507752293910609, -0.5314960629921260393 ) ) ;
#62372=CARTESIAN_POINT ( 'NONE',  ( -0.3949938075777409408, -0.1058382717557502933, -2.880577427821522374 ) ) ;
#62375=CARTESIAN_POINT ( 'NONE',  ( 0.1958661417322836440, -0.3392501089628017219, -1.343832020997375531 ) ) ;
#62377=CARTESIAN_POINT ( 'NONE',  ( 0.4724409448818896462, 0.1265901696524990294, -2.644356955380577912 ) ) ;
#62384=CARTESIAN_POINT ( 'NONE',  ( 0.1049643490035303689, 0.3917322834645668994, -0.7033927577089746919 ) ) ;
#62390=CARTESIAN_POINT ( 'NONE',  ( 0.000000000000000000, 0.000000000000000000, -2.755905511811024056 ) ) ;
#62392=ORIENTED_EDGE ( 'NONE', *, *, #66038, .F. ) ;
#62393=CARTESIAN_POINT ( 'NONE',  ( 0.1049643490035303967, 0.3917322834645670659, -2.037420890584989319 ) ) ;
#62399=CARTESIAN_POINT ( 'NONE',  ( 0.1049643490035304938, -0.3917322834645669549, -1.272309711286089273 ) ) ;
#62409=CARTESIAN_POINT ( 'NONE',  ( 0.3392501089628018329, 0.1958661417322835607, -2.800524934383201714 ) ) ;
#62417=CARTESIAN_POINT ( 'NONE',  ( -0.2867679344610364334, -0.2867679344610367109, -0.7736220472440945573 ) ) ;
#62421=CARTESIAN_POINT ( 'NONE',  ( -0.1998031496062994405, 0.3460692066303957537, -2.294619422572178102 ) ) ;
#62430=CARTESIAN_POINT ( 'NONE',  ( 0.3460692066303959202, -0.1998031496062991630, -0.3392388451443569819 ) ) ;
#62432=( BOUNDED_CURVE ( )  B_SPLINE_CURVE ( 2, ( #5645, #82270, #24588, #51069, #70443, #12801, #168, #69631, #68805, #75953, #37226, #38042, #11976 ),
 .UNSPECIFIED., .F., .F. ) 
 B_SPLINE_CURVE_WITH_KNOTS ( ( 3, 2, 2, 2, 2, 2, 3 ),
 ( 0.8375000000000000222, 0.8416666666666666741, 0.8458333333333333259, 0.8499999999999999778, 0.8541666666666666297, 0.8583333333333332815, 0.8625000000000000444 ),
 .UNSPECIFIED. ) 
 CURVE ( )  GEOMETRIC_REPRESENTATION_ITEM ( )  RATIONAL_B_SPLINE_CURVE ( ( 1.000000000000000000, 0.9659258262890683122, 1.000000000000000000, 0.9659258262890683122, 1.000000000000000000, 0.9659258262890683122, 1.000000000000000000, 0.9659258262890683122, 1.000000000000000000, 0.9659258262890683122, 1.000000000000000000, 0.9659258262890683122, 1.000000000000000000 ) ) 
 REPRESENTATION_ITEM ( '' )  );
#62433=CARTESIAN_POINT ( 'NONE',  ( -0.1049643490035307020, 0.3917322834645669549, -0.3136482939632545541 ) ) ;
#62440=CARTESIAN_POINT ( 'NONE',  ( -0.2867679344610366554, 0.2867679344610365444, -1.517041051672229024 ) ) ;
#62450=CARTESIAN_POINT ( 'NONE',  ( -0.3392501089628017219, -0.1958661417322836995, -0.8366334890101857491 ) ) ;
#62454=CARTESIAN_POINT ( 'NONE',  ( 0.4724409448818898682, 2.892866454678787531E-17, -2.242125984251968518 ) ) ;
#62457=ADVANCED_FACE ( 'NONE', ( #55544 ), #11789, .T. ) ;
#62471=VERTEX_POINT ( 'NONE', #3814 ) ;
#62476=CARTESIAN_POINT ( 'NONE',  ( -0.3460692066303958092, -0.1998031496062994683, -0.05249343832020999384 ) ) ;
#62477=CARTESIAN_POINT ( 'NONE',  ( -0.3996062992125986590, 0.1070741851644051723, -2.629265091863517423 ) ) ;
#62482=CARTESIAN_POINT ( 'NONE',  ( 0.3460692066303959757, -0.1998031496062991907, -2.152230971128608950 ) ) ;
#62484=CARTESIAN_POINT ( 'NONE',  ( -0.3949938075777409408, -0.1058382717557502933, -1.305774278215223072 ) ) ;
#62485=CARTESIAN_POINT ( 'NONE',  ( -9.787531504996567848E-17, 0.3996062992125986035, -2.834645669291338432 ) ) ;
#62487=CARTESIAN_POINT ( 'NONE',  ( -0.2867679344610366554, 0.2867679344610365444, -0.6417322834645668994 ) ) ;
#62491=CARTESIAN_POINT ( 'NONE',  ( -9.674558042662122972E-17, 0.3949938075777409963, -2.596456692913385655 ) ) ;
#62495=CARTESIAN_POINT ( 'NONE',  ( -0.4091458600556402980, -0.2362204724409451284, -2.414698162729658648 ) ) ;
#62496=CARTESIAN_POINT ( 'NONE',  ( 0.3996062992125986035, 2.446882876249141962E-17, -2.165354330708661568 ) ) ;
#62503=CARTESIAN_POINT ( 'NONE',  ( 0.3392501089628018329, -0.1958661417322834497, -2.704705093666980087 ) ) ;
#62510=CARTESIAN_POINT ( 'NONE',  ( -0.1049643490035302024, -0.3917322834645671215, -0.3143044619422573072 ) ) ;
#62511=CARTESIAN_POINT ( 'NONE',  ( -0.3392501089628017219, -0.1958661417322836718, -1.461942257217847763 ) ) ;
#62512=CARTESIAN_POINT ( 'NONE',  ( -0.1049643490035302024, -0.3917322834645671215, -2.269028871391075786 ) ) ;
#62515=CARTESIAN_POINT ( 'NONE',  ( -0.1058382717557497937, -0.3949938075777411628, -2.749343832020997969 ) ) ;
#62519=CARTESIAN_POINT ( 'NONE',  ( -0.2925321140481932924, 0.2925321140481931814, -0.9645669291338579976 ) ) ;
#62525=CARTESIAN_POINT ( 'NONE',  ( -0.3917322834645669549, -0.1049643490035306603, -0.6030183727034120755 ) ) ;
#62531=CARTESIAN_POINT ( 'NONE',  ( 0.3392501089628018329, 0.1958661417322835607, -0.2808398950131232863 ) ) ;
#62536=CARTESIAN_POINT ( 'NONE',  ( 0.3458507752293908943, -0.3458507752293908943, -1.830708661417322913 ) ) ;
#62549=CARTESIAN_POINT ( 'NONE',  ( 0.1049643490035303689, 0.3917322834645668994, -0.5459124427483446063 ) ) ;
#62551=CARTESIAN_POINT ( 'NONE',  ( -9.594673741351313045E-17, 0.3917322834645670104, -1.029527559055118280 ) ) ;
#62557=CARTESIAN_POINT ( 'NONE',  ( -0.2867679344610364334, -0.2867679344610367109, -2.255905511811023612 ) ) ;
#62560=CARTESIAN_POINT ( 'NONE',  ( 0.2362204724409451007, -0.4091458600556402980, -0.9560367454068241511 ) ) ;
#62571=CARTESIAN_POINT ( 'NONE',  ( 0.3460692066303958092, 0.1998031496062993018, -1.940288713910761187 ) ) ;
#62579=CARTESIAN_POINT ( 'NONE',  ( -0.1998031496062994405, 0.3460692066303957537, -0.08989501312335959615 ) ) ;
#62580=CARTESIAN_POINT ( 'NONE',  ( -0.1998031496062991907, -0.3460692066303959757, -0.6955380577427822120 ) ) ;
#62581=CARTESIAN_POINT ( 'NONE',  ( -0.3420746716998661618, 0.1974969037888702206, -0.1837270341207349611 ) ) ;
#62587=CARTESIAN_POINT ( 'NONE',  ( -0.1974969037888704149, -0.3420746716998661063, -0.7723097112860893843 ) ) ;
#62592=CARTESIAN_POINT ( 'NONE',  ( 5.785732909357575061E-17, -0.4724409448818898682, -1.023622047244094446 ) ) ;
#62593=CARTESIAN_POINT ( 'NONE',  ( -0.3996062992125985480, -0.1070741851644057135, -2.408136482939632561 ) ) ;
#62597=CARTESIAN_POINT ( 'NONE',  ( -0.1958661417322833942, -0.3392501089628018884, -0.8497568485902381452 ) ) ;
#62609=CARTESIAN_POINT ( 'NONE',  ( -0.2867679344610364334, -0.2867679344610367109, -1.153543307086613900 ) ) ;
#62612=CARTESIAN_POINT ( 'NONE',  ( 0.2891555358219910499, -0.2891555358219909944, -1.515748031496063186 ) ) ;
#62620=CARTESIAN_POINT ( 'NONE',  ( 0.4724409448818898682, 2.892866454678787531E-17, -1.220472440944881942 ) ) ;
#62624=CARTESIAN_POINT ( 'NONE',  ( -0.1958661417322836718, 0.3392501089628017219, 0.05971128608923875758 ) ) ;
#62630=CARTESIAN_POINT ( 'NONE',  ( 0.2925321140481932369, 0.2925321140481932369, -2.185039370078739829 ) ) ;
#62633=CARTESIAN_POINT ( 'NONE',  ( 0.1070741851644054776, -0.3996062992125984925, -1.736876640419947604 ) ) ;
#62637=CARTESIAN_POINT ( 'NONE',  ( -0.4091458600556402980, -0.2362204724409451284, -0.3674540682414698112 ) ) ;
#62639=CARTESIAN_POINT ( 'NONE',  ( 0.2867679344610365999, -0.2867679344610365444, 0.06692913385826775030 ) ) ;
#62647=CARTESIAN_POINT ( 'NONE',  ( 0.3458507752293908943, 0.3458507752293908943, -2.261811023622047223 ) ) ;
#62650=CARTESIAN_POINT ( 'NONE',  ( 0.1058382717557499880, 0.3949938075777409408, -2.432414698162729927 ) ) ;
#62672=CARTESIAN_POINT ( 'NONE',  ( -0.3996062992125985480, -7.340648628747423112E-17, -0.5885826771653542844 ) ) ;
#62673=CARTESIAN_POINT ( 'NONE',  ( 0.1958661417322836440, -0.3392501089628017219, -2.381233595800524849 ) ) ;
#62688=CARTESIAN_POINT ( 'NONE',  ( -0.3917322834645669549, -0.1049643490035306603, -1.390419947506561504 ) ) ;
#62695=CARTESIAN_POINT ( 'NONE',  ( -0.2925321140481930149, -0.2925321140481933480, -2.340551181102362488 ) ) ;
#62698=CARTESIAN_POINT ( 'NONE',  ( 0.3460692066303959757, -0.1998031496062991907, -1.049868766404199460 ) ) ;
#62701=CARTESIAN_POINT ( 'NONE',  ( 0.1049643490035303689, 0.3917322834645670104, -2.820209973753280419 ) ) ;
#62714=CARTESIAN_POINT ( 'NONE',  ( -0.3392501089628019995, 0.1958661417322832277, -2.788057742782152459 ) ) ;
#62717=CARTESIAN_POINT ( 'NONE',  ( -0.3420746716998661618, 0.1974969037888702206, -0.02624671916010504202 ) ) ;
#62718=ORIENTED_EDGE ( 'NONE', *, *, #78043, .T. ) ;
#62725=CARTESIAN_POINT ( 'NONE',  ( -0.1049643490035302301, -0.3917322834645671770, -1.328759473262154378 ) ) ;
#62727=CARTESIAN_POINT ( 'NONE',  ( 0.3917322834645670104, 2.398668435337828261E-17, -2.722440944881889369 ) ) ;
#62732=CARTESIAN_POINT ( 'NONE',  ( -0.1998031496062994683, 0.3460692066303958092, -0.9580052493438320216 ) ) ;
#62734=CARTESIAN_POINT ( 'NONE',  ( -0.2925321140481930149, -0.2925321140481933480, -0.4507874015748031815 ) ) ;
#62737=CARTESIAN_POINT ( 'NONE',  ( 0.1998031496062994405, -0.3460692066303958092, -2.454068241469816058 ) ) ;
#62739=CARTESIAN_POINT ( 'NONE',  ( 4.797336870675656522E-17, -0.3917322834645670104, -1.738188976377952777 ) ) ;
#62743=CARTESIAN_POINT ( 'NONE',  ( -1.157146581871515012E-16, 0.4724409448818898682, -1.021653543307086576 ) ) ;
#62747=CARTESIAN_POINT ( 'NONE',  ( 0.3420746716998660508, 0.1974969037888705814, -0.8379265091863515869 ) ) ;
#62749=CARTESIAN_POINT ( 'NONE',  ( 0.2362204724409451007, -0.4091458600556402980, -1.113517060367454015 ) ) ;
#62752=CARTESIAN_POINT ( 'NONE',  ( 0.000000000000000000, 0.000000000000000000, -2.755905511811024056 ) ) ;
#62760=CARTESIAN_POINT ( 'NONE',  ( -0.3460692066303960313, 0.1998031496062989965, -1.835301837270341352 ) ) ;
#62776=CARTESIAN_POINT ( 'NONE',  ( 0.1049643490035303689, 0.3917322834645670104, -0.8654855643044619962 ) ) ;
#62792=CARTESIAN_POINT ( 'NONE',  ( 0.2925321140481932369, 0.2925321140481932369, -1.082677165354330562 ) ) ;
#62794=CARTESIAN_POINT ( 'NONE',  ( -0.1049643490035301885, -0.3917322834645671215, -1.954068241469816281 ) ) ;
#62798=CARTESIAN_POINT ( 'NONE',  ( 0.4724409448818898682, 2.892866454678787531E-17, -0.4330708661417322913 ) ) ;
#62799=CARTESIAN_POINT ( 'NONE',  ( 0.2891555358219910499, -0.2891555358219909944, -2.933070866141733291 ) ) ;
#62802=CARTESIAN_POINT ( 'NONE',  ( 0.1049643490035304938, -0.3917322834645669549, -1.494750656167978642 ) ) ;
#62804=CARTESIAN_POINT ( 'NONE',  ( -0.4091458600556402980, -0.2362204724409451284, -2.572178477690288734 ) ) ;
#62810=CARTESIAN_POINT ( 'NONE',  ( 0.3392501089628018329, -0.1958661417322834497, -0.8149413141394206139 ) ) ;
#62819=CARTESIAN_POINT ( 'NONE',  ( 0.3917322834645670659, -0.1049643490035303273, -1.998050811844831243 ) ) ;
#62825=CARTESIAN_POINT ( 'NONE',  ( -0.3392501089628019995, 0.1958661417322832277, -1.370734908136483021 ) ) ;
#62835=CARTESIAN_POINT ( 'NONE',  ( 0.3392501089628018884, -0.1958661417322834220, -2.931758530183726563 ) ) ;
#62842=CARTESIAN_POINT ( 'NONE',  ( -0.1958661417322834220, -0.3392501089628018884, -1.252624671916010568 ) ) ;
#62843=CARTESIAN_POINT ( 'NONE',  ( 0.2925321140481932369, -0.2925321140481931814, -2.852362204724409711 ) ) ;
#62852=CARTESIAN_POINT ( 'NONE',  ( -0.3996062992125986590, 0.1070741851644051723, -0.5820209973753280863 ) ) ;
#62854=CARTESIAN_POINT ( 'NONE',  ( -0.1049643490035302024, -0.3917322834645671215, -0.3792650918635169233 ) ) ;
#62870=CARTESIAN_POINT ( 'NONE',  ( 0.1049643490035303967, 0.3917322834645670659, -0.9350586858605794971 ) ) ;
#62875=CARTESIAN_POINT ( 'NONE',  ( -0.4724409448818898682, -8.678599364036362592E-17, -2.005905511811023612 ) ) ;
#62889=EDGE_LOOP ( 'NONE', ( #72008, #32686, #42113, #6614 ) ) ;
#62894=CARTESIAN_POINT ( 'NONE',  ( 0.3996062992125985480, 0.1070741851644054637, -0.1246719160104987068 ) ) ;
#62895=CARTESIAN_POINT ( 'NONE',  ( -0.1070741851644056997, 0.3996062992125984925, -2.445538057742782101 ) ) ;
#62900=CARTESIAN_POINT ( 'NONE',  ( -0.1998031496062994683, 0.3460692066303958092, -2.217847769028871596 ) ) ;
#62901=CARTESIAN_POINT ( 'NONE',  ( -0.1058382717557497937, -0.3949938075777411628, -1.646981627296588035 ) ) ;
#62902=CARTESIAN_POINT ( 'NONE',  ( -0.1998031496062991907, -0.3460692066303959757, -2.900262467191600635 ) ) ;
#62904=CARTESIAN_POINT ( 'NONE',  ( 0.3917322834645670104, 2.398668435337828261E-17, -0.5826771653543306728 ) ) ;
#62908=EDGE_CURVE ( 'NONE', #48835, #59512, #19780, .T. ) ;
#62909=CARTESIAN_POINT ( 'NONE',  ( -0.3420746716998662729, 0.1974969037888702206, -2.622703412073491336 ) ) ;
#62914=CARTESIAN_POINT ( 'NONE',  ( 0.4091458600556404646, -0.2362204724409448231, -2.782152230971128848 ) ) ;
#62915=CARTESIAN_POINT ( 'NONE',  ( -0.1070741851644051862, -0.3996062992125987146, -2.119422572178477626 ) ) ;
#62922=CARTESIAN_POINT ( 'NONE',  ( -0.2867679344610365999, 0.2867679344610364889, -0.2618110236220473341 ) ) ;
#62928=CARTESIAN_POINT ( 'NONE',  ( -0.2867679344610365999, 0.2867679344610364889, -0.5767716535433071723 ) ) ;
#62929=CARTESIAN_POINT ( 'NONE',  ( 0.3917322834645670104, 2.398668435337828261E-17, -1.370078740157480324 ) ) ;
#62930=( BOUNDED_CURVE ( )  B_SPLINE_CURVE ( 2, ( #17644, #3766, #43276, #68973, #11323, #82032, #75713, #18054, #43687, #80797, #23114, #32737, #20119 ),
 .UNSPECIFIED., .F., .F. ) 
 B_SPLINE_CURVE_WITH_KNOTS ( ( 3, 2, 2, 2, 2, 2, 3 ),
 ( 0.3875000000000000111, 0.3916666666666666630, 0.3958333333333333148, 0.4000000000000000222, 0.4041666666666667296, 0.4083333333333333814, 0.4125000000000000333 ),
 .UNSPECIFIED. ) 
 CURVE ( )  GEOMETRIC_REPRESENTATION_ITEM ( )  RATIONAL_B_SPLINE_CURVE ( ( 1.000000000000000000, 0.9659258262890683122, 1.000000000000000000, 0.9659258262890683122, 1.000000000000000000, 0.9659258262890683122, 1.000000000000000000, 0.9659258262890683122, 1.000000000000000000, 0.9659258262890683122, 1.000000000000000000, 0.9659258262890678681, 1.000000000000000444 ) ) 
 REPRESENTATION_ITEM ( '' )  );
#62931=CARTESIAN_POINT ( 'NONE',  ( -0.3917322834645671215, 0.1049643490035301469, -2.702099737532808632 ) ) ;
#62934=CARTESIAN_POINT ( 'NONE',  ( 0.3949938075777409963, 2.418639510665530435E-17, -2.795275590551181022 ) ) ;
#62938=CARTESIAN_POINT ( 'NONE',  ( -0.1070741851644056997, 0.3996062992125986035, -1.266404199475065440 ) ) ;
#62943=CARTESIAN_POINT ( 'NONE',  ( -0.3392501089628019995, 0.1958661417322832277, -0.2683727034120735877 ) ) ;
#62953=CARTESIAN_POINT ( 'NONE',  ( 0.4724409448818898682, 2.892866454678787531E-17, -2.007874015748031482 ) ) ;
#62963=CARTESIAN_POINT ( 'NONE',  ( -0.3917322834645668994, -0.1049643490035306742, -0.4409255661079247157 ) ) ;
#62965=CARTESIAN_POINT ( 'NONE',  ( 0.1049643490035303689, 0.3917322834645670104, -0.7080052493438320216 ) ) ;
#62970=CARTESIAN_POINT ( 'NONE',  ( 0.3392501089628018329, 0.1958661417322835607, -2.643044619422571628 ) ) ;
#62973=CARTESIAN_POINT ( 'NONE',  ( 5.785732909357575061E-17, -0.4724409448818898682, -0.7854330708661416693 ) ) ;
#62985=CARTESIAN_POINT ( 'NONE',  ( -0.1070741851644056997, 0.3996062992125984925, -2.130577427821522374 ) ) ;
#62993=CARTESIAN_POINT ( 'NONE',  ( 0.1998031496062994128, -0.3460692066303957537, -0.6410761154855643129 ) ) ;
#62994=CARTESIAN_POINT ( 'NONE',  ( 4.893765752498283924E-17, -0.3996062992125986035, -0.8661417322834645827 ) ) ;
#62995=CARTESIAN_POINT ( 'NONE',  ( -0.3420746716998659953, -0.1974969037888706647, -0.3674540682414698667 ) ) ;
#63001=CARTESIAN_POINT ( 'NONE',  ( 0.3420746716998660508, -0.1974969037888704149, -1.126640419947506633 ) ) ;
#63006=CARTESIAN_POINT ( 'NONE',  ( -0.4724409448818895907, -0.1265901696524993070, -1.778215223097112663 ) ) ;
#63007=CARTESIAN_POINT ( 'NONE',  ( -0.2925321140481932369, 0.2925321140481931814, -2.696850393700787052 ) ) ;
#63009=EDGE_CURVE ( 'NONE', #2500, #58583, #48283, .T. ) ;
#63021=CARTESIAN_POINT ( 'NONE',  ( -0.2867679344610365999, 0.2867679344610364889, -1.586614173228346747 ) ) ;
#63024=CARTESIAN_POINT ( 'NONE',  ( -0.2891555358219908833, -0.2891555358219912164, -1.476377952755905332 ) ) ;
#63029=CARTESIAN_POINT ( 'NONE',  ( 0.2925321140481932369, 0.2925321140481932369, 0.01968503937007873641 ) ) ;
#63036=CARTESIAN_POINT ( 'NONE',  ( 0.3917322834645670104, 2.398668435337828261E-17, -0.04527559055118119541 ) ) ;
#63042=CARTESIAN_POINT ( 'NONE',  ( 4.893765752498283924E-17, -0.3996062992125986035, -1.968503937007873850 ) ) ;
#63044=CARTESIAN_POINT ( 'NONE',  ( -0.1070741851644051862, -0.3996062992125986590, -1.566272965879265344 ) ) ;
#63048=CARTESIAN_POINT ( 'NONE',  ( 0.2362204724409451007, -0.4091458600556402980, -0.5643044619422572516 ) ) ;
#63049=ADVANCED_FACE ( 'NONE', ( #48478 ), #41751, .T. ) ;
#63050=CARTESIAN_POINT ( 'NONE',  ( 0.2017716535433070613, -0.2017716535433070890, -0.3937007874015748254 ) ) ;
#63051=CARTESIAN_POINT ( 'NONE',  ( -0.3392501089628019995, 0.1958661417322832277, -2.788057742782152459 ) ) ;
#63057=CARTESIAN_POINT ( 'NONE',  ( 0.3458507752293908943, 0.3458507752293908943, -2.576771653543307394 ) ) ;
#63060=CARTESIAN_POINT ( 'NONE',  ( 0.3949938075777409963, 2.418639510665530743E-17, -2.399606299212599048 ) ) ;
#63082=CARTESIAN_POINT ( 'NONE',  ( 0.1998031496062994128, -0.3460692066303957537, -0.7985564304461942875 ) ) ;
#63083=CARTESIAN_POINT ( 'NONE',  ( 0.1049643490035304938, -0.3917322834645669549, -2.059711286089238591 ) ) ;
#63099=CARTESIAN_POINT ( 'NONE',  ( 0.2867679344610365999, 0.2867679344610365999, -1.797244094488188892 ) ) ;
#63104=CARTESIAN_POINT ( 'NONE',  ( 0.3996062992125985480, 2.446882876249141654E-17, -2.714566929133858331 ) ) ;
#63107=CARTESIAN_POINT ( 'NONE',  ( 4.893765752498283924E-17, -0.3996062992125986035, -0.8661417322834645827 ) ) ;
#63109=CARTESIAN_POINT ( 'NONE',  ( 0.3392501089628018329, 0.1958661417322835607, -2.643044619422571628 ) ) ;
#63121=CARTESIAN_POINT ( 'NONE',  ( -0.3917322834645669549, -0.1049643490035306603, -2.650262467191601079 ) ) ;
#63124=CARTESIAN_POINT ( 'NONE',  ( -0.1974969037888703871, -0.3420746716998661063, -0.3805774278215224293 ) ) ;
#63131=CARTESIAN_POINT ( 'NONE',  ( 0.1958661417322834775, 0.3392501089628018884, -1.715898580873702617 ) ) ;
#63133=CARTESIAN_POINT ( 'NONE',  ( -0.3392501089628017219, -0.1958661417322836718, -2.814304461942257252 ) ) ;
#63138=CARTESIAN_POINT ( 'NONE',  ( 0.2925321140481932369, -0.2925321140481932369, -1.043307086614173151 ) ) ;
#63140=CARTESIAN_POINT ( 'NONE',  ( -0.1070741851644051862, -0.3996062992125986590, -0.3064304461942257141 ) ) ;
#63142=CARTESIAN_POINT ( 'NONE',  ( 0.3996062992125986590, -0.1070741851644053111, -2.316272965879265122 ) ) ;
#63143=CARTESIAN_POINT ( 'NONE',  ( 0.2867679344610365999, 0.2867679344610365999, -1.639763779527558807 ) ) ;
#63147=CARTESIAN_POINT ( 'NONE',  ( 0.1265901696524989462, 0.4724409448818897572, -1.015091863517060267 ) ) ;
#63150=CARTESIAN_POINT ( 'NONE',  ( 0.1058382717557499880, 0.3949938075777409408, -1.172572178477690574 ) ) ;
#63152=CARTESIAN_POINT ( 'NONE',  ( -0.4724409448818898682, -8.678599364036362592E-17, -1.061023622047243986 ) ) ;
#63163=CARTESIAN_POINT ( 'NONE',  ( -0.2925321140481930149, -0.2925321140481933480, -1.868110236220472675 ) ) ;
#63177=CARTESIAN_POINT ( 'NONE',  ( 0.3917322834645670104, -0.1049643490035303411, -0.8261154855643043637 ) ) ;
#63185=FACE_OUTER_BOUND ( 'NONE', #5041, .T. ) ;
#63195=FACE_OUTER_BOUND ( 'NONE', #44142, .T. ) ;
#63198=CARTESIAN_POINT ( 'NONE',  ( 0.4091458600556404646, -0.2362204724409448231, -0.2624671916010498651 ) ) ;
#63200=CARTESIAN_POINT ( 'NONE',  ( -0.1974969037888703871, -0.3420746716998661063, -2.900262467191600635 ) ) ;
#63203=CARTESIAN_POINT ( 'NONE',  ( -0.1049643490035302024, -0.3917322834645671215, -1.324146981627296826 ) ) ;
#63206=CARTESIAN_POINT ( 'NONE',  ( -0.1265901696524993347, 0.4724409448818895907, -2.683727034120735322 ) ) ;
#63213=CARTESIAN_POINT ( 'NONE',  ( -0.3917322834645669549, -7.196005306013483243E-17, -0.7493245162391581893 ) ) ;
#63220=CARTESIAN_POINT ( 'NONE',  ( 0.2867679344610366554, 0.2867679344610366554, -1.866817216044307060 ) ) ;
#63227=CARTESIAN_POINT ( 'NONE',  ( 0.2867679344610365999, 0.2867679344610365999, -1.482283464566929387 ) ) ;
#63236=CARTESIAN_POINT ( 'NONE',  ( -0.2867679344610364334, -0.2867679344610367109, -2.570866141732283339 ) ) ;
#63237=ORIENTED_EDGE ( 'NONE', *, *, #31645, .F. ) ;
#63243=CARTESIAN_POINT ( 'NONE',  ( -0.1049643490035307020, 0.3917322834645669549, -1.036089238845144589 ) ) ;
#63244=CARTESIAN_POINT ( 'NONE',  ( -0.4091458600556405756, 0.2362204724409446288, 0.05446194225721784354 ) ) ;
#63246=CARTESIAN_POINT ( 'NONE',  ( -0.1058382717557503072, 0.3949938075777408852, 0.07414698162729657649 ) ) ;
#63255=CARTESIAN_POINT ( 'NONE',  ( -0.2925321140481930149, -0.2925321140481933480, -0.4507874015748031815 ) ) ;
#63257=CARTESIAN_POINT ( 'NONE',  ( -0.3392501089628017219, -0.1958661417322836718, -0.2020997375328083545 ) ) ;
#63259=CARTESIAN_POINT ( 'NONE',  ( 0.000000000000000000, 0.000000000000000000, -2.755905511811024056 ) ) ;
#63272=CARTESIAN_POINT ( 'NONE',  ( 0.3917322834645670659, -0.1049643490035303273, -0.8956886071204221977 ) ) ;
#63277=CARTESIAN_POINT ( 'NONE',  ( -0.4724409448818899238, 0.1265901696524986686, -2.471784776902887337 ) ) ;
#63293=ORIENTED_EDGE ( 'NONE', *, *, #32000, .T. ) ;
#63298=CARTESIAN_POINT ( 'NONE',  ( -9.787531504996567848E-17, 0.3996062992125986035, -0.3149606299212598381 ) ) ;
#63299=CARTESIAN_POINT ( 'NONE',  ( -9.787531504996566615E-17, 0.3996062992125985480, -2.753937007874015741 ) ) ;
#63304=CARTESIAN_POINT ( 'NONE',  ( 0.1998031496062992740, 0.3460692066303959757, -2.349081364829396446 ) ) ;
#63305=CARTESIAN_POINT ( 'NONE',  ( -0.3949938075777409408, -0.1058382717557502933, -1.463254593175853158 ) ) ;
#63306=CARTESIAN_POINT ( 'NONE',  ( -0.1070741851644056997, 0.3996062992125986035, -2.841207349081364963 ) ) ;
#63308=CARTESIAN_POINT ( 'NONE',  ( -0.2867679344610366554, 0.2867679344610365444, -0.4842519685039368693 ) ) ;
#63311=CARTESIAN_POINT ( 'NONE',  ( -0.3949938075777408852, -0.1058382717557502933, -2.642388451443569597 ) ) ;
#63316=CARTESIAN_POINT ( 'NONE',  ( -0.1265901696524993347, 0.4724409448818895907, -2.683727034120735322 ) ) ;
#63317=CARTESIAN_POINT ( 'NONE',  ( 0.1998031496062994405, -0.3460692066303958092, -2.296587926509186417 ) ) ;
#63323=CARTESIAN_POINT ( 'NONE',  ( 0.3392501089628018884, -0.1958661417322834220, -0.03215223097112869521 ) ) ;
#63331=CARTESIAN_POINT ( 'NONE',  ( 0.2867679344610365999, 0.2867679344610365999, -0.5374015748031496509 ) ) ;
#63332=CARTESIAN_POINT ( 'NONE',  ( 0.1049643490035304938, -0.3917322834645669549, -1.337270341207349000 ) ) ;
#63333=CARTESIAN_POINT ( 'NONE',  ( -0.3392501089628019995, 0.1958661417322832277, -2.853018372703412187 ) ) ;
#63336=CARTESIAN_POINT ( 'NONE',  ( -0.2925321140481930704, -0.2925321140481933480, -0.05905511811023622659 ) ) ;
#63340=CARTESIAN_POINT ( 'NONE',  ( 0.1998031496062992740, 0.3460692066303959757, -1.246719160104986734 ) ) ;
#63345=CARTESIAN_POINT ( 'NONE',  ( 0.2867679344610365999, -0.2867679344610365444, -0.3405511811023621549 ) ) ;
#63355=CARTESIAN_POINT ( 'NONE',  ( 0.3458507752293908943, 0.3458507752293908943, -2.027559055118109743 ) ) ;
#63362=CARTESIAN_POINT ( 'NONE',  ( 5.785732909357575061E-17, -0.4724409448818898682, -2.675196850393700920 ) ) ;
#63365=CARTESIAN_POINT ( 'NONE',  ( -0.1958661417322836440, 0.3392501089628016664, -0.4081171671577935034 ) ) ;
#63367=CARTESIAN_POINT ( 'NONE',  ( -0.1958661417322834220, -0.3392501089628018884, -0.7801837270341208663 ) ) ;
#63372=CARTESIAN_POINT ( 'NONE',  ( 0.1958661417322836440, -0.3392501089628017219, -2.918635170603674389 ) ) ;
#63375=CARTESIAN_POINT ( 'NONE',  ( -0.2362204724409451284, 0.4091458600556402425, -1.034776902887139194 ) ) ;
#63387=ORIENTED_EDGE ( 'NONE', *, *, #50646, .F. ) ;
#63388=CARTESIAN_POINT ( 'NONE',  ( 0.3996062992125985480, 2.446882876249141654E-17, -2.084645669291338432 ) ) ;
#63391=CARTESIAN_POINT ( 'NONE',  ( -0.2925321140481932369, 0.2925321140481931259, -1.513779527559055094 ) ) ;
#63395=CARTESIAN_POINT ( 'NONE',  ( -0.2017716535433071445, -0.2017716535433071445, -0.3937007874015748254 ) ) ;
#63397=CARTESIAN_POINT ( 'NONE',  ( -0.3996062992125985480, -7.340648628747423112E-17, -0.5885826771653542844 ) ) ;
#63398=CARTESIAN_POINT ( 'NONE',  ( 0.3996062992125986590, -0.1070741851644053111, -1.056430446194225992 ) ) ;
#63399=CARTESIAN_POINT ( 'NONE',  ( 0.3949938075777411073, -0.1058382717557499464, -0.2690288713910761742 ) ) ;
#63400=CARTESIAN_POINT ( 'NONE',  ( 0.3790285851608848899, 0.1011035889004421734, -1.220472440944882164 ) ) ;
#63405=CARTESIAN_POINT ( 'NONE',  ( -9.674558042662122972E-17, 0.3949938075777409963, -1.494094488188976388 ) ) ;
#63411=CARTESIAN_POINT ( 'NONE',  ( 0.3458507752293908943, -0.3458507752293908943, -1.515748031496062742 ) ) ;
#63412=CARTESIAN_POINT ( 'NONE',  ( -0.3460692066303958092, -0.1998031496062994683, -2.572178477690288734 ) ) ;
#63427=CARTESIAN_POINT ( 'NONE',  ( -0.1958661417322836718, 0.3392501089628017219, -1.422572178477690574 ) ) ;
#63430=CARTESIAN_POINT ( 'NONE',  ( -0.1058382717557503211, 0.3949938075777409408, -1.581364829396325389 ) ) ;
#63435=CARTESIAN_POINT ( 'NONE',  ( 0.3996062992125986035, 0.1070741851644054776, -0.2821522309711286258 ) ) ;
#63448=CARTESIAN_POINT ( 'NONE',  ( 4.893765752498283924E-17, -0.3996062992125986035, -2.125984251968504157 ) ) ;
#63451=CARTESIAN_POINT ( 'NONE',  ( 0.1998031496062992463, 0.3460692066303959202, -1.638451443569553634 ) ) ;
#63457=CARTESIAN_POINT ( 'NONE',  ( -0.4724409448818895907, -0.1265901696524993070, -0.6758530183727035068 ) ) ;
#63460=CARTESIAN_POINT ( 'NONE',  ( 4.797336870675656522E-17, -0.3917322834645670104, -0.07086614173228342195 ) ) ;
#63462=CARTESIAN_POINT ( 'NONE',  ( -0.3917322834645671215, 0.1049643490035301469, -2.007217847769029007 ) ) ;
#63466=CARTESIAN_POINT ( 'NONE',  ( -0.4724409448818899238, 0.1265901696524986686, -2.629265091863517423 ) ) ;
#63469=CARTESIAN_POINT ( 'NONE',  ( 0.3949938075777409963, 2.418639510665530743E-17, -2.242125984251968518 ) ) ;
#63490=CARTESIAN_POINT ( 'NONE',  ( 0.3460692066303959202, -0.1998031496062991630, -0.6541994750656167090 ) ) ;
#63491=CARTESIAN_POINT ( 'NONE',  ( 0.3392501089628018329, 0.1958661417322835607, -2.263123359580052618 ) ) ;
#63501=CARTESIAN_POINT ( 'NONE',  ( 0.4724409448818898682, 2.892866454678787531E-17, -1.062992125984252079 ) ) ;
#63503=CARTESIAN_POINT ( 'NONE',  ( -0.1958661417322833942, -0.3392501089628018884, -1.952119053314647523 ) ) ;
#63511=CARTESIAN_POINT ( 'NONE',  ( -0.1049643490035302024, -0.3917322834645671215, -2.046587926509185973 ) ) ;
#63512=CARTESIAN_POINT ( 'NONE',  ( -0.05722014593895823065, 0.3876764156950353035, -1.220472440944881720 ) ) ;
#63516=CARTESIAN_POINT ( 'NONE',  ( -9.787531504996566615E-17, 0.3996062992125985480, -2.753937007874015741 ) ) ;
#63518=CARTESIAN_POINT ( 'NONE',  ( -0.3996062992125987146, 0.1070741851644051862, -0.8202099737532806412 ) ) ;
#63520=CARTESIAN_POINT ( 'NONE',  ( -0.3917322834645670104, -7.196005306013484475E-17, -2.551181102362204633 ) ) ;
#63532=CARTESIAN_POINT ( 'NONE',  ( -0.3917322834645671215, 0.1049643490035301469, -0.1824146981627296216 ) ) ;
#63535=CARTESIAN_POINT ( 'NONE',  ( -0.3949938075777409963, -7.255918531996591613E-17, -0.3543307086614174151 ) ) ;
#63542=CARTESIAN_POINT ( 'NONE',  ( 0.1049643490035304799, -0.3917322834645670104, -1.499363147802836860 ) ) ;
#63544=CARTESIAN_POINT ( 'NONE',  ( -0.2867679344610365999, 0.2867679344610364889, -2.781496062992125040 ) ) ;
#63548=CARTESIAN_POINT ( 'NONE',  ( 0.2925321140481932369, -0.2925321140481932369, -0.7283464566929134243 ) ) ;
#63550=CARTESIAN_POINT ( 'NONE',  ( 0.3460692066303959202, -0.1998031496062991630, -0.4967191601049869010 ) ) ;
#63551=CARTESIAN_POINT ( 'NONE',  ( -0.1070741851644051862, -0.3996062992125986590, 0.008530183727034094596 ) ) ;
#63553=CARTESIAN_POINT ( 'NONE',  ( -0.2925321140481930704, -0.2925321140481933480, -2.893700787401574992 ) ) ;
#63555=CARTESIAN_POINT ( 'NONE',  ( -0.3392501089628017219, -0.1958661417322836718, -1.711942257217847763 ) ) ;
#63560=CARTESIAN_POINT ( 'NONE',  ( -0.3458507752293906723, -0.3458507752293910609, -1.710629921259842812 ) ) ;
#63564=CARTESIAN_POINT ( 'NONE',  ( 0.2891555358219910499, 0.2891555358219910499, -0.8444881889763782290 ) ) ;
#63573=CARTESIAN_POINT ( 'NONE',  ( 0.3460692066303959202, -0.1998031496062991630, -1.914041994750656395 ) ) ;
#63578=ADVANCED_FACE ( 'NONE', ( #50533, #76237 ), #19390, .T. ) ;
#63589=CARTESIAN_POINT ( 'NONE',  ( -0.1049643490035302024, -0.3917322834645671215, -0.7867454068241470644 ) ) ;
#63609=CARTESIAN_POINT ( 'NONE',  ( -0.1049643490035307020, 0.3917322834645669549, -2.045931758530183497 ) ) ;
#63612=CARTESIAN_POINT ( 'NONE',  ( 0.2362204724409451007, -0.4091458600556402980, -0.2493438320209973857 ) ) ;
#63613=CARTESIAN_POINT ( 'NONE',  ( 0.2891555358219910499, -0.2891555358219909944, -2.775590551181102317 ) ) ;
#63616=CARTESIAN_POINT ( 'NONE',  ( 0.1958661417322834775, 0.3392501089628018884, -1.553805774278215202 ) ) ;
#63618=CARTESIAN_POINT ( 'NONE',  ( -0.4724409448818898682, -8.678599364036362592E-17, -2.874015748031495843 ) ) ;
#63625=CARTESIAN_POINT ( 'NONE',  ( -0.2867679344610364334, -0.2867679344610368219, -0.9264898705698668691 ) ) ;
#63632=CARTESIAN_POINT ( 'NONE',  ( -9.594673741351313045E-17, 0.3917322834645670659, -2.043982570375014962 ) ) ;
#63639=CARTESIAN_POINT ( 'NONE',  ( 0.1958661417322836440, -0.3392501089628017219, -1.278871391076115582 ) ) ;
#63644=CARTESIAN_POINT ( 'NONE',  ( -0.002049465651541999486, 0.3981765293560903807, -3.148631409696656626E-18 ) ) ;
#63648=CARTESIAN_POINT ( 'NONE',  ( 0.3917322834645670104, 2.398668435337828261E-17, -2.787401574803149096 ) ) ;
#63655=CARTESIAN_POINT ( 'NONE',  ( -0.3392501089628017219, -0.1958661417322836718, -1.239501312335958172 ) ) ;
#63656=CARTESIAN_POINT ( 'NONE',  ( 0.4724409448818897572, -0.1265901696524988906, -0.1883202099737532054 ) ) ;
#63659=CARTESIAN_POINT ( 'NONE',  ( -0.3949938075777411073, 0.1058382717557497660, 0.2053805774278214813 ) ) ;
#63669=CARTESIAN_POINT ( 'NONE',  ( -0.3460692066303957537, -0.1998031496062994405, -0.4442257217847768724 ) ) ;
#63671=CARTESIAN_POINT ( 'NONE',  ( 0.3392501089628018329, 0.1958661417322835607, -0.4383202099737532609 ) ) ;
#63687=CARTESIAN_POINT ( 'NONE',  ( -0.2867679344610365444, -0.2867679344610367664, -1.000675483760841811 ) ) ;
#63691=CARTESIAN_POINT ( 'NONE',  ( -0.4091458600556405756, 0.2362204724409446288, -2.307742782152230721 ) ) ;
#63708=CARTESIAN_POINT ( 'NONE',  ( 0.1070741851644054915, -0.3996062992125985480, -0.2427821522309711599 ) ) ;
#63709=CARTESIAN_POINT ( 'NONE',  ( -0.2925321140481930149, -0.2925321140481933480, -2.655511811023622215 ) ) ;
#63714=CARTESIAN_POINT ( 'NONE',  ( 0.1070741851644054915, -0.3996062992125986035, -2.132545931758530244 ) ) ;
#63715=CARTESIAN_POINT ( 'NONE',  ( 4.837279021331060870E-17, -0.3949938075777409963, -1.338582677165354173 ) ) ;
#63716=CARTESIAN_POINT ( 'NONE',  ( 0.3996062992125986035, 0.1070741851644054776, -2.801837270341207553 ) ) ;
#63719=CARTESIAN_POINT ( 'NONE',  ( 0.3917322834645670104, 2.398668435337828261E-17, -0.7401574803149605364 ) ) ;
#63722=CARTESIAN_POINT ( 'NONE',  ( -0.1058382717557503072, 0.3949938075777408852, -2.760498687664042716 ) ) ;
#63726=CARTESIAN_POINT ( 'NONE',  ( -0.3458507752293909498, 0.3458507752293907833, -2.696850393700787052 ) ) ;
#63727=CARTESIAN_POINT ( 'NONE',  ( -0.1070741851644056997, 0.3996062992125986035, -2.368766404199475151 ) ) ;
#63734=CARTESIAN_POINT ( 'NONE',  ( -0.3392501089628017219, -0.1958661417322836718, 0.02034120734908127781 ) ) ;
#63742=CARTESIAN_POINT ( 'NONE',  ( 0.3917322834645670104, 2.398668435337828261E-17, -0.5177165354330709457 ) ) ;
#63743=CARTESIAN_POINT ( 'NONE',  ( 0.1958661417322836440, -0.3392501089628017219, -1.343832020997375531 ) ) ;
#63744=CARTESIAN_POINT ( 'NONE',  ( -9.594673741351313045E-17, 0.3917322834645670104, -2.826771653543306506 ) ) ;
#63746=CARTESIAN_POINT ( 'NONE',  ( -0.1998031496062994683, 0.3460692066303958092, -0.1706036745406824540 ) ) ;
#63750=CARTESIAN_POINT ( 'NONE',  ( -0.3460692066303960868, 0.1998031496062990242, -1.601049868766404094 ) ) ;
#63754=CARTESIAN_POINT ( 'NONE',  ( 0.2867679344610365999, -0.2867679344610365444, -0.8129921259842518566 ) ) ;
#63763=CARTESIAN_POINT ( 'NONE',  ( 0.4091458600556404646, -0.2362204724409448231, -2.152230971128608950 ) ) ;
#63766=EDGE_CURVE ( 'NONE', #58800, #80266, #56870, .T. ) ;
#63774=CARTESIAN_POINT ( 'NONE',  ( 0.2867679344610365999, 0.2867679344610365999, -1.005230028050182245 ) ) ;
#63777=CARTESIAN_POINT ( 'NONE',  ( 0.1049643490035304799, -0.3917322834645669549, -0.6423884514435697080 ) ) ;
#63783=CARTESIAN_POINT ( 'NONE',  ( -0.1958661417322836995, 0.3392501089628017219, 0.1476184794937513700 ) ) ;
#63786=CARTESIAN_POINT ( 'NONE',  ( 0.3458507752293908943, 0.3458507752293908943, -1.001968503937007871 ) ) ;
#63794=DIRECTION ( 'NONE',  ( 0.000000000000000000, 0.000000000000000000, 1.000000000000000000 ) ) ;
#63799=CARTESIAN_POINT ( 'NONE',  ( 0.3996062992125984925, 0.1070741851644054637, -2.406167979002624246 ) ) ;
#63803=CARTESIAN_POINT ( 'NONE',  ( -0.1998031496062991630, -0.3460692066303959202, -1.244750656167979086 ) ) ;
#63809=CARTESIAN_POINT ( 'NONE',  ( -0.1070741851644051862, -0.3996062992125986035, -0.4639107611548556331 ) ) ;
#63810=CARTESIAN_POINT ( 'NONE',  ( -0.3996062992125986035, -7.340648628747425578E-17, -0.8267716535433070613 ) ) ;
#63811=CARTESIAN_POINT ( 'NONE',  ( 0.3420746716998660508, -0.1974969037888703871, -0.1049868766404199877 ) ) ;
#63817=CARTESIAN_POINT ( 'NONE',  ( 0.1058382717557500852, -0.3949938075777408852, -1.264435695538058013 ) ) ;
#63822=CARTESIAN_POINT ( 'NONE',  ( -0.4724409448818898682, -8.678599364036362592E-17, -1.614173228346456712 ) ) ;
#63831=CARTESIAN_POINT ( 'NONE',  ( 0.2867679344610365999, 0.2867679344610365999, -2.107592232774591068 ) ) ;
#63838=CARTESIAN_POINT ( 'NONE',  ( 0.1049643490035304938, -0.3917322834645669549, -1.494750656167978642 ) ) ;
#63841=CARTESIAN_POINT ( 'NONE',  ( 0.1974969037888706369, -0.3420746716998659953, -1.666666666666666741 ) ) ;
#63846=CARTESIAN_POINT ( 'NONE',  ( -0.1998031496062994683, 0.3460692066303958092, -0.1706036745406823985 ) ) ;
#63854=CARTESIAN_POINT ( 'NONE',  ( -0.2867679344610365999, 0.2867679344610364889, -0.5767716535433071723 ) ) ;
#63861=CARTESIAN_POINT ( 'NONE',  ( -0.1998031496062994405, 0.3460692066303957537, -2.137139107611548905 ) ) ;
#63866=CARTESIAN_POINT ( 'NONE',  ( -0.3458507752293909498, 0.3458507752293907833, -0.6496062992125984925 ) ) ;
#63868=CARTESIAN_POINT ( 'NONE',  ( 0.3917322834645670104, -0.1049643490035303411, -0.1036745406824146343 ) ) ;
#63869=CARTESIAN_POINT ( 'NONE',  ( -0.3917322834645669549, -0.1049643490035306603, -2.177821522309711266 ) ) ;
#63873=CARTESIAN_POINT ( 'NONE',  ( -0.4724409448818895907, -0.1265901696524993070, -2.799868766404198794 ) ) ;
#63876=CARTESIAN_POINT ( 'NONE',  ( 0.3949938075777409963, 2.418639510665530743E-17, -2.084645669291338876 ) ) ;
#63884=CARTESIAN_POINT ( 'NONE',  ( 0.3392501089628018329, 0.1958661417322835607, -1.540682414698162805 ) ) ;
#63887=CARTESIAN_POINT ( 'NONE',  ( -0.2362204724409451284, 0.4091458600556402425, 0.06758530183727033680 ) ) ;
#63900=CARTESIAN_POINT ( 'NONE',  ( 0.3460692066303959202, -0.1998031496062991630, -1.284120734908136496 ) ) ;
#63902=CARTESIAN_POINT ( 'NONE',  ( 0.3917322834645670104, 2.398668435337828261E-17, -2.407480314960630086 ) ) ;
#63913=CARTESIAN_POINT ( 'NONE',  ( 0.3392501089628018884, -0.1958661417322833942, -2.306449761976065105 ) ) ;
#63920=CARTESIAN_POINT ( 'NONE',  ( 0.1958661417322834775, 0.3392501089628018884, -2.118766404199475151 ) ) ;
#63921=CARTESIAN_POINT ( 'NONE',  ( -0.3758920641862481538, 0.1123167701215816577, -1.220472440944881942 ) ) ;
#63926=CARTESIAN_POINT ( 'NONE',  ( 0.1070741851644053527, 0.3996062992125985480, -2.747375328083989210 ) ) ;
#63928=CARTESIAN_POINT ( 'NONE',  ( 0.3460692066303959757, -0.1998031496062991907, -1.207349081364829324 ) ) ;
#63930=CARTESIAN_POINT ( 'NONE',  ( 0.3917322834645670104, 2.398668435337828261E-17, -2.944881889763779181 ) ) ;
#63931=VERTEX_POINT ( 'NONE', #33695 ) ;
#63943=CARTESIAN_POINT ( 'NONE',  ( 0.1049643490035304938, -0.3917322834645669549, -0.2349081364829396223 ) ) ;
#63946=CARTESIAN_POINT ( 'NONE',  ( 4.837279021331060870E-17, -0.3949938075777409963, -0.7086614173228346081 ) ) ;
#63954=CARTESIAN_POINT ( 'NONE',  ( -0.1049643490035302301, -0.3917322834645671770, -1.643720103183414105 ) ) ;
#63956=CARTESIAN_POINT ( 'NONE',  ( -0.1958661417322834220, -0.3392501089628018884, -2.827427821522309426 ) ) ;
#63960=CARTESIAN_POINT ( 'NONE',  ( -0.1070741851644051862, -0.3996062992125987146, -1.017060367454067915 ) ) ;
#63962=CARTESIAN_POINT ( 'NONE',  ( -0.1070741851644051862, -0.3996062992125986590, -0.1489501312335958227 ) ) ;
#63963=CARTESIAN_POINT ( 'NONE',  ( 0.3460692066303959202, -0.1998031496062991630, -0.02427821522309713681 ) ) ;
#63965=CARTESIAN_POINT ( 'NONE',  ( 0.3460692066303959202, 0.1998031496062993295, -2.808398950131233640 ) ) ;
#63966=CARTESIAN_POINT ( 'NONE',  ( -0.1958661417322834220, -0.3392501089628018884, -1.882545931758530244 ) ) ;
#63972=CARTESIAN_POINT ( 'NONE',  ( -0.4091458600556402980, -0.2362204724409451284, -1.546587926509186639 ) ) ;
#63975=CARTESIAN_POINT ( 'NONE',  ( -0.3420746716998662729, 0.1974969037888702206, -1.047900262467191590 ) ) ;
#63985=CARTESIAN_POINT ( 'NONE',  ( -0.2925321140481932369, 0.2925321140481931259, -2.143700787401574548 ) ) ;
#63987=CARTESIAN_POINT ( 'NONE',  ( 0.3917322834645669549, 2.398668435337827645E-17, -1.772946563483252858 ) ) ;
#64000=CARTESIAN_POINT ( 'NONE',  ( 0.3392501089628018884, -0.1958661417322834220, -0.9770341207349081403 ) ) ;
#64002=VECTOR ( 'NONE', #41551, 39.37007874015748143 ) ;
#64026=CARTESIAN_POINT ( 'NONE',  ( -1.157146581871515012E-16, 0.4724409448818898682, -0.4724409448818898127 ) ) ;
#64027=CARTESIAN_POINT ( 'NONE',  ( 0.3996062992125986590, -0.1070741851644053111, -0.2690288713910760632 ) ) ;
#64030=CARTESIAN_POINT ( 'NONE',  ( 0.3917322834645669549, 0.1049643490035304660, -2.006561679790026531 ) ) ;
#64033=CARTESIAN_POINT ( 'NONE',  ( 0.4724409448818898682, 2.892866454678787531E-17, -2.952755905511811108 ) ) ;
#64040=CARTESIAN_POINT ( 'NONE',  ( 0.2867679344610365999, 0.2867679344610365999, -0.8477497130895521593 ) ) ;
#64047=CARTESIAN_POINT ( 'NONE',  ( -0.2867679344610365444, -0.2867679344610367664, -2.103037688485251522 ) ) ;
#64055=CARTESIAN_POINT ( 'NONE',  ( 0.3392501089628018329, 0.1958661417322835607, -1.318241469816273215 ) ) ;
#64060=CARTESIAN_POINT ( 'NONE',  ( -0.02500110683994623273, 0.3941128856533804847, 9.485496803828530434E-13 ) ) ;
#64073=CARTESIAN_POINT ( 'NONE',  ( -0.3458507752293906723, -0.3458507752293910609, -0.3740157480314960092 ) ) ;
#64074=CARTESIAN_POINT ( 'NONE',  ( -0.1958661417322834220, -0.3392501089628018884, -1.095144356955380704 ) ) ;
#64075=CARTESIAN_POINT ( 'NONE',  ( 0.1265901696524989462, 0.4724409448818897572, -0.2276902887139107545 ) ) ;
#64078=CARTESIAN_POINT ( 'NONE',  ( -0.3996062992125985480, -7.340648628747423112E-17, -2.793307086614173151 ) ) ;
#64084=CARTESIAN_POINT ( 'NONE',  ( -9.674558042662122972E-17, 0.3949938075777409963, -0.2342519685039370914 ) ) ;
#64092=CARTESIAN_POINT ( 'NONE',  ( 0.1070741851644053388, 0.3996062992125986035, -1.015091863517060267 ) ) ;
#64094=CARTESIAN_POINT ( 'NONE',  ( 0.3917322834645670104, -0.1049643490035303411, -0.2611548556430445256 ) ) ;
#64108=CARTESIAN_POINT ( 'NONE',  ( 0.3917322834645670659, 2.398668435337828261E-17, -0.9022502869104481737 ) ) ;
#64113=CARTESIAN_POINT ( 'NONE',  ( 0.3458507752293908943, -0.3458507752293908943, -2.537401574803149984 ) ) ;
#64131=CARTESIAN_POINT ( 'NONE',  ( -0.1070741851644051862, -0.3996062992125986590, -0.3871391076115485719 ) ) ;
#64132=CARTESIAN_POINT ( 'NONE',  ( -0.3996062992125984925, -0.1070741851644056858, -2.484908136482939955 ) ) ;
#64139=CARTESIAN_POINT ( 'NONE',  ( -0.2925321140481930704, -0.2925321140481933480, -2.263779527559055094 ) ) ;
#64140=CARTESIAN_POINT ( 'NONE',  ( 0.3420746716998659953, 0.1974969037888705536, -2.020997375328084100 ) ) ;
#64141=CARTESIAN_POINT ( 'NONE',  ( 0.1998031496062994405, -0.3460692066303958092, -2.926509186351706315 ) ) ;
#64143=CARTESIAN_POINT ( 'NONE',  ( -0.3917322834645669549, -0.1049643490035306603, -0.9829396325459317518 ) ) ;
#64146=CARTESIAN_POINT ( 'NONE',  ( 0.3949938075777408852, 0.1058382717557500435, -2.721128608923885306 ) ) ;
#64150=CARTESIAN_POINT ( 'NONE',  ( -0.2362204724409451284, 0.4091458600556402425, -2.847769028871391050 ) ) ;
#64151=CARTESIAN_POINT ( 'NONE',  ( 4.893765752498283924E-17, -0.3996062992125986035, -2.125984251968504157 ) ) ;
#64152=CARTESIAN_POINT ( 'NONE',  ( -0.3917322834645670104, -0.1049643490035307020, -0.9875521241807894146 ) ) ;
#64159=CARTESIAN_POINT ( 'NONE',  ( -0.3392501089628019995, 0.1958661417322832277, -0.2683727034120735877 ) ) ;
#64167=CARTESIAN_POINT ( 'NONE',  ( 0.2867679344610365999, -0.2867679344610365444, -0.6555118110236222151 ) ) ;
#64168=CARTESIAN_POINT ( 'NONE',  ( 0.3917322834645670104, -0.1049643490035303411, -1.678477690288713964 ) ) ;
#64169=CARTESIAN_POINT ( 'NONE',  ( 0.1049643490035303689, 0.3917322834645670104, -2.820209973753280419 ) ) ;
#64171=CARTESIAN_POINT ( 'NONE',  ( -0.1998031496062994683, 0.3460692066303958092, -0.01312335958005251234 ) ) ;
#64175=CARTESIAN_POINT ( 'NONE',  ( -9.787531504996567848E-17, 0.3996062992125986035, -1.417322834645669216 ) ) ;
#64180=CARTESIAN_POINT ( 'NONE',  ( -0.3392501089628017219, -0.1958661417322836718, -0.7670603674540683592 ) ) ;
#64188=CARTESIAN_POINT ( 'NONE',  ( 0.4091458600556404646, -0.2362204724409448231, -1.994750656167979086 ) ) ;
#64197=CARTESIAN_POINT ( 'NONE',  ( -0.3458507752293906723, -0.3458507752293910609, -2.655511811023621771 ) ) ;
#64200=CARTESIAN_POINT ( 'NONE',  ( -0.1958661417322836440, 0.3392501089628016664, -0.7230777970790532860 ) ) ;
#64202=CARTESIAN_POINT ( 'NONE',  ( -0.3917322834645669549, -0.1049643490035306603, -0.9179790026246720247 ) ) ;
#64207=CARTESIAN_POINT ( 'NONE',  ( -0.1958661417322836718, 0.3392501089628017219, -2.839895013123359568 ) ) ;
#64210=CARTESIAN_POINT ( 'NONE',  ( -0.3458507752293906723, -0.3458507752293910609, -1.238188976377952999 ) ) ;
#64222=CARTESIAN_POINT ( 'NONE',  ( 0.1998031496062994128, -0.3460692066303957537, -2.215879265091863726 ) ) ;
#64226=CARTESIAN_POINT ( 'NONE',  ( -0.3460692066303960313, 0.1998031496062989965, -1.362860892388451539 ) ) ;
#64232=CARTESIAN_POINT ( 'NONE',  ( -0.1070741851644057135, 0.3996062992125984925, -0.7132545931758530466 ) ) ;
#64233=CARTESIAN_POINT ( 'NONE',  ( 0.3996062992125986035, 2.446882876249141962E-17, -0.7480314960629921295 ) ) ;
#64234=CARTESIAN_POINT ( 'NONE',  ( 0.3949938075777409963, 2.418639510665530435E-17, -0.1181102362204724948 ) ) ;
#64240=CARTESIAN_POINT ( 'NONE',  ( -9.674558042662122972E-17, 0.3949938075777409963, -1.179133858267716661 ) ) ;
#64245=CARTESIAN_POINT ( 'NONE',  ( 5.785732909357575061E-17, -0.4724409448818898682, -1.496062992125984259 ) ) ;
#64247=CARTESIAN_POINT ( 'NONE',  ( -0.3996062992125986590, 0.1070741851644051862, -2.552493438320209140 ) ) ;
#64254=CARTESIAN_POINT ( 'NONE',  ( -0.1049643490035306742, 0.3917322834645668994, -1.976358636974066663 ) ) ;
#64260=CARTESIAN_POINT ( 'NONE',  ( 0.3917322834645670104, -0.1049643490035303411, -1.520997375328083656 ) ) ;
#64263=CARTESIAN_POINT ( 'NONE',  ( -0.1058382717557497937, -0.3949938075777411628, -1.804461942257217899 ) ) ;
#64268=CARTESIAN_POINT ( 'NONE',  ( 0.1070741851644054915, -0.3996062992125986035, -0.08530183727034119923 ) ) ;
#64274=CARTESIAN_POINT ( 'NONE',  ( 4.797336870675656522E-17, -0.3917322834645670104, -0.3208661417322835607 ) ) ;
#64280=EDGE_LOOP ( 'NONE', ( #12281, #29598, #30422, #27833 ) ) ;
#64281=CARTESIAN_POINT ( 'NONE',  ( -0.3460692066303957537, -0.1998031496062994405, -2.019028871391076230 ) ) ;
#64286=CARTESIAN_POINT ( 'NONE',  ( -0.3458507752293909498, 0.3458507752293907833, -0.8070866141732284671 ) ) ;
#64288=CARTESIAN_POINT ( 'NONE',  ( 0.3917322834645670104, -0.1049643490035303411, -0.2611548556430445256 ) ) ;
#64289=CARTESIAN_POINT ( 'NONE',  ( -0.1049643490035301885, -0.3917322834645671215, -2.046587926509185973 ) ) ;
#64293=CARTESIAN_POINT ( 'NONE',  ( 0.1265901696524990294, -0.4724409448818896462, -2.681758530183727895 ) ) ;
#64297=CARTESIAN_POINT ( 'NONE',  ( -0.1974969037888706924, 0.3420746716998658843, -2.609580052493438718 ) ) ;
#64305=CARTESIAN_POINT ( 'NONE',  ( 0.3392501089628018884, -0.1958661417322834220, -1.356955380577427928 ) ) ;
#64308=CARTESIAN_POINT ( 'NONE',  ( -0.1265901696524986964, -0.4724409448818899238, -0.1489501312335958227 ) ) ;
#64320=CARTESIAN_POINT ( 'NONE',  ( -0.1998031496062991630, -0.3460692066303959202, -1.087270341207349000 ) ) ;
#64321=CARTESIAN_POINT ( 'NONE',  ( 0.1958661417322834775, 0.3392501089628018884, -2.591207349081364519 ) ) ;
#64331=FACE_OUTER_BOUND ( 'NONE', #32879, .T. ) ;
#64332=CARTESIAN_POINT ( 'NONE',  ( -0.3917322834645671770, 0.1049643490035302024, -1.919310654364516200 ) ) ;
#64338=CARTESIAN_POINT ( 'NONE',  ( -0.3917322834645670104, -7.196005306013484475E-17, -1.856299212598425230 ) ) ;
#64346=CARTESIAN_POINT ( 'NONE',  ( 0.3996062992125986590, -0.1070741851644053111, -1.213910761154855189 ) ) ;
#64348=CARTESIAN_POINT ( 'NONE',  ( -0.1958661417322833942, -0.3392501089628018884, 0.09512504117354141087 ) ) ;
#64362=CARTESIAN_POINT ( 'NONE',  ( -0.1049643490035307020, 0.3917322834645669549, 0.001312335958005295946 ) ) ;
#64365=CARTESIAN_POINT ( 'NONE',  ( -0.2891555358219908833, -0.2891555358219912164, -0.5314960629921261503 ) ) ;
#64368=CARTESIAN_POINT ( 'NONE',  ( -0.4724409448818898682, -8.678599364036362592E-17, -1.218503937007874072 ) ) ;
#64372=CARTESIAN_POINT ( 'NONE',  ( -0.2867679344610365444, -0.2867679344610367664, -1.473116428642731401 ) ) ;
#64379=CARTESIAN_POINT ( 'NONE',  ( 0.3460692066303959202, 0.1998031496062993295, -1.076115485564304475 ) ) ;
#64381=CARTESIAN_POINT ( 'NONE',  ( -0.2925321140481930149, -0.2925321140481933480, -0.9232283464566929387 ) ) ;
#64382=CARTESIAN_POINT ( 'NONE',  ( 0.1070741851644053388, 0.3996062992125986035, -0.2276902887139107545 ) ) ;
#64384=CARTESIAN_POINT ( 'NONE',  ( -0.1070741851644051862, -0.3996062992125987146, -2.749343832020996636 ) ) ;
#64385=CARTESIAN_POINT ( 'NONE',  ( -0.3917322834645671215, 0.1049643490035301469, -1.534776902887139194 ) ) ;
#64391=CARTESIAN_POINT ( 'NONE',  ( 0.2362204724409451007, -0.4091458600556402980, -1.428477690288713964 ) ) ;
#64394=CARTESIAN_POINT ( 'NONE',  ( 0.3420746716998660508, 0.1974969037888705814, -1.310367454068241511 ) ) ;
#64404=CARTESIAN_POINT ( 'NONE',  ( -0.1070741851644056997, 0.3996062992125984925, -1.973097112860892510 ) ) ;
#64407=CARTESIAN_POINT ( 'NONE',  ( 0.3917322834645668994, 0.1049643490035304522, -1.622027928312648859 ) ) ;
#64418=FACE_OUTER_BOUND ( 'NONE', #14623, .T. ) ;
#64420=CARTESIAN_POINT ( 'NONE',  ( 0.1958661417322834775, 0.3392501089628018884, -0.8589238845144357981 ) ) ;
#64440=CARTESIAN_POINT ( 'NONE',  ( 0.1049643490035304799, -0.3917322834645669549, -2.439632545931758045 ) ) ;
#64443=CARTESIAN_POINT ( 'NONE',  ( -1.157146581871515012E-16, 0.4724409448818898682, -0.9448818897637796255 ) ) ;
#64444=CARTESIAN_POINT ( 'NONE',  ( -0.1070741851644056997, 0.3996062992125986035, -0.1640419947506562004 ) ) ;
#64447=CARTESIAN_POINT ( 'NONE',  ( 0.3917322834645670104, 2.398668435337828261E-17, -1.842519685039370136 ) ) ;
#64458=CARTESIAN_POINT ( 'NONE',  ( -0.3917322834645670659, 0.1049643490035301607, -1.215203781331021915 ) ) ;
#64465=CARTESIAN_POINT ( 'NONE',  ( -0.3917322834645670104, -0.1049643490035307020, -2.404874958826459075 ) ) ;
#64473=CARTESIAN_POINT ( 'NONE',  ( 0.3917322834645670104, 2.398668435337828261E-17, -1.935039370078740273 ) ) ;
#64477=CARTESIAN_POINT ( 'NONE',  ( 0.000000000000000000, 0.000000000000000000, -2.755905511811024056 ) ) ;
#64490=CARTESIAN_POINT ( 'NONE',  ( 0.4091458600556404646, -0.2362204724409448231, -0.1817585301837270351 ) ) ;
#64493=CARTESIAN_POINT ( 'NONE',  ( 0.3996062992125986035, -0.1070741851644052972, -2.708005249343832688 ) ) ;
#64498=CARTESIAN_POINT ( 'NONE',  ( 0.3420746716998660508, 0.1974969037888705814, 0.1069553805774278443 ) ) ;
#64505=CARTESIAN_POINT ( 'NONE',  ( -0.3996062992125985480, -7.340648628747423112E-17, -0.9035433070866141225 ) ) ;
#64508=CARTESIAN_POINT ( 'NONE',  ( -9.594673741351313045E-17, 0.3917322834645670104, -0.4645669291338582751 ) ) ;
#64523=CARTESIAN_POINT ( 'NONE',  ( -0.3973686378485497550, -0.03056273350765931207, -1.220472440944882386 ) ) ;
#64525=CARTESIAN_POINT ( 'NONE',  ( -0.4091458600556402980, -0.2362204724409451284, -2.491469816272966042 ) ) ;
#64537=EDGE_CURVE ( 'NONE', #54535, #5751, #2547, .T. ) ;
#64542=CARTESIAN_POINT ( 'NONE',  ( 0.1998031496062994405, -0.3460692066303958092, -0.2493438320209974135 ) ) ;
#64543=CARTESIAN_POINT ( 'NONE',  ( -0.1265901696524993347, 0.4724409448818896462, -1.185695538057742748 ) ) ;
#64548=CARTESIAN_POINT ( 'NONE',  ( 0.1998031496062994405, -0.3460692066303958092, -2.769028871391076230 ) ) ;
#64549=CARTESIAN_POINT ( 'NONE',  ( -0.3949938075777409963, -7.255918531996591613E-17, -1.771653543307086576 ) ) ;
#64550=CARTESIAN_POINT ( 'NONE',  ( -9.594673741351313045E-17, 0.3917322834645670104, -0.4645669291338582751 ) ) ;
#64552=CARTESIAN_POINT ( 'NONE',  ( -0.2867679344610364334, -0.2867679344610367109, -1.153543307086613900 ) ) ;
#64554=CARTESIAN_POINT ( 'NONE',  ( 0.2867679344610365999, 0.2867679344610365999, -1.232283464566929387 ) ) ;
#64556=CARTESIAN_POINT ( 'NONE',  ( 0.3917322834645668994, 0.1049643490035304522, 0.1102555362542800566 ) ) ;
#64561=CARTESIAN_POINT ( 'NONE',  ( -0.1265901696524993347, 0.4724409448818895907, -2.841207349081364963 ) ) ;
#64562=CARTESIAN_POINT ( 'NONE',  ( 0.2925321140481932369, -0.2925321140481932369, -2.460629921259842146 ) ) ;
#64563=CARTESIAN_POINT ( 'NONE',  ( -0.1049643490035302301, -0.3917322834645671770, -1.013798843340894207 ) ) ;
#64569=CARTESIAN_POINT ( 'NONE',  ( 0.2867679344610365999, 0.2867679344610365999, -0.06496062992125994917 ) ) ;
#64577=CARTESIAN_POINT ( 'NONE',  ( 0.3917322834645670104, -0.1049643490035303411, -0.5111548556430445256 ) ) ;
#64578=CARTESIAN_POINT ( 'NONE',  ( 0.1958661417322836440, -0.3392501089628017219, -1.816272965879265122 ) ) ;
#64579=CARTESIAN_POINT ( 'NONE',  ( 0.2867679344610365999, 0.2867679344610365999, -2.807086614173227357 ) ) ;
#64580=EDGE_CURVE ( 'NONE', #66690, #21828, #35356, .T. ) ;
#64582=CARTESIAN_POINT ( 'NONE',  ( -0.1070741851644056997, 0.3996062992125986035, -0.006561679790026264843 ) ) ;
#64586=CARTESIAN_POINT ( 'NONE',  ( -0.3996062992125986035, -7.340648628747425578E-17, -1.929133858267716439 ) ) ;
#64590=CARTESIAN_POINT ( 'NONE',  ( 0.3951562584566663539, 0.01150853369506588293, -1.929133858268277546 ) ) ;
#64591=CARTESIAN_POINT ( 'NONE',  ( 0.2867679344610365999, 0.2867679344610365999, -0.8523622047244096001 ) ) ;
#64602=CARTESIAN_POINT ( 'NONE',  ( -0.2017716535433071445, -0.2017716535433071445, -0.3937007874015748254 ) ) ;
#64605=ORIENTED_EDGE ( 'NONE', *, *, #53516, .F. ) ;
#64610=CARTESIAN_POINT ( 'NONE',  ( 0.1049643490035303689, 0.3917322834645668994, -0.8608730726696044444 ) ) ;
#64619=CARTESIAN_POINT ( 'NONE',  ( -0.3392501089628019995, 0.1958661417322832277, -2.853018372703412187 ) ) ;
#64622=CARTESIAN_POINT ( 'NONE',  ( -0.1265901696524986964, -0.4724409448818899238, -1.093832020997375087 ) ) ;
#64637=CARTESIAN_POINT ( 'NONE',  ( 0.3996062992125984925, 0.1070741851644054637, -2.563648293963254776 ) ) ;
#64641=CARTESIAN_POINT ( 'NONE',  ( -0.1070741851644051862, -0.3996062992125986590, -1.881233595800524849 ) ) ;
#64645=CARTESIAN_POINT ( 'NONE',  ( -0.1265901696524986964, -0.4724409448818899238, -0.07217847769028870597 ) ) ;
#64647=CARTESIAN_POINT ( 'NONE',  ( 0.3996062992125984925, 0.1070741851644054499, -0.5164041994750655507 ) ) ;
#64648=CARTESIAN_POINT ( 'NONE',  ( -0.2925321140481932924, 0.2925321140481931814, -0.9645669291338579976 ) ) ;
#64649=CARTESIAN_POINT ( 'NONE',  ( -0.1058382717557497937, -0.3949938075777411628, -0.8595800524934383846 ) ) ;
#64655=CARTESIAN_POINT ( 'NONE',  ( -0.1974969037888706924, 0.3420746716998658843, -1.349737532808398921 ) ) ;
#64660=CARTESIAN_POINT ( 'NONE',  ( 0.4724409448818898682, 2.892866454678787531E-17, -1.692913385826771533 ) ) ;
#64661=CARTESIAN_POINT ( 'NONE',  ( 0.1070741851644054915, -0.3996062992125985480, -2.604986876640420057 ) ) ;
#64662=VERTEX_POINT ( 'NONE', #69815 ) ;
#64668=CARTESIAN_POINT ( 'NONE',  ( 0.1958661417322836162, -0.3392501089628018329, -2.061660474244408014 ) ) ;
#64675=CARTESIAN_POINT ( 'NONE',  ( 0.3392501089628018884, -0.1958661417322834220, -1.356955380577427928 ) ) ;
#64678=CARTESIAN_POINT ( 'NONE',  ( 0.1058382717557499880, 0.3949938075777411073, -1.725721784776902856 ) ) ;
#64683=CARTESIAN_POINT ( 'NONE',  ( 0.1998031496062992740, 0.3460692066303959757, 0.01312335958005248458 ) ) ;
#64688=CARTESIAN_POINT ( 'NONE',  ( -0.1958661417322836718, 0.3392501089628017219, 0.2171916010498686767 ) ) ;
#64691=CARTESIAN_POINT ( 'NONE',  ( -9.594673741351313045E-17, 0.3917322834645670104, -0.3996062992125985480 ) ) ;
#64698=CARTESIAN_POINT ( 'NONE',  ( -0.1070741851644051862, -0.3996062992125986590, -2.196194225721784576 ) ) ;
#64703=CARTESIAN_POINT ( 'NONE',  ( 5.785732909357575061E-17, -0.4724409448818898682, -0.7086614173228346081 ) ) ;
#64705=CARTESIAN_POINT ( 'NONE',  ( 0.3917322834645670104, 2.398668435337828261E-17, -0.1102362204724409017 ) ) ;
#64706=CARTESIAN_POINT ( 'NONE',  ( -0.1049643490035301885, -0.3917322834645671215, -2.204068241469816503 ) ) ;
#64710=CARTESIAN_POINT ( 'NONE',  ( 0.3458507752293908943, -0.3458507752293908943, -2.852362204724409711 ) ) ;
#64715=CARTESIAN_POINT ( 'NONE',  ( -0.1974969037888706924, 0.3420746716998658843, -2.767060367454068803 ) ) ;
#64724=CARTESIAN_POINT ( 'NONE',  ( 0.3917322834645669549, 0.1049643490035304660, -1.534120734908136052 ) ) ;
#64727=CARTESIAN_POINT ( 'NONE',  ( 0.3458507752293908943, 0.3458507752293908943, -0.05708661417322836301 ) ) ;
#64740=CARTESIAN_POINT ( 'NONE',  ( -9.787531504996566615E-17, 0.3996062992125985480, -1.179133858267716661 ) ) ;
#64741=CARTESIAN_POINT ( 'NONE',  ( -0.1958661417322834220, -0.3392501089628018884, -2.512467191601049699 ) ) ;
#64750=CARTESIAN_POINT ( 'NONE',  ( 0.4724409448818898682, 2.892866454678787531E-17, -0.7480314960629921295 ) ) ;
#64751=CARTESIAN_POINT ( 'NONE',  ( 0.1049643490035303967, 0.3917322834645670659, -2.509861835466878244 ) ) ;
#64752=EDGE_LOOP ( 'NONE', ( #81179, #27392, #72342, #55378 ) ) ;
#64757=CARTESIAN_POINT ( 'NONE',  ( -0.1958661417322836718, 0.3392501089628017219, -1.987532808398950079 ) ) ;
#64762=CARTESIAN_POINT ( 'NONE',  ( -0.3996062992125986035, 0.1070741851644051584, -2.629265091863516979 ) ) ;
#64764=CARTESIAN_POINT ( 'NONE',  ( 0.3996062992125986590, -0.1070741851644053111, -1.371391076115485053 ) ) ;
#64766=CARTESIAN_POINT ( 'NONE',  ( 0.3392501089628018884, -0.1958661417322833942, -0.1017253525272460019 ) ) ;
#64767=ORIENTED_EDGE ( 'NONE', *, *, #57587, .T. ) ;
#64780=CARTESIAN_POINT ( 'NONE',  ( -0.2867679344610364334, -0.2867679344610367109, -0.3661417322834645827 ) ) ;
#64782=VERTEX_POINT ( 'NONE', #62258 ) ;
#64783=CARTESIAN_POINT ( 'NONE',  ( 0.1974969037888704704, 0.3420746716998660508, -0.6167979002624671692 ) ) ;
#64786=DIRECTION ( 'NONE',  ( 0.000000000000000000, 0.000000000000000000, 1.000000000000000000 ) ) ;
#64790=CARTESIAN_POINT ( 'NONE',  ( -0.2867679344610365444, -0.2867679344610367664, -1.630596743603361265 ) ) ;
#64796=CARTESIAN_POINT ( 'NONE',  ( 0.1998031496062992740, 0.3460692066303959757, -1.246719160104986734 ) ) ;
#64798=CARTESIAN_POINT ( 'NONE',  ( 0.3996062992125984925, 0.1070741851644054637, -0.6738845144356955252 ) ) ;
#64799=CARTESIAN_POINT ( 'NONE',  ( 0.1070741851644054776, -0.3996062992125984925, -0.3195538057742782212 ) ) ;
#64801=CARTESIAN_POINT ( 'NONE',  ( 0.1070741851644053527, 0.3996062992125986590, -2.670603674540682260 ) ) ;
#64802=CARTESIAN_POINT ( 'NONE',  ( 0.3917322834645670104, 2.398668435337828261E-17, -2.092519685039370358 ) ) ;
#64808=CARTESIAN_POINT ( 'NONE',  ( -0.2362204724409447953, -0.4091458600556404646, -1.559711286089238591 ) ) ;
#64811=CARTESIAN_POINT ( 'NONE',  ( -0.3949938075777409963, -7.255918531996591613E-17, -1.375984251968503713 ) ) ;
#64822=CARTESIAN_POINT ( 'NONE',  ( -0.3996062992125986590, 0.1070741851644051723, -2.314304461942256808 ) ) ;
#64824=( BOUNDED_CURVE ( )  B_SPLINE_CURVE ( 2, ( #12029, #57856, #14111, #19994, #51957, #70929, #44802, #40184, #71340, #224, #51125, #27131, #13274 ),
 .UNSPECIFIED., .F., .F. ) 
 B_SPLINE_CURVE_WITH_KNOTS ( ( 3, 2, 2, 2, 2, 2, 3 ),
 ( 0.8625000000000000444, 0.8666666666666666963, 0.8708333333333333481, 0.8750000000000001110, 0.8791666666666667629, 0.8833333333333334147, 0.8875000000000000666 ),
 .UNSPECIFIED. ) 
 CURVE ( )  GEOMETRIC_REPRESENTATION_ITEM ( )  RATIONAL_B_SPLINE_CURVE ( ( 1.000000000000000000, 0.9659258262890683122, 1.000000000000000000, 0.9659258262890683122, 1.000000000000000000, 0.9659258262890683122, 1.000000000000000000, 0.9659258262890683122, 1.000000000000000000, 0.9659258262890683122, 1.000000000000000000, 0.9659258262890674240, 1.000000000000000888 ) ) 
 REPRESENTATION_ITEM ( '' )  );
#64826=CARTESIAN_POINT ( 'NONE',  ( -0.1049643490035306742, 0.3917322834645668994, -1.976358636974066663 ) ) ;
#64835=CARTESIAN_POINT ( 'NONE',  ( -0.4724409448818898682, -8.678599364036362592E-17, -2.401574803149606474 ) ) ;
#64840=CARTESIAN_POINT ( 'NONE',  ( 0.1958661417322836440, -0.3392501089628017219, -1.436351706036745446 ) ) ;
#64861=CARTESIAN_POINT ( 'NONE',  ( 0.3917322834645669549, 0.1049643490035304660, -2.479002624671915900 ) ) ;
#64864=CARTESIAN_POINT ( 'NONE',  ( -0.4091458600556405756, 0.2362204724409446288, -0.9711286089238845287 ) ) ;
#64865=CARTESIAN_POINT ( 'NONE',  ( 0.3460692066303959202, 0.1998031496062993295, -0.1312335958005249603 ) ) ;
#64868=CARTESIAN_POINT ( 'NONE',  ( 0.1049643490035304938, -0.3917322834645669549, -1.967191601049868899 ) ) ;
#64869=EDGE_LOOP ( 'NONE', ( #64767, #63293, #71489 ) ) ;
#64872=CARTESIAN_POINT ( 'NONE',  ( 0.2362204724409451007, -0.4091458600556402980, -2.926509186351706315 ) ) ;
#64879=CARTESIAN_POINT ( 'NONE',  ( 0.3392501089628018329, 0.1958661417322835052, -1.313628978181415441 ) ) ;
#64886=CARTESIAN_POINT ( 'NONE',  ( -0.1958661417322833942, -0.3392501089628018884, -2.424559998196537336 ) ) ;
#64896=CARTESIAN_POINT ( 'NONE',  ( 0.1049643490035303689, 0.3917322834645670104, -1.967847769028871374 ) ) ;
#64907=( BOUNDED_SURFACE ( )  B_SPLINE_SURFACE ( 1, 2, ( 
 ( #19650, #71007, #64688, #7027, #32696, #53298, #53711, #66791, #21330, #33954, #54127, #21738, #79010, #3219, #22575, #60040, #54544, #22981, #73092, #79841, #15868, #41920, #48648, #80259, #3632, #29300, #47402, #28053, #22158, #47817, #1972, #74343, #16275, #54962, #34375, #9126, #28466, #2396, #80669, #16689, #60865, #9944, #79418, #35616, #73519, #9533, #46982, #15442, #41516, #35204, #72676, #42328, #15025, #40681, #67201, #28881, #34796, #59618, #8704, #66366, #41103, #48236, #60456, #73932, #2807, #27636, #67613, #61279, #8288, #30119, #43148, #81076, #10371, #30537, #81489, #55371, #62943, #82307, #36438, #30940, #82710, #49478, #56201, #75584, #18333, #25030, #56607, #63345, #5680, #23805, #4454, #81902, #24213, #61703, #50703, #75991, #31348, #10778, #68845, #4863, #62111, #57014, #76401, #37267, #69670, #55781, #12013, #49884, #69261, #23393, #75171, #17923, #11608, #49060, #18733, #74759, #29708, #43560, #5277, #11191, #36029, #68438, #17107, #17516, #24626, #36852, #50293, #62525, #4043, #43973, #37667, #68027, #42742, #65010, #19136, #58260, #207, #1049, #70911, #38497, #51942, #51108, #83123, #26703, #13261, #52779, #38079, #19979, #6094, #44375, #78488, #52358, #64180, #76805, #39325, #39748, #78065, #77647, #26281, #63754, #625, #45211, #25860, #38911, #20395, #64591, #45630, #6927, #70067, #65444, #25442, #12422, #71324, #51519, #7776, #44785, #31769, #58684, #33014, #57430, #77223, #46048, #32598, #27116, #71741, #70482, #59104, #12839, #1459, #33444, #13673, #6514, #32184, #57839, #19552, #7346, #14096, #21225, #33852, #40581, #60356, #46880, #3115, #14921, #14516, #54025, #22052, #72574, #67098, #41414, #78904, #34693, #59935, #60765, #47297, #66261, #28363, #27534, #59517, #28781, #72986, #29198, #40169, #79736, #65853, #20812, #54865, #54444, #8601, #53191, #15761, #16171, #80155, #47713, #2703, #8186, #73413, #21637, #2290, #15338, #22473, #41002, #9429, #66684, #46467, #41816, #1872, #72161, #35098, #27951, #67507, #34273, #53610, #48133, #73831, #79318, #9020, #9843, #35514, #3532, #61178, #82106, #13053, #74243, #38706, #45001, #37880, #17720, #48544, #64385, #18127, #70700, #43347, #43759, #56811, #11398, #22881, #44179, #11817, #69049, #76606, #12631, #50089, #44584, #6721, #63143, #69871, #5889, #31979, #32391, #70278, #77019, #19352, #37470, #69465, #12223, #63555, #37055, #80570, #6303, #62739, #24419, #82510, #18535, #75785, #5075, #30744, #50905, #2, #5484, #25654, #31561, #82920, #56407, #31145, #57218, #25240, #24826, #50494, #76197, #18936, #38290, #63966, #57639, #51316, #1673, #13464, #47098, #39121, #19772, #65663, #7990, #1266, #26076, #58481, #71121, #77861, #14315, #846, #40382, #52156, #51736, #33654, #59317, #26503, #21027, #78703, #32814, #71961, #13887, #14730, #26914, #20190, #27330, #64802, #7141, #66065, #52574, #66478, #77438, #52990, #45425, #58054, #8813, #8401, #45841, #71540, #46687, #53415, #34068, #72380, #39974, #39546, #59732, #58906, #65235, #78283, #2086, #20614, #27751, #46266, #420, #79124, #7572, #33245, #21441, #72787, #15137, #40793, #60155, #48757, #23090, #28166, #41622, #74456, #60978, #17219, #36138, #34906, #49170, #53823, #74875, #81186, #74038, #79537, #2507, #42851, #54240, #23503, #21850, #79957, #9646, #47514, #73206, #80369, #47929, #15556, #29407, #16803, #2920, #80774, #68544, #15975, #22682, #42032, #68139, #34489, #42439, #29815, #55476, #73633, #22270, #48341, #16385, #41215, #66903, #10484, #9234, #60569, #35315, #54658, #28584, #67311, #3328, #3743, #61810, #28992, #4150, #67726, #35724, #10061, #61394, #55066, #50813, #44087, #76101, #30230, #50404, #11724, #49996, #63051, #76514, #31051, #18445, #5389, #36545, #6205, #49586, #62221, #69781, #75693, #31883, #75281, #4559, #25145 ),
 ( #55892, #81604, #25555, #30650, #57543, #23920, #56314, #69370, #17624, #43256, #56720, #24326, #68953, #5794, #18843, #62639, #57126, #51222, #18034, #82417, #12126, #44489, #76920, #82820, #83234, #19248, #43668, #82012, #24736, #37783, #11303, #44900, #70180, #10885, #36962, #37380, #63460, #4983, #31464, #12533, #38193, #63868, #64705, #14630, #1167, #71863, #25976, #7045, #26818, #14213, #51634, #59632, #77339, #32294, #78184, #20515, #13789, #38610, #71024, #322, #32714, #52476, #13368, #52893, #58381, #64288, #46167, #39871, #39021, #33555, #7894, #45329, #65560, #26400, #27234, #39446, #742, #59218, #19667, #52057, #78606, #65134, #79026, #6623, #1579, #57954, #70598, #21345, #20929, #77763, #20095, #46585, #65967, #33138, #72284, #40286, #45746, #71441, #7470, #8304, #58810, #33971, #1988, #27651, #53313, #12952, #46998, #34810, #9960, #21752, #22995, #29313, #8717, #60881, #61292, #53725, #74358, #15457, #79855, #79433, #67214, #9547, #22587, #35217, #47415, #54141, #3647, #41528, #66804, #34388, #41115, #60053, #48248, #2820, #9139, #54558, #2409, #3232, #28067, #41933, #60469, #28481, #73106, #80681, #73533, #54974, #22172, #16289, #35631, #48660, #72692, #73944, #15039, #47830, #15880, #28896, #40695, #67628, #80272, #66380, #26670, #72542, #45596, #46432, #72124, #14889, #26247, #34238, #78867, #40136, #33409, #8568, #52325, #51906, #39290, #71290, #40549, #14482, #21193, #8154, #1839, #59899, #77613, #46011, #46847, #65821, #58224, #19946, #59485, #66230, #59071, #72953, #64976, #1017, #33819, #13637, #78031, #27499, #7313, #38876, #53576, #53155, #2251, #27917, #65406, #32982, #21603, #20361, #32561, #47263, #27082, #79285, #71707, #64554, #58650, #14061, #6892, #591, #52744, #39715, #7744, #1426, #78452, #20778, #31336, #51507, #32171, #30524, #83111, #63332, #63743, #44363, #24200, #43547, #62929, #6082, #69247, #70055, #50690, #57001, #17911, #82698, #17503, #56594, #76793, #11594, #57827, #38484, #62511, #76388, #44773, #49871, #25847, #37254, #69656, #75571, #25017, #18721, #31756, #12409, #5263, #18318, #70470, #38067, #30927, #4849, #82294, #56187, #57418, #24613, #50280, #25430, #81889, #51095, #75978, #19124, #43960, #12000, #37654, #6501, #5669, #64168, #12827, #195, #43135, #68831, #11178, #36838, #72565, #45620, #77637, #33005, #8592, #33843, #45197, #14912, #65001, #27524, #615, #1450, #27107, #53180, #64578, #40572, #59509, #78478, #71732, #46871, #7337, #6916, #19969, #26271, #78895, #52770, #1863, #46458, #40160, #66253, #32587, #1040, #21216, #20802, #13250, #58250, #14507, #34264, #14087, #27942, #71314, #39314, #72152, #51932, #58675, #65844, #13662, #77211, #59924, #8177, #2279, #19540, #20386, #26694, #70900, #52349, #38899, #78056, #65435, #46037, #39739, #7768, #33434, #59095, #67917, #80144, #36328, #55258, #54017, #68333, #47288, #10672, #16993, #9833, #72977, #21627, #62003, #73401, #42636, #15329, #15752, #28772, #66674, #79309, #16159, #67088, #40994, #48532, #10254, #22045, #16577, #4339, #35089, #41806, #61168, #3938, #53600, #42222, #48951, #74652, #9420, #41405, #67498, #35504, #9012, #34684, #61592, #60348, #79728, #54434, #73822, #47705, #2695, #28355, #22871, #80967, #60756, #23281, #3519, #54855, #3107, #22465, #29188, #80560, #48125, #74233, #35925, #29597, #37562, #63236, #56498, #81378, #30421, #43039, #49774, #69560, #56089, #12315, #24105, #23691, #5576, #31242, #81794, #76297, #50589, #4748, #43857, #69146, #69961, #82200, #75474, #56908, #36734, #68735, #37973, #24518, #38387, #49365, #50184, #11077, #75061, #75881, #63648, #17815, #62409, #24922, #25335, #5987, #82604, #11908, #17409, #18627, #30833, #11496, #18222, #31658, #44270, #57316, #83013, #55669, #50998, #43448, #37150, #76696, #62835, #19030, #5169 ) ),
 .UNSPECIFIED., .F., .F., .F. ) 
 B_SPLINE_SURFACE_WITH_KNOTS ( ( 2, 2 ),
 ( 3, 2, 2, 2, 2, 2, 2, 2, 2, 2, 2, 2, 2, 2, 2, 2, 2, 2, 2, 2, 2, 2, 2, 2, 2, 2, 2, 2, 2, 2, 2, 2, 2, 2, 2, 2, 2, 2, 2, 2, 2, 2, 2, 2, 2, 2, 2, 2, 2, 2, 2, 2, 2, 2, 2, 2, 2, 2, 2, 2, 2, 2, 2, 2, 2, 2, 2, 2, 2, 2, 2, 2, 2, 2, 2, 2, 2, 2, 2, 2, 2, 2, 2, 2, 2, 2, 2, 2, 2, 2, 2, 2, 2, 2, 2, 2, 2, 2, 2, 2, 2, 2, 2, 2, 2, 2, 2, 2, 2, 2, 2, 2, 2, 2, 2, 2, 2, 2, 2, 2, 2, 2, 2, 2, 2, 2, 2, 2, 2, 2, 2, 2, 2, 2, 2, 2, 2, 2, 2, 2, 2, 2, 2, 2, 2, 2, 2, 2, 2, 2, 2, 2, 2, 2, 2, 2, 2, 2, 2, 2, 2, 2, 2, 2, 2, 2, 2, 2, 2, 2, 2, 2, 2, 2, 2, 2, 2, 2, 2, 2, 2, 2, 2, 2, 2, 2, 2, 2, 2, 2, 2, 2, 2, 2, 2, 2, 2, 2, 2, 2, 2, 2, 2, 2, 2, 2, 2, 2, 2, 2, 2, 2, 2, 2, 2, 2, 2, 2, 2, 2, 2, 2, 2, 2, 2, 2, 2, 2, 2, 2, 2, 2, 2, 2, 2, 2, 2, 3 ),
 ( 0.000000000000000000, 1.000000000000000000 ),
 ( 0.000000000000000000, 0.004166666666666666609, 0.008333333333333333218, 0.01250000000000000069, 0.01666666666666666644, 0.02083333333333333218, 0.02500000000000000139, 0.02916666666666666713, 0.03333333333333333287, 0.03749999999999999861, 0.04166666666666666435, 0.04583333333333333010, 0.05000000000000000278, 0.05416666666666666852, 0.05833333333333333426, 0.06250000000000000000, 0.06666666666666666574, 0.07083333333333333148, 0.07499999999999999722, 0.07916666666666666297, 0.08333333333333332871, 0.08749999999999999445, 0.09166666666666666019, 0.09583333333333333981, 0.1000000000000000056, 0.1041666666666666713, 0.1083333333333333370, 0.1125000000000000028, 0.1166666666666666685, 0.1208333333333333343, 0.1250000000000000000, 0.1291666666666666796, 0.1333333333333333315, 0.1375000000000000111, 0.1416666666666666630, 0.1458333333333333426, 0.1499999999999999944, 0.1541666666666666741, 0.1583333333333333259, 0.1625000000000000056, 0.1666666666666666574, 0.1708333333333333370, 0.1749999999999999889, 0.1791666666666666685, 0.1833333333333333204, 0.1875000000000000000, 0.1916666666666666796, 0.1958333333333333315, 0.2000000000000000111, 0.2041666666666666630, 0.2083333333333333426, 0.2124999999999999944, 0.2166666666666666741, 0.2208333333333333259, 0.2250000000000000056, 0.2291666666666666574, 0.2333333333333333370, 0.2374999999999999889, 0.2416666666666666685, 0.2458333333333333204, 0.2500000000000000000, 0.2541666666666666519, 0.2583333333333333592, 0.2625000000000000111, 0.2666666666666666630, 0.2708333333333333148, 0.2750000000000000222, 0.2791666666666666741, 0.2833333333333333259, 0.2874999999999999778, 0.2916666666666666852, 0.2958333333333333370, 0.2999999999999999889, 0.3041666666666666408, 0.3083333333333333481, 0.3125000000000000000, 0.3166666666666666519, 0.3208333333333333592, 0.3250000000000000111, 0.3291666666666666630, 0.3333333333333333148, 0.3375000000000000222, 0.3416666666666666741, 0.3458333333333333259, 0.3499999999999999778, 0.3541666666666666852, 0.3583333333333333370, 0.3624999999999999889, 0.3666666666666666408, 0.3708333333333333481, 0.3750000000000000000, 0.3791666666666666519, 0.3833333333333333592, 0.3875000000000000111, 0.3916666666666666630, 0.3958333333333333148, 0.4000000000000000222, 0.4041666666666666741, 0.4083333333333333259, 0.4124999999999999778, 0.4166666666666666852, 0.4208333333333333370, 0.4249999999999999889, 0.4291666666666666408, 0.4333333333333333481, 0.4375000000000000000, 0.4416666666666666519, 0.4458333333333333592, 0.4500000000000000111, 0.4541666666666666630, 0.4583333333333333148, 0.4625000000000000222, 0.4666666666666666741, 0.4708333333333333259, 0.4749999999999999778, 0.4791666666666666852, 0.4833333333333333370, 0.4874999999999999889, 0.4916666666666666408, 0.4958333333333333481, 0.5000000000000000000, 0.5041666666666666519, 0.5083333333333333037, 0.5124999999999999556, 0.5166666666666667185, 0.5208333333333333703, 0.5250000000000000222, 0.5291666666666666741, 0.5333333333333333259, 0.5374999999999999778, 0.5416666666666666297, 0.5458333333333332815, 0.5500000000000000444, 0.5541666666666666963, 0.5583333333333333481, 0.5625000000000000000, 0.5666666666666666519, 0.5708333333333333037, 0.5749999999999999556, 0.5791666666666667185, 0.5833333333333333703, 0.5875000000000000222, 0.5916666666666666741, 0.5958333333333333259, 0.5999999999999999778, 0.6041666666666666297, 0.6083333333333332815, 0.6125000000000000444, 0.6166666666666666963, 0.6208333333333333481, 0.6250000000000000000, 0.6291666666666666519, 0.6333333333333333037, 0.6374999999999999556, 0.6416666666666667185, 0.6458333333333333703, 0.6500000000000000222, 0.6541666666666666741, 0.6583333333333333259, 0.6624999999999999778, 0.6666666666666666297, 0.6708333333333332815, 0.6750000000000000444, 0.6791666666666666963, 0.6833333333333333481, 0.6875000000000000000, 0.6916666666666666519, 0.6958333333333333037, 0.6999999999999999556, 0.7041666666666667185, 0.7083333333333333703, 0.7125000000000000222, 0.7166666666666666741, 0.7208333333333333259, 0.7249999999999999778, 0.7291666666666666297, 0.7333333333333332815, 0.7375000000000000444, 0.7416666666666666963, 0.7458333333333333481, 0.7500000000000000000, 0.7541666666666666519, 0.7583333333333333037, 0.7624999999999999556, 0.7666666666666667185, 0.7708333333333333703, 0.7750000000000000222, 0.7791666666666666741, 0.7833333333333333259, 0.7874999999999999778, 0.7916666666666666297, 0.7958333333333332815, 0.8000000000000000444, 0.8041666666666666963, 0.8083333333333333481, 0.8125000000000000000, 0.8166666666666666519, 0.8208333333333333037, 0.8249999999999999556, 0.8291666666666667185, 0.8333333333333333703, 0.8375000000000000222, 0.8416666666666666741, 0.8458333333333333259, 0.8499999999999999778, 0.8541666666666666297, 0.8583333333333332815, 0.8625000000000000444, 0.8666666666666666963, 0.8708333333333333481, 0.8750000000000000000, 0.8791666666666666519, 0.8833333333333333037, 0.8874999999999999556, 0.8916666666666667185, 0.8958333333333333703, 0.9000000000000000222, 0.9041666666666666741, 0.9083333333333333259, 0.9124999999999999778, 0.9166666666666666297, 0.9208333333333332815, 0.9250000000000000444, 0.9291666666666666963, 0.9333333333333333481, 0.9375000000000000000, 0.9416666666666666519, 0.9458333333333333037, 0.9499999999999999556, 0.9541666666666667185, 0.9583333333333333703, 0.9625000000000000222, 0.9666666666666666741, 0.9708333333333333259, 0.9749999999999999778, 0.9791666666666666297, 0.9833333333333332815, 0.9875000000000000444 ),
 .UNSPECIFIED. ) 
 GEOMETRIC_REPRESENTATION_ITEM ( )  RATIONAL_B_SPLINE_SURFACE ( (
 ( 1.000000000000000000, 0.9659258262890683122, 1.000000000000000000, 0.9659258262890683122, 1.000000000000000000, 0.9659258262890683122, 1.000000000000000000, 0.9659258262890683122, 1.000000000000000000, 0.9659258262890683122, 1.000000000000000000, 0.9659258262890683122, 1.000000000000000000, 0.9659258262890683122, 1.000000000000000000, 0.9659258262890683122, 1.000000000000000000, 0.9659258262890683122, 1.000000000000000000, 0.9659258262890683122, 1.000000000000000000, 0.9659258262890683122, 1.000000000000000000, 0.9659258262890683122, 1.000000000000000000, 0.9659258262890683122, 1.000000000000000000, 0.9659258262890683122, 1.000000000000000000, 0.9659258262890683122, 1.000000000000000000, 0.9659258262890683122, 1.000000000000000000, 0.9659258262890683122, 1.000000000000000000, 0.9659258262890683122, 1.000000000000000000, 0.9659258262890683122, 1.000000000000000000, 0.9659258262890683122, 1.000000000000000000, 0.9659258262890683122, 1.000000000000000000, 0.9659258262890683122, 1.000000000000000000, 0.9659258262890683122, 1.000000000000000000, 0.9659258262890683122, 1.000000000000000000, 0.9659258262890683122, 1.000000000000000000, 0.9659258262890683122, 1.000000000000000000, 0.9659258262890683122, 1.000000000000000000, 0.9659258262890683122, 1.000000000000000000, 0.9659258262890683122, 1.000000000000000000, 0.9659258262890683122, 1.000000000000000000, 0.9659258262890683122, 1.000000000000000000, 0.9659258262890683122, 1.000000000000000000, 0.9659258262890683122, 1.000000000000000000, 0.9659258262890683122, 1.000000000000000000, 0.9659258262890683122, 1.000000000000000000, 0.9659258262890683122, 1.000000000000000000, 0.9659258262890683122, 1.000000000000000000, 0.9659258262890683122, 1.000000000000000000, 0.9659258262890683122, 1.000000000000000000, 0.9659258262890683122, 1.000000000000000000, 0.9659258262890683122, 1.000000000000000000, 0.9659258262890683122, 1.000000000000000000, 0.9659258262890683122, 1.000000000000000000, 0.9659258262890683122, 1.000000000000000000, 0.9659258262890683122, 1.000000000000000000, 0.9659258262890683122, 1.000000000000000000, 0.9659258262890683122, 1.000000000000000000, 0.9659258262890683122, 1.000000000000000000, 0.9659258262890683122, 1.000000000000000000, 0.9659258262890683122, 1.000000000000000000, 0.9659258262890683122, 1.000000000000000000, 0.9659258262890683122, 1.000000000000000000, 0.9659258262890683122, 1.000000000000000000, 0.9659258262890683122, 1.000000000000000000, 0.9659258262890683122, 1.000000000000000000, 0.9659258262890683122, 1.000000000000000000, 0.9659258262890683122, 1.000000000000000000, 0.9659258262890683122, 1.000000000000000000, 0.9659258262890683122, 1.000000000000000000, 0.9659258262890683122, 1.000000000000000000, 0.9659258262890683122, 1.000000000000000000, 0.9659258262890683122, 1.000000000000000000, 0.9659258262890683122, 1.000000000000000000, 0.9659258262890683122, 1.000000000000000000, 0.9659258262890683122, 1.000000000000000000, 0.9659258262890683122, 1.000000000000000000, 0.9659258262890683122, 1.000000000000000000, 0.9659258262890683122, 1.000000000000000000, 0.9659258262890683122, 1.000000000000000000, 0.9659258262890683122, 1.000000000000000000, 0.9659258262890683122, 1.000000000000000000, 0.9659258262890683122, 1.000000000000000000, 0.9659258262890683122, 1.000000000000000000, 0.9659258262890683122, 1.000000000000000000, 0.9659258262890683122, 1.000000000000000000, 0.9659258262890683122, 1.000000000000000000, 0.9659258262890683122, 1.000000000000000000, 0.9659258262890683122, 1.000000000000000000, 0.9659258262890683122, 1.000000000000000000, 0.9659258262890683122, 1.000000000000000000, 0.9659258262890683122, 1.000000000000000000, 0.9659258262890683122, 1.000000000000000000, 0.9659258262890683122, 1.000000000000000000, 0.9659258262890683122, 1.000000000000000000, 0.9659258262890683122, 1.000000000000000000, 0.9659258262890683122, 1.000000000000000000, 0.9659258262890683122, 1.000000000000000000, 0.9659258262890683122, 1.000000000000000000, 0.9659258262890683122, 1.000000000000000000, 0.9659258262890683122, 1.000000000000000000, 0.9659258262890683122, 1.000000000000000000, 0.9659258262890683122, 1.000000000000000000, 0.9659258262890683122, 1.000000000000000000, 0.9659258262890683122, 1.000000000000000000, 0.9659258262890683122, 1.000000000000000000, 0.9659258262890683122, 1.000000000000000000, 0.9659258262890683122, 1.000000000000000000, 0.9659258262890683122, 1.000000000000000000, 0.9659258262890683122, 1.000000000000000000, 0.9659258262890683122, 1.000000000000000000, 0.9659258262890683122, 1.000000000000000000, 0.9659258262890683122, 1.000000000000000000, 0.9659258262890683122, 1.000000000000000000, 0.9659258262890683122, 1.000000000000000000, 0.9659258262890683122, 1.000000000000000000, 0.9659258262890683122, 1.000000000000000000, 0.9659258262890683122, 1.000000000000000000, 0.9659258262890683122, 1.000000000000000000, 0.9659258262890683122, 1.000000000000000000, 0.9659258262890683122, 1.000000000000000000, 0.9659258262890683122, 1.000000000000000000, 0.9659258262890683122, 1.000000000000000000, 0.9659258262890683122, 1.000000000000000000, 0.9659258262890683122, 1.000000000000000000, 0.9659258262890683122, 1.000000000000000000, 0.9659258262890683122, 1.000000000000000000, 0.9659258262890683122, 1.000000000000000000, 0.9659258262890683122, 1.000000000000000000, 0.9659258262890683122, 1.000000000000000000, 0.9659258262890683122, 1.000000000000000000, 0.9659258262890683122, 1.000000000000000000, 0.9659258262890683122, 1.000000000000000000, 0.9659258262890683122, 1.000000000000000000, 0.9659258262890683122, 1.000000000000000000, 0.9659258262890683122, 1.000000000000000000, 0.9659258262890683122, 1.000000000000000000, 0.9659258262890683122, 1.000000000000000000, 0.9659258262890683122, 1.000000000000000000, 0.9659258262890683122, 1.000000000000000000, 0.9659258262890683122, 1.000000000000000000, 0.9659258262890683122, 1.000000000000000000, 0.9659258262890683122, 1.000000000000000000, 0.9659258262890683122, 1.000000000000000000, 0.9659258262890683122, 1.000000000000000000, 0.9659258262890683122, 1.000000000000000000, 0.9659258262890683122, 1.000000000000000000, 0.9659258262890683122, 1.000000000000000000, 0.9659258262890683122, 1.000000000000000000, 0.9659258262890683122, 1.000000000000000000, 0.9659258262890683122, 1.000000000000000000, 0.9659258262890683122, 1.000000000000000000, 0.9659258262890683122, 1.000000000000000000, 0.9659258262890683122, 1.000000000000000000, 0.9659258262890683122, 1.000000000000000000, 0.9659258262890683122, 1.000000000000000000, 0.9659258262890683122, 1.000000000000000000, 0.9659258262890683122, 1.000000000000000000, 0.9659258262890683122, 1.000000000000000000, 0.9659258262890683122, 1.000000000000000000, 0.9659258262890683122, 1.000000000000000000, 0.9659258262890683122, 1.000000000000000000, 0.9659258262890683122, 1.000000000000000000, 0.9659258262890683122, 1.000000000000000000, 0.9659258262890683122, 1.000000000000000000, 0.9659258262890683122, 1.000000000000000000, 0.9659258262890683122, 1.000000000000000000, 0.9659258262890683122, 1.000000000000000000, 0.9659258262890683122, 1.000000000000000000, 0.9659258262890683122, 1.000000000000000000, 0.9659258262890683122, 1.000000000000000000, 0.9659258262890683122, 1.000000000000000000, 0.9659258262890683122, 1.000000000000000000, 0.9659258262890683122, 1.000000000000000000, 0.9659258262890683122, 1.000000000000000000, 0.9659258262890683122, 1.000000000000000000, 0.9659258262890683122, 1.000000000000000000, 0.9659258262890683122, 1.000000000000000000, 0.9659258262890683122, 1.000000000000000000, 0.9659258262890683122, 1.000000000000000000, 0.9659258262890683122, 1.000000000000000000, 0.9659258262890683122, 1.000000000000000000, 0.9659258262890683122, 1.000000000000000000, 0.9659258262890683122, 1.000000000000000000, 0.9659258262890683122, 1.000000000000000000, 0.9659258262890683122, 1.000000000000000000, 0.9659258262890683122, 1.000000000000000000, 0.9659258262890683122, 1.000000000000000000, 0.9659258262890683122, 1.000000000000000000, 0.9659258262890683122, 1.000000000000000000, 0.9659258262890683122, 1.000000000000000000, 0.9659258262890683122, 1.000000000000000000, 0.9659258262890683122, 1.000000000000000000, 0.9659258262890683122, 1.000000000000000000, 0.9659258262890683122, 1.000000000000000000, 0.9659258262890683122, 1.000000000000000000, 0.9659258262890683122, 1.000000000000000000, 0.9659258262890683122, 1.000000000000000000, 0.9659258262890683122, 1.000000000000000000, 0.9659258262890683122, 1.000000000000000000, 0.9659258262890683122, 1.000000000000000000, 0.9659258262890683122, 1.000000000000000000, 0.9659258262890683122, 1.000000000000000000, 0.9659258262890683122, 1.000000000000000000, 0.9659258262890683122, 1.000000000000000000, 0.9659258262890683122, 1.000000000000000000, 0.9659258262890683122, 1.000000000000000000, 0.9659258262890683122, 1.000000000000000000, 0.9659258262890683122, 1.000000000000000000, 0.9659258262890683122, 1.000000000000000000, 0.9659258262890683122, 1.000000000000000000, 0.9659258262890683122, 1.000000000000000000, 0.9659258262890683122, 1.000000000000000000, 0.9659258262890683122, 1.000000000000000000, 0.9659258262890683122, 1.000000000000000000, 0.9659258262890683122, 1.000000000000000000, 0.9659258262890683122, 1.000000000000000000, 0.9659258262890683122, 1.000000000000000000, 0.9659258262890683122, 1.000000000000000000, 0.9659258262890683122, 1.000000000000000000, 0.9659258262890683122, 1.000000000000000000, 0.9659258262890683122, 1.000000000000000000, 0.9659258262890683122, 1.000000000000000000, 0.9659258262890683122, 1.000000000000000000, 0.9659258262890683122, 1.000000000000000000, 0.9659258262890683122, 1.000000000000000000, 0.9659258262890683122, 1.000000000000000000, 0.9659258262890683122, 1.000000000000000000, 0.9659258262890683122, 1.000000000000000000, 0.9659258262890683122, 1.000000000000000000, 0.9659258262890683122, 1.000000000000000000, 0.9659258262890683122, 1.000000000000000000, 0.9659258262890683122, 1.000000000000000000, 0.9659258262890683122, 1.000000000000000000, 0.9659258262890683122, 1.000000000000000000, 0.9659258262890683122, 1.000000000000000000, 0.9659258262890683122, 1.000000000000000000, 0.9659258262890683122, 1.000000000000000000, 0.9659258262890683122, 1.000000000000000000, 0.9659258262890683122, 1.000000000000000000, 0.9659258262890683122, 1.000000000000000000, 0.9659258262890683122, 1.000000000000000000, 0.9659258262890683122, 1.000000000000000000, 0.9659258262890683122, 1.000000000000000000, 0.9659258262890683122, 1.000000000000000000, 0.9659258262890683122, 1.000000000000000000, 0.9659258262890683122, 1.000000000000000000, 0.9659258262890683122, 1.000000000000000000),
 ( 1.000000000000000000, 0.9659258262890683122, 1.000000000000000000, 0.9659258262890683122, 1.000000000000000000, 0.9659258262890683122, 1.000000000000000000, 0.9659258262890683122, 1.000000000000000000, 0.9659258262890683122, 1.000000000000000000, 0.9659258262890683122, 1.000000000000000000, 0.9659258262890683122, 1.000000000000000000, 0.9659258262890683122, 1.000000000000000000, 0.9659258262890683122, 1.000000000000000000, 0.9659258262890683122, 1.000000000000000000, 0.9659258262890683122, 1.000000000000000000, 0.9659258262890683122, 1.000000000000000000, 0.9659258262890683122, 1.000000000000000000, 0.9659258262890683122, 1.000000000000000000, 0.9659258262890683122, 1.000000000000000000, 0.9659258262890683122, 1.000000000000000000, 0.9659258262890683122, 1.000000000000000000, 0.9659258262890683122, 1.000000000000000000, 0.9659258262890683122, 1.000000000000000000, 0.9659258262890683122, 1.000000000000000000, 0.9659258262890683122, 1.000000000000000000, 0.9659258262890683122, 1.000000000000000000, 0.9659258262890683122, 1.000000000000000000, 0.9659258262890683122, 1.000000000000000000, 0.9659258262890683122, 1.000000000000000000, 0.9659258262890683122, 1.000000000000000000, 0.9659258262890683122, 1.000000000000000000, 0.9659258262890683122, 1.000000000000000000, 0.9659258262890683122, 1.000000000000000000, 0.9659258262890683122, 1.000000000000000000, 0.9659258262890683122, 1.000000000000000000, 0.9659258262890683122, 1.000000000000000000, 0.9659258262890683122, 1.000000000000000000, 0.9659258262890683122, 1.000000000000000000, 0.9659258262890683122, 1.000000000000000000, 0.9659258262890683122, 1.000000000000000000, 0.9659258262890683122, 1.000000000000000000, 0.9659258262890683122, 1.000000000000000000, 0.9659258262890683122, 1.000000000000000000, 0.9659258262890683122, 1.000000000000000000, 0.9659258262890683122, 1.000000000000000000, 0.9659258262890683122, 1.000000000000000000, 0.9659258262890683122, 1.000000000000000000, 0.9659258262890683122, 1.000000000000000000, 0.9659258262890683122, 1.000000000000000000, 0.9659258262890683122, 1.000000000000000000, 0.9659258262890683122, 1.000000000000000000, 0.9659258262890683122, 1.000000000000000000, 0.9659258262890683122, 1.000000000000000000, 0.9659258262890683122, 1.000000000000000000, 0.9659258262890683122, 1.000000000000000000, 0.9659258262890683122, 1.000000000000000000, 0.9659258262890683122, 1.000000000000000000, 0.9659258262890683122, 1.000000000000000000, 0.9659258262890683122, 1.000000000000000000, 0.9659258262890683122, 1.000000000000000000, 0.9659258262890683122, 1.000000000000000000, 0.9659258262890683122, 1.000000000000000000, 0.9659258262890683122, 1.000000000000000000, 0.9659258262890683122, 1.000000000000000000, 0.9659258262890683122, 1.000000000000000000, 0.9659258262890683122, 1.000000000000000000, 0.9659258262890683122, 1.000000000000000000, 0.9659258262890683122, 1.000000000000000000, 0.9659258262890683122, 1.000000000000000000, 0.9659258262890683122, 1.000000000000000000, 0.9659258262890683122, 1.000000000000000000, 0.9659258262890683122, 1.000000000000000000, 0.9659258262890683122, 1.000000000000000000, 0.9659258262890683122, 1.000000000000000000, 0.9659258262890683122, 1.000000000000000000, 0.9659258262890683122, 1.000000000000000000, 0.9659258262890683122, 1.000000000000000000, 0.9659258262890683122, 1.000000000000000000, 0.9659258262890683122, 1.000000000000000000, 0.9659258262890683122, 1.000000000000000000, 0.9659258262890683122, 1.000000000000000000, 0.9659258262890683122, 1.000000000000000000, 0.9659258262890683122, 1.000000000000000000, 0.9659258262890683122, 1.000000000000000000, 0.9659258262890683122, 1.000000000000000000, 0.9659258262890683122, 1.000000000000000000, 0.9659258262890683122, 1.000000000000000000, 0.9659258262890683122, 1.000000000000000000, 0.9659258262890683122, 1.000000000000000000, 0.9659258262890683122, 1.000000000000000000, 0.9659258262890683122, 1.000000000000000000, 0.9659258262890683122, 1.000000000000000000, 0.9659258262890683122, 1.000000000000000000, 0.9659258262890683122, 1.000000000000000000, 0.9659258262890683122, 1.000000000000000000, 0.9659258262890683122, 1.000000000000000000, 0.9659258262890683122, 1.000000000000000000, 0.9659258262890683122, 1.000000000000000000, 0.9659258262890683122, 1.000000000000000000, 0.9659258262890683122, 1.000000000000000000, 0.9659258262890683122, 1.000000000000000000, 0.9659258262890683122, 1.000000000000000000, 0.9659258262890683122, 1.000000000000000000, 0.9659258262890683122, 1.000000000000000000, 0.9659258262890683122, 1.000000000000000000, 0.9659258262890683122, 1.000000000000000000, 0.9659258262890683122, 1.000000000000000000, 0.9659258262890683122, 1.000000000000000000, 0.9659258262890683122, 1.000000000000000000, 0.9659258262890683122, 1.000000000000000000, 0.9659258262890683122, 1.000000000000000000, 0.9659258262890683122, 1.000000000000000000, 0.9659258262890683122, 1.000000000000000000, 0.9659258262890683122, 1.000000000000000000, 0.9659258262890683122, 1.000000000000000000, 0.9659258262890683122, 1.000000000000000000, 0.9659258262890683122, 1.000000000000000000, 0.9659258262890683122, 1.000000000000000000, 0.9659258262890683122, 1.000000000000000000, 0.9659258262890683122, 1.000000000000000000, 0.9659258262890683122, 1.000000000000000000, 0.9659258262890683122, 1.000000000000000000, 0.9659258262890683122, 1.000000000000000000, 0.9659258262890683122, 1.000000000000000000, 0.9659258262890683122, 1.000000000000000000, 0.9659258262890683122, 1.000000000000000000, 0.9659258262890683122, 1.000000000000000000, 0.9659258262890683122, 1.000000000000000000, 0.9659258262890683122, 1.000000000000000000, 0.9659258262890683122, 1.000000000000000000, 0.9659258262890683122, 1.000000000000000000, 0.9659258262890683122, 1.000000000000000000, 0.9659258262890683122, 1.000000000000000000, 0.9659258262890683122, 1.000000000000000000, 0.9659258262890683122, 1.000000000000000000, 0.9659258262890683122, 1.000000000000000000, 0.9659258262890683122, 1.000000000000000000, 0.9659258262890683122, 1.000000000000000000, 0.9659258262890683122, 1.000000000000000000, 0.9659258262890683122, 1.000000000000000000, 0.9659258262890683122, 1.000000000000000000, 0.9659258262890683122, 1.000000000000000000, 0.9659258262890683122, 1.000000000000000000, 0.9659258262890683122, 1.000000000000000000, 0.9659258262890683122, 1.000000000000000000, 0.9659258262890683122, 1.000000000000000000, 0.9659258262890683122, 1.000000000000000000, 0.9659258262890683122, 1.000000000000000000, 0.9659258262890683122, 1.000000000000000000, 0.9659258262890683122, 1.000000000000000000, 0.9659258262890683122, 1.000000000000000000, 0.9659258262890683122, 1.000000000000000000, 0.9659258262890683122, 1.000000000000000000, 0.9659258262890683122, 1.000000000000000000, 0.9659258262890683122, 1.000000000000000000, 0.9659258262890683122, 1.000000000000000000, 0.9659258262890683122, 1.000000000000000000, 0.9659258262890683122, 1.000000000000000000, 0.9659258262890683122, 1.000000000000000000, 0.9659258262890683122, 1.000000000000000000, 0.9659258262890683122, 1.000000000000000000, 0.9659258262890683122, 1.000000000000000000, 0.9659258262890683122, 1.000000000000000000, 0.9659258262890683122, 1.000000000000000000, 0.9659258262890683122, 1.000000000000000000, 0.9659258262890683122, 1.000000000000000000, 0.9659258262890683122, 1.000000000000000000, 0.9659258262890683122, 1.000000000000000000, 0.9659258262890683122, 1.000000000000000000, 0.9659258262890683122, 1.000000000000000000, 0.9659258262890683122, 1.000000000000000000, 0.9659258262890683122, 1.000000000000000000, 0.9659258262890683122, 1.000000000000000000, 0.9659258262890683122, 1.000000000000000000, 0.9659258262890683122, 1.000000000000000000, 0.9659258262890683122, 1.000000000000000000, 0.9659258262890683122, 1.000000000000000000, 0.9659258262890683122, 1.000000000000000000, 0.9659258262890683122, 1.000000000000000000, 0.9659258262890683122, 1.000000000000000000, 0.9659258262890683122, 1.000000000000000000, 0.9659258262890683122, 1.000000000000000000, 0.9659258262890683122, 1.000000000000000000, 0.9659258262890683122, 1.000000000000000000, 0.9659258262890683122, 1.000000000000000000, 0.9659258262890683122, 1.000000000000000000, 0.9659258262890683122, 1.000000000000000000, 0.9659258262890683122, 1.000000000000000000, 0.9659258262890683122, 1.000000000000000000, 0.9659258262890683122, 1.000000000000000000, 0.9659258262890683122, 1.000000000000000000, 0.9659258262890683122, 1.000000000000000000, 0.9659258262890683122, 1.000000000000000000, 0.9659258262890683122, 1.000000000000000000, 0.9659258262890683122, 1.000000000000000000, 0.9659258262890683122, 1.000000000000000000, 0.9659258262890683122, 1.000000000000000000, 0.9659258262890683122, 1.000000000000000000, 0.9659258262890683122, 1.000000000000000000, 0.9659258262890683122, 1.000000000000000000, 0.9659258262890683122, 1.000000000000000000, 0.9659258262890683122, 1.000000000000000000, 0.9659258262890683122, 1.000000000000000000, 0.9659258262890683122, 1.000000000000000000, 0.9659258262890683122, 1.000000000000000000, 0.9659258262890683122, 1.000000000000000000, 0.9659258262890683122, 1.000000000000000000, 0.9659258262890683122, 1.000000000000000000, 0.9659258262890683122, 1.000000000000000000, 0.9659258262890683122, 1.000000000000000000, 0.9659258262890683122, 1.000000000000000000, 0.9659258262890683122, 1.000000000000000000, 0.9659258262890683122, 1.000000000000000000, 0.9659258262890683122, 1.000000000000000000, 0.9659258262890683122, 1.000000000000000000, 0.9659258262890683122, 1.000000000000000000, 0.9659258262890683122, 1.000000000000000000, 0.9659258262890683122, 1.000000000000000000, 0.9659258262890683122, 1.000000000000000000, 0.9659258262890683122, 1.000000000000000000, 0.9659258262890683122, 1.000000000000000000, 0.9659258262890683122, 1.000000000000000000, 0.9659258262890683122, 1.000000000000000000, 0.9659258262890683122, 1.000000000000000000, 0.9659258262890683122, 1.000000000000000000, 0.9659258262890683122, 1.000000000000000000, 0.9659258262890683122, 1.000000000000000000, 0.9659258262890683122, 1.000000000000000000, 0.9659258262890683122, 1.000000000000000000, 0.9659258262890683122, 1.000000000000000000, 0.9659258262890683122, 1.000000000000000000, 0.9659258262890683122, 1.000000000000000000, 0.9659258262890683122, 1.000000000000000000, 0.9659258262890683122, 1.000000000000000000, 0.9659258262890683122, 1.000000000000000000, 0.9659258262890683122, 1.000000000000000000, 0.9659258262890683122, 1.000000000000000000, 0.9659258262890683122, 1.000000000000000000, 0.9659258262890683122, 1.000000000000000000, 0.9659258262890683122, 1.000000000000000000, 0.9659258262890683122, 1.000000000000000000) ) ) 
 REPRESENTATION_ITEM ( '' )  SURFACE ( )  );
#64912=CARTESIAN_POINT ( 'NONE',  ( -0.4724409448818896462, -0.1265901696524993070, -0.3608923884514435576 ) ) ;
#64913=CARTESIAN_POINT ( 'NONE',  ( -0.1265901696524993347, 0.4724409448818895907, -0.2408136482939632061 ) ) ;
#64916=CARTESIAN_POINT ( 'NONE',  ( -0.3949938075777411073, 0.1058382717557497660, 0.04790026246719160385 ) ) ;
#64921=CARTESIAN_POINT ( 'NONE',  ( -0.3420746716998662729, 0.1974969037888702206, 0.05446194225721785048 ) ) ;
#64928=CARTESIAN_POINT ( 'NONE',  ( 0.3996062992125986035, -0.1070741851644052972, -0.9757217847769029673 ) ) ;
#64930=CARTESIAN_POINT ( 'NONE',  ( -0.3917322834645671215, 0.1049643490035301469, -0.6548556430446192955 ) ) ;
#64942=CARTESIAN_POINT ( 'NONE',  ( -0.3969271875946644434, -0.02899565511876312993, -1.220472440944881942 ) ) ;
#64944=CARTESIAN_POINT ( 'NONE',  ( -0.4724409448818895907, -0.1265901696524993070, -2.484908136482939955 ) ) ;
#64965=CARTESIAN_POINT ( 'NONE',  ( 0.2925321140481932369, -0.2925321140481931814, -0.5708661417322833387 ) ) ;
#64970=CARTESIAN_POINT ( 'NONE',  ( 0.3996062992125986590, -0.1070741851644053111, -2.788713910761154047 ) ) ;
#64971=CARTESIAN_POINT ( 'NONE',  ( -0.3420746716998659953, -0.1974969037888706647, -1.784776902887138972 ) ) ;
#64972=CARTESIAN_POINT ( 'NONE',  ( -0.3917322834645670104, -7.196005306013484475E-17, -0.6614173228346454936 ) ) ;
#64974=CARTESIAN_POINT ( 'NONE',  ( 4.797336870675656522E-17, -0.3917322834645670104, -1.173228346456692828 ) ) ;
#64976=CARTESIAN_POINT ( 'NONE',  ( -9.594673741351313045E-17, 0.3917322834645670104, -1.094488188976378007 ) ) ;
#64979=CARTESIAN_POINT ( 'NONE',  ( -0.3392501089628019439, 0.1958661417322832554, 0.05120041814404382302 ) ) ;
#64986=CARTESIAN_POINT ( 'NONE',  ( -0.3460692066303958092, -0.1998031496062994683, -2.572178477690288734 ) ) ;
#64987=CARTESIAN_POINT ( 'NONE',  ( -0.1958661417322833942, -0.3392501089628018884, -1.007237163550868120 ) ) ;
#64992=CARTESIAN_POINT ( 'NONE',  ( -0.3917322834645671215, 0.1049643490035301469, -0.7473753280839893209 ) ) ;
#65001=CARTESIAN_POINT ( 'NONE',  ( -0.3392501089628017219, -0.1958661417322836718, -1.776902887139107490 ) ) ;
#65003=CARTESIAN_POINT ( 'NONE',  ( -0.3996062992125986035, -7.340648628747425578E-17, -0.03937007874015750059 ) ) ;
#65010=CARTESIAN_POINT ( 'NONE',  ( 0.1049643490035304938, -0.3917322834645669549, -0.6423884514435697080 ) ) ;
#65022=DIRECTION ( 'NONE',  ( 0.000000000000000000, -0.000000000000000000, 1.000000000000000000 ) ) ;
#65031=CARTESIAN_POINT ( 'NONE',  ( 0.3392501089628018329, -0.1958661417322834497, -0.8149413141394206139 ) ) ;
#65034=CARTESIAN_POINT ( 'NONE',  ( 0.1049643490035303689, 0.3917322834645670104, -1.180446194225721834 ) ) ;
#65040=CARTESIAN_POINT ( 'NONE',  ( 0.1958661417322834775, 0.3392501089628018884, -0.1410954312674034816 ) ) ;
#65044=CARTESIAN_POINT ( 'NONE',  ( 0.4724409448818897572, -0.1265901696524988906, -1.290682414698162583 ) ) ;
#65060=CARTESIAN_POINT ( 'NONE',  ( 4.893765752498283308E-17, -0.3996062992125985480, -2.202755905511811108 ) ) ;
#65064=CARTESIAN_POINT ( 'NONE',  ( -0.1998031496062991630, -0.3460692066303959202, -1.717191601049869121 ) ) ;
#65068=CARTESIAN_POINT ( 'NONE',  ( 5.785732909357575061E-17, -0.4724409448818898682, -0.07874015748031495954 ) ) ;
#65070=CARTESIAN_POINT ( 'NONE',  ( 0.3996062992125985480, -0.1070741851644052972, -1.133202099737532720 ) ) ;
#65071=CARTESIAN_POINT ( 'NONE',  ( -0.1998031496062991907, -0.3460692066303959757, -1.325459317585301777 ) ) ;
#65072=VECTOR ( 'NONE', #9794, 39.37007874015748143 ) ;
#65073=CARTESIAN_POINT ( 'NONE',  ( -0.3949938075777409408, -0.1058382717557502933, -0.6758530183727035068 ) ) ;
#65079=CARTESIAN_POINT ( 'NONE',  ( -0.1058382717557503072, 0.3949938075777408852, -1.815616797900262869 ) ) ;
#65084=CARTESIAN_POINT ( 'NONE',  ( 0.4091458600556404646, -0.2362204724409448231, -2.152230971128608950 ) ) ;
#65087=ORIENTED_EDGE ( 'NONE', *, *, #71325, .F. ) ;
#65092=CARTESIAN_POINT ( 'NONE',  ( -0.1049643490035301746, -0.3917322834645670659, -2.356936064795589036 ) ) ;
#65099=CARTESIAN_POINT ( 'NONE',  ( -0.2867679344610364334, -0.2867679344610367109, 0.1712598425196849850 ) ) ;
#65101=CARTESIAN_POINT ( 'NONE',  ( 0.3917322834645669549, 0.1049643490035304660, -2.006561679790026531 ) ) ;
#65104=CARTESIAN_POINT ( 'NONE',  ( 4.837279021331060870E-17, -0.3949938075777409963, -1.811023622047243986 ) ) ;
#65109=CARTESIAN_POINT ( 'NONE',  ( -0.2925321140481932924, 0.2925321140481931814, -0.6496062992125984925 ) ) ;
#65118=CARTESIAN_POINT ( 'NONE',  ( 0.2867679344610365999, -0.2867679344610365444, -0.4980314960629922405 ) ) ;
#65127=CARTESIAN_POINT ( 'NONE',  ( 4.893765752498283308E-17, -0.3996062992125985480, -1.887795275590550936 ) ) ;
#65132=CARTESIAN_POINT ( 'NONE',  ( 0.4091458600556404646, -0.2362204724409448231, -0.8923884514435694859 ) ) ;
#65134=CARTESIAN_POINT ( 'NONE',  ( -0.2867679344610364334, -0.2867679344610367109, -0.3661417322834645827 ) ) ;
#65135=CARTESIAN_POINT ( 'NONE',  ( 0.2867679344610366554, -0.2867679344610365444, -2.072834645669292097 ) ) ;
#65139=CARTESIAN_POINT ( 'NONE',  ( -0.3460692066303957537, -0.1998031496062994405, -0.1292650918635170898 ) ) ;
#65141=CARTESIAN_POINT ( 'NONE',  ( 5.785732909357575061E-17, -0.4724409448818898682, -1.100393700787401619 ) ) ;
#65145=CARTESIAN_POINT ( 'NONE',  ( -0.1058382717557497660, -0.3949938075777411073, -2.511154855643044748 ) ) ;
#65152=CARTESIAN_POINT ( 'NONE',  ( 0.3392501089628018884, -0.1958661417322834220, -1.829396325459317518 ) ) ;
#65156=CARTESIAN_POINT ( 'NONE',  ( -0.3458507752293906723, -0.3458507752293910609, 0.02165354330708659653 ) ) ;
#65170=CARTESIAN_POINT ( 'NONE',  ( -0.3460692066303957537, -0.1998031496062994405, -1.231627296587926468 ) ) ;
#65171=CARTESIAN_POINT ( 'NONE',  ( -0.3917322834645670104, -7.196005306013484475E-17, -2.801181102362204633 ) ) ;
#65180=CARTESIAN_POINT ( 'NONE',  ( 0.3460692066303959202, 0.1998031496062993295, 0.02624671916010497957 ) ) ;
#65181=CARTESIAN_POINT ( 'NONE',  ( 0.3917322834645670659, -0.1049643490035303273, -2.313011441766091192 ) ) ;
#65184=CARTESIAN_POINT ( 'NONE',  ( 0.02707642104390755797, -0.3965571307776183940, -3.856971560569892101E-17 ) ) ;
#65188=CARTESIAN_POINT ( 'NONE',  ( -0.3917322834645669549, -0.1049643490035306603, -2.335301837270341352 ) ) ;
#65193=CARTESIAN_POINT ( 'NONE',  ( -0.1998031496062991907, -0.3460692066303959757, -1.955380577427821454 ) ) ;
#65195=CARTESIAN_POINT ( 'NONE',  ( 0.3996062992125986035, 0.1070741851644054776, -1.384514435695537671 ) ) ;
#65198=CARTESIAN_POINT ( 'NONE',  ( -0.1049643490035302301, -0.3917322834645671770, -0.06891695357711476178 ) ) ;
#65209=CARTESIAN_POINT ( 'NONE',  ( -0.1958661417322834220, -0.3392501089628018884, -0.2152230971128608339 ) ) ;
#65212=CARTESIAN_POINT ( 'NONE',  ( 0.3949938075777409963, 2.418639510665530435E-17, -0.5905511811023622659 ) ) ;
#65228=CARTESIAN_POINT ( 'NONE',  ( -0.3460692066303958092, -0.1998031496062994683, -1.469816272965879245 ) ) ;
#65230=CARTESIAN_POINT ( 'NONE',  ( -0.1998031496062991630, -0.3460692066303959202, -0.6148293963254594097 ) ) ;
#65232=CARTESIAN_POINT ( 'NONE',  ( 4.893765752498283308E-17, -0.3996062992125985480, 0.001968503937007844932 ) ) ;
#65234=CARTESIAN_POINT ( 'NONE',  ( -0.1998031496062994683, 0.3460692066303958092, -2.690288713910760965 ) ) ;
#65235=CARTESIAN_POINT ( 'NONE',  ( 0.2867679344610365999, -0.2867679344610365444, -2.230314960629921295 ) ) ;
#65241=CARTESIAN_POINT ( 'NONE',  ( -0.2362204724409451284, 0.4091458600556402425, -1.507217847769029007 ) ) ;
#65244=CARTESIAN_POINT ( 'NONE',  ( -0.3420746716998662729, 0.1974969037888702206, -1.520341207349081181 ) ) ;
#65255=CARTESIAN_POINT ( 'NONE',  ( 0.2925321140481932369, -0.2925321140481931814, -2.064960629921259727 ) ) ;
#65257=CARTESIAN_POINT ( 'NONE',  ( -0.3917322834645668994, -0.1049643490035306742, -2.173209030674854159 ) ) ;
#65270=CARTESIAN_POINT ( 'NONE',  ( -0.3460692066303957537, -0.1998031496062994405, 0.02821522309711285356 ) ) ;
#65272=CARTESIAN_POINT ( 'NONE',  ( -0.1958661417322836718, 0.3392501089628017219, -1.357611548556430625 ) ) ;
#65288=CARTESIAN_POINT ( 'NONE',  ( 0.3986795681651734702, 0.0008564280371857875508, -1.220472440944881720 ) ) ;
#65294=CARTESIAN_POINT ( 'NONE',  ( -0.1958661417322834220, -0.3392501089628018884, -2.419947506561679784 ) ) ;
#65298=CARTESIAN_POINT ( 'NONE',  ( -0.4091458600556405756, 0.2362204724409446288, -0.6561679790026246906 ) ) ;
#65299=CARTESIAN_POINT ( 'NONE',  ( -0.2925321140481930704, -0.2925321140481933480, -0.2165354330708662012 ) ) ;
#65302=CARTESIAN_POINT ( 'NONE',  ( 0.3917322834645670104, 2.398668435337828261E-17, -2.000000000000000000 ) ) ;
#65313=CARTESIAN_POINT ( 'NONE',  ( -0.1958661417322836440, 0.3392501089628016664, -1.195518741960943210 ) ) ;
#65320=CARTESIAN_POINT ( 'NONE',  ( 0.3917322834645670104, 0.1049643490035304660, -2.326134801346143366 ) ) ;
#65329=CARTESIAN_POINT ( 'NONE',  ( 0.3392501089628018884, -0.1958661417322834220, -1.921916010498687877 ) ) ;
#65345=CARTESIAN_POINT ( 'NONE',  ( 0.2362204724409449064, 0.4091458600556404646, -0.3786089238845143923 ) ) ;
#65348=CARTESIAN_POINT ( 'NONE',  ( -0.3949938075777409963, -7.255918531996591613E-17, -0.1161417322834646104 ) ) ;
#65353=CARTESIAN_POINT ( 'NONE',  ( 0.2891555358219910499, 0.2891555358219910499, 0.1003937007874015630 ) ) ;
#65360=CARTESIAN_POINT ( 'NONE',  ( -0.2925321140481930149, -0.2925321140481933480, -0.9232283464566929387 ) ) ;
#65363=CARTESIAN_POINT ( 'NONE',  ( -0.3392501089628019995, 0.1958661417322832277, -0.8057742782152230721 ) ) ;
#65379=CARTESIAN_POINT ( 'NONE',  ( 0.1265901696524990294, -0.4724409448818896462, -2.839238845144356649 ) ) ;
#65386=CARTESIAN_POINT ( 'NONE',  ( -0.4724409448818882584, 0.1265901696525017217, -2.080052493438319772 ) ) ;
#65396=CARTESIAN_POINT ( 'NONE',  ( 0.3996062992125985480, 0.1070741851644054637, -0.5971128608923884640 ) ) ;
#65401=CARTESIAN_POINT ( 'NONE',  ( 0.2925321140481932369, 0.2925321140481932369, -2.814960629921259727 ) ) ;
#65402=CARTESIAN_POINT ( 'NONE',  ( 0.1974969037888704704, 0.3420746716998660508, -1.719160104986876769 ) ) ;
#65403=CARTESIAN_POINT ( 'NONE',  ( 0.3917322834645670104, 2.398668435337828261E-17, -0.4251968503937007537 ) ) ;
#65404=CARTESIAN_POINT ( 'NONE',  ( 0.3917322834645670104, 2.398668435337828261E-17, -1.212598425196850238 ) ) ;
#65406=CARTESIAN_POINT ( 'NONE',  ( 4.797336870675656522E-17, -0.3917322834645670104, -1.173228346456692828 ) ) ;
#65408=CARTESIAN_POINT ( 'NONE',  ( -0.3392501089628018329, -0.1958661417322836440, 0.1824340139445687625 ) ) ;
#65416=CARTESIAN_POINT ( 'NONE',  ( -0.1998031496062994683, 0.3460692066303958092, -2.690288713910760965 ) ) ;
#65417=CARTESIAN_POINT ( 'NONE',  ( -0.1958661417322836995, 0.3392501089628017219, -1.269704355151917818 ) ) ;
#65426=CARTESIAN_POINT ( 'NONE',  ( -0.3392501089628019995, 0.1958661417322832277, -0.7408136482939633449 ) ) ;
#65434=CARTESIAN_POINT ( 'NONE',  ( 0.4724409448818898682, 2.892866454678787531E-17, -0.5098425196850393526 ) ) ;
#65435=CARTESIAN_POINT ( 'NONE',  ( -0.1958661417322834220, -0.3392501089628018884, -2.104986876640420057 ) ) ;
#65437=CARTESIAN_POINT ( 'NONE',  ( 0.3460692066303959757, -0.1998031496062991907, -0.5774278215223097588 ) ) ;
#65444=CARTESIAN_POINT ( 'NONE',  ( -0.1049643490035307020, 0.3917322834645669549, -0.8786089238845143923 ) ) ;
#65463=CARTESIAN_POINT ( 'NONE',  ( 0.1958661417322836162, -0.3392501089628018329, -0.9592982695199985255 ) ) ;
#65466=CARTESIAN_POINT ( 'NONE',  ( 0.1049643490035304799, -0.3917322834645669549, -1.114829396325459410 ) ) ;
#65472=CARTESIAN_POINT ( 'NONE',  ( -0.2867679344610365444, -0.2867679344610367664, -0.2132739089576921876 ) ) ;
#65477=CARTESIAN_POINT ( 'NONE',  ( 0.2362204724409451007, -0.4091458600556402980, -1.428477690288713964 ) ) ;
#65492=CARTESIAN_POINT ( 'NONE',  ( 0.2925321140481932369, -0.2925321140481931814, -2.537401574803149984 ) ) ;
#65496=CARTESIAN_POINT ( 'NONE',  ( -0.1070741851644056997, 0.3996062992125984925, -1.973097112860892510 ) ) ;
#65501=CARTESIAN_POINT ( 'NONE',  ( -0.3996062992125986035, -0.01591673448991143269, -1.219479340321616867 ) ) ;
#65502=CARTESIAN_POINT ( 'NONE',  ( 0.3460692066303959757, -0.1998031496062991907, -1.522309711286089273 ) ) ;
#65503=CARTESIAN_POINT ( 'NONE',  ( 4.837279021331060870E-17, -0.3949938075777409963, -0.5511811023622048555 ) ) ;
#65508=CARTESIAN_POINT ( 'NONE',  ( -0.3420746716998662729, 0.1974969037888702206, -1.677821522309711710 ) ) ;
#65513=CARTESIAN_POINT ( 'NONE',  ( 0.3458507752293908943, 0.3458507752293908943, -1.870078740157480546 ) ) ;
#65522=CARTESIAN_POINT ( 'NONE',  ( 0.3917322834645668994, -0.1049643490035303134, -2.553786458496376088 ) ) ;
#65523=CARTESIAN_POINT ( 'NONE',  ( -0.1070741851644051862, -0.3996062992125986590, -2.826115485564304475 ) ) ;
#65528=CARTESIAN_POINT ( 'NONE',  ( 0.2867679344610365999, 0.2867679344610365999, -2.737513492617110522 ) ) ;
#65530=CARTESIAN_POINT ( 'NONE',  ( 0.3917322834645669549, 0.1049643490035304660, -1.691601049868766360 ) ) ;
#65533=CARTESIAN_POINT ( 'NONE',  ( -0.1974969037888706647, 0.3420746716998658843, -2.060367454068241067 ) ) ;
#65540=CARTESIAN_POINT ( 'NONE',  ( 0.3996062992125986035, 2.446882876249141962E-17, -0.7480314960629921295 ) ) ;
#65548=CARTESIAN_POINT ( 'NONE',  ( -0.1049643490035302024, -0.3917322834645671215, -0.3143044619422573072 ) ) ;
#65558=CARTESIAN_POINT ( 'NONE',  ( 0.4091458600556404646, -0.2362204724409448231, -1.207349081364829324 ) ) ;
#65560=CARTESIAN_POINT ( 'NONE',  ( -9.594673741351313045E-17, 0.3917322834645670104, -0.3070866141732283006 ) ) ;
#65561=CARTESIAN_POINT ( 'NONE',  ( 0.3392501089628018329, 0.1958661417322835607, -2.263123359580052618 ) ) ;
#65565=CARTESIAN_POINT ( 'NONE',  ( 0.3996062992125984925, 0.1070741851644054637, 0.1135170603674540285 ) ) ;
#65570=CARTESIAN_POINT ( 'NONE',  ( -0.2891555358219909388, -0.2891555358219912164, -2.655511811023621771 ) ) ;
#65577=CARTESIAN_POINT ( 'NONE',  ( 0.3917322834645670104, 2.398668435337828261E-17, -2.000000000000000000 ) ) ;
#65580=CARTESIAN_POINT ( 'NONE',  ( -1.157146581871515012E-16, 0.4724409448818898682, -0.07677165354330710290 ) ) ;
#65594=CARTESIAN_POINT ( 'NONE',  ( 0.2925321140481932369, -0.2925321140481931814, -1.277559055118109965 ) ) ;
#65595=CARTESIAN_POINT ( 'NONE',  ( -0.1958661417322836718, 0.3392501089628017219, -2.774934383202099841 ) ) ;
#65598=VECTOR ( 'NONE', #29033, 39.37007874015748143 ) ;
#65606=CARTESIAN_POINT ( 'NONE',  ( -0.3996062992125986035, -0.1070741851644056997, -0.2034120734908136108 ) ) ;
#65607=CARTESIAN_POINT ( 'NONE',  ( 0.3392501089628018329, 0.1958661417322835607, -2.490176796096799539 ) ) ;
#65614=CARTESIAN_POINT ( 'NONE',  ( -0.1958661417322836718, 0.3392501089628017219, -2.459973753280839670 ) ) ;
#65619=CARTESIAN_POINT ( 'NONE',  ( -0.2925321140481930704, -0.2925321140481933480, -1.948818897637795144 ) ) ;
#65621=CARTESIAN_POINT ( 'NONE',  ( 0.1070741851644054915, -0.3996062992125986035, -1.817585301837270517 ) ) ;
#65623=CARTESIAN_POINT ( 'NONE',  ( 0.1049643490035303967, 0.3917322834645670659, 0.009823203903200209905 ) ) ;
#65624=EDGE_LOOP ( 'NONE', ( #61771, #20695, #17191, #71927, #40786 ) ) ;
#65636=CARTESIAN_POINT ( 'NONE',  ( 0.3392501089628018329, 0.1958661417322835607, -0.7532808398950130435 ) ) ;
#65639=CARTESIAN_POINT ( 'NONE',  ( -0.2891555358219911054, 0.2891555358219909388, -0.8070866141732284671 ) ) ;
#65648=EDGE_CURVE ( 'NONE', #17964, #400, #2458, .T. ) ;
#65651=CARTESIAN_POINT ( 'NONE',  ( 5.785732909357575061E-17, -0.4724409448818898682, -2.755905511811023612 ) ) ;
#65655=CARTESIAN_POINT ( 'NONE',  ( 0.3460692066303959757, -0.1998031496062991907, -1.364829396325459188 ) ) ;
#65657=CARTESIAN_POINT ( 'NONE',  ( -0.3996062992125986590, 0.1070741851644051723, -0.5820209973753280863 ) ) ;
#65658=CARTESIAN_POINT ( 'NONE',  ( 0.3460692066303959202, -0.1998031496062991630, -0.3392388451443569819 ) ) ;
#65660=CARTESIAN_POINT ( 'NONE',  ( 0.4091458600556404646, -0.2362204724409448231, 0.05249343832020997302 ) ) ;
#65661=( BOUNDED_CURVE ( )  B_SPLINE_CURVE ( 2, ( #28754, #4321, #41388, #73805, #10653, #48107, #35072 ),
 .UNSPECIFIED., .F., .F. ) 
 B_SPLINE_CURVE_WITH_KNOTS ( ( 3, 2, 2, 3 ),
 ( 0.05000000000000000278, 0.05416666666666666852, 0.05833333333333333426, 0.06250000000000000000 ),
 .UNSPECIFIED. ) 
 CURVE ( )  GEOMETRIC_REPRESENTATION_ITEM ( )  RATIONAL_B_SPLINE_CURVE ( ( 1.000000000000000000, 0.9659258262890683122, 1.000000000000000000, 0.9659258262890683122, 1.000000000000000000, 0.9659258262890683122, 1.000000000000000000 ) ) 
 REPRESENTATION_ITEM ( '' )  );
#65663=CARTESIAN_POINT ( 'NONE',  ( 0.3917322834645670104, 2.398668435337828261E-17, -1.935039370078740273 ) ) ;
#65670=CARTESIAN_POINT ( 'NONE',  ( -0.2362204724409447953, -0.4091458600556404646, -1.717191601049868677 ) ) ;
#65673=CARTESIAN_POINT ( 'NONE',  ( 4.837279021331061486E-17, -0.3949938075777409963, -1.415354330708661346 ) ) ;
#65679=CARTESIAN_POINT ( 'NONE',  ( -0.4724409448818898682, -8.678599364036362592E-17, -2.005905511811023612 ) ) ;
#65683=CARTESIAN_POINT ( 'NONE',  ( -0.2925321140481930149, -0.2925321140481933480, -2.498031496062992574 ) ) ;
#65684=CARTESIAN_POINT ( 'NONE',  ( -0.3917322834645670659, 0.1049643490035301607, -2.160085671094801540 ) ) ;
#65697=CARTESIAN_POINT ( 'NONE',  ( -0.1049643490035302024, -0.3917322834645671215, -1.574146981627296604 ) ) ;
#65709=ORIENTED_EDGE ( 'NONE', *, *, #75114, .T. ) ;
#65719=CARTESIAN_POINT ( 'NONE',  ( 0.3392501089628018884, -0.1958661417322834220, -2.301837270341207553 ) ) ;
#65721=CARTESIAN_POINT ( 'NONE',  ( -9.787531504996567848E-17, 0.3996062992125986035, -0.1574803149606299746 ) ) ;
#65724=CARTESIAN_POINT ( 'NONE',  ( 0.3917322834645670104, -0.1049643490035303411, -1.835958005249343827 ) ) ;
#65725=VERTEX_POINT ( 'NONE', #74404 ) ;
#65735=CARTESIAN_POINT ( 'NONE',  ( 0.3917322834645668994, 0.1049643490035304522, -1.307067298391389354 ) ) ;
#65741=CARTESIAN_POINT ( 'NONE',  ( 4.797336870675656522E-17, -0.3917322834645670659, -2.280203042815959869 ) ) ;
#65743=VERTEX_POINT ( 'NONE', #21797 ) ;
#65749=CARTESIAN_POINT ( 'NONE',  ( 0.2867679344610365999, 0.2867679344610365999, -1.954724409448818978 ) ) ;
#65762=CARTESIAN_POINT ( 'NONE',  ( -0.1265901696524986964, -0.4724409448818899238, -0.4639107611548556331 ) ) ;
#65766=CARTESIAN_POINT ( 'NONE',  ( 0.1058382717557500852, -0.3949938075777408852, -0.004593175853018378711 ) ) ;
#65771=CARTESIAN_POINT ( 'NONE',  ( -0.1058382717557503072, 0.3949938075777408852, -0.2408136482939632617 ) ) ;
#65778=CARTESIAN_POINT ( 'NONE',  ( -0.3996062992125984925, -0.1070741851644056858, -1.067585301837270517 ) ) ;
#65780=CARTESIAN_POINT ( 'NONE',  ( 0.1049643490035304938, -0.3917322834645669549, -0.5498687664041993495 ) ) ;
#65782=CARTESIAN_POINT ( 'NONE',  ( -0.3458507752293906723, -0.3458507752293910609, -0.4507874015748031815 ) ) ;
#65794=CARTESIAN_POINT ( 'NONE',  ( -0.2925321140481932369, 0.2925321140481931259, 0.2185039370078740162 ) ) ;
#65801=EDGE_CURVE ( 'NONE', #64662, #35562, #28940, .T. ) ;
#65811=CARTESIAN_POINT ( 'NONE',  ( -0.3996062992125986035, -7.340648628747425578E-17, -0.9842519685039369248 ) ) ;
#65816=CARTESIAN_POINT ( 'NONE',  ( -0.3460692066303960868, 0.1998031496062990242, -2.545931758530183497 ) ) ;
#65817=CARTESIAN_POINT ( 'NONE',  ( -0.2891555358219911054, 0.2891555358219909388, -1.751968503937008093 ) ) ;
#65818=CARTESIAN_POINT ( 'NONE',  ( 0.3392501089628018884, -0.1958661417322834220, -0.7270341207349080292 ) ) ;
#65819=CARTESIAN_POINT ( 'NONE',  ( 0.1958661417322836440, -0.3392501089628017219, -1.028871391076115360 ) ) ;
#65821=CARTESIAN_POINT ( 'NONE',  ( 0.3917322834645670104, -0.1049643490035303411, -1.048556430446194287 ) ) ;
#65823=CARTESIAN_POINT ( 'NONE',  ( 0.3917322834645668994, -0.1049643490035303134, -0.03410141912629739008 ) ) ;
#65829=CARTESIAN_POINT ( 'NONE',  ( 0.3996062992125986590, -0.1070741851644053111, -2.788713910761154047 ) ) ;
#65830=CARTESIAN_POINT ( 'NONE',  ( 0.1049643490035304799, -0.3917322834645670104, -1.184402517881576911 ) ) ;
#65835=CARTESIAN_POINT ( 'NONE',  ( 0.1049643490035304938, -0.3917322834645669549, -0.6423884514435697080 ) ) ;
#65843=CARTESIAN_POINT ( 'NONE',  ( 0.4091458600556403535, 0.2362204724409449896, -0.5229658792650918597 ) ) ;
#65844=CARTESIAN_POINT ( 'NONE',  ( 0.2867679344610365999, 0.2867679344610365999, -2.019685039370078261 ) ) ;
#65846=CARTESIAN_POINT ( 'NONE',  ( 0.1070741851644053527, 0.3996062992125986590, -0.3083989501312335846 ) ) ;
#65853=CARTESIAN_POINT ( 'NONE',  ( -0.3392501089628017219, -0.1958661417322836718, -1.239501312335958172 ) ) ;
#65867=ORIENTED_EDGE ( 'NONE', *, *, #82467, .T. ) ;
#65873=CARTESIAN_POINT ( 'NONE',  ( 0.2867679344610365999, -0.2867679344610365999, -1.280820579231284340 ) ) ;
#65882=CARTESIAN_POINT ( 'NONE',  ( 0.1049643490035304799, -0.3917322834645670104, -0.08204031315716725503 ) ) ;
#65886=CARTESIAN_POINT ( 'NONE',  ( 0.2362204724409449064, 0.4091458600556404646, -1.795931758530183719 ) ) ;
#65900=CARTESIAN_POINT ( 'NONE',  ( -9.674558042662122972E-17, 0.3949938075777409963, 0.2381889763779528046 ) ) ;
#65905=CARTESIAN_POINT ( 'NONE',  ( 4.893765752498283308E-17, -0.3996062992125985480, -1.730314960629921517 ) ) ;
#65910=CARTESIAN_POINT ( 'NONE',  ( -0.3996062992125985480, -7.340648628747423112E-17, -1.218503937007874072 ) ) ;
#65911=CARTESIAN_POINT ( 'NONE',  ( -0.3996062992125987146, 0.1070741851644051862, -1.450131233595800317 ) ) ;
#65912=CARTESIAN_POINT ( 'NONE',  ( -0.2891555358219911054, 0.2891555358219909388, -0.6496062992125984925 ) ) ;
#65918=CARTESIAN_POINT ( 'NONE',  ( 0.3949938075777409408, -0.1058382717557499186, -1.763123359580052396 ) ) ;
#65923=CARTESIAN_POINT ( 'NONE',  ( 0.2362204724409449064, 0.4091458600556404646, -2.191601049868766360 ) ) ;
#65924=CARTESIAN_POINT ( 'NONE',  ( 0.3922539627124315142, -0.006303098004669925071, -2.755905511811024944 ) ) ;
#65926=ORIENTED_EDGE ( 'NONE', *, *, #48857, .T. ) ;
#65930=CARTESIAN_POINT ( 'NONE',  ( 0.3917322834645668994, 0.1049643490035304522, -2.566909818076428706 ) ) ;
#65937=CARTESIAN_POINT ( 'NONE',  ( 0.3392501089628018329, -0.1958661417322834497, -2.704705093666980087 ) ) ;
#65939=CARTESIAN_POINT ( 'NONE',  ( -0.2867679344610364334, -0.2867679344610367109, -1.940944881889763884 ) ) ;
#65942=CARTESIAN_POINT ( 'NONE',  ( -0.1974969037888706647, 0.3420746716998658843, -2.375328083989501238 ) ) ;
#65947=CARTESIAN_POINT ( 'NONE',  ( -0.1070741851644056997, 0.3996062992125986035, -0.4790026246719158998 ) ) ;
#65954=CARTESIAN_POINT ( 'NONE',  ( -0.1049643490035307020, 0.3917322834645669549, -0.7211286089238846397 ) ) ;
#65959=CARTESIAN_POINT ( 'NONE',  ( -0.2867679344610365999, 0.2867679344610364889, 0.1456692913385827237 ) ) ;
#65965=CARTESIAN_POINT ( 'NONE',  ( -0.2362204724409451284, 0.4091458600556402425, -1.115485564304461885 ) ) ;
#65967=CARTESIAN_POINT ( 'NONE',  ( 0.3392501089628018329, 0.1958661417322835607, -0.4383202099737532609 ) ) ;
#65968=CARTESIAN_POINT ( 'NONE',  ( -0.3392501089628019995, 0.1958661417322832277, -2.473097112860892288 ) ) ;
#65971=CARTESIAN_POINT ( 'NONE',  ( 0.3460692066303959202, -0.1998031496062991630, -0.02427821522309713681 ) ) ;
#65976=CARTESIAN_POINT ( 'NONE',  ( -0.3949938075777411073, 0.1058382717557497660, -2.471784776902887337 ) ) ;
#65983=CARTESIAN_POINT ( 'NONE',  ( -0.1958661417322836718, 0.3392501089628017219, -2.052493438320210029 ) ) ;
#65987=CARTESIAN_POINT ( 'NONE',  ( -0.1265901696524993347, 0.4724409448818895907, -0.3982939632545932085 ) ) ;
#66000=CARTESIAN_POINT ( 'NONE',  ( 0.2925321140481932369, 0.2925321140481932369, -1.474409448818897683 ) ) ;
#66001=CARTESIAN_POINT ( 'NONE',  ( -0.2867679344610364334, -0.2867679344610367109, -2.820866141732283339 ) ) ;
#66006=( BOUNDED_CURVE ( )  B_SPLINE_CURVE ( 2, ( #25091, #76866, #82769, #19198, #70545, #38144, #6155, #56262, #30998, #44036, #55839, #81548, #23866 ),
 .UNSPECIFIED., .F., .F. ) 
 B_SPLINE_CURVE_WITH_KNOTS ( ( 3, 2, 2, 2, 2, 2, 3 ),
 ( 0.8125000000000000000, 0.8166666666666666519, 0.8208333333333333037, 0.8249999999999999556, 0.8291666666666667185, 0.8333333333333333703, 0.8375000000000000222 ),
 .UNSPECIFIED. ) 
 CURVE ( )  GEOMETRIC_REPRESENTATION_ITEM ( )  RATIONAL_B_SPLINE_CURVE ( ( 1.000000000000000000, 0.9659258262890683122, 1.000000000000000000, 0.9659258262890683122, 1.000000000000000000, 0.9659258262890683122, 1.000000000000000000, 0.9659258262890683122, 1.000000000000000000, 0.9659258262890683122, 1.000000000000000000, 0.9659258262890683122, 1.000000000000000000 ) ) 
 REPRESENTATION_ITEM ( '' )  );
#66010=CARTESIAN_POINT ( 'NONE',  ( 0.3460692066303959757, -0.1998031496062991907, -0.1049868766404199599 ) ) ;
#66011=CARTESIAN_POINT ( 'NONE',  ( 0.3917322834645670104, 0.1049643490035304660, -2.326134801346143366 ) ) ;
#66018=CARTESIAN_POINT ( 'NONE',  ( 0.1049643490035303689, 0.3917322834645670104, -2.282808398950130879 ) ) ;
#66026=CARTESIAN_POINT ( 'NONE',  ( 0.1958661417322836718, -0.3392501089628017219, -0.5610429378290832103 ) ) ;
#66038=EDGE_CURVE ( 'NONE', #2797, #23246, #66006, .T. ) ;
#66039=CARTESIAN_POINT ( 'NONE',  ( 0.3392501089628018329, 0.1958661417322835607, -0.4383202099737532609 ) ) ;
#66042=CARTESIAN_POINT ( 'NONE',  ( 0.3949938075777411073, -0.1058382717557499464, -0.8989501312335956840 ) ) ;
#66054=CARTESIAN_POINT ( 'NONE',  ( -0.4724409448818898682, -8.678599364036362592E-17, -2.716535433070865757 ) ) ;
#66059=CARTESIAN_POINT ( 'NONE',  ( -0.3996062992125986035, -7.340648628747425578E-17, -1.141732283464566899 ) ) ;
#66061=CARTESIAN_POINT ( 'NONE',  ( 0.2925321140481932369, 0.2925321140481932369, -0.8444881889763780070 ) ) ;
#66062=CARTESIAN_POINT ( 'NONE',  ( -0.3996062992125985480, -7.340648628747423112E-17, -0.7460629921259841479 ) ) ;
#66064=CARTESIAN_POINT ( 'NONE',  ( 0.4724409448818898682, 2.892866454678787531E-17, -0.1181102362204724532 ) ) ;
#66065=CARTESIAN_POINT ( 'NONE',  ( 0.3392501089628018329, 0.1958661417322835607, -2.105643044619422533 ) ) ;
#66071=CARTESIAN_POINT ( 'NONE',  ( -0.1265901696524993347, 0.4724409448818895907, -1.973097112860892510 ) ) ;
#66074=CARTESIAN_POINT ( 'NONE',  ( 0.3949938075777409408, -0.1058382717557499186, -1.605643044619423199 ) ) ;
#66084=CARTESIAN_POINT ( 'NONE',  ( -0.1998031496062991630, -0.3460692066303959202, -2.504593175853018661 ) ) ;
#66085=CARTESIAN_POINT ( 'NONE',  ( -0.2867679344610364334, -0.2867679344610368219, -2.186332390254906777 ) ) ;
#66094=CARTESIAN_POINT ( 'NONE',  ( -0.4724409448818896462, -0.1265901696524993070, -0.8333333333333332593 ) ) ;
#66098=CARTESIAN_POINT ( 'NONE',  ( -0.2925321140481932369, 0.2925321140481931259, -0.2539370078740156855 ) ) ;
#66100=CARTESIAN_POINT ( 'NONE',  ( 0.3392501089628018884, -0.1958661417322834220, -1.449475065616798064 ) ) ;
#66109=CARTESIAN_POINT ( 'NONE',  ( 0.3460692066303958092, 0.1998031496062993018, -0.9954068241469815614 ) ) ;
#66125=CARTESIAN_POINT ( 'NONE',  ( -0.3460692066303958092, -0.1998031496062994683, -0.6824146981627295938 ) ) ;
#66128=CARTESIAN_POINT ( 'NONE',  ( -0.1049643490035307020, 0.3917322834645669549, -2.045931758530183497 ) ) ;
#66139=CARTESIAN_POINT ( 'NONE',  ( 0.1958661417322834497, 0.3392501089628018329, -1.169272022800837973 ) ) ;
#66146=CARTESIAN_POINT ( 'NONE',  ( 0.3392501089628018329, 0.1958661417322835607, -2.490176796096799539 ) ) ;
#66155=CARTESIAN_POINT ( 'NONE',  ( -0.1958661417322834220, -0.3392501089628018884, -1.882545931758530244 ) ) ;
#66162=CARTESIAN_POINT ( 'NONE',  ( 0.4724409448818898682, 0.000000000000000000, -2.755905511811024056 ) ) ;
#66164=CARTESIAN_POINT ( 'NONE',  ( 0.3996062992125986590, -0.1070741851644053111, -1.686351706036745446 ) ) ;
#66169=CARTESIAN_POINT ( 'NONE',  ( 0.3458507752293908943, 0.3458507752293908943, -0.5295275590551181688 ) ) ;
#66173=CARTESIAN_POINT ( 'NONE',  ( 0.3949938075777409963, 2.418639510665530743E-17, -0.03740157480314962313 ) ) ;
#66180=CARTESIAN_POINT ( 'NONE',  ( 0.2891555358219910499, -0.2891555358219909944, -0.3326771653543307283 ) ) ;
#66185=CARTESIAN_POINT ( 'NONE',  ( 0.2362204724409451007, -0.4091458600556402980, -0.1686351706036745557 ) ) ;
#66188=CARTESIAN_POINT ( 'NONE',  ( 0.3996062992125985480, 2.446882876249141654E-17, -1.454724409448818978 ) ) ;
#66190=CARTESIAN_POINT ( 'NONE',  ( -0.1049643490035302024, -0.3917322834645671215, -0.5367454068241469534 ) ) ;
#66203=CARTESIAN_POINT ( 'NONE',  ( 0.3458507752293908943, -0.3458507752293908943, -2.694881889763780070 ) ) ;
#66220=CARTESIAN_POINT ( 'NONE',  ( 0.1998031496062992740, 0.3460692066303959757, -0.7742782152230971437 ) ) ;
#66224=CARTESIAN_POINT ( 'NONE',  ( 0.3460692066303959202, 0.1998031496062993295, -2.493438320209973469 ) ) ;
#66225=CARTESIAN_POINT ( 'NONE',  ( 0.1058382717557500713, -0.3949938075777409408, -2.290026246719159886 ) ) ;
#66227=CARTESIAN_POINT ( 'NONE',  ( -0.3392501089628017219, -0.1958661417322836718, -0.3595800524934382736 ) ) ;
#66230=CARTESIAN_POINT ( 'NONE',  ( 0.2867679344610365999, 0.2867679344610365999, -1.074803149606299080 ) ) ;
#66232=CARTESIAN_POINT ( 'NONE',  ( -0.3917322834645668994, -0.1049643490035306742, 0.1889956937345949883 ) ) ;
#66238=CARTESIAN_POINT ( 'NONE',  ( 0.1070741851644054915, -0.3996062992125986035, -2.604986876640420057 ) ) ;
#66239=CARTESIAN_POINT ( 'NONE',  ( 0.1958661417322836718, -0.3392501089628017219, -1.190964197671602998 ) ) ;
#66244=CARTESIAN_POINT ( 'NONE',  ( 0.3917322834645669549, 0.1049643490035304660, -0.5242782152230972548 ) ) ;
#66252=CARTESIAN_POINT ( 'NONE',  ( 0.3078094465266739133, -0.2432155562296511031, -1.929133858267716661 ) ) ;
#66253=CARTESIAN_POINT ( 'NONE',  ( -0.3917322834645671215, 0.1049643490035301469, -1.914698162729658648 ) ) ;
#66255=CARTESIAN_POINT ( 'NONE',  ( -0.1070741851644056997, 0.3996062992125986035, -0.6364829396325458744 ) ) ;
#66261=CARTESIAN_POINT ( 'NONE',  ( 0.1049643490035303689, 0.3917322834645670104, -1.180446194225722056 ) ) ;
#66273=CARTESIAN_POINT ( 'NONE',  ( -0.1070741851644051862, -0.3996062992125986035, -2.038713910761154491 ) ) ;
#66277=ORIENTED_EDGE ( 'NONE', *, *, #78409, .T. ) ;
#66283=CARTESIAN_POINT ( 'NONE',  ( -9.594673741351310580E-17, 0.3917322834645669549, -1.339875697341520455 ) ) ;
#66287=CARTESIAN_POINT ( 'NONE',  ( -0.3917322834645670104, -7.196005306013484475E-17, -1.068897637795275690 ) ) ;
#66293=CARTESIAN_POINT ( 'NONE',  ( 0.3917322834645670659, -0.1049643490035303273, -0.2657673472779021884 ) ) ;
#66296=CARTESIAN_POINT ( 'NONE',  ( 0.3458507752293908943, 0.3458507752293908943, -1.474409448818897683 ) ) ;
#66312=CARTESIAN_POINT ( 'NONE',  ( 0.3996062992125985480, 2.446882876249141654E-17, -2.714566929133858331 ) ) ;
#66317=CARTESIAN_POINT ( 'NONE',  ( 0.2925321140481932369, 0.2925321140481932369, -1.789370078740157410 ) ) ;
#66322=CARTESIAN_POINT ( 'NONE',  ( 0.1998031496062992463, 0.3460692066303959202, -1.008530183727034180 ) ) ;
#66323=CARTESIAN_POINT ( 'NONE',  ( 0.1070741851644053527, 0.3996062992125986590, -1.568241469816272993 ) ) ;
#66324=CARTESIAN_POINT ( 'NONE',  ( 0.3420746716998660508, -0.1974969037888703871, -0.7349081364829396223 ) ) ;
#66327=CARTESIAN_POINT ( 'NONE',  ( 0.3917322834645670104, -0.1049643490035303273, -0.1036745406824146343 ) ) ;
#66331=CARTESIAN_POINT ( 'NONE',  ( 0.3420746716998660508, 0.1974969037888705814, -1.782808398950131101 ) ) ;
#66335=CARTESIAN_POINT ( 'NONE',  ( 0.1265901696524989462, 0.4724409448818897572, -1.883202099737532276 ) ) ;
#66336=CARTESIAN_POINT ( 'NONE',  ( 0.2263583204867608833, 0.3204081651523129071, -2.755905511811024056 ) ) ;
#66344=CARTESIAN_POINT ( 'NONE',  ( -0.3917322834645670659, 0.1049643490035301607, -2.475046301016061268 ) ) ;
#66350=CARTESIAN_POINT ( 'NONE',  ( 0.3917322834645668994, -0.1049643490035303134, -2.711266773457006174 ) ) ;
#66353=CARTESIAN_POINT ( 'NONE',  ( -0.3392501089628019995, 0.1958661417322832277, -1.908136482939632561 ) ) ;
#66356=CARTESIAN_POINT ( 'NONE',  ( 4.837279021331060870E-17, -0.3949938075777409963, -2.283464566929133799 ) ) ;
#66361=CARTESIAN_POINT ( 'NONE',  ( -0.3996062992125987146, 0.1070741851644051862, -0.6627296587926508886 ) ) ;
#66366=CARTESIAN_POINT ( 'NONE',  ( -0.1049643490035302024, -0.3917322834645671215, -0.1568241469816273603 ) ) ;
#66378=CARTESIAN_POINT ( 'NONE',  ( -0.4091458600556405756, 0.2362204724409446288, -1.286089238845144367 ) ) ;
#66380=CARTESIAN_POINT ( 'NONE',  ( 0.2867679344610365999, -0.2867679344610365444, -0.8779527559055116948 ) ) ;
#66381=CARTESIAN_POINT ( 'NONE',  ( 0.2867679344610366554, 0.2867679344610366554, -2.427165354330708791 ) ) ;
#66384=CARTESIAN_POINT ( 'NONE',  ( -9.787531504996566615E-17, 0.3996062992125985480, 0.08070866141732281618 ) ) ;
#66388=CARTESIAN_POINT ( 'NONE',  ( 0.3392501089628018329, 0.1958661417322835052, 0.1036938564642537891 ) ) ;
#66391=CIRCLE ( 'NONE', #9972, 0.2952755905511810774 ) ;
#66396=CARTESIAN_POINT ( 'NONE',  ( -0.3917322834645669549, -0.1049643490035306603, -1.770341207349081181 ) ) ;
#66400=CARTESIAN_POINT ( 'NONE',  ( 0.1265901696524990294, -0.4724409448818896462, -0.4770341207349080848 ) ) ;
#66413=ORIENTED_EDGE ( 'NONE', *, *, #74544, .F. ) ;
#66414=CARTESIAN_POINT ( 'NONE',  ( -0.3996062992125986590, 0.1070741851644051723, -1.526902887139107490 ) ) ;
#66423=CARTESIAN_POINT ( 'NONE',  ( 0.3996062992125986035, 2.446882876249141962E-17, -0.2755905511811023723 ) ) ;
#66424=CARTESIAN_POINT ( 'NONE',  ( -0.3392501089628017219, -0.1958661417322836995, -2.726397268537744445 ) ) ;
#66430=CARTESIAN_POINT ( 'NONE',  ( 0.1049643490035304938, -0.3917322834645669549, -2.217191601049868677 ) ) ;
#66435=CARTESIAN_POINT ( 'NONE',  ( 0.3996062992125985480, 0.1070741851644054637, -2.014435695538057125 ) ) ;
#66437=ORIENTED_EDGE ( 'NONE', *, *, #17226, .F. ) ;
#66438=CARTESIAN_POINT ( 'NONE',  ( -0.3917322834645671770, 0.1049643490035302024, -0.5019878197188469837 ) ) ;
#66452=CARTESIAN_POINT ( 'NONE',  ( -0.3917322834645670104, -7.196005306013484475E-17, -0.8188976377952754682 ) ) ;
#66455=CARTESIAN_POINT ( 'NONE',  ( -0.3949938075777411628, 0.1058382717557497937, -0.9776902887139109488 ) ) ;
#66472=CARTESIAN_POINT ( 'NONE',  ( -0.1070741851644056997, 0.3996062992125986035, -1.896325459317584894 ) ) ;
#66474=CARTESIAN_POINT ( 'NONE',  ( 0.1998031496062992463, 0.3460692066303959202, -1.166010498687663821 ) ) ;
#66475=CARTESIAN_POINT ( 'NONE',  ( 0.1070741851644053388, 0.3996062992125986035, -0.3851706036745406458 ) ) ;
#66477=CARTESIAN_POINT ( 'NONE',  ( -0.4724409448818899238, 0.1265901696524986686, -0.03280839895013123314 ) ) ;
#66478=CARTESIAN_POINT ( 'NONE',  ( 0.1958661417322834775, 0.3392501089628018884, -2.118766404199475151 ) ) ;
#66484=CARTESIAN_POINT ( 'NONE',  ( 0.4091458600556404646, -0.2362204724409448231, -1.914041994750656395 ) ) ;
#66487=CARTESIAN_POINT ( 'NONE',  ( -0.1058382717557503072, 0.3949938075777408852, -1.973097112860892510 ) ) ;
#66498=CARTESIAN_POINT ( 'NONE',  ( -0.1998031496062991630, -0.3460692066303959202, -2.662073490813648746 ) ) ;
#66499=CARTESIAN_POINT ( 'NONE',  ( 4.797336870675655290E-17, -0.3917322834645669549, -2.206017429624985038 ) ) ;
#66514=CARTESIAN_POINT ( 'NONE',  ( 0.2925321140481932369, -0.2925321140481931814, -0.3326771653543306728 ) ) ;
#66516=CARTESIAN_POINT ( 'NONE',  ( -0.1958661417322836718, 0.3392501089628017219, -1.672572178477690352 ) ) ;
#66526=CARTESIAN_POINT ( 'NONE',  ( 0.1998031496062992463, 0.3460692066303959202, -1.166010498687663821 ) ) ;
#66541=CARTESIAN_POINT ( 'NONE',  ( -0.2925321140481930704, -0.2925321140481933480, -0.5314960629921260393 ) ) ;
#66544=CARTESIAN_POINT ( 'NONE',  ( -0.3917322834645670104, -7.196005306013484475E-17, -2.393700787401574992 ) ) ;
#66555=CARTESIAN_POINT ( 'NONE',  ( 0.3917322834645668994, 0.1049643490035304522, -1.464547613352018773 ) ) ;
#66561=CARTESIAN_POINT ( 'NONE',  ( -0.3392501089628017219, -0.1958661417322836995, -2.883877583498374531 ) ) ;
#66570=CARTESIAN_POINT ( 'NONE',  ( 0.1958661417322836440, -0.3392501089628017219, -2.223753280839895208 ) ) ;
#66577=CARTESIAN_POINT ( 'NONE',  ( -0.1998031496062994405, 0.3460692066303957537, 0.06758530183727033680 ) ) ;
#66579=CARTESIAN_POINT ( 'NONE',  ( -0.2925321140481932924, 0.2925321140481931814, -1.751968503937007648 ) ) ;
#66585=CARTESIAN_POINT ( 'NONE',  ( 0.4724409448818896462, 0.1265901696524990294, -0.8313648293963252778 ) ) ;
#66589=CARTESIAN_POINT ( 'NONE',  ( -0.2891555358219909388, -0.2891555358219912164, -0.2933070866141732624 ) ) ;
#66594=CARTESIAN_POINT ( 'NONE',  ( -0.3420746716998660508, -0.1974969037888706924, -0.4442257217847768724 ) ) ;
#66602=CARTESIAN_POINT ( 'NONE',  ( -0.3460692066303960313, 0.1998031496062989965, -1.520341207349081403 ) ) ;
#66604=CARTESIAN_POINT ( 'NONE',  ( -0.3917322834645669549, -0.1049643490035306603, -0.9829396325459317518 ) ) ;
#66616=CARTESIAN_POINT ( 'NONE',  ( -0.1070741851644056997, 0.3996062992125984925, 0.2316272965879264956 ) ) ;
#66630=( BOUNDED_CURVE ( )  B_SPLINE_CURVE ( 2, ( #23822, #81915, #49491, #42343, #75183, #17529, #28897, #44697, #16290, #68856, #11205, #4877, #25356 ),
 .UNSPECIFIED., .F., .F. ) 
 B_SPLINE_CURVE_WITH_KNOTS ( ( 3, 2, 2, 2, 2, 2, 3 ),
 ( 0.3375000000000000222, 0.3416666666666666741, 0.3458333333333333259, 0.3499999999999999778, 0.3541666666666666852, 0.3583333333333333370, 0.3624999999999999889 ),
 .UNSPECIFIED. ) 
 CURVE ( )  GEOMETRIC_REPRESENTATION_ITEM ( )  RATIONAL_B_SPLINE_CURVE ( ( 1.000000000000000000, 0.9659258262890683122, 1.000000000000000000, 0.9659258262890683122, 1.000000000000000000, 0.9659258262890683122, 1.000000000000000000, 0.9659258262890683122, 1.000000000000000000, 0.9659258262890683122, 1.000000000000000000, 0.9659258262890683122, 1.000000000000000000 ) ) 
 REPRESENTATION_ITEM ( '' )  );
#66634=CARTESIAN_POINT ( 'NONE',  ( -0.2925321140481930704, -0.2925321140481933480, -0.6889763779527556808 ) ) ;
#66639=ADVANCED_FACE ( 'NONE', ( #15498 ), #28111, .T. ) ;
#66640=CARTESIAN_POINT ( 'NONE',  ( -0.2925321140481930704, -0.2925321140481933480, -2.893700787401574992 ) ) ;
#66641=CARTESIAN_POINT ( 'NONE',  ( 0.1974969037888706369, -0.3420746716998659953, -2.296587926509186417 ) ) ;
#66642=ORIENTED_EDGE ( 'NONE', *, *, #27425, .T. ) ;
#66644=CARTESIAN_POINT ( 'NONE',  ( 0.1049643490035304938, -0.3917322834645669549, -1.022309711286088829 ) ) ;
#66651=CARTESIAN_POINT ( 'NONE',  ( 0.1958661417322836162, -0.3392501089628018329, -0.4868573246381086017 ) ) ;
#66657=CARTESIAN_POINT ( 'NONE',  ( 0.2925321140481932369, -0.2925321140481932369, -2.933070866141732402 ) ) ;
#66658=CARTESIAN_POINT ( 'NONE',  ( -0.3917322834645670104, -0.1049643490035307020, -1.459993069062679005 ) ) ;
#66664=CARTESIAN_POINT ( 'NONE',  ( 0.2867679344610365999, 0.2867679344610365999, -0.6948818897637795144 ) ) ;
#66672=CARTESIAN_POINT ( 'NONE',  ( -0.1882840440700958018, -0.3436793299040552530, -1.929133858267716439 ) ) ;
#66674=CARTESIAN_POINT ( 'NONE',  ( -0.1958661417322834220, -0.3392501089628018884, -2.262467191601049699 ) ) ;
#66676=CARTESIAN_POINT ( 'NONE',  ( -9.787531504996567848E-17, 0.3996062992125986035, -0.4724409448818898127 ) ) ;
#66684=CARTESIAN_POINT ( 'NONE',  ( -0.2867679344610365999, 0.2867679344610364889, -1.364173228346456268 ) ) ;
#66685=EDGE_CURVE ( 'NONE', #45904, #58800, #80523, .T. ) ;
#66686=CARTESIAN_POINT ( 'NONE',  ( 0.1070741851644054776, -0.3996062992125984925, -1.894356955380577023 ) ) ;
#66690=VERTEX_POINT ( 'NONE', #7833 ) ;
#66706=CARTESIAN_POINT ( 'NONE',  ( -0.3917322834645670659, 0.1049643490035301607, -1.372684096291651556 ) ) ;
#66715=CARTESIAN_POINT ( 'NONE',  ( 4.797336870675656522E-17, -0.3917322834645670659, -0.07547863336714100146 ) ) ;
#66718=CARTESIAN_POINT ( 'NONE',  ( -0.3458507752293909498, 0.3458507752293907833, -1.671259842519685179 ) ) ;
#66733=CARTESIAN_POINT ( 'NONE',  ( -0.1058382717557497660, -0.3949938075777411073, 0.1660104986876640432 ) ) ;
#66739=CARTESIAN_POINT ( 'NONE',  ( -0.1070741851644056997, 0.3996062992125984925, -2.130577427821522818 ) ) ;
#66748=CARTESIAN_POINT ( 'NONE',  ( -0.1070741851644051862, -0.3996062992125987146, -1.174540682414698001 ) ) ;
#66749=CARTESIAN_POINT ( 'NONE',  ( -0.3420746716998659953, -0.1974969037888706647, -1.154855643044619518 ) ) ;
#66750=CARTESIAN_POINT ( 'NONE',  ( 0.1998031496062994405, -0.3460692066303958092, -2.296587926509186417 ) ) ;
#66752=CARTESIAN_POINT ( 'NONE',  ( -0.3392501089628019995, 0.1958661417322832277, -0.3333333333333333148 ) ) ;
#66756=CARTESIAN_POINT ( 'NONE',  ( -0.3949938075777409963, -7.255918531996591613E-17, -1.690944881889764329 ) ) ;
#66760=CARTESIAN_POINT ( 'NONE',  ( 0.1265901696524990294, -0.4724409448818896462, -2.132545931758530244 ) ) ;
#66769=CARTESIAN_POINT ( 'NONE',  ( 0.1049643490035303689, 0.3917322834645668994, -2.278195907315273327 ) ) ;
#66776=CARTESIAN_POINT ( 'NONE',  ( 0.1958661417322836440, -0.3392501089628017219, 0.1384514435695537171 ) ) ;
#66778=CARTESIAN_POINT ( 'NONE',  ( 0.2867679344610365999, 0.2867679344610365999, -1.704724409448818978 ) ) ;
#66781=CARTESIAN_POINT ( 'NONE',  ( -0.3949938075777409963, -7.255918531996591613E-17, -2.401574803149606474 ) ) ;
#66782=ORIENTED_EDGE ( 'NONE', *, *, #11244, .T. ) ;
#66786=CARTESIAN_POINT ( 'NONE',  ( -0.3460692066303960868, 0.1998031496062990242, -0.6561679790026246906 ) ) ;
#66791=CARTESIAN_POINT ( 'NONE',  ( -0.3917322834645669549, -0.1049643490035306603, 0.1843832020997374643 ) ) ;
#66797=CARTESIAN_POINT ( 'NONE',  ( -0.3917322834645669549, -0.1049643490035306603, -0.03805774278215218187 ) ) ;
#66802=CARTESIAN_POINT ( 'NONE',  ( -0.4724409448818899238, 0.1265901696524986686, -1.450131233595800317 ) ) ;
#66804=CARTESIAN_POINT ( 'NONE',  ( -0.3392501089628017219, -0.1958661417322836718, -0.6745406824146981117 ) ) ;
#66806=CARTESIAN_POINT ( 'NONE',  ( 4.797336870675656522E-17, -0.3917322834645670104, -2.525590551181102317 ) ) ;
#66810=CARTESIAN_POINT ( 'NONE',  ( -0.1070741851644051862, -0.3996062992125986590, 0.008530183727034094596 ) ) ;
#66815=CARTESIAN_POINT ( 'NONE',  ( 0.1958661417322836162, -0.3392501089628018329, 0.1430639352044112689 ) ) ;
#66817=CARTESIAN_POINT ( 'NONE',  ( -0.3392501089628017219, -0.1958661417322836718, -0.6095800524934383846 ) ) ;
#66822=CARTESIAN_POINT ( 'NONE',  ( 0.1958661417322836440, -0.3392501089628017219, -1.973753280839895208 ) ) ;
#66826=CARTESIAN_POINT ( 'NONE',  ( 0.4091458600556403535, 0.2362204724409449896, -0.5229658792650918597 ) ) ;
#66836=CARTESIAN_POINT ( 'NONE',  ( -0.3460692066303957537, -0.1998031496062994405, -1.389107611548556553 ) ) ;
#66846=CARTESIAN_POINT ( 'NONE',  ( -0.1998031496062994683, 0.3460692066303958092, -0.01312335958005250193 ) ) ;
#66847=CARTESIAN_POINT ( 'NONE',  ( -0.1974969037888706647, 0.3420746716998658843, -0.01312335958005255224 ) ) ;
#66853=CARTESIAN_POINT ( 'NONE',  ( -9.594673741351313045E-17, 0.3917322834645670104, -2.289370078740157410 ) ) ;
#66859=CARTESIAN_POINT ( 'NONE',  ( 0.4091458600556404646, -0.2362204724409448231, -0.5774278215223097588 ) ) ;
#66864=CARTESIAN_POINT ( 'NONE',  ( -0.3392501089628019995, 0.1958661417322831999, -0.3379458249681908666 ) ) ;
#66877=CARTESIAN_POINT ( 'NONE',  ( 0.3917322834645670104, 2.398668435337828261E-17, -0.4251968503937007537 ) ) ;
#66880=CARTESIAN_POINT ( 'NONE',  ( 0.2891555358219910499, 0.2891555358219910499, -1.240157480314960869 ) ) ;
#66891=CARTESIAN_POINT ( 'NONE',  ( 5.785732909357575061E-17, -0.4724409448818898682, -0.6279527559055118058 ) ) ;
#66896=CARTESIAN_POINT ( 'NONE',  ( 0.2925321140481932369, -0.2925321140481932369, -1.673228346456692828 ) ) ;
#66899=CARTESIAN_POINT ( 'NONE',  ( 0.2925321140481932369, -0.2925321140481931814, -0.9625984251968502381 ) ) ;
#66900=CARTESIAN_POINT ( 'NONE',  ( 0.1070741851644054776, -0.3996062992125984925, -0.6345144356955381149 ) ) ;
#66902=CARTESIAN_POINT ( 'NONE',  ( -0.4091458600556405756, 0.2362204724409446288, 0.1312335958005249326 ) ) ;
#66903=CARTESIAN_POINT ( 'NONE',  ( -0.2867679344610365999, 0.2867679344610364889, -2.624015748031495399 ) ) ;
#66909=CARTESIAN_POINT ( 'NONE',  ( 0.2362204724409451007, -0.4091458600556402980, -2.058398950131233640 ) ) ;
#66912=CARTESIAN_POINT ( 'NONE',  ( 0.3420746716998660508, -0.1974969037888704149, -1.756561679790026309 ) ) ;
#66921=CARTESIAN_POINT ( 'NONE',  ( -0.3996062992125984925, -0.1070741851644056858, -2.642388451443570041 ) ) ;
#66923=CARTESIAN_POINT ( 'NONE',  ( 0.1049643490035303689, 0.3917322834645668994, -2.435676222275903857 ) ) ;
#66935=CARTESIAN_POINT ( 'NONE',  ( 0.3460692066303959202, -0.1998031496062991630, -0.3392388451443569819 ) ) ;
#66938=CARTESIAN_POINT ( 'NONE',  ( -0.3392501089628017219, -0.1958661417322836718, -1.869422572178477848 ) ) ;
#66947=CARTESIAN_POINT ( 'NONE',  ( 0.3460692066303958092, 0.1998031496062993018, -0.8379265091863516979 ) ) ;
#66961=CARTESIAN_POINT ( 'NONE',  ( -0.3996062992125986035, -0.1070741851644056997, -0.6758530183727035068 ) ) ;
#66964=CARTESIAN_POINT ( 'NONE',  ( 0.3392501089628018884, -0.1958661417322834220, -2.144356955380577467 ) ) ;
#66974=CARTESIAN_POINT ( 'NONE',  ( -0.3917322834645669549, -7.196005306013483243E-17, -1.379245776081677866 ) ) ;
#66980=CARTESIAN_POINT ( 'NONE',  ( 0.3949938075777411073, -0.1058382717557499464, 0.04593175853018367782 ) ) ;
#66990=CARTESIAN_POINT ( 'NONE',  ( -0.3392501089628019995, 0.1958661417322832277, -2.315616797900262647 ) ) ;
#66997=CARTESIAN_POINT ( 'NONE',  ( -9.787531504996566615E-17, 0.3996062992125985480, -0.07677165354330710290 ) ) ;
#66999=CARTESIAN_POINT ( 'NONE',  ( -0.1070741851644056997, 0.3996062992125986035, -1.896325459317584894 ) ) ;
#67004=CARTESIAN_POINT ( 'NONE',  ( 0.4724409448818897572, -0.1265901696524988906, -0.6607611548556431291 ) ) ;
#67007=CARTESIAN_POINT ( 'NONE',  ( -0.1058382717557503072, 0.3949938075777408852, -0.5557742782152231831 ) ) ;
#67012=CARTESIAN_POINT ( 'NONE',  ( -0.1974969037888706924, 0.3420746716998658843, -0.4048556430446195176 ) ) ;
#67019=CARTESIAN_POINT ( 'NONE',  ( -0.1998031496062994405, 0.3460692066303957537, -1.349737532808399143 ) ) ;
#67021=CARTESIAN_POINT ( 'NONE',  ( -0.1049643490035307020, 0.3917322834645669549, -1.101049868766403872 ) ) ;
#67023=CARTESIAN_POINT ( 'NONE',  ( -0.2502216998114409341, 0.3021538998228462392, 1.649893717844496181E-17 ) ) ;
#67049=CARTESIAN_POINT ( 'NONE',  ( -0.1998031496062991907, -0.3460692066303959757, -0.6955380577427822120 ) ) ;
#67053=CARTESIAN_POINT ( 'NONE',  ( 0.4091458600556404646, -0.2362204724409448231, 0.05249343832020997302 ) ) ;
#67054=CARTESIAN_POINT ( 'NONE',  ( 0.3420746716998660508, -0.1974969037888703871, -2.467191601049868677 ) ) ;
#67057=CARTESIAN_POINT ( 'NONE',  ( -0.3917322834645671215, 0.1049643490035301469, -1.127296587926509108 ) ) ;
#67062=EDGE_CURVE ( 'NONE', #25317, #51716, #48191, .T. ) ;
#67064=CARTESIAN_POINT ( 'NONE',  ( 0.3917322834645669549, 2.398668435337827645E-17, -0.3556237288375834749 ) ) ;
#67071=CARTESIAN_POINT ( 'NONE',  ( 0.2362204724409449064, 0.4091458600556404646, -1.089238845144356871 ) ) ;
#67072=CARTESIAN_POINT ( 'NONE',  ( -0.1049643490035302301, -0.3917322834645671770, -1.643720103183414105 ) ) ;
#67078=CARTESIAN_POINT ( 'NONE',  ( -0.2867679344610364334, -0.2867679344610367109, -1.088582677165354173 ) ) ;
#67088=CARTESIAN_POINT ( 'NONE',  ( 0.1049643490035304938, -0.3917322834645669549, -2.282152230971128404 ) ) ;
#67098=CARTESIAN_POINT ( 'NONE',  ( 0.3392501089628018884, -0.1958661417322834220, -1.134514435695538115 ) ) ;
#67099=CARTESIAN_POINT ( 'NONE',  ( -0.3996062992125986590, 0.1070741851644051723, -2.314304461942256808 ) ) ;
#67107=CARTESIAN_POINT ( 'NONE',  ( -0.1998031496062994405, 0.3460692066303957537, -2.137139107611548905 ) ) ;
#67109=LINE ( 'NONE', #9032, #16785 ) ;
#67116=CARTESIAN_POINT ( 'NONE',  ( 0.3917322834645668994, 0.1049643490035304522, -1.149586983430759490 ) ) ;
#67126=CARTESIAN_POINT ( 'NONE',  ( -0.1049643490035307158, 0.3917322834645670104, -0.6332214155193720551 ) ) ;
#67129=CARTESIAN_POINT ( 'NONE',  ( 0.4724409448818898682, 2.892866454678787531E-17, -1.769685039370078927 ) ) ;
#67148=CARTESIAN_POINT ( 'NONE',  ( -0.1070741851644051862, -0.3996062992125986590, -2.826115485564304475 ) ) ;
#67153=CARTESIAN_POINT ( 'NONE',  ( -0.2925321140481930149, -0.2925321140481933480, -2.183070866141731958 ) ) ;
#67159=CARTESIAN_POINT ( 'NONE',  ( 0.1070741851644053527, 0.3996062992125986590, -1.725721784776903078 ) ) ;
#67160=CARTESIAN_POINT ( 'NONE',  ( 0.3949938075777409408, 0.1058382717557500574, -1.227034120734908473 ) ) ;
#67161=CARTESIAN_POINT ( 'NONE',  ( -0.3460692066303960868, 0.1998031496062990242, -2.388451443569553856 ) ) ;
#67163=CARTESIAN_POINT ( 'NONE',  ( -0.1958661417322836718, 0.3392501089628017219, -0.1627296587926508609 ) ) ;
#67167=CARTESIAN_POINT ( 'NONE',  ( 0.1058382717557500852, -0.3949938075777408852, -2.051837270341207109 ) ) ;
#67172=CARTESIAN_POINT ( 'NONE',  ( 0.1265901696524990294, -0.4724409448818896462, -2.290026246719159442 ) ) ;
#67173=CARTESIAN_POINT ( 'NONE',  ( 0.1070741851644053527, 0.3996062992125986590, -1.883202099737532276 ) ) ;
#67181=CARTESIAN_POINT ( 'NONE',  ( 4.797336870675656522E-17, -0.3917322834645670104, 0.1515748031496061965 ) ) ;
#67187=CARTESIAN_POINT ( 'NONE',  ( 0.3392501089628018884, -0.1958661417322834220, -0.3471128608923885195 ) ) ;
#67189=CARTESIAN_POINT ( 'NONE',  ( -0.1049643490035307020, 0.3917322834645669549, -2.360892388451444113 ) ) ;
#67192=CARTESIAN_POINT ( 'NONE',  ( 0.1058382717557499880, 0.3949938075777411073, -2.355643044619422533 ) ) ;
#67196=CARTESIAN_POINT ( 'NONE',  ( 0.2925321140481932369, -0.2925321140481932369, -1.043307086614173151 ) ) ;
#67198=CARTESIAN_POINT ( 'NONE',  ( -0.2017716535433071445, 0.2017716535433070613, -0.3937007874015748254 ) ) ;
#67201=CARTESIAN_POINT ( 'NONE',  ( -0.3917322834645670104, -7.196005306013484475E-17, -0.1240157480314961758 ) ) ;
#67207=CARTESIAN_POINT ( 'NONE',  ( -0.1049643490035302024, -0.3917322834645671215, -0.06430446194225715451 ) ) ;
#67211=( NAMED_UNIT ( * ) PLANE_ANGLE_UNIT ( ) SI_UNIT ( $, .RADIAN. ) );
#67212=CARTESIAN_POINT ( 'NONE',  ( 0.4724409448818896462, 0.1265901696524990294, -1.856955380577427928 ) ) ;
#67214=CARTESIAN_POINT ( 'NONE',  ( -9.594673741351313045E-17, 0.3917322834645670104, -0.6220472440944880832 ) ) ;
#67215=CARTESIAN_POINT ( 'NONE',  ( 0.3917322834645669549, 0.1049643490035304660, -2.256561679790026531 ) ) ;
#67218=CARTESIAN_POINT ( 'NONE',  ( 0.2925321140481932369, 0.2925321140481932369, -0.5295275590551181688 ) ) ;
#67224=CARTESIAN_POINT ( 'NONE',  ( 0.1958661417322836162, -0.3392501089628018329, -0.1718966947168485970 ) ) ;
#67227=CARTESIAN_POINT ( 'NONE',  ( -0.1049643490035301885, -0.3917322834645671215, -0.4717847769028871707 ) ) ;
#67228=EDGE_CURVE ( 'NONE', #23851, #72980, #71831, .T. ) ;
#67233=CARTESIAN_POINT ( 'NONE',  ( 0.1049643490035304938, -0.3917322834645669549, -2.282152230971128404 ) ) ;
#67236=CARTESIAN_POINT ( 'NONE',  ( 0.2362204724409451007, -0.4091458600556402980, -0.1686351706036745557 ) ) ;
#67247=CARTESIAN_POINT ( 'NONE',  ( -0.1998031496062994405, 0.3460692066303957537, -1.664698162729658426 ) ) ;
#67255=CARTESIAN_POINT ( 'NONE',  ( -0.1998031496062991630, -0.3460692066303959202, -0.1423884514435695692 ) ) ;
#67256=CARTESIAN_POINT ( 'NONE',  ( 0.3460692066303959202, 0.1998031496062993295, -0.4461942257217847430 ) ) ;
#67257=CARTESIAN_POINT ( 'NONE',  ( -0.1958661417322833942, -0.3392501089628018884, -2.739520628117797063 ) ) ;
#67263=CARTESIAN_POINT ( 'NONE',  ( -0.2891555358219911054, 0.2891555358219909388, -0.7263779527559056648 ) ) ;
#67268=CARTESIAN_POINT ( 'NONE',  ( 0.4091458600556404646, -0.2362204724409448231, -0.8923884514435694859 ) ) ;
#67269=CARTESIAN_POINT ( 'NONE',  ( -0.1998031496062991907, -0.3460692066303959757, -2.112860892388451539 ) ) ;
#67272=CARTESIAN_POINT ( 'NONE',  ( 0.1049643490035303967, 0.3917322834645670659, -0.4626177409786895178 ) ) ;
#67284=CARTESIAN_POINT ( 'NONE',  ( 0.1049643490035303689, 0.3917322834645670104, -0.4580052493438320216 ) ) ;
#67287=CARTESIAN_POINT ( 'NONE',  ( 4.837279021331060870E-17, -0.3949938075777409963, -1.023622047244094446 ) ) ;
#67297=CARTESIAN_POINT ( 'NONE',  ( -0.4091458600556402980, -0.2362204724409451284, -0.9973753280839895430 ) ) ;
#67303=CARTESIAN_POINT ( 'NONE',  ( -0.2925321140481930704, -0.2925321140481933480, -1.633858267716534973 ) ) ;
#67306=CARTESIAN_POINT ( 'NONE',  ( -0.1998031496062991630, -0.3460692066303959202, -1.244750656167979086 ) ) ;
#67307=CARTESIAN_POINT ( 'NONE',  ( 0.2925321140481932369, -0.2925321140481931814, -0.6476377952755905110 ) ) ;
#67310=CARTESIAN_POINT ( 'NONE',  ( -0.4724409448818898682, -8.678599364036362592E-17, 0.1181102362204724532 ) ) ;
#67311=CARTESIAN_POINT ( 'NONE',  ( -0.1958661417322834220, -0.3392501089628018884, -2.669947506561679784 ) ) ;
#67317=CARTESIAN_POINT ( 'NONE',  ( -0.2362204724409447953, -0.4091458600556404646, -1.874671916010498762 ) ) ;
#67321=CARTESIAN_POINT ( 'NONE',  ( 0.1058382717557499880, 0.3949938075777409408, -1.645013123359580831 ) ) ;
#67331=CARTESIAN_POINT ( 'NONE',  ( -0.3996062992125986590, 0.1070741851644051723, -2.471784776902887337 ) ) ;
#67333=CARTESIAN_POINT ( 'NONE',  ( 0.2867679344610365999, -0.2867679344610365999, -2.383182783955693829 ) ) ;
#67345=CARTESIAN_POINT ( 'NONE',  ( -0.3460692066303960313, 0.1998031496062989965, -0.4179790026246719137 ) ) ;
#67347=CARTESIAN_POINT ( 'NONE',  ( 0.3917322834645670104, 2.398668435337828261E-17, -1.777559055118110409 ) ) ;
#67356=CARTESIAN_POINT ( 'NONE',  ( -0.2925321140481930149, -0.2925321140481933480, -0.9232283464566929387 ) ) ;
#67365=CARTESIAN_POINT ( 'NONE',  ( 0.3021538998228436301, 0.2502216998114438762, -1.220472440944881942 ) ) ;
#67368=CARTESIAN_POINT ( 'NONE',  ( 0.4724409448818898682, 2.892866454678787531E-17, -0.4330708661417322913 ) ) ;
#67371=CARTESIAN_POINT ( 'NONE',  ( 0.1070741851644054915, -0.3996062992125986035, -0.4002624671916010235 ) ) ;
#67374=CARTESIAN_POINT ( 'NONE',  ( 0.2867679344610365999, 0.2867679344610365999, -2.019685039370078261 ) ) ;
#67384=CARTESIAN_POINT ( 'NONE',  ( -0.3917322834645669549, -7.196005306013483243E-17, -1.536726091042307951 ) ) ;
#67390=CARTESIAN_POINT ( 'NONE',  ( -0.1958661417322833942, -0.3392501089628018884, -2.897000943078426705 ) ) ;
#67398=CARTESIAN_POINT ( 'NONE',  ( 0.3917322834645670104, 0.1049643490035304660, -1.066292281661104457 ) ) ;
#67400=CARTESIAN_POINT ( 'NONE',  ( 0.3392501089628018884, -0.1958661417322834220, -2.394356955380577467 ) ) ;
#67408=CARTESIAN_POINT ( 'NONE',  ( 0.1998031496062992740, 0.3460692066303959757, -1.719160104986876769 ) ) ;
#67413=CARTESIAN_POINT ( 'NONE',  ( 0.4091458600556404646, -0.2362204724409448231, -0.4967191601049869010 ) ) ;
#67417=CARTESIAN_POINT ( 'NONE',  ( 0.3949938075777409408, -0.1058382717557499186, -0.5032808398950131545 ) ) ;
#67422=CARTESIAN_POINT ( 'NONE',  ( -0.3949938075777408852, -0.1058382717557502933, -0.5951443569553805935 ) ) ;
#67429=CARTESIAN_POINT ( 'NONE',  ( 0.3460692066303959202, -0.1998031496062991630, -1.441601049868766582 ) ) ;
#67431=CARTESIAN_POINT ( 'NONE',  ( 0.3392501089628018884, -0.1958661417322834220, -0.8845144356955378928 ) ) ;
#67433=CARTESIAN_POINT ( 'NONE',  ( -0.3796925558546807578, -0.09865214182457832104, -3.091116300196737326E-17 ) ) ;
#67446=CARTESIAN_POINT ( 'NONE',  ( 0.000000000000000000, 0.000000000000000000, -2.755905511811024056 ) ) ;
#67459=CARTESIAN_POINT ( 'NONE',  ( 0.3460692066303959757, -0.1998031496062991907, -1.049868766404199460 ) ) ;
#67463=CARTESIAN_POINT ( 'NONE',  ( -0.4091458600556402980, -0.2362204724409451284, -0.05249343832020997302 ) ) ;
#67464=CARTESIAN_POINT ( 'NONE',  ( -9.674558042662121740E-17, 0.3949938075777409963, -2.519685039370078705 ) ) ;
#67467=CARTESIAN_POINT ( 'NONE',  ( -0.1049643490035302024, -0.3917322834645671215, -1.009186351706036433 ) ) ;
#67475=CARTESIAN_POINT ( 'NONE',  ( -0.3917322834645670659, 0.1049643490035301607, -0.2703218915672423450 ) ) ;
#67482=CARTESIAN_POINT ( 'NONE',  ( -0.3917322834645671770, 0.1049643490035302024, -1.604350024443256695 ) ) ;
#67488=CARTESIAN_POINT ( 'NONE',  ( -0.2867679344610364334, -0.2867679344610367109, -0.9311023622047245318 ) ) ;
#67497=CARTESIAN_POINT ( 'NONE',  ( -0.4724409448818898682, -8.678599364036362592E-17, -0.9035433070866141225 ) ) ;
#67498=CARTESIAN_POINT ( 'NONE',  ( -0.3917322834645670104, -7.196005306013484475E-17, -2.393700787401574992 ) ) ;
#67505=CARTESIAN_POINT ( 'NONE',  ( -0.1958661417322834220, -0.3392501089628018884, -0.6227034120734910028 ) ) ;
#67507=CARTESIAN_POINT ( 'NONE',  ( -0.1958661417322834220, -0.3392501089628018884, -1.410104986876640654 ) ) ;
#67508=CARTESIAN_POINT ( 'NONE',  ( -0.3460692066303960313, 0.1998031496062989965, -2.465223097112860806 ) ) ;
#67527=CARTESIAN_POINT ( 'NONE',  ( 0.2867679344610365999, -0.2867679344610365999, -1.438300894191914425 ) ) ;
#67537=CARTESIAN_POINT ( 'NONE',  ( -0.3392501089628019995, 0.1958661417322831999, -0.6529064548894508713 ) ) ;
#67539=( BOUNDED_CURVE ( )  B_SPLINE_CURVE ( 2, ( #33059, #7818, #58729, #52398, #59147, #1504, #20855, #46507, #29651, #61646, #16629, #54905, #30062 ),
 .UNSPECIFIED., .F., .F. ) 
 B_SPLINE_CURVE_WITH_KNOTS ( ( 3, 2, 2, 2, 2, 2, 3 ),
 ( 0.7374999999999999334, 0.7416666666666665853, 0.7458333333333333481, 0.7500000000000000000, 0.7541666666666666519, 0.7583333333333334147, 0.7625000000000000666 ),
 .UNSPECIFIED. ) 
 CURVE ( )  GEOMETRIC_REPRESENTATION_ITEM ( )  RATIONAL_B_SPLINE_CURVE ( ( 1.000000000000000888, 0.9659258262890674240, 1.000000000000000000, 0.9659258262890683122, 1.000000000000000000, 0.9659258262890683122, 1.000000000000000000, 0.9659258262890683122, 1.000000000000000000, 0.9659258262890683122, 1.000000000000000000, 0.9659258262890674240, 1.000000000000000888 ) ) 
 REPRESENTATION_ITEM ( '' )  );
#67541=CARTESIAN_POINT ( 'NONE',  ( 0.4724409448818898682, 2.892866454678787531E-17, -0.2755905511811023723 ) ) ;
#67542=CARTESIAN_POINT ( 'NONE',  ( 5.785732909357575061E-17, -0.4724409448818898682, -2.045275590551181022 ) ) ;
#67565=CARTESIAN_POINT ( 'NONE',  ( 0.1998031496062994128, -0.3460692066303957537, -2.215879265091863726 ) ) ;
#67570=CARTESIAN_POINT ( 'NONE',  ( -0.3460692066303960868, 0.1998031496062990242, -1.601049868766404094 ) ) ;
#67571=CARTESIAN_POINT ( 'NONE',  ( 0.1058382717557499880, 0.3949938075777411073, -1.095800524934383180 ) ) ;
#67572=CARTESIAN_POINT ( 'NONE',  ( 0.1998031496062992740, 0.3460692066303959757, -2.664041994750656173 ) ) ;
#67574=CARTESIAN_POINT ( 'NONE',  ( -0.3917322834645671215, 0.1049643490035301469, -0.02493438320209968861 ) ) ;
#67578=CARTESIAN_POINT ( 'NONE',  ( 0.2891555358219910499, -0.2891555358219909944, -2.064960629921260171 ) ) ;
#67582=CARTESIAN_POINT ( 'NONE',  ( -0.3458507752293906723, -0.3458507752293910609, -2.578740157480315265 ) ) ;
#67583=CARTESIAN_POINT ( 'NONE',  ( 0.3996062992125986035, 0.1070741851644054776, -1.699475065616798064 ) ) ;
#67584=CARTESIAN_POINT ( 'NONE',  ( 0.2362204724409449064, 0.4091458600556404646, -2.740813648293963567 ) ) ;
#67586=EDGE_LOOP ( 'NONE', ( #24668, #54134, #74832, #41911 ) ) ;
#67592=CARTESIAN_POINT ( 'NONE',  ( -0.3917322834645671215, 0.1049643490035301469, 0.1975065616797899160 ) ) ;
#67599=CARTESIAN_POINT ( 'NONE',  ( 0.3917322834645670104, -0.1049643490035303411, -0.1961942257217848817 ) ) ;
#67601=CARTESIAN_POINT ( 'NONE',  ( 0.3917322834645670104, 2.398668435337828261E-17, -2.157480314960630086 ) ) ;
#67604=CARTESIAN_POINT ( 'NONE',  ( -0.1974969037888703871, -0.3420746716998661063, -2.112860892388451539 ) ) ;
#67608=CARTESIAN_POINT ( 'NONE',  ( 0.2925321140481932369, 0.2925321140481932369, -1.082677165354330562 ) ) ;
#67610=CARTESIAN_POINT ( 'NONE',  ( -0.3458507752293906723, -0.3458507752293910609, -0.7657480314960628531 ) ) ;
#67612=CARTESIAN_POINT ( 'NONE',  ( 0.004548682155579284771, -0.3974711515625322655, -2.755905511811026276 ) ) ;
#67613=CARTESIAN_POINT ( 'NONE',  ( 0.3917322834645670104, 2.398668435337828261E-17, -0.2027559055118111353 ) ) ;
#67620=CARTESIAN_POINT ( 'NONE',  ( 0.1049643490035304938, -0.3917322834645669549, -0.07742782152230967552 ) ) ;
#67623=DIRECTION ( 'NONE',  ( 0.000000000000000000, 0.000000000000000000, 1.000000000000000000 ) ) ;
#67625=CARTESIAN_POINT ( 'NONE',  ( 0.4091458600556404646, -0.2362204724409448231, -1.522309711286089273 ) ) ;
#67628=CARTESIAN_POINT ( 'NONE',  ( 0.1049643490035304938, -0.3917322834645669549, -0.8648293963254591876 ) ) ;
#67630=CARTESIAN_POINT ( 'NONE',  ( 0.1467283321115955275, 0.3676198365746946584, -2.752234641088710632 ) ) ;
#67637=CARTESIAN_POINT ( 'NONE',  ( -0.1958661417322834497, -0.3392501089628018884, 0.1693106543645162554 ) ) ;
#67639=CARTESIAN_POINT ( 'NONE',  ( -0.2867679344610364334, -0.2867679344610367109, -0.4586614173228347746 ) ) ;
#67644=CARTESIAN_POINT ( 'NONE',  ( -0.1958661417322834220, -0.3392501089628018884, -2.419947506561679784 ) ) ;
#67647=CARTESIAN_POINT ( 'NONE',  ( 0.1265901696524990294, -0.4724409448818896462, -0.3195538057742782212 ) ) ;
#67658=CARTESIAN_POINT ( 'NONE',  ( 0.3996062992125984925, 0.1070741851644054637, -1.461286089238844843 ) ) ;
#67666=CARTESIAN_POINT ( 'NONE',  ( 0.3460692066303959202, -0.1998031496062991630, -0.3392388451443569819 ) ) ;
#67667=CARTESIAN_POINT ( 'NONE',  ( -0.2925321140481930704, -0.2925321140481933480, -0.6889763779527556808 ) ) ;
#67669=CARTESIAN_POINT ( 'NONE',  ( -0.2867679344610365444, -0.2867679344610367664, -2.890439263288400618 ) ) ;
#67675=CARTESIAN_POINT ( 'NONE',  ( -0.1058382717557497660, -0.3949938075777411073, -0.7788713910761156933 ) ) ;
#67680=CARTESIAN_POINT ( 'NONE',  ( 0.4724409448818896462, 0.1265901696524990294, -1.227034120734908029 ) ) ;
#67681=CARTESIAN_POINT ( 'NONE',  ( 0.2925321140481932369, 0.2925321140481932369, -2.342519685039369914 ) ) ;
#67685=CARTESIAN_POINT ( 'NONE',  ( -0.3917322834645671770, 0.1049643490035302024, -0.3445075047582172312 ) ) ;
#67697=CARTESIAN_POINT ( 'NONE',  ( 0.3392501089628018884, -0.1958661417322834220, -1.041994750656167756 ) ) ;
#67700=CARTESIAN_POINT ( 'NONE',  ( -0.1058382717557497937, -0.3949938075777411628, -0.8595800524934383846 ) ) ;
#67710=CARTESIAN_POINT ( 'NONE',  ( -0.4724409448818904234, 0.1265901696524979470, -0.4245406824146981117 ) ) ;
#67711=CARTESIAN_POINT ( 'NONE',  ( -0.2362204724409447953, -0.4091458600556404646, -0.6148293963254594097 ) ) ;
#67717=CARTESIAN_POINT ( 'NONE',  ( -0.1998031496062991907, -0.3460692066303959757, -1.640419947506561726 ) ) ;
#67720=CARTESIAN_POINT ( 'NONE',  ( -0.3996062992125985480, -7.340648628747423112E-17, -1.061023622047243986 ) ) ;
#67724=CARTESIAN_POINT ( 'NONE',  ( -0.1265901696524993347, 0.4724409448818895907, -0.6364829396325458744 ) ) ;
#67726=CARTESIAN_POINT ( 'NONE',  ( 0.3392501089628018884, -0.1958661417322834220, -2.709317585301837195 ) ) ;
#67732=CARTESIAN_POINT ( 'NONE',  ( 0.3458507752293908943, -0.3458507752293908943, -2.379921259842520342 ) ) ;
#67737=CARTESIAN_POINT ( 'NONE',  ( 0.3949938075777408852, 0.1058382717557500435, -1.933727034120735100 ) ) ;
#67747=CARTESIAN_POINT ( 'NONE',  ( 0.3392501089628018329, 0.1958661417322835052, -2.573471497866454794 ) ) ;
#67760=CARTESIAN_POINT ( 'NONE',  ( -0.2925321140481930149, -0.2925321140481933480, -0.2933070866141732069 ) ) ;
#67762=CARTESIAN_POINT ( 'NONE',  ( -0.1049643490035307020, 0.3917322834645669549, -1.823490813648294129 ) ) ;
#67771=CARTESIAN_POINT ( 'NONE',  ( 0.2925321140481932369, -0.2925321140481931814, -1.120078740157480324 ) ) ;
#67773=CARTESIAN_POINT ( 'NONE',  ( 0.4724409448818898682, 2.892866454678787531E-17, -2.165354330708661568 ) ) ;
#67779=CARTESIAN_POINT ( 'NONE',  ( -0.3392501089628017219, -0.1958661417322836718, -1.396981627296587813 ) ) ;
#67780=CARTESIAN_POINT ( 'NONE',  ( 0.3401783215957711048, 0.1988659768032686181, -1.220472440944881720 ) ) ;
#67784=CARTESIAN_POINT ( 'NONE',  ( -0.3996062992125985480, -7.340648628747423112E-17, -2.320866141732283783 ) ) ;
#67787=CARTESIAN_POINT ( 'NONE',  ( 0.3460692066303959202, 0.1998031496062993295, -0.6036745406824146620 ) ) ;
#67790=AXIS2_PLACEMENT_3D ( 'NONE', #82161, #30793, #56867 ) ;
#67791=CARTESIAN_POINT ( 'NONE',  ( 0.3917322834645670104, -0.1049643490035303411, -2.150918635170603554 ) ) ;
#67801=CARTESIAN_POINT ( 'NONE',  ( -0.3917322834645668994, -0.1049643490035306742, -1.385807455871704175 ) ) ;
#67805=CARTESIAN_POINT ( 'NONE',  ( -0.3392501089628017219, -0.1958661417322836718, 0.1128608923884514836 ) ) ;
#67808=CARTESIAN_POINT ( 'NONE',  ( -0.3949938075777409963, -7.255918531996591613E-17, 0.1181102362204723977 ) ) ;
#67816=CARTESIAN_POINT ( 'NONE',  ( 0.1958661417322836718, -0.3392501089628017219, -1.348444512632232861 ) ) ;
#67818=CARTESIAN_POINT ( 'NONE',  ( 0.1958661417322834775, 0.3392501089628018884, -2.433727034120734878 ) ) ;
#67824=CARTESIAN_POINT ( 'NONE',  ( 0.1070741851644054776, -0.3996062992125984925, 0.1528871391076115360 ) ) ;
#67826=CARTESIAN_POINT ( 'NONE',  ( -0.3460692066303960868, 0.1998031496062990242, -2.388451443569553856 ) ) ;
#67831=CARTESIAN_POINT ( 'NONE',  ( 0.4724409448818897572, -0.1265901696524988906, -1.290682414698162583 ) ) ;
#67834=CARTESIAN_POINT ( 'NONE',  ( -0.3420746716998660508, -0.1974969037888706924, -0.7591863517060368771 ) ) ;
#67839=CARTESIAN_POINT ( 'NONE',  ( -9.674558042662122972E-17, 0.3949938075777409963, -0.5492125984251968740 ) ) ;
#67847=CARTESIAN_POINT ( 'NONE',  ( 0.2925321140481932369, -0.2925321140481931814, -1.435039370078740495 ) ) ;
#67849=CARTESIAN_POINT ( 'NONE',  ( -0.2867679344610365999, 0.2867679344610364889, -1.114173228346456712 ) ) ;
#67851=CARTESIAN_POINT ( 'NONE',  ( -0.09156050430092219083, -0.3808816823641230087, -1.492482962822815952E-17 ) ) ;
#67860=( BOUNDED_CURVE ( )  B_SPLINE_CURVE ( 2, ( #76144, #37420, #13412, #44945, #18883, #57167, #70642, #82866, #39067, #12998, #50855, #5834, #64750 ),
 .UNSPECIFIED., .F., .F. ) 
 B_SPLINE_CURVE_WITH_KNOTS ( ( 3, 2, 2, 2, 2, 2, 3 ),
 ( 0.2624999999999999556, 0.2666666666666666075, 0.2708333333333333148, 0.2750000000000000222, 0.2791666666666666741, 0.2833333333333333814, 0.2875000000000000333 ),
 .UNSPECIFIED. ) 
 CURVE ( )  GEOMETRIC_REPRESENTATION_ITEM ( )  RATIONAL_B_SPLINE_CURVE ( ( 1.000000000000000444, 0.9659258262890678681, 1.000000000000000000, 0.9659258262890683122, 1.000000000000000000, 0.9659258262890683122, 1.000000000000000000, 0.9659258262890683122, 1.000000000000000000, 0.9659258262890683122, 1.000000000000000000, 0.9659258262890678681, 1.000000000000000444 ) ) 
 REPRESENTATION_ITEM ( '' )  );
#67861=CARTESIAN_POINT ( 'NONE',  ( 0.3458507752293908943, 0.3458507752293908943, -0.2145669291338582751 ) ) ;
#67875=EDGE_CURVE ( 'NONE', #60134, #72980, #7998, .T. ) ;
#67878=CARTESIAN_POINT ( 'NONE',  ( 0.1998031496062994405, -0.3460692066303958092, -1.194225721784776928 ) ) ;
#67882=CARTESIAN_POINT ( 'NONE',  ( -0.4724409448818899238, 0.1265901696524986686, -0.03280839895013123314 ) ) ;
#67883=CARTESIAN_POINT ( 'NONE',  ( -0.3949938075777411628, 0.1058382717557497937, -2.552493438320210473 ) ) ;
#67886=CARTESIAN_POINT ( 'NONE',  ( 0.1049643490035303689, 0.3917322834645670104, -1.087926509186351476 ) ) ;
#67888=CARTESIAN_POINT ( 'NONE',  ( -1.157146581871515012E-16, 0.4724409448818898682, -2.362204724409448620 ) ) ;
#67890=CARTESIAN_POINT ( 'NONE',  ( 0.4724409448818898682, 2.892866454678787531E-17, -0.8248031496062991907 ) ) ;
#67895=CARTESIAN_POINT ( 'NONE',  ( -0.2867679344610366554, 0.2867679344610365444, -0.2571985319871897824 ) ) ;
#67901=CARTESIAN_POINT ( 'NONE',  ( -0.1998031496062991907, -0.3460692066303959757, -2.900262467191600635 ) ) ;
#67902=CARTESIAN_POINT ( 'NONE',  ( -9.594673741351313045E-17, 0.3917322834645670659, -1.571541625493125149 ) ) ;
#67909=CARTESIAN_POINT ( 'NONE',  ( 0.1958661417322836440, -0.3392501089628017219, -0.8064304461942258806 ) ) ;
#67917=CARTESIAN_POINT ( 'NONE',  ( 0.3392501089628018884, -0.1958661417322834220, -2.144356955380577467 ) ) ;
#67924=CARTESIAN_POINT ( 'NONE',  ( -0.1049643490035307020, 0.3917322834645669549, -0.8786089238845143923 ) ) ;
#67926=CARTESIAN_POINT ( 'NONE',  ( 0.3996062992125984925, 0.1070741851644054637, -2.248687664041994605 ) ) ;
#67937=CARTESIAN_POINT ( 'NONE',  ( -0.2867679344610365999, 0.2867679344610364889, -0.01181102362204719709 ) ) ;
#67944=CARTESIAN_POINT ( 'NONE',  ( -9.594673741351310580E-17, 0.3917322834645669549, -1.654836327262780182 ) ) ;
#67952=CARTESIAN_POINT ( 'NONE',  ( 4.797336870675656522E-17, -0.3917322834645670659, -0.3904392632884007841 ) ) ;
#67956=CARTESIAN_POINT ( 'NONE',  ( -0.4091458600556405756, 0.2362204724409446288, -2.150262467191601079 ) ) ;
#67979=CARTESIAN_POINT ( 'NONE',  ( -0.2925321140481932369, 0.2925321140481931259, -2.301181102362204633 ) ) ;
#67984=CARTESIAN_POINT ( 'NONE',  ( -0.3996062992125986035, -7.340648628747425578E-17, -1.929133858267716439 ) ) ;
#67985=CARTESIAN_POINT ( 'NONE',  ( -0.3420746716998661618, 0.1974969037888702206, -1.286089238845144367 ) ) ;
#67986=CARTESIAN_POINT ( 'NONE',  ( 0.1998031496062992740, 0.3460692066303959757, -2.349081364829396446 ) ) ;
#67987=CARTESIAN_POINT ( 'NONE',  ( -0.3458507752293909498, 0.3458507752293908388, -0.6496062992125984925 ) ) ;
#67988=CARTESIAN_POINT ( 'NONE',  ( -0.1049643490035301885, -0.3917322834645671215, -0.2217847769028870319 ) ) ;
#67992=CARTESIAN_POINT ( 'NONE',  ( 0.3949938075777409408, -0.1058382717557499186, -2.235564304461942431 ) ) ;
#67996=CARTESIAN_POINT ( 'NONE',  ( -0.4091458600556402980, -0.2362204724409451284, -2.257217847769029007 ) ) ;
#67997=CARTESIAN_POINT ( 'NONE',  ( 0.1998031496062992740, 0.3460692066303959757, -1.719160104986876769 ) ) ;
#68005=CARTESIAN_POINT ( 'NONE',  ( 0.3392501089628018329, 0.1958661417322835607, 0.09908136482939623735 ) ) ;
#68013=CARTESIAN_POINT ( 'NONE',  ( 0.1049643490035303689, 0.3917322834645670104, -0.07808398950131241467 ) ) ;
#68015=CARTESIAN_POINT ( 'NONE',  ( 0.2867679344610365999, -0.2867679344610365444, -2.452755905511811108 ) ) ;
#68018=CARTESIAN_POINT ( 'NONE',  ( 0.3420746716998660508, -0.1974969037888703871, -2.782152230971128848 ) ) ;
#68023=CARTESIAN_POINT ( 'NONE',  ( -0.2925321140481930704, -0.2925321140481933480, -0.8464566929133857665 ) ) ;
#68026=CARTESIAN_POINT ( 'NONE',  ( 4.893765752498283924E-17, -0.3996062992125986035, -2.755905511811023612 ) ) ;
#68027=CARTESIAN_POINT ( 'NONE',  ( -0.1049643490035302024, -0.3917322834645671215, -0.6292650918635172008 ) ) ;
#68033=CARTESIAN_POINT ( 'NONE',  ( -0.3392501089628017219, -0.1958661417322836718, -0.2020997375328083545 ) ) ;
#68038=CARTESIAN_POINT ( 'NONE',  ( 0.4724409448818898682, 2.892866454678787531E-17, -1.692913385826771533 ) ) ;
#68048=CARTESIAN_POINT ( 'NONE',  ( -9.594673741351310580E-17, 0.3917322834645669549, -0.08003317765648111648 ) ) ;
#68050=CARTESIAN_POINT ( 'NONE',  ( 0.3392501089628018329, 0.1958661417322835607, -0.5308398950131234528 ) ) ;
#68055=CARTESIAN_POINT ( 'NONE',  ( 0.1049643490035303689, 0.3917322834645670104, -2.505249343832020248 ) ) ;
#68060=CARTESIAN_POINT ( 'NONE',  ( -1.157146581871515012E-16, 0.4724409448818898682, -0.8641732283464567121 ) ) ;
#68071=CARTESIAN_POINT ( 'NONE',  ( -0.2925321140481930149, -0.2925321140481933480, -2.183070866141731958 ) ) ;
#68080=CARTESIAN_POINT ( 'NONE',  ( -0.3996062992125985480, -7.340648628747423112E-17, -0.1161417322834645965 ) ) ;
#68081=CARTESIAN_POINT ( 'NONE',  ( -0.3996062992125987146, 0.1070741851644051862, -0.3477690288713909950 ) ) ;
#68082=CARTESIAN_POINT ( 'NONE',  ( -0.1049643490035302301, -0.3917322834645671770, -2.903562622868453680 ) ) ;
#68088=CARTESIAN_POINT ( 'NONE',  ( 0.3420746716998660508, -0.1974969037888704149, -0.8116797900262466836 ) ) ;
#68093=CARTESIAN_POINT ( 'NONE',  ( -0.4724409448818898682, -8.678599364036362592E-17, -1.141732283464566899 ) ) ;
#68094=CARTESIAN_POINT ( 'NONE',  ( 0.3996062992125986035, -0.1070741851644053111, -2.473753280839894764 ) ) ;
#68097=CARTESIAN_POINT ( 'NONE',  ( 0.1958661417322834775, 0.3392501089628018884, -0.9284970060705530770 ) ) ;
#68108=CARTESIAN_POINT ( 'NONE',  ( -0.3917322834645671215, 0.1049643490035301469, -1.127296587926509108 ) ) ;
#68111=CARTESIAN_POINT ( 'NONE',  ( -0.1058382717557497937, -0.3949938075777411628, -1.332020997375328086 ) ) ;
#68115=AXIS2_PLACEMENT_3D ( 'NONE', #55409, #81115, #76841 ) ;
#68118=CARTESIAN_POINT ( 'NONE',  ( -0.3996062992125986035, -0.1070741851644056997, 0.1115485564304461580 ) ) ;
#68130=CARTESIAN_POINT ( 'NONE',  ( 0.1070741851644054915, -0.3996062992125986035, -1.660104986876640210 ) ) ;
#68133=CARTESIAN_POINT ( 'NONE',  ( -0.3996062992125985480, -7.340648628747423112E-17, -1.218503937007874072 ) ) ;
#68137=CARTESIAN_POINT ( 'NONE',  ( -0.2362204724409451284, 0.4091458600556402425, -0.4855643044619422644 ) ) ;
#68139=CARTESIAN_POINT ( 'NONE',  ( 0.3917322834645670104, -0.1049643490035303411, -2.558398950131233196 ) ) ;
#68145=CARTESIAN_POINT ( 'NONE',  ( -0.4724409448818898682, -8.678599364036362592E-17, -2.320866141732283783 ) ) ;
#68148=CARTESIAN_POINT ( 'NONE',  ( 0.1974969037888704704, 0.3420746716998660508, -1.953412073490814027 ) ) ;
#68158=CARTESIAN_POINT ( 'NONE',  ( -0.1958661417322836440, 0.3392501089628016664, -2.612841576606612204 ) ) ;
#68173=CARTESIAN_POINT ( 'NONE',  ( 0.3996062992125985480, 2.446882876249141654E-17, -0.8248031496062991907 ) ) ;
#68175=CARTESIAN_POINT ( 'NONE',  ( 0.2867679344610365999, -0.2867679344610365444, -1.757874015748031260 ) ) ;
#68186=CARTESIAN_POINT ( 'NONE',  ( 0.1070741851644053388, 0.3996062992125986035, -1.487532808398950301 ) ) ;
#68189=ORIENTED_EDGE ( 'NONE', *, *, #67875, .F. ) ;
#68194=CARTESIAN_POINT ( 'NONE',  ( -0.2867679344610364334, -0.2867679344610367109, -1.403543307086614123 ) ) ;
#68199=CARTESIAN_POINT ( 'NONE',  ( 0.3996062992125985480, -0.1070741851644052972, -2.550524934383202158 ) ) ;
#68201=CARTESIAN_POINT ( 'NONE',  ( 0.1070741851644054915, -0.3996062992125986035, -0.7152230971128609172 ) ) ;
#68205=CARTESIAN_POINT ( 'NONE',  ( 0.3392501089628018884, -0.1958661417322834220, -2.774278215223096922 ) ) ;
#68216=CARTESIAN_POINT ( 'NONE',  ( 0.1049643490035304522, -0.3917322834645668994, -1.740138164533121756 ) ) ;
#68221=CARTESIAN_POINT ( 'NONE',  ( 0.3917322834645670104, 2.398668435337828261E-17, -2.879921259842519454 ) ) ;
#68224=CARTESIAN_POINT ( 'NONE',  ( 4.797336870675656522E-17, -0.3917322834645670659, -2.752643987697849237 ) ) ;
#68232=CARTESIAN_POINT ( 'NONE',  ( 0.1049643490035303967, 0.3917322834645670659, -1.250019315781839113 ) ) ;
#68234=CARTESIAN_POINT ( 'NONE',  ( -0.1049643490035302024, -0.3917322834645671215, -2.046587926509185973 ) ) ;
#68239=CARTESIAN_POINT ( 'NONE',  ( 0.1070741851644053527, 0.3996062992125986590, -0.6233595800524933672 ) ) ;
#68243=CARTESIAN_POINT ( 'NONE',  ( 0.3996062992125986590, -0.1070741851644053111, -2.158792650918635037 ) ) ;
#68249=CARTESIAN_POINT ( 'NONE',  ( 0.1265901696524990294, -0.4724409448818896462, -1.106955380577427706 ) ) ;
#68252=CARTESIAN_POINT ( 'NONE',  ( 0.1058382717557499880, 0.3949938075777409408, -0.5426509186351705649 ) ) ;
#68265=CARTESIAN_POINT ( 'NONE',  ( -0.1998031496062991630, -0.3460692066303959202, -1.559711286089239035 ) ) ;
#68267=CARTESIAN_POINT ( 'NONE',  ( 0.3392501089628018329, 0.1958661417322835607, -0.9107611548556429071 ) ) ;
#68282=DIRECTION ( 'NONE',  ( 1.000000000000000000, 0.000000000000000000, 0.000000000000000000 ) ) ;
#68289=CARTESIAN_POINT ( 'NONE',  ( -0.3917322834645671770, 0.1049643490035302024, -2.076790969325146730 ) ) ;
#68300=CARTESIAN_POINT ( 'NONE',  ( -0.3996062992125986035, -0.1070741851644056997, -2.880577427821522374 ) ) ;
#68301=CARTESIAN_POINT ( 'NONE',  ( 0.3949938075777409408, 0.1058382717557500574, -2.801837270341207553 ) ) ;
#68304=CARTESIAN_POINT ( 'NONE',  ( -0.1958661417322836718, 0.3392501089628017219, -1.580052493438320216 ) ) ;
#68306=CARTESIAN_POINT ( 'NONE',  ( -0.4724409448818895907, -0.1265901696524993070, -2.565616797900262647 ) ) ;
#68311=CARTESIAN_POINT ( 'NONE',  ( 4.797336870675655290E-17, -0.3917322834645669549, -0.4737339650580559280 ) ) ;
#68317=CARTESIAN_POINT ( 'NONE',  ( -0.3996062992125986035, -0.1070741851644056997, -2.880577427821522374 ) ) ;
#68318=CARTESIAN_POINT ( 'NONE',  ( -0.1958661417322836995, 0.3392501089628017219, -1.427184670112547682 ) ) ;
#68324=CARTESIAN_POINT ( 'NONE',  ( -0.3392501089628017219, -0.1958661417322836718, -0.7670603674540683592 ) ) ;
#68333=CARTESIAN_POINT ( 'NONE',  ( 0.2867679344610365999, 0.2867679344610365999, -2.177165354330708347 ) ) ;
#68339=CYLINDRICAL_SURFACE ( 'NONE', #73365, 0.4724409448818898682 ) ;
#68340=CARTESIAN_POINT ( 'NONE',  ( 0.1049643490035304938, -0.3917322834645669549, -0.9573490813648293241 ) ) ;
#68343=CARTESIAN_POINT ( 'NONE',  ( 4.893765752498283308E-17, -0.3996062992125985480, -2.360236220472441193 ) ) ;
#68363=CARTESIAN_POINT ( 'NONE',  ( 0.1958661417322836162, -0.3392501089628018329, -1.746699844323147843 ) ) ;
#68372=CARTESIAN_POINT ( 'NONE',  ( -0.3917322834645671770, 0.1049643490035302024, -0.3445075047582172312 ) ) ;
#68375=CARTESIAN_POINT ( 'NONE',  ( -0.4724409448818895907, -0.1265901696524993070, -1.854986876640420057 ) ) ;
#68386=CARTESIAN_POINT ( 'NONE',  ( 0.4724409448818898682, 0.000000000000000000, -2.755905511811024056 ) ) ;
#68395=CARTESIAN_POINT ( 'NONE',  ( 0.3460692066303959202, -0.1998031496062991630, -2.386482939632545985 ) ) ;
#68400=CARTESIAN_POINT ( 'NONE',  ( 0.2925321140481932369, 0.2925321140481932369, -1.712598425196850460 ) ) ;
#68401=CARTESIAN_POINT ( 'NONE',  ( 0.1974969037888704704, 0.3420746716998660508, -1.089238845144357093 ) ) ;
#68402=CARTESIAN_POINT ( 'NONE',  ( 4.893765752498283924E-17, -0.3996062992125986035, -2.598425196850393970 ) ) ;
#68403=CARTESIAN_POINT ( 'NONE',  ( 0.1049643490035303689, 0.3917322834645670104, -0.4580052493438320216 ) ) ;
#68407=CARTESIAN_POINT ( 'NONE',  ( 0.1058382717557500852, -0.3949938075777408852, -2.366797900262467280 ) ) ;
#68410=CARTESIAN_POINT ( 'NONE',  ( -0.4724409448818899238, 0.1265901696524986686, -2.552493438320210029 ) ) ;
#68411=CARTESIAN_POINT ( 'NONE',  ( 0.2925321140481932369, -0.2925321140481932369, -1.830708661417322913 ) ) ;
#68417=CARTESIAN_POINT ( 'NONE',  ( -0.1049643490035306742, 0.3917322834645668994, -2.763760211777216202 ) ) ;
#68424=CARTESIAN_POINT ( 'NONE',  ( 0.3917322834645669549, 0.1049643490035304660, -0.05183727034120744204 ) ) ;
#68426=CARTESIAN_POINT ( 'NONE',  ( 0.3917322834645670104, 2.398668435337828261E-17, -2.472440944881889813 ) ) ;
#68429=CARTESIAN_POINT ( 'NONE',  ( 0.3949938075777409408, 0.1058382717557500574, -2.801837270341207553 ) ) ;
#68433=CARTESIAN_POINT ( 'NONE',  ( 0.1998031496062992740, 0.3460692066303959757, -0.9317585301837270073 ) ) ;
#68438=CARTESIAN_POINT ( 'NONE',  ( -0.1049643490035307020, 0.3917322834645669549, -0.5636482939632546652 ) ) ;
#68444=CARTESIAN_POINT ( 'NONE',  ( -0.1958661417322836718, 0.3392501089628017219, -0.3202099737532808077 ) ) ;
#68448=CARTESIAN_POINT ( 'NONE',  ( -1.157146581871515012E-16, 0.4724409448818898682, -1.574803149606299302 ) ) ;
#68451=CARTESIAN_POINT ( 'NONE',  ( 0.1049643490035304799, -0.3917322834645669549, -2.689632545931758489 ) ) ;
#68456=VECTOR ( 'NONE', #44881, 39.37007874015748143 ) ;
#68459=CARTESIAN_POINT ( 'NONE',  ( -0.2867679344610366554, 0.2867679344610365444, -0.2571985319871897824 ) ) ;
#68461=CARTESIAN_POINT ( 'NONE',  ( 4.797336870675656522E-17, -0.3917322834645670104, -0.4783464566929135353 ) ) ;
#68466=CARTESIAN_POINT ( 'NONE',  ( 0.3917322834645669549, 0.1049643490035304660, -2.479002624671915900 ) ) ;
#68469=CARTESIAN_POINT ( 'NONE',  ( 0.2362204724409451007, -0.4091458600556402980, -0.7985564304461942875 ) ) ;
#68477=CARTESIAN_POINT ( 'NONE',  ( -0.3458507752293909498, 0.3458507752293908388, -0.3346456692913385433 ) ) ;
#68480=CARTESIAN_POINT ( 'NONE',  ( 0.2925321140481932369, -0.2925321140481931814, -1.907480314960629197 ) ) ;
#68488=CARTESIAN_POINT ( 'NONE',  ( -0.1070741851644057135, 0.3996062992125984925, -0.3982939632545931530 ) ) ;
#68489=CARTESIAN_POINT ( 'NONE',  ( -0.2925321140481930704, -0.2925321140481933480, -0.3740157480314960092 ) ) ;
#68490=CARTESIAN_POINT ( 'NONE',  ( 4.837279021331060870E-17, -0.3949938075777409963, 0.07874015748031490403 ) ) ;
#68495=CARTESIAN_POINT ( 'NONE',  ( -0.1974969037888704149, -0.3420746716998661063, -1.087270341207349000 ) ) ;
#68500=CARTESIAN_POINT ( 'NONE',  ( -1.157146581871515012E-16, 0.4724409448818898682, -1.259842519685039353 ) ) ;
#68501=CARTESIAN_POINT ( 'NONE',  ( -0.1070741851644057135, 0.3996062992125985480, -2.211286089238845065 ) ) ;
#68504=CARTESIAN_POINT ( 'NONE',  ( -0.1049643490035307158, 0.3917322834645670104, -0.6332214155193720551 ) ) ;
#68515=CARTESIAN_POINT ( 'NONE',  ( 0.1049643490035303689, 0.3917322834645670104, -0.9304461942257216123 ) ) ;
#68518=CARTESIAN_POINT ( 'NONE',  ( -0.3420746716998661618, 0.1974969037888702206, -1.286089238845144367 ) ) ;
#68528=CARTESIAN_POINT ( 'NONE',  ( 0.4091458600556403535, 0.2362204724409449896, -0.3654855643044619407 ) ) ;
#68529=CARTESIAN_POINT ( 'NONE',  ( 4.797336870675656522E-17, -0.3917322834645670104, 0.1515748031496061965 ) ) ;
#68535=CARTESIAN_POINT ( 'NONE',  ( 0.3996062992125986035, 2.446882876249141962E-17, -2.165354330708661568 ) ) ;
#68538=CARTESIAN_POINT ( 'NONE',  ( -0.3996062992125986590, 0.1070741851644051723, -1.684383202099737353 ) ) ;
#68539=CARTESIAN_POINT ( 'NONE',  ( -0.02899565511876225909, 0.3969271875946638328, -2.755905511811026276 ) ) ;
#68542=CARTESIAN_POINT ( 'NONE',  ( -0.4091458600556405756, 0.2362204724409446288, -0.4986876640419947715 ) ) ;
#68544=CARTESIAN_POINT ( 'NONE',  ( 0.1049643490035304938, -0.3917322834645669549, -2.532152230971127960 ) ) ;
#68550=CARTESIAN_POINT ( 'NONE',  ( 0.4724409448818896462, 0.1265901696524990294, -2.248687664041994605 ) ) ;
#68552=CARTESIAN_POINT ( 'NONE',  ( -0.2891555358219911054, 0.2891555358219909388, -2.143700787401574548 ) ) ;
#68558=CARTESIAN_POINT ( 'NONE',  ( 0.4091458600556404646, -0.2362204724409448231, -2.229002624671915900 ) ) ;
#68574=CARTESIAN_POINT ( 'NONE',  ( 0.1998031496062992463, 0.3460692066303959202, -0.8510498687664042050 ) ) ;
#68576=CARTESIAN_POINT ( 'NONE',  ( -0.3392501089628019995, 0.1958661417322832277, -2.315616797900262647 ) ) ;
#68585=CARTESIAN_POINT ( 'NONE',  ( 0.1998031496062994128, -0.3460692066303957537, -1.585958005249344049 ) ) ;
#68587=CARTESIAN_POINT ( 'NONE',  ( -0.4724409448818898682, -8.678599364036362592E-17, -2.244094488188976388 ) ) ;
#68588=ORIENTED_EDGE ( 'NONE', *, *, #34764, .T. ) ;
#68592=CARTESIAN_POINT ( 'NONE',  ( -0.2867679344610364334, -0.2867679344610367109, -1.561023622047243986 ) ) ;
#68598=CARTESIAN_POINT ( 'NONE',  ( -0.3460692066303957537, -0.1998031496062994405, -2.333989501312335957 ) ) ;
#68600=CARTESIAN_POINT ( 'NONE',  ( -0.3996062992125987146, 0.1070741851644051862, -0.9776902887139107268 ) ) ;
#68603=CARTESIAN_POINT ( 'NONE',  ( 0.3392501089628018329, 0.1958661417322835607, -2.485564304461941987 ) ) ;
#68613=CARTESIAN_POINT ( 'NONE',  ( 0.2867679344610365999, 0.2867679344610365999, -1.950111917813961426 ) ) ;
#68616=CARTESIAN_POINT ( 'NONE',  ( 0.3917322834645670104, -0.1049643490035303411, 0.05380577427821527092 ) ) ;
#68619=CARTESIAN_POINT ( 'NONE',  ( 0.3420746716998659953, 0.1974969037888705536, -0.2887139107611549349 ) ) ;
#68627=CARTESIAN_POINT ( 'NONE',  ( -0.1049643490035307158, 0.3917322834645670104, -1.420622990322521373 ) ) ;
#68629=CARTESIAN_POINT ( 'NONE',  ( -0.3917322834645671215, 0.1049643490035301469, -2.637139107611548461 ) ) ;
#68634=AXIS2_PLACEMENT_3D ( 'NONE', #3112, #58364, #14199 ) ;
#68635=CARTESIAN_POINT ( 'NONE',  ( 0.3996062992125986035, 0.1070741851644054776, -0.7545931758530182165 ) ) ;
#68637=CARTESIAN_POINT ( 'NONE',  ( -0.1998031496062991630, -0.3460692066303959202, -0.4573490813648293796 ) ) ;
#68639=CARTESIAN_POINT ( 'NONE',  ( 0.3996062992125986035, 0.1070741851644054776, -2.329396325459317296 ) ) ;
#68643=CARTESIAN_POINT ( 'NONE',  ( 0.2362204724409451007, -0.4091458600556402980, -1.270997375328083878 ) ) ;
#68647=CARTESIAN_POINT ( 'NONE',  ( 0.1058382717557500852, -0.3949938075777408852, -0.4770341207349081403 ) ) ;
#68662=CARTESIAN_POINT ( 'NONE',  ( -0.3460692066303957537, -0.1998031496062994405, -1.704068241469816281 ) ) ;
#68664=CARTESIAN_POINT ( 'NONE',  ( 0.3917322834645670104, -0.1049643490035303411, -1.363517060367453793 ) ) ;
#68666=CARTESIAN_POINT ( 'NONE',  ( -0.1324727617108180378, -0.3692639355350240127, -1.489137855930807863E-17 ) ) ;
#68678=CARTESIAN_POINT ( 'NONE',  ( -0.4724409448818896462, -0.1265901696524993070, -0.2801837270341207553 ) ) ;
#68693=CARTESIAN_POINT ( 'NONE',  ( 0.1049643490035304799, -0.3917322834645669549, -1.967191601049868899 ) ) ;
#68697=CARTESIAN_POINT ( 'NONE',  ( -0.4724409448818899238, 0.1265901696524986686, -0.3477690288713909950 ) ) ;
#68698=CARTESIAN_POINT ( 'NONE',  ( -0.3949938075777409408, -0.1058382717557502933, -2.565616797900262647 ) ) ;
#68701=CARTESIAN_POINT ( 'NONE',  ( -0.3392501089628019995, 0.1958661417322832277, -1.435695538057742970 ) ) ;
#68703=CARTESIAN_POINT ( 'NONE',  ( 0.4724409448818897572, -0.1265901696524988906, -2.631233595800525293 ) ) ;
#68704=CARTESIAN_POINT ( 'NONE',  ( 0.000000000000000000, 0.000000000000000000, -1.929133858267716661 ) ) ;
#68710=CARTESIAN_POINT ( 'NONE',  ( 0.1958661417322836162, -0.3392501089628018329, -0.6443376395987383543 ) ) ;
#68717=CARTESIAN_POINT ( 'NONE',  ( -0.3917322834645670659, -7.196005306013484475E-17, -1.925872334154542509 ) ) ;
#68721=EDGE_CURVE ( 'NONE', #32199, #58583, #13072, .T. ) ;
#68724=CARTESIAN_POINT ( 'NONE',  ( 0.1958661417322834775, 0.3392501089628018884, -1.016404199475065662 ) ) ;
#68735=CARTESIAN_POINT ( 'NONE',  ( -0.2867679344610364334, -0.2867679344610367109, -2.728346456692912536 ) ) ;
#68742=CARTESIAN_POINT ( 'NONE',  ( -0.3392501089628017219, -0.1958661417322836718, -0.6095800524934383846 ) ) ;
#68743=CARTESIAN_POINT ( 'NONE',  ( -0.4724409448818895907, -0.1265901696524993070, 0.1922572178477690297 ) ) ;
#68745=CARTESIAN_POINT ( 'NONE',  ( 0.1998031496062994128, -0.3460692066303957537, -2.530839895013123453 ) ) ;
#68755=CARTESIAN_POINT ( 'NONE',  ( 0.1998031496062992463, 0.3460692066303959202, -0.5360892388451443669 ) ) ;
#68757=CARTESIAN_POINT ( 'NONE',  ( 0.3392501089628018329, 0.1958661417322835607, -0.1233595800524933950 ) ) ;
#68764=CARTESIAN_POINT ( 'NONE',  ( 0.3917322834645669549, 2.398668435337827645E-17, -1.457985933561992686 ) ) ;
#68773=CARTESIAN_POINT ( 'NONE',  ( 0.2867679344610366554, 0.2867679344610366554, -0.6069746963592669298 ) ) ;
#68777=CARTESIAN_POINT ( 'NONE',  ( 0.3458507752293908943, -0.3458507752293908943, -2.222440944881889813 ) ) ;
#68796=CARTESIAN_POINT ( 'NONE',  ( -0.1998031496062994683, 0.3460692066303958092, -0.01312335958005251234 ) ) ;
#68797=CARTESIAN_POINT ( 'NONE',  ( 0.1070741851644054776, -0.3996062992125984925, -2.524278215223096478 ) ) ;
#68802=CARTESIAN_POINT ( 'NONE',  ( -0.1998031496062991907, -0.3460692066303959757, -1.955380577427821454 ) ) ;
#68803=CARTESIAN_POINT ( 'NONE',  ( 0.1974969037888706369, -0.3420746716998659953, -1.509186351706036655 ) ) ;
#68804=CARTESIAN_POINT ( 'NONE',  ( -0.3460692066303958092, -0.1998031496062994683, -2.729658792650918375 ) ) ;
#68805=CARTESIAN_POINT ( 'NONE',  ( -0.2362204724409451284, 0.4091458600556402425, -2.532808398950130879 ) ) ;
#68806=CARTESIAN_POINT ( 'NONE',  ( 0.1049643490035303689, 0.3917322834645670104, -0.6154855643044617741 ) ) ;
#68811=CARTESIAN_POINT ( 'NONE',  ( -0.1058382717557503072, 0.3949938075777408852, -2.130577427821521930 ) ) ;
#68815=CARTESIAN_POINT ( 'NONE',  ( -0.4724409448818898682, -8.678599364036362592E-17, -2.559055118110236560 ) ) ;
#68816=CARTESIAN_POINT ( 'NONE',  ( -0.2925321140481932924, 0.2925321140481931814, -2.224409448818897239 ) ) ;
#68817=CARTESIAN_POINT ( 'NONE',  ( -0.03757601356356682354, 0.4709442531824372113, -2.755905511811023612 ) ) ;
#68824=CARTESIAN_POINT ( 'NONE',  ( -0.3392501089628019439, 0.1958661417322832554, -2.783445251147295352 ) ) ;
#68830=CARTESIAN_POINT ( 'NONE',  ( -0.3392501089628017219, -0.1958661417322836718, -0.2946194225721785465 ) ) ;
#68831=CARTESIAN_POINT ( 'NONE',  ( 0.2867679344610365999, 0.2867679344610365999, -1.704724409448818978 ) ) ;
#68832=( BOUNDED_CURVE ( )  B_SPLINE_CURVE ( 2, ( #49601, #76117, #17639, #56328, #75295, #44101, #55080, #18458, #69794, #12140, #68558, #10498, #75708 ),
 .UNSPECIFIED., .F., .F. ) 
 B_SPLINE_CURVE_WITH_KNOTS ( ( 3, 2, 2, 2, 2, 2, 3 ),
 ( 0.7625000000000000666, 0.7666666666666668295, 0.7708333333333334814, 0.7750000000000001332, 0.7791666666666667851, 0.7833333333333334370, 0.7875000000000000888 ),
 .UNSPECIFIED. ) 
 CURVE ( )  GEOMETRIC_REPRESENTATION_ITEM ( )  RATIONAL_B_SPLINE_CURVE ( ( 0.9999999999999991118, 0.9659258262890692004, 1.000000000000000000, 0.9659258262890683122, 1.000000000000000000, 0.9659258262890683122, 1.000000000000000000, 0.9659258262890683122, 1.000000000000000000, 0.9659258262890683122, 1.000000000000000000, 0.9659258262890674240, 1.000000000000000888 ) ) 
 REPRESENTATION_ITEM ( '' )  );
#68833=CARTESIAN_POINT ( 'NONE',  ( 0.1049643490035304938, -0.3917322834645669549, -2.124671916010498762 ) ) ;
#68836=CARTESIAN_POINT ( 'NONE',  ( 0.2891555358219910499, 0.2891555358219910499, -2.657480314960630530 ) ) ;
#68840=CARTESIAN_POINT ( 'NONE',  ( 0.3460692066303959202, 0.1998031496062993295, -1.233595800524934338 ) ) ;
#68845=CARTESIAN_POINT ( 'NONE',  ( -0.1958661417322836718, 0.3392501089628017219, -0.4127296587926510552 ) ) ;
#68850=CARTESIAN_POINT ( 'NONE',  ( 0.3392501089628018329, 0.1958661417322835607, -0.1233595800524933950 ) ) ;
#68851=ORIENTED_EDGE ( 'NONE', *, *, #55159, .T. ) ;
#68854=CARTESIAN_POINT ( 'NONE',  ( -0.4724409448818898682, -8.678599364036362592E-17, -1.771653543307086576 ) ) ;
#68856=CARTESIAN_POINT ( 'NONE',  ( -0.3458507752293909498, 0.3458507752293908388, -0.9645669291338581086 ) ) ;
#68863=CARTESIAN_POINT ( 'NONE',  ( -0.3392501089628019439, 0.1958661417322832554, -0.4212405267378459550 ) ) ;
#68865=CARTESIAN_POINT ( 'NONE',  ( 0.2867679344610366554, 0.2867679344610366554, -1.009842519685039353 ) ) ;
#68871=CARTESIAN_POINT ( 'NONE',  ( 0.1958661417322836440, -0.3392501089628017219, -2.131233595800524849 ) ) ;
#68874=CARTESIAN_POINT ( 'NONE',  ( -0.1265901696524986964, -0.4724409448818899238, -0.9363517060367454459 ) ) ;
#68882=CARTESIAN_POINT ( 'NONE',  ( -0.4724409448818899238, 0.1265901696524986964, -0.3477690288713910505 ) ) ;
#68885=CARTESIAN_POINT ( 'NONE',  ( 0.2925321140481932369, 0.2925321140481932369, -1.946850393700787274 ) ) ;
#68893=CARTESIAN_POINT ( 'NONE',  ( -0.2925321140481930149, -0.2925321140481933480, -0.2933070866141732624 ) ) ;
#68894=CARTESIAN_POINT ( 'NONE',  ( 0.1998031496062994405, -0.3460692066303958092, -0.5643044619422572516 ) ) ;
#68895=CARTESIAN_POINT ( 'NONE',  ( -0.1974969037888703871, -0.3420746716998661063, -0.3805774278215224293 ) ) ;
#68900=CARTESIAN_POINT ( 'NONE',  ( -0.1058382717557503072, 0.3949938075777408852, -0.8707349081364829102 ) ) ;
#68906=CARTESIAN_POINT ( 'NONE',  ( 0.4724409448818896462, 0.1265901696524990294, -1.069553805774278166 ) ) ;
#68907=CARTESIAN_POINT ( 'NONE',  ( 0.1998031496062994405, -0.3460692066303958092, -2.139107611548556331 ) ) ;
#68910=CARTESIAN_POINT ( 'NONE',  ( 0.3917322834645670659, 2.398668435337828261E-17, -0.9022502869104481737 ) ) ;
#68913=EDGE_CURVE ( 'NONE', #66690, #56483, #43353, .T. ) ;
#68923=CARTESIAN_POINT ( 'NONE',  ( -0.1958661417322834220, -0.3392501089628018884, -0.8451443569553805935 ) ) ;
#68926=CARTESIAN_POINT ( 'NONE',  ( 0.1974969037888704704, 0.3420746716998660508, -1.561679790026246684 ) ) ;
#68931=CARTESIAN_POINT ( 'NONE',  ( 0.2925321140481932369, -0.2925321140481932369, 0.05905511811023619884 ) ) ;
#68938=CARTESIAN_POINT ( 'NONE',  ( -0.1049643490035307020, 0.3917322834645669549, -0.09120734908136493568 ) ) ;
#68944=CARTESIAN_POINT ( 'NONE',  ( -0.3996062992125987146, 0.1070741851644051862, -1.922572178477689908 ) ) ;
#68947=CARTESIAN_POINT ( 'NONE',  ( -0.1070741851644051862, -0.3996062992125986590, -1.723753280839894986 ) ) ;
#68948=CARTESIAN_POINT ( 'NONE',  ( -0.03056273350765576630, 0.3973686378485519755, -2.755905511811022723 ) ) ;
#68951=CARTESIAN_POINT ( 'NONE',  ( -0.2362204724409447953, -0.4091458600556404646, -0.2230971128608923715 ) ) ;
#68953=CARTESIAN_POINT ( 'NONE',  ( 4.797336870675656522E-17, -0.3917322834645670104, 0.08661417322834651100 ) ) ;
#68959=CARTESIAN_POINT ( 'NONE',  ( -0.4724409448818898682, -8.678599364036362592E-17, -2.478346456692913868 ) ) ;
#68961=CARTESIAN_POINT ( 'NONE',  ( 0.2891555358219910499, 0.2891555358219910499, -2.261811023622047667 ) ) ;
#68973=CARTESIAN_POINT ( 'NONE',  ( 0.3458507752293908943, 0.3458507752293908943, -1.001968503937007871 ) ) ;
#68984=CARTESIAN_POINT ( 'NONE',  ( -0.2925321140481930149, -0.2925321140481933480, -0.9232283464566929387 ) ) ;
#68985=CARTESIAN_POINT ( 'NONE',  ( 0.1958661417322834775, 0.3392501089628018884, -2.276246719160105236 ) ) ;
#69001=CARTESIAN_POINT ( 'NONE',  ( -0.3917322834645670104, -7.196005306013484475E-17, -1.383858267716535417 ) ) ;
#69006=CARTESIAN_POINT ( 'NONE',  ( 0.3996062992125985480, 2.446882876249141654E-17, -2.399606299212598604 ) ) ;
#69008=CARTESIAN_POINT ( 'NONE',  ( 0.1070741851644054915, -0.3996062992125986035, -1.030183727034120533 ) ) ;
#69011=CARTESIAN_POINT ( 'NONE',  ( 0.2867679344610365999, 0.2867679344610365999, -2.649606299212598604 ) ) ;
#69017=CIRCLE ( 'NONE', #73052, 0.2952755905511810774 ) ;
#69024=CARTESIAN_POINT ( 'NONE',  ( -9.594673741351313045E-17, 0.3917322834645670104, -2.761811023622046779 ) ) ;
#69027=CARTESIAN_POINT ( 'NONE',  ( 0.2891555358219910499, -0.2891555358219909944, -0.2559055118110237226 ) ) ;
#69031=CARTESIAN_POINT ( 'NONE',  ( 0.4724409448818895907, 0.1265901696524994180, -0.1246719160104987345 ) ) ;
#69036=CARTESIAN_POINT ( 'NONE',  ( -0.3917322834645670104, -0.1049643490035307020, -1.302512754102049142 ) ) ;
#69038=CARTESIAN_POINT ( 'NONE',  ( 0.2867679344610365999, -0.2867679344610365444, -2.860236220472440749 ) ) ;
#69044=CARTESIAN_POINT ( 'NONE',  ( 0.1070741851644053527, 0.3996062992125986590, -0.7808398950131233418 ) ) ;
#69046=CARTESIAN_POINT ( 'NONE',  ( -0.1998031496062991630, -0.3460692066303959202, -0.1423884514435695414 ) ) ;
#69048=CARTESIAN_POINT ( 'NONE',  ( -0.3996062992125986035, -7.340648628747425578E-17, -2.086614173228346303 ) ) ;
#69049=CARTESIAN_POINT ( 'NONE',  ( 0.2867679344610365999, -0.2867679344610365444, -1.600393700787401619 ) ) ;
#69053=CARTESIAN_POINT ( 'NONE',  ( 0.4724409448818898682, 2.892866454678787531E-17, -0.9822834645669291653 ) ) ;
#69056=CARTESIAN_POINT ( 'NONE',  ( 4.837279021331061486E-17, -0.3949938075777409963, -0.9429133858267715329 ) ) ;
#69069=CARTESIAN_POINT ( 'NONE',  ( -0.1070741851644051862, -0.3996062992125986590, -1.723753280839895208 ) ) ;
#69072=CARTESIAN_POINT ( 'NONE',  ( 0.1049643490035304938, -0.3917322834645669549, -1.494750656167978642 ) ) ;
#69087=CARTESIAN_POINT ( 'NONE',  ( -9.594673741351313045E-17, 0.3917322834645670104, -1.187007874015748143 ) ) ;
#69102=LINE ( 'NONE', #17770, #45960 ) ;
#69103=CARTESIAN_POINT ( 'NONE',  ( -9.787531504996567848E-17, 0.3996062992125986035, -1.102362204724409489 ) ) ;
#69108=CARTESIAN_POINT ( 'NONE',  ( -0.4724409448818895907, -0.1265901696524993070, -0.3608923884514435576 ) ) ;
#69109=CARTESIAN_POINT ( 'NONE',  ( 0.1058382717557500713, -0.3949938075777409408, -2.919947506561680228 ) ) ;
#69112=CARTESIAN_POINT ( 'NONE',  ( -0.1049643490035302024, -0.3917322834645671215, -1.481627296587926690 ) ) ;
#69114=CARTESIAN_POINT ( 'NONE',  ( 0.2362204724409451007, -0.4091458600556402980, -2.454068241469816058 ) ) ;
#69120=CARTESIAN_POINT ( 'NONE',  ( -0.1958661417322834497, -0.3392501089628018884, -0.6180909204386334510 ) ) ;
#69128=CARTESIAN_POINT ( 'NONE',  ( -0.3917322834645670104, -0.1049643490035307020, -2.089914328905198904 ) ) ;
#69134=CARTESIAN_POINT ( 'NONE',  ( 0.3917322834645669549, 0.1049643490035304660, -1.311679790026246906 ) ) ;
#69144=CARTESIAN_POINT ( 'NONE',  ( 0.3458507752293908943, -0.3458507752293908943, -0.9625984251968502381 ) ) ;
#69146=CARTESIAN_POINT ( 'NONE',  ( -0.2867679344610365999, 0.2867679344610364889, -2.688976377952755570 ) ) ;
#69153=CARTESIAN_POINT ( 'NONE',  ( 0.1958661417322834775, 0.3392501089628018884, -1.173884514435695525 ) ) ;
#69154=CARTESIAN_POINT ( 'NONE',  ( 0.1265901696524990294, -0.4724409448818896462, 0.1528871391076115360 ) ) ;
#69156=CARTESIAN_POINT ( 'NONE',  ( 0.1070741851644053388, 0.3996062992125986035, -2.747375328083988766 ) ) ;
#69165=CARTESIAN_POINT ( 'NONE',  ( -0.1998031496062994405, 0.3460692066303957537, -0.5623359580052492701 ) ) ;
#69167=CARTESIAN_POINT ( 'NONE',  ( -0.3392501089628019995, 0.1958661417322832277, -0.1758530183727033402 ) ) ;
#69182=CARTESIAN_POINT ( 'NONE',  ( 0.3392501089628018329, 0.1958661417322835607, -0.9153736464905005699 ) ) ;
#69187=CARTESIAN_POINT ( 'NONE',  ( 0.1265901696524990294, -0.4724409448818896462, -1.894356955380577023 ) ) ;
#69192=( BOUNDED_CURVE ( )  B_SPLINE_CURVE ( 2, ( #5946, #37110, #24477, #56459, #82562, #62794, #24881, #68693, #56046, #50549, #30379, #37932, #76253, #50143, #75840, #31615, #50959, #62368, #81754, #63609, #18182, #82974, #12274, #49323, #75024, #76656, #70333, #25293, #36693, #75433, #57276, #44636, #5536, #17370, #12689, #55629, #38348, #4706, #81338, #17773, #23652, #24065, #44230, #69920, #43814, #11868, #37521, #29964, #43000, #11035, #43405, #31201, #77919, #19833, #58965, #14786, #72436, #46744, #65719, #45058, #6776, #26131, #13110, #1322, #1732, #46325, #39605, #71596, #78760, #78341, #52216, #59373, #33712, #14374, #32448, #72018, #65294, #45899, #13948, #64440, #40442, #58110, #40031, #33304, #39177, #64861, #8050, #27388, #38763, #476, #53049, #7199, #51793, #26971, #77497, #13521, #70759, #52636, #21085, #20672, #6363, #32035, #57694, #7633, #77073, #56, #25710, #51370, #45482, #19407, #71179, #32871, #58539, #905, #26562, #20250, #35783, #59789, #54298, #2143, #80012, #27811, #53471, #22327, #79594, #35372, #74512, #48813, #23144 ),
 .UNSPECIFIED., .F., .F. ) 
 B_SPLINE_CURVE_WITH_KNOTS ( ( 3, 2, 2, 2, 2, 2, 2, 2, 2, 2, 2, 2, 2, 2, 2, 2, 2, 2, 2, 2, 2, 2, 2, 2, 2, 2, 2, 2, 2, 2, 2, 2, 2, 2, 2, 2, 2, 2, 2, 2, 2, 2, 2, 2, 2, 2, 2, 2, 2, 2, 2, 2, 2, 2, 2, 2, 2, 2, 2, 2, 2, 2, 2, 2, 3 ),
 ( 0.6649931759405284248, 0.6666666666666666297, 0.6708333333333332815, 0.6750000000000000444, 0.6791666666666666963, 0.6833333333333333481, 0.6875000000000000000, 0.6916666666666666519, 0.6958333333333333037, 0.6999999999999999556, 0.7041666666666667185, 0.7083333333333333703, 0.7125000000000000222, 0.7166666666666666741, 0.7208333333333333259, 0.7249999999999999778, 0.7291666666666666297, 0.7333333333333332815, 0.7375000000000000444, 0.7416666666666666963, 0.7458333333333333481, 0.7500000000000000000, 0.7541666666666666519, 0.7583333333333333037, 0.7624999999999999556, 0.7666666666666667185, 0.7708333333333333703, 0.7750000000000000222, 0.7791666666666666741, 0.7833333333333333259, 0.7874999999999999778, 0.7916666666666666297, 0.7958333333333332815, 0.8000000000000000444, 0.8041666666666666963, 0.8083333333333333481, 0.8125000000000000000, 0.8166666666666666519, 0.8208333333333333037, 0.8249999999999999556, 0.8291666666666667185, 0.8333333333333333703, 0.8375000000000000222, 0.8416666666666666741, 0.8458333333333333259, 0.8499999999999999778, 0.8541666666666666297, 0.8583333333333332815, 0.8625000000000000444, 0.8666666666666666963, 0.8708333333333333481, 0.8750000000000000000, 0.8791666666666666519, 0.8833333333333333037, 0.8874999999999999556, 0.8916666666666667185, 0.8958333333333333703, 0.9000000000000000222, 0.9041666666666666741, 0.9083333333333333259, 0.9124999999999999778, 0.9166666666666666297, 0.9208333333333332815, 0.9250000000000000444, 0.9274931759404547726 ),
 .UNSPECIFIED. ) 
 CURVE ( )  GEOMETRIC_REPRESENTATION_ITEM ( )  RATIONAL_B_SPLINE_CURVE ( ( 0.9836222570913433216, 0.9863145247105440383, 1.000000000000000000, 0.9659258262890683122, 1.000000000000000000, 0.9659258262890683122, 1.000000000000000000, 0.9659258262890683122, 1.000000000000000000, 0.9659258262890683122, 1.000000000000000000, 0.9659258262890683122, 1.000000000000000000, 0.9659258262890683122, 1.000000000000000000, 0.9659258262890683122, 1.000000000000000000, 0.9659258262890683122, 1.000000000000000000, 0.9659258262890683122, 1.000000000000000000, 0.9659258262890683122, 1.000000000000000000, 0.9659258262890683122, 1.000000000000000000, 0.9659258262890683122, 1.000000000000000000, 0.9659258262890683122, 1.000000000000000000, 0.9659258262890683122, 1.000000000000000000, 0.9659258262890683122, 1.000000000000000000, 0.9659258262890683122, 1.000000000000000000, 0.9659258262890683122, 1.000000000000000000, 0.9659258262890683122, 1.000000000000000000, 0.9659258262890683122, 1.000000000000000000, 0.9659258262890683122, 1.000000000000000000, 0.9659258262890683122, 1.000000000000000000, 0.9659258262890683122, 1.000000000000000000, 0.9659258262890683122, 1.000000000000000000, 0.9659258262890683122, 1.000000000000000000, 0.9659258262890683122, 1.000000000000000000, 0.9659258262890683122, 1.000000000000000000, 0.9659258262890683122, 1.000000000000000000, 0.9659258262890683122, 1.000000000000000000, 0.9659258262890683122, 1.000000000000000000, 0.9659258262890683122, 1.000000000000000000, 0.9659258262890683122, 1.000000000000000000, 0.9659258262890683122, 1.000000000000000000, 0.9659258262890683122, 1.000000000000000000, 0.9659258262890683122, 1.000000000000000000, 0.9659258262890683122, 1.000000000000000000, 0.9659258262890683122, 1.000000000000000000, 0.9659258262890683122, 1.000000000000000000, 0.9659258262890683122, 1.000000000000000000, 0.9659258262890683122, 1.000000000000000000, 0.9659258262890683122, 1.000000000000000000, 0.9659258262890683122, 1.000000000000000000, 0.9659258262890683122, 1.000000000000000000, 0.9659258262890683122, 1.000000000000000000, 0.9659258262890683122, 1.000000000000000000, 0.9659258262890683122, 1.000000000000000000, 0.9659258262890683122, 1.000000000000000000, 0.9659258262890683122, 1.000000000000000000, 0.9659258262890683122, 1.000000000000000000, 0.9659258262890683122, 1.000000000000000000, 0.9659258262890683122, 1.000000000000000000, 0.9659258262890683122, 1.000000000000000000, 0.9659258262890683122, 1.000000000000000000, 0.9659258262890683122, 1.000000000000000000, 0.9659258262890683122, 1.000000000000000000, 0.9659258262890683122, 1.000000000000000000, 0.9659258262890683122, 1.000000000000000000, 0.9659258262890683122, 1.000000000000000000, 0.9659258262890683122, 1.000000000000000000, 0.9659258262890683122, 1.000000000000000000, 0.9659258262890683122, 1.000000000000000000, 0.9659258262890683122, 1.000000000000000000, 0.9659258262890683122, 1.000000000000000000, 0.9796113015791271250, 0.9836222570911059560 ) ) 
 REPRESENTATION_ITEM ( '' )  );
#69210=CARTESIAN_POINT ( 'NONE',  ( -0.1998031496062994405, 0.3460692066303957537, -2.767060367454068359 ) ) ;
#69215=CARTESIAN_POINT ( 'NONE',  ( 0.3460692066303959202, 0.1998031496062993295, -2.178477690288713742 ) ) ;
#69217=CARTESIAN_POINT ( 'NONE',  ( -0.3949938075777409408, -0.1058382717557502933, -1.620734908136483243 ) ) ;
#69218=CARTESIAN_POINT ( 'NONE',  ( -0.1998031496062994683, 0.3460692066303958092, -2.690288713910760965 ) ) ;
#69220=CARTESIAN_POINT ( 'NONE',  ( -0.1958661417322836718, 0.3392501089628017219, -0.6351706036745405903 ) ) ;
#69224=CARTESIAN_POINT ( 'NONE',  ( 0.3949938075777409963, 2.418639510665530743E-17, -2.399606299212599048 ) ) ;
#69229=CARTESIAN_POINT ( 'NONE',  ( 0.3458507752293908943, 0.3458507752293908943, -2.814960629921259727 ) ) ;
#69230=CARTESIAN_POINT ( 'NONE',  ( -0.3996062992125986035, -7.340648628747425578E-17, -2.244094488188976388 ) ) ;
#69238=CARTESIAN_POINT ( 'NONE',  ( 4.797336870675656522E-17, -0.3917322834645670104, -0.1633858267716536417 ) ) ;
#69246=CARTESIAN_POINT ( 'NONE',  ( 4.797336870675656522E-17, -0.3917322834645670104, -0.4783464566929135353 ) ) ;
#69247=CARTESIAN_POINT ( 'NONE',  ( 0.3392501089628018329, 0.1958661417322835607, -1.383202099737532942 ) ) ;
#69248=CARTESIAN_POINT ( 'NONE',  ( 0.1049643490035304938, -0.3917322834645669549, -2.912073490813647858 ) ) ;
#69252=CARTESIAN_POINT ( 'NONE',  ( -0.3420746716998659953, -0.1974969037888706647, -2.887139107611548461 ) ) ;
#69256=CARTESIAN_POINT ( 'NONE',  ( 4.893765752498283924E-17, -0.3996062992125986035, -1.338582677165354173 ) ) ;
#69261=CARTESIAN_POINT ( 'NONE',  ( 4.797336870675656522E-17, -0.3917322834645670104, -0.4783464566929135353 ) ) ;
#69270=CARTESIAN_POINT ( 'NONE',  ( 0.1265901696524989462, 0.4724409448818897572, -2.198162729658792447 ) ) ;
#69277=CARTESIAN_POINT ( 'NONE',  ( 0.4091458600556404646, -0.2362204724409448231, -2.309711286089239035 ) ) ;
#69281=CARTESIAN_POINT ( 'NONE',  ( 0.3917322834645668994, 0.1049643490035304522, -0.3621854086276097839 ) ) ;
#69283=CARTESIAN_POINT ( 'NONE',  ( -0.2867679344610366554, 0.2867679344610365444, -0.7342519685039371469 ) ) ;
#69288=CARTESIAN_POINT ( 'NONE',  ( 0.3392501089628018884, -0.1958661417322834220, -2.616797900262466836 ) ) ;
#69291=CARTESIAN_POINT ( 'NONE',  ( 0.4724409448818897572, -0.1265901696524988906, -0.9757217847769029673 ) ) ;
#69304=CARTESIAN_POINT ( 'NONE',  ( 0.1070741851644054776, -0.3996062992125984925, -2.051837270341206665 ) ) ;
#69312=CARTESIAN_POINT ( 'NONE',  ( -0.1070741851644051862, -0.3996062992125986035, -0.6213910761154856077 ) ) ;
#69313=CARTESIAN_POINT ( 'NONE',  ( 0.3460692066303959202, 0.1998031496062993295, -1.076115485564304475 ) ) ;
#69314=CARTESIAN_POINT ( 'NONE',  ( 0.1974969037888706369, -0.3420746716998659953, -0.4068241469816273326 ) ) ;
#69320=CARTESIAN_POINT ( 'NONE',  ( -0.3420746716998662729, 0.1974969037888702206, -1.362860892388451539 ) ) ;
#69326=CARTESIAN_POINT ( 'NONE',  ( 0.1265901696524989462, 0.4724409448818897572, -1.095800524934382958 ) ) ;
#69340=CARTESIAN_POINT ( 'NONE',  ( 4.797336870675656522E-17, -0.3917322834645670104, -1.015748031496062964 ) ) ;
#69343=CARTESIAN_POINT ( 'NONE',  ( -0.2891555358219911054, 0.2891555358219909388, -1.437007874015748143 ) ) ;
#69348=CARTESIAN_POINT ( 'NONE',  ( -0.3996062992125987146, 0.1070741851644051862, -0.03280839895013124008 ) ) ;
#69355=CARTESIAN_POINT ( 'NONE',  ( -0.1049643490035307020, 0.3917322834645669549, 0.2237532808398949025 ) ) ;
#69361=CARTESIAN_POINT ( 'NONE',  ( 0.2925321140481932369, -0.2925321140481932369, -1.988188976377952777 ) ) ;
#69364=CARTESIAN_POINT ( 'NONE',  ( -0.2925321140481930149, -0.2925321140481933480, -1.710629921259842812 ) ) ;
#69368=CARTESIAN_POINT ( 'NONE',  ( 0.1265901696524989462, 0.4724409448818897572, -0.3083989501312335846 ) ) ;
#69370=CARTESIAN_POINT ( 'NONE',  ( -0.3917322834645669549, -0.1049643490035306603, 0.1194225721784776956 ) ) ;
#69377=CARTESIAN_POINT ( 'NONE',  ( -0.2362204724409447953, -0.4091458600556404646, -2.347112860892388575 ) ) ;
#69379=CARTESIAN_POINT ( 'NONE',  ( -0.1058382717557497660, -0.3949938075777411073, -2.196194225721785021 ) ) ;
#69402=CARTESIAN_POINT ( 'NONE',  ( 0.3996062992125984925, 0.1070741851644054637, -0.8313648293963252778 ) ) ;
#69403=CARTESIAN_POINT ( 'NONE',  ( 0.1049643490035303689, 0.3917322834645670104, -2.440288713910760521 ) ) ;
#69418=CARTESIAN_POINT ( 'NONE',  ( 0.1049643490035303689, 0.3917322834645670104, -2.125328083989501682 ) ) ;
#69419=CARTESIAN_POINT ( 'NONE',  ( 0.1789624963018512649, 0.3486222174624337145, -1.220472440944881276 ) ) ;
#69425=CARTESIAN_POINT ( 'NONE',  ( 0.2925321140481931814, 0.2925321140481931814, -2.261811023622047223 ) ) ;
#69427=CARTESIAN_POINT ( 'NONE',  ( 0.2925321140481932369, 0.2925321140481932369, -1.082677165354330562 ) ) ;
#69429=CARTESIAN_POINT ( 'NONE',  ( 0.1958661417322834775, 0.3392501089628018884, -2.656167979002624691 ) ) ;
#69442=CARTESIAN_POINT ( 'NONE',  ( 0.1049643490035304938, -0.3917322834645669549, -2.847112860892388131 ) ) ;
#69445=CARTESIAN_POINT ( 'NONE',  ( -0.2891555358219908833, -0.2891555358219912164, -0.3740157480314962313 ) ) ;
#69453=CARTESIAN_POINT ( 'NONE',  ( 0.3392501089628018329, 0.1958661417322835607, -1.702775221293650443 ) ) ;
#69455=CARTESIAN_POINT ( 'NONE',  ( -0.1049643490035302024, -0.3917322834645671215, -2.519028871391075786 ) ) ;
#69460=CARTESIAN_POINT ( 'NONE',  ( -0.3996062992125987146, 0.1070741851644051862, -0.8202099737532806412 ) ) ;
#69462=CARTESIAN_POINT ( 'NONE',  ( 0.1998031496062994128, -0.3460692066303957537, -0.3261154855643044748 ) ) ;
#69464=CARTESIAN_POINT ( 'NONE',  ( 0.2925321140481932369, -0.2925321140481932369, -2.460629921259842146 ) ) ;
#69465=CARTESIAN_POINT ( 'NONE',  ( -0.3917322834645670104, -7.196005306013484475E-17, -1.698818897637795367 ) ) ;
#69469=CARTESIAN_POINT ( 'NONE',  ( 0.4724409448818896462, 0.1265901696524990294, -0.9888451443569553634 ) ) ;
#69472=CARTESIAN_POINT ( 'NONE',  ( -0.3420746716998662729, 0.1974969037888702206, -0.8904199475065616154 ) ) ;
#69483=CARTESIAN_POINT ( 'NONE',  ( -0.1998031496062991630, -0.3460692066303959202, -1.717191601049869121 ) ) ;
#69500=CARTESIAN_POINT ( 'NONE',  ( 0.2867679344610365999, 0.2867679344610365999, -1.167322834645669438 ) ) ;
#69515=CARTESIAN_POINT ( 'NONE',  ( 0.3458507752293908943, -0.3458507752293908943, -0.5708661417322833387 ) ) ;
#69522=CARTESIAN_POINT ( 'NONE',  ( -1.157146581871515012E-16, 0.4724409448818898682, -0.3149606299212598381 ) ) ;
#69523=CARTESIAN_POINT ( 'NONE',  ( -0.2891555358219911054, 0.2891555358219909388, -2.696850393700787496 ) ) ;
#69526=CARTESIAN_POINT ( 'NONE',  ( -0.2867679344610365999, 0.2867679344610364889, -1.271653543307086798 ) ) ;
#69528=CARTESIAN_POINT ( 'NONE',  ( 0.3458507752293908943, -0.3458507752293908943, -2.460629921259842146 ) ) ;
#69529=DIRECTION ( 'NONE',  ( -0.000000000000000000, -0.000000000000000000, -1.000000000000000000 ) ) ;
#69535=CARTESIAN_POINT ( 'NONE',  ( -0.2867679344610366554, 0.2867679344610365444, -0.8871197918297093477 ) ) ;
#69543=CARTESIAN_POINT ( 'NONE',  ( 0.2867679344610366554, 0.2867679344610366554, -2.024297531004936701 ) ) ;
#69551=CARTESIAN_POINT ( 'NONE',  ( -0.3917322834645671215, 0.1049643490035301469, -1.219816272965879023 ) ) ;
#69558=CARTESIAN_POINT ( 'NONE',  ( 0.4724409448818898127, -0.1265901696524988629, -0.9757217847769029673 ) ) ;
#69560=CARTESIAN_POINT ( 'NONE',  ( 0.2867679344610365999, -0.2867679344610365444, -2.610236220472441193 ) ) ;
#69566=CARTESIAN_POINT ( 'NONE',  ( 0.2362204724409451007, -0.4091458600556402980, -0.4068241469816273326 ) ) ;
#69567=CARTESIAN_POINT ( 'NONE',  ( 0.1958661417322836440, -0.3392501089628017219, -1.121391076115485719 ) ) ;
#69568=CARTESIAN_POINT ( 'NONE',  ( 0.4724409448818898682, 2.892866454678787531E-17, 0.1200787401574803098 ) ) ;
#69570=CARTESIAN_POINT ( 'NONE',  ( -0.1070741851644056997, 0.3996062992125984925, -2.760498687664041384 ) ) ;
#69580=CARTESIAN_POINT ( 'NONE',  ( 0.1070741851644054776, -0.3996062992125984925, -0.3195538057742782212 ) ) ;
#69582=CARTESIAN_POINT ( 'NONE',  ( -0.3917322834645670104, -7.196005306013484475E-17, -0.03149606299212594218 ) ) ;
#69597=CARTESIAN_POINT ( 'NONE',  ( 4.797336870675656522E-17, -0.3917322834645670659, -1.020360523130920738 ) ) ;
#69602=CARTESIAN_POINT ( 'NONE',  ( -0.2362204724409451284, 0.4091458600556402425, -2.294619422572178102 ) ) ;
#69606=DIRECTION ( 'NONE',  ( 0.000000000000000000, 0.000000000000000000, 1.000000000000000000 ) ) ;
#69622=CARTESIAN_POINT ( 'NONE',  ( 0.1998031496062992740, 0.3460692066303959757, -0.1443569553805774397 ) ) ;
#69623=CARTESIAN_POINT ( 'NONE',  ( -0.1070741851644056997, 0.3996062992125984925, -2.760498687664041384 ) ) ;
#69628=CARTESIAN_POINT ( 'NONE',  ( 0.1998031496062994405, -0.3460692066303958092, -2.296587926509186417 ) ) ;
#69629=CARTESIAN_POINT ( 'NONE',  ( 0.1974969037888704704, 0.3420746716998660508, -1.404199475065616820 ) ) ;
#69631=CARTESIAN_POINT ( 'NONE',  ( -0.1265901696524993347, 0.4724409448818896462, -2.526246719160104792 ) ) ;
#69632=CARTESIAN_POINT ( 'NONE',  ( 0.2867679344610366554, -0.2867679344610365444, -0.7204724409448818312 ) ) ;
#69635=CARTESIAN_POINT ( 'NONE',  ( -0.1058382717557503072, 0.3949938075777408852, -2.445538057742782101 ) ) ;
#69640=CARTESIAN_POINT ( 'NONE',  ( 0.4091458600556404646, -0.2362204724409448231, -2.939632545931758489 ) ) ;
#69641=CARTESIAN_POINT ( 'NONE',  ( 0.1998031496062992740, 0.3460692066303959757, -2.349081364829396446 ) ) ;
#69642=CYLINDRICAL_SURFACE ( 'NONE', #39931, 0.4724409448818898682 ) ;
#69648=CARTESIAN_POINT ( 'NONE',  ( -0.1958661417322834220, -0.3392501089628018884, -0.3077427821522311091 ) ) ;
#69655=CARTESIAN_POINT ( 'NONE',  ( 0.2867679344610365999, -0.2867679344610365444, -0.4980314960629922405 ) ) ;
#69656=CARTESIAN_POINT ( 'NONE',  ( 0.1958661417322836440, -0.3392501089628017219, -1.501312335958005173 ) ) ;
#69657=CARTESIAN_POINT ( 'NONE',  ( 0.2867679344610365999, -0.2867679344610365444, -2.767716535433069946 ) ) ;
#69660=CARTESIAN_POINT ( 'NONE',  ( 0.1058382717557499880, 0.3949938075777411073, -2.670603674540682260 ) ) ;
#69665=CARTESIAN_POINT ( 'NONE',  ( 0.1070741851644054915, -0.3996062992125986035, -1.502624671916010346 ) ) ;
#69670=CARTESIAN_POINT ( 'NONE',  ( -0.3392501089628017219, -0.1958661417322836718, -0.4520997375328084655 ) ) ;
#69680=CARTESIAN_POINT ( 'NONE',  ( -1.157146581871515012E-16, 0.4724409448818898682, -2.047244094488188892 ) ) ;
#69690=CARTESIAN_POINT ( 'NONE',  ( 0.1958661417322836162, -0.3392501089628018329, -0.3293770096774785161 ) ) ;
#69692=CARTESIAN_POINT ( 'NONE',  ( 4.797336870675656522E-17, -0.3917322834645670104, -0.9507874015748032370 ) ) ;
#69697=CARTESIAN_POINT ( 'NONE',  ( 0.3917322834645670104, 2.398668435337828261E-17, -2.787401574803149096 ) ) ;
#69701=CARTESIAN_POINT ( 'NONE',  ( 0.4724409448818896462, 0.1265901696524990294, -0.6738845144356955252 ) ) ;
#69713=CARTESIAN_POINT ( 'NONE',  ( -9.787531504996566615E-17, 0.3996062992125985480, -1.809055118110236560 ) ) ;
#69721=CARTESIAN_POINT ( 'NONE',  ( -0.1070741851644057135, 0.3996062992125984925, -0.8707349081364829102 ) ) ;
#69722=CARTESIAN_POINT ( 'NONE',  ( 0.3996062992125986590, -0.1070741851644053111, -0.8989501312335956840 ) ) ;
#69723=CARTESIAN_POINT ( 'NONE',  ( -0.1058382717557497937, -0.3949938075777411628, -0.3871391076115485719 ) ) ;
#69729=CARTESIAN_POINT ( 'NONE',  ( 0.1974969037888704704, 0.3420746716998660508, -1.166010498687664265 ) ) ;
#69735=CARTESIAN_POINT ( 'NONE',  ( 0.2362204724409451007, -0.4091458600556402980, -1.509186351706036655 ) ) ;
#69748=CARTESIAN_POINT ( 'NONE',  ( -9.594673741351313045E-17, 0.3917322834645670104, -1.251968503937008093 ) ) ;
#69751=CARTESIAN_POINT ( 'NONE',  ( 0.2891555358219910499, 0.2891555358219910499, -1.397637795275590733 ) ) ;
#69756=CARTESIAN_POINT ( 'NONE',  ( -9.787531504996567848E-17, 0.3996062992125986035, -0.1574803149606299191 ) ) ;
#69764=CARTESIAN_POINT ( 'NONE',  ( -0.3917322834645669549, -0.1049643490035306603, 0.02690288713910752097 ) ) ;
#69767=ADVANCED_FACE ( 'NONE', ( #11187 ), #36434, .T. ) ;
#69771=CARTESIAN_POINT ( 'NONE',  ( -0.1070741851644056997, 0.3996062992125986035, -2.053805774278214979 ) ) ;
#69774=CARTESIAN_POINT ( 'NONE',  ( 0.1998031496062994128, -0.3460692066303957537, -1.585958005249344049 ) ) ;
#69779=CARTESIAN_POINT ( 'NONE',  ( 0.2362204724409451007, -0.4091458600556402980, -1.036745406824147064 ) ) ;
#69781=CARTESIAN_POINT ( 'NONE',  ( 0.1049643490035304938, -0.3917322834645669549, -2.847112860892388131 ) ) ;
#69783=CARTESIAN_POINT ( 'NONE',  ( -9.594673741351313045E-17, 0.3917322834645670104, -2.131889763779527769 ) ) ;
#69787=CARTESIAN_POINT ( 'NONE',  ( -0.3458507752293906723, -0.3458507752293910609, -2.655511811023622215 ) ) ;
#69789=CARTESIAN_POINT ( 'NONE',  ( -0.1058382717557497660, -0.3949938075777411073, -2.038713910761155379 ) ) ;
#69794=CARTESIAN_POINT ( 'NONE',  ( 0.2362204724409451007, -0.4091458600556402980, -2.215879265091863726 ) ) ;
#69809=CARTESIAN_POINT ( 'NONE',  ( 0.2925321140481932369, 0.2925321140481932369, -0.6870078740157479213 ) ) ;
#69810=CARTESIAN_POINT ( 'NONE',  ( -0.1049643490035302024, -0.3917322834645671215, -2.046587926509185973 ) ) ;
#69815=CARTESIAN_POINT ( 'NONE',  ( -0.4724409448818898682, -8.678599364036362592E-17, -0.1161417322834645827 ) ) ;
#69820=CARTESIAN_POINT ( 'NONE',  ( 0.1958661417322836718, -0.3392501089628017219, -1.978365772474752537 ) ) ;
#69826=CARTESIAN_POINT ( 'NONE',  ( -0.2867679344610365999, 0.2867679344610364889, -1.836614173228346747 ) ) ;
#69833=CARTESIAN_POINT ( 'NONE',  ( -0.1070741851644051862, -0.3996062992125987146, -0.7020997375328084100 ) ) ;
#69835=CARTESIAN_POINT ( 'NONE',  ( 0.1049643490035304938, -0.3917322834645669549, -2.597112860892388131 ) ) ;
#69847=CARTESIAN_POINT ( 'NONE',  ( -9.594673741351313045E-17, 0.3917322834645670104, 0.007874015748031542791 ) ) ;
#69850=CARTESIAN_POINT ( 'NONE',  ( -0.1974969037888703871, -0.3420746716998661063, -0.2230971128608924547 ) ) ;
#69858=CARTESIAN_POINT ( 'NONE',  ( 0.3917322834645670659, 2.398668435337828261E-17, -1.847132176674227688 ) ) ;
#69860=CARTESIAN_POINT ( 'NONE',  ( -0.3392501089628019995, 0.1958661417322832277, -2.473097112860892288 ) ) ;
#69865=CARTESIAN_POINT ( 'NONE',  ( -0.2925321140481932924, 0.2925321140481931814, -0.8070866141732284671 ) ) ;
#69867=CARTESIAN_POINT ( 'NONE',  ( -0.3996062992125986590, 0.1070741851644051723, -0.4245406824146981672 ) ) ;
#69868=CARTESIAN_POINT ( 'NONE',  ( -0.1070741851644056997, 0.3996062992125984925, -0.08333333333333337034 ) ) ;
#69870=CARTESIAN_POINT ( 'NONE',  ( -0.3996062992125987146, 0.1070741851644051862, -2.867454068241469756 ) ) ;
#69871=CARTESIAN_POINT ( 'NONE',  ( 0.1958661417322834775, 0.3392501089628018884, -1.646325459317585338 ) ) ;
#69875=CARTESIAN_POINT ( 'NONE',  ( -0.4724409448818898682, -8.678599364036362592E-17, -1.690944881889763884 ) ) ;
#69878=CARTESIAN_POINT ( 'NONE',  ( -9.674558042662122972E-17, 0.3949938075777409963, -0.8641732283464566011 ) ) ;
#69887=CARTESIAN_POINT ( 'NONE',  ( 0.1070741851644054776, -0.3996062992125984925, -1.894356955380577023 ) ) ;
#69890=DIRECTION ( 'NONE',  ( 1.000000000000000000, 0.000000000000000000, 0.000000000000000000 ) ) ;
#69901=CARTESIAN_POINT ( 'NONE',  ( 0.3392501089628018329, 0.1958661417322835607, -1.003280839895013266 ) ) ;
#69909=FACE_OUTER_BOUND ( 'NONE', #46929, .T. ) ;
#69920=CARTESIAN_POINT ( 'NONE',  ( -0.1049643490035307020, 0.3917322834645669549, -2.203412073490813583 ) ) ;
#69923=CARTESIAN_POINT ( 'NONE',  ( 0.3458507752293908943, 0.3458507752293908943, -0.4527559055118109965 ) ) ;
#69924=CARTESIAN_POINT ( 'NONE',  ( 0.2891555358219910499, -0.2891555358219909944, -2.618110236220472675 ) ) ;
#69925=VERTEX_POINT ( 'NONE', #24209 ) ;
#69927=CARTESIAN_POINT ( 'NONE',  ( 4.797336870675656522E-17, -0.3917322834645670104, -1.488188976377952777 ) ) ;
#69929=CARTESIAN_POINT ( 'NONE',  ( -0.4091458600556402980, -0.2362204724409451284, -2.887139107611548461 ) ) ;
#69936=CARTESIAN_POINT ( 'NONE',  ( -0.3917322834645669549, -7.196005306013483243E-17, -0.9068048311997882749 ) ) ;
#69944=CARTESIAN_POINT ( 'NONE',  ( 0.1049643490035303967, 0.3917322834645670659, -1.879940575624358789 ) ) ;
#69952=CARTESIAN_POINT ( 'NONE',  ( -0.2867679344610365999, 0.2867679344610364889, -1.521653543307086354 ) ) ;
#69961=CARTESIAN_POINT ( 'NONE',  ( -0.3392501089628019995, 0.1958661417322832277, -2.695538057742782101 ) ) ;
#69967=CARTESIAN_POINT ( 'NONE',  ( 0.4724409448818898682, 2.892866454678787531E-17, -0.4330708661417322913 ) ) ;
#69968=CARTESIAN_POINT ( 'NONE',  ( 0.3392501089628018329, 0.1958661417322835607, -1.003280839895013266 ) ) ;
#69969=CARTESIAN_POINT ( 'NONE',  ( -0.1265901696524986964, -0.4724409448818899238, 0.008530183727034111943 ) ) ;
#69972=CARTESIAN_POINT ( 'NONE',  ( 0.1974969037888706092, -0.3420746716998660508, 0.1463254593175853102 ) ) ;
#69982=CARTESIAN_POINT ( 'NONE',  ( 0.3996062992125984925, 0.1070741851644054637, -0.5164041994750655507 ) ) ;
#69984=CARTESIAN_POINT ( 'NONE',  ( 0.3917322834645669549, 0.1049643490035304660, -0.4317585301837270628 ) ) ;
#69998=CARTESIAN_POINT ( 'NONE',  ( 0.3917322834645670659, -0.1049643490035303273, -0.7382082921597920011 ) ) ;
#70002=CARTESIAN_POINT ( 'NONE',  ( -0.3458507752293906723, -0.3458507752293910609, -2.340551181102362488 ) ) ;
#70022=CARTESIAN_POINT ( 'NONE',  ( 0.2925321140481932369, 0.2925321140481932369, -0.4527559055118110520 ) ) ;
#70023=CARTESIAN_POINT ( 'NONE',  ( 0.2925321140481932369, 0.2925321140481932369, -2.576771653543307394 ) ) ;
#70028=CARTESIAN_POINT ( 'NONE',  ( -0.3996062992125986035, -0.1070741851644056997, -2.250656167979002920 ) ) ;
#70029=CARTESIAN_POINT ( 'NONE',  ( 0.2891555358219910499, -0.2891555358219909944, -1.358267716535433101 ) ) ;
#70032=CARTESIAN_POINT ( 'NONE',  ( 0.3917322834645669549, 0.1049643490035304660, -0.4317585301837270073 ) ) ;
#70035=CARTESIAN_POINT ( 'NONE',  ( 0.2891555358219910499, 0.2891555358219910499, -2.419291338582677753 ) ) ;
#70039=CARTESIAN_POINT ( 'NONE',  ( 0.4724409448818895907, 0.1265901696524994180, -0.04396325459317588363 ) ) ;
#70040=CARTESIAN_POINT ( 'NONE',  ( 0.3996062992125986035, 2.446882876249141962E-17, -2.322834645669291209 ) ) ;
#70046=CARTESIAN_POINT ( 'NONE',  ( -0.1958661417322834220, -0.3392501089628018884, 0.007217847769028785422 ) ) ;
#70054=CARTESIAN_POINT ( 'NONE',  ( -0.1958661417322836718, 0.3392501089628017219, -0.5702099737532808632 ) ) ;
#70055=CARTESIAN_POINT ( 'NONE',  ( 0.2867679344610365999, 0.2867679344610365999, -1.389763779527558807 ) ) ;
#70056=CARTESIAN_POINT ( 'NONE',  ( 0.1958661417322834775, 0.3392501089628018884, -2.656167979002624691 ) ) ;
#70058=CARTESIAN_POINT ( 'NONE',  ( 0.3460692066303959202, 0.1998031496062993295, -0.1312335958005249603 ) ) ;
#70062=CARTESIAN_POINT ( 'NONE',  ( -0.3460692066303960868, 0.1998031496062990242, -1.286089238845144367 ) ) ;
#70067=CARTESIAN_POINT ( 'NONE',  ( -9.594673741351313045E-17, 0.3917322834645670104, -0.8720472440944883052 ) ) ;
#70077=CARTESIAN_POINT ( 'NONE',  ( 0.4091458600556403535, 0.2362204724409449896, -2.020997375328084100 ) ) ;
#70083=CARTESIAN_POINT ( 'NONE',  ( 0.4724409448818915891, -0.1265901696524958653, -2.316272965879265566 ) ) ;
#70087=CARTESIAN_POINT ( 'NONE',  ( 0.3917322834645668994, -0.1049643490035303134, -0.5065423640081871959 ) ) ;
#70089=CARTESIAN_POINT ( 'NONE',  ( 0.3917322834645669549, 0.1049643490035304660, -0.6817585301837267853 ) ) ;
#70094=CARTESIAN_POINT ( 'NONE',  ( -0.3917322834645669549, -0.1049643490035306603, -2.715223097112861250 ) ) ;
#70099=CARTESIAN_POINT ( 'NONE',  ( 0.1265901696524989462, 0.4724409448818897572, -1.015091863517060267 ) ) ;
#70112=CARTESIAN_POINT ( 'NONE',  ( 0.1070741851644054776, -0.3996062992125984925, -2.209317585301837195 ) ) ;
#70116=CARTESIAN_POINT ( 'NONE',  ( -0.1070741851644056997, 0.3996062992125984925, -1.185695538057742526 ) ) ;
#70122=CARTESIAN_POINT ( 'NONE',  ( -0.1998031496062994405, 0.3460692066303957537, -0.7198162729658792447 ) ) ;
#70123=CARTESIAN_POINT ( 'NONE',  ( 0.1070741851644053527, 0.3996062992125986590, -0.7808398950131233418 ) ) ;
#70124=CARTESIAN_POINT ( 'NONE',  ( -0.1974969037888703871, -0.3420746716998661063, -0.06561679790026252179 ) ) ;
#70130=CARTESIAN_POINT ( 'NONE',  ( -0.3420746716998662729, 0.1974969037888702206, -1.520341207349081181 ) ) ;
#70135=CARTESIAN_POINT ( 'NONE',  ( -0.4091458600556405756, 0.2362204724409446288, -1.443569553805774230 ) ) ;
#70143=CARTESIAN_POINT ( 'NONE',  ( -9.594673741351310580E-17, 0.3917322834645669549, -1.812316642223410046 ) ) ;
#70150=CARTESIAN_POINT ( 'NONE',  ( 0.3917322834645670104, 2.398668435337828261E-17, -1.527559055118110409 ) ) ;
#70153=CARTESIAN_POINT ( 'NONE',  ( 0.2891555358219910499, -0.2891555358219909944, -1.673228346456693272 ) ) ;
#70158=CARTESIAN_POINT ( 'NONE',  ( -0.1070741851644056997, 0.3996062992125986035, -0.3215223097112860362 ) ) ;
#70165=CARTESIAN_POINT ( 'NONE',  ( 0.1958661417322834775, 0.3392501089628018884, 0.08595800524934374409 ) ) ;
#70170=EDGE_LOOP ( 'NONE', ( #36215, #74029, #72240, #41207 ) ) ;
#70171=ORIENTED_EDGE ( 'NONE', *, *, #68721, .F. ) ;
#70172=CARTESIAN_POINT ( 'NONE',  ( -9.787531504996566615E-17, 0.3996062992125985480, -1.809055118110236560 ) ) ;
#70178=CARTESIAN_POINT ( 'NONE',  ( 5.785732909357575061E-17, -0.4724409448818898682, -0.8661417322834645827 ) ) ;
#70180=CARTESIAN_POINT ( 'NONE',  ( -0.3392501089628017219, -0.1958661417322836718, -0.04461942257217842850 ) ) ;
#70182=CARTESIAN_POINT ( 'NONE',  ( 0.2867679344610366554, 0.2867679344610366554, -1.954724409448818978 ) ) ;
#70186=CARTESIAN_POINT ( 'NONE',  ( -0.3458507752293909498, 0.3458507752293907833, -2.773622047244094002 ) ) ;
#70189=CARTESIAN_POINT ( 'NONE',  ( 0.1058382717557500852, -0.3949938075777408852, -2.051837270341207109 ) ) ;
#70198=CARTESIAN_POINT ( 'NONE',  ( -0.2362204724409451284, 0.4091458600556402425, -0.08989501312335958227 ) ) ;
#70210=CARTESIAN_POINT ( 'NONE',  ( -0.1998031496062991630, -0.3460692066303959202, -1.244750656167979086 ) ) ;
#70211=CARTESIAN_POINT ( 'NONE',  ( 0.2867679344610365999, 0.2867679344610365999, -2.269685039370078705 ) ) ;
#70223=CARTESIAN_POINT ( 'NONE',  ( 0.2867679344610366554, -0.2867679344610365999, -2.299888082186038574 ) ) ;
#70230=CARTESIAN_POINT ( 'NONE',  ( -9.594673741351313045E-17, 0.3917322834645670104, -1.974409448818897683 ) ) ;
#70235=CARTESIAN_POINT ( 'NONE',  ( 0.3460692066303958092, 0.1998031496062993018, -2.727690288713910949 ) ) ;
#70237=CARTESIAN_POINT ( 'NONE',  ( 0.2925321140481932369, -0.2925321140481932369, -1.200787401574803015 ) ) ;
#70239=CARTESIAN_POINT ( 'NONE',  ( 0.1958661417322834775, 0.3392501089628018884, 0.01638488369322645480 ) ) ;
#70253=CARTESIAN_POINT ( 'NONE',  ( -0.1958661417322834220, -0.3392501089628018884, -0.05774278215223092176 ) ) ;
#70256=CARTESIAN_POINT ( 'NONE',  ( -0.3949938075777409963, -7.255918531996591613E-17, -0.1968503937007874682 ) ) ;
#70263=ADVANCED_FACE ( 'NONE', ( #81629 ), #24756, .T. ) ;
#70264=CARTESIAN_POINT ( 'NONE',  ( 0.3392501089628018329, 0.1958661417322835607, -1.860255536254279862 ) ) ;
#70266=CARTESIAN_POINT ( 'NONE',  ( -0.3917322834645671215, 0.1049643490035301469, -2.479658792650918375 ) ) ;
#70268=CIRCLE ( 'NONE', #28652, 0.4724409448818898682 ) ;
#70271=CARTESIAN_POINT ( 'NONE',  ( -0.3460692066303960868, 0.1998031496062990242, -0.8136482939632546652 ) ) ;
#70273=CARTESIAN_POINT ( 'NONE',  ( 0.3460692066303958092, 0.1998031496062993018, -0.2080052493438320216 ) ) ;
#70274=CARTESIAN_POINT ( 'NONE',  ( 0.1070741851644054776, -0.3996062992125984925, -0.1620734908136483299 ) ) ;
#70276=CARTESIAN_POINT ( 'NONE',  ( 0.2925321140481932369, -0.2925321140481932369, -2.618110236220472675 ) ) ;
#70278=CARTESIAN_POINT ( 'NONE',  ( -0.1958661417322836718, 0.3392501089628017219, -1.672572178477690352 ) ) ;
#70283=CARTESIAN_POINT ( 'NONE',  ( -0.4724409448818898682, -8.678599364036362592E-17, -1.533464566929133799 ) ) ;
#70287=CARTESIAN_POINT ( 'NONE',  ( -0.3949938075777408852, -0.1058382717557502933, -1.067585301837270739 ) ) ;
#70296=CARTESIAN_POINT ( 'NONE',  ( -0.2925321140481930149, -0.2925321140481933480, -2.183070866141731958 ) ) ;
#70299=CARTESIAN_POINT ( 'NONE',  ( 4.797336870675655290E-17, -0.3917322834645669549, -1.733576484743095669 ) ) ;
#70312=CARTESIAN_POINT ( 'NONE',  ( -0.3392501089628017219, -0.1958661417322836718, -0.9245406824146982228 ) ) ;
#70333=CARTESIAN_POINT ( 'NONE',  ( -0.3392501089628017219, -0.1958661417322836718, -2.091863517060367439 ) ) ;
#70337=CARTESIAN_POINT ( 'NONE',  ( 0.1265901696524989462, 0.4724409448818897572, -0.4658792650918635592 ) ) ;
#70338=CARTESIAN_POINT ( 'NONE',  ( 0.1070741851644054915, -0.3996062992125986035, 0.07217847769028869209 ) ) ;
#70339=ORIENTED_EDGE ( 'NONE', *, *, #3924, .T. ) ;
#70342=CARTESIAN_POINT ( 'NONE',  ( 0.3917322834645670104, -0.1049643490035303411, -1.993438320209974135 ) ) ;
#70344=CARTESIAN_POINT ( 'NONE',  ( 0.4724409448818896462, 0.1265901696524990294, -2.801837270341207553 ) ) ;
#70350=CARTESIAN_POINT ( 'NONE',  ( 0.1049643490035304522, -0.3917322834645668994, -0.6377759598087122672 ) ) ;
#70357=CARTESIAN_POINT ( 'NONE',  ( 0.1958661417322834775, 0.3392501089628018884, -2.030859210794962344 ) ) ;
#70364=CARTESIAN_POINT ( 'NONE',  ( -0.3917322834645670104, -7.196005306013484475E-17, -1.226377952755905776 ) ) ;
#70369=CARTESIAN_POINT ( 'NONE',  ( -0.002674255378528274645, 0.3979867861068626111, 1.060393565908085801E-17 ) ) ;
#70379=CARTESIAN_POINT ( 'NONE',  ( -0.3996062992125986035, -1.273259842764937629E-12, -1.929133858267794599 ) ) ;
#70380=CARTESIAN_POINT ( 'NONE',  ( 0.3392501089628018329, 0.1958661417322835607, -1.318241469816273215 ) ) ;
#70381=CARTESIAN_POINT ( 'NONE',  ( 0.2362204724409449064, 0.4091458600556404646, -0.06364829396325459576 ) ) ;
#70384=CARTESIAN_POINT ( 'NONE',  ( 0.3460692066303958092, 0.1998031496062993018, -2.727690288713910949 ) ) ;
#70390=CARTESIAN_POINT ( 'NONE',  ( 0.1974969037888706092, -0.3420746716998660508, -0.01115485564304462274 ) ) ;
#70397=CARTESIAN_POINT ( 'NONE',  ( 0.3996062992125984925, 0.1070741851644054637, -0.8313648293963252778 ) ) ;
#70399=CARTESIAN_POINT ( 'NONE',  ( 0.1049643490035304938, -0.3917322834645669549, -0.07742782152230967552 ) ) ;
#70413=CARTESIAN_POINT ( 'NONE',  ( 0.3392501089628018884, -0.1958661417322833942, -0.7316466123697656920 ) ) ;
#70418=CARTESIAN_POINT ( 'NONE',  ( -0.4724409448818898682, -8.678599364036362592E-17, -2.635826771653543066 ) ) ;
#70434=CARTESIAN_POINT ( 'NONE',  ( -0.3996062992125985480, -0.1070741851644057135, -0.5183727034120735322 ) ) ;
#70435=CARTESIAN_POINT ( 'NONE',  ( 0.1998031496062994128, -0.3460692066303957537, -2.845800524934383624 ) ) ;
#70440=CARTESIAN_POINT ( 'NONE',  ( 0.1998031496062992740, 0.3460692066303959757, -2.191601049868766360 ) ) ;
#70441=CARTESIAN_POINT ( 'NONE',  ( -0.1974969037888703871, -0.3420746716998661063, -1.640419947506561948 ) ) ;
#70442=CARTESIAN_POINT ( 'NONE',  ( 4.893765752498283924E-17, -0.3996062992125986035, -2.755905511811023612 ) ) ;
#70443=CARTESIAN_POINT ( 'NONE',  ( 0.2362204724409449064, 0.4091458600556404646, -2.506561679790026087 ) ) ;
#70445=CARTESIAN_POINT ( 'NONE',  ( 0.3917322834645670104, 2.398668435337828261E-17, -0.8976377952755905110 ) ) ;
#70448=CARTESIAN_POINT ( 'NONE',  ( -0.2891555358219909388, -0.2891555358219912164, -2.655511811023621771 ) ) ;
#70452=CARTESIAN_POINT ( 'NONE',  ( -1.157146581871515012E-16, 0.4724409448818898682, -2.834645669291338432 ) ) ;
#70453=CARTESIAN_POINT ( 'NONE',  ( 0.3996062992125986035, 0.1070741851644054776, -2.014435695538057569 ) ) ;
#70454=CARTESIAN_POINT ( 'NONE',  ( -0.3917322834645671770, 0.1049643490035302024, -0.9744287646007369075 ) ) ;
#70461=CARTESIAN_POINT ( 'NONE',  ( -0.1049643490035307020, 0.3917322834645669549, -0.2486876640419948270 ) ) ;
#70469=CARTESIAN_POINT ( 'NONE',  ( -0.2867679344610365999, 0.2867679344610364889, -0.7342519685039372579 ) ) ;
#70470=CARTESIAN_POINT ( 'NONE',  ( 0.1958661417322834775, 0.3392501089628018884, -1.553805774278215202 ) ) ;
#70471=CARTESIAN_POINT ( 'NONE',  ( 0.2867679344610365999, -0.2867679344610365444, -2.610236220472441193 ) ) ;
#70473=CARTESIAN_POINT ( 'NONE',  ( 0.2925321140481932369, 0.2925321140481932369, -0.1377952755905512139 ) ) ;
#70477=CARTESIAN_POINT ( 'NONE',  ( 0.3996062992125986590, -0.1070741851644053111, -1.528871391076114916 ) ) ;
#70481=CARTESIAN_POINT ( 'NONE',  ( 0.3937527723457950324, -0.009287274676460888917, -1.929133858267718660 ) ) ;
#70482=CARTESIAN_POINT ( 'NONE',  ( 0.3917322834645670104, -0.1049643490035303411, -0.9835958005249345604 ) ) ;
#70491=CARTESIAN_POINT ( 'NONE',  ( -0.4724409448818899238, 0.1265901696524986686, -1.922572178477689908 ) ) ;
#70501=CARTESIAN_POINT ( 'NONE',  ( -0.3392501089628019439, 0.1958661417322832554, -0.7362011566591059042 ) ) ;
#70503=CARTESIAN_POINT ( 'NONE',  ( 0.3917322834645670104, -0.1049643490035303273, -0.8261154855643044748 ) ) ;
#70509=CARTESIAN_POINT ( 'NONE',  ( -0.1958661417322836718, 0.3392501089628017219, -2.682414698162729483 ) ) ;
#70513=CARTESIAN_POINT ( 'NONE',  ( -0.4724409448818899238, 0.1265901696524986686, -1.211942257217847541 ) ) ;
#70517=AXIS2_PLACEMENT_3D ( 'NONE', #24211, #17105, #56199 ) ;
#70526=CARTESIAN_POINT ( 'NONE',  ( -0.3996062992125985480, -7.340648628747423112E-17, -2.478346456692913868 ) ) ;
#70531=CARTESIAN_POINT ( 'NONE',  ( -0.2925321140481930149, -0.2925321140481933480, -1.238188976377952999 ) ) ;
#70535=CARTESIAN_POINT ( 'NONE',  ( -0.2362204724409447953, -0.4091458600556404646, -0.06561679790026246628 ) ) ;
#70537=CARTESIAN_POINT ( 'NONE',  ( 0.3460692066303958092, 0.1998031496062993018, -0.5229658792650918597 ) ) ;
#70538=CARTESIAN_POINT ( 'NONE',  ( -0.1070741851644051862, -0.3996062992125987146, -1.017060367454067915 ) ) ;
#70539=CARTESIAN_POINT ( 'NONE',  ( 0.2891555358219910499, -0.2891555358219909944, -0.09842519685039378963 ) ) ;
#70542=ADVANCED_FACE ( 'NONE', ( #18466 ), #17646, .T. ) ;
#70545=CARTESIAN_POINT ( 'NONE',  ( -0.2362204724409447953, -0.4091458600556404646, -2.347112860892388575 ) ) ;
#70546=CARTESIAN_POINT ( 'NONE',  ( 0.3949938075777409963, 2.418639510665530743E-17, -1.139763779527559251 ) ) ;
#70551=CARTESIAN_POINT ( 'NONE',  ( 0.2362204724409449064, 0.4091458600556404646, -1.404199475065616820 ) ) ;
#70560=CARTESIAN_POINT ( 'NONE',  ( -0.3917322834645668994, -0.1049643490035306742, -2.015728715714224517 ) ) ;
#70568=CARTESIAN_POINT ( 'NONE',  ( -0.2867679344610364334, -0.2867679344610367109, -1.625984251968503491 ) ) ;
#70571=CARTESIAN_POINT ( 'NONE',  ( -0.2891555358219908833, -0.2891555358219912164, -1.791338582677165725 ) ) ;
#70572=VERTEX_POINT ( 'NONE', #51244 ) ;
#70576=CARTESIAN_POINT ( 'NONE',  ( -0.3460692066303958092, -0.1998031496062994683, -0.05249343832020997996 ) ) ;
#70580=CARTESIAN_POINT ( 'NONE',  ( 0.4724409448818898682, 0.000000000000000000, -2.755905511811024056 ) ) ;
#70584=CARTESIAN_POINT ( 'NONE',  ( 0.3917322834645670104, 2.398668435337828261E-17, -0.3602362204724410266 ) ) ;
#70591=CARTESIAN_POINT ( 'NONE',  ( 0.1070741851644053388, 0.3996062992125986035, -1.959973753280839892 ) ) ;
#70596=CARTESIAN_POINT ( 'NONE',  ( -0.1265901696524986964, -0.4724409448818899238, -0.7020997375328084100 ) ) ;
#70598=CARTESIAN_POINT ( 'NONE',  ( 0.1958661417322836440, -0.3392501089628017219, -0.3989501312335957950 ) ) ;
#70599=CARTESIAN_POINT ( 'NONE',  ( 0.1049643490035304799, -0.3917322834645669549, -2.217191601049868677 ) ) ;
#70603=CARTESIAN_POINT ( 'NONE',  ( -0.2362204724409451284, 0.4091458600556402425, -2.767060367454068359 ) ) ;
#70607=CARTESIAN_POINT ( 'NONE',  ( 0.1058382717557500852, -0.3949938075777408852, -2.524278215223097366 ) ) ;
#70615=CARTESIAN_POINT ( 'NONE',  ( 0.1049643490035304938, -0.3917322834645669549, -1.652230971128608505 ) ) ;
#70618=CARTESIAN_POINT ( 'NONE',  ( -0.3458507752293909498, 0.3458507752293907833, 0.06102362204724409017 ) ) ;
#70630=CARTESIAN_POINT ( 'NONE',  ( -0.2925321140481930149, -0.2925321140481933480, -1.238188976377952999 ) ) ;
#70631=CARTESIAN_POINT ( 'NONE',  ( 0.3917322834645670104, -0.1049643490035303411, -2.558398950131233196 ) ) ;
#70642=CARTESIAN_POINT ( 'NONE',  ( 5.785732909357575061E-17, -0.4724409448818898682, -0.7086614173228346081 ) ) ;
#70643=CARTESIAN_POINT ( 'NONE',  ( -0.2867679344610365444, -0.2867679344610367664, -1.945557373524620992 ) ) ;
#70650=CARTESIAN_POINT ( 'NONE',  ( -0.1958661417322836718, 0.3392501089628017219, -2.145013123359580387 ) ) ;
#70658=CARTESIAN_POINT ( 'NONE',  ( 4.893765752498283924E-17, -0.3996062992125986035, -1.338582677165354173 ) ) ;
#70660=CARTESIAN_POINT ( 'NONE',  ( -0.3917322834645670104, -7.196005306013484475E-17, -2.866141732283464361 ) ) ;
#70675=CARTESIAN_POINT ( 'NONE',  ( -0.3917322834645671215, 0.1049643490035301469, -0.3398950131233596239 ) ) ;
#70678=CARTESIAN_POINT ( 'NONE',  ( 0.1974969037888704704, 0.3420746716998660508, -0.4593175853018373056 ) ) ;
#70688=CARTESIAN_POINT ( 'NONE',  ( -0.3392501089628017219, -0.1958661417322836995, -1.781515378773965042 ) ) ;
#70694=CARTESIAN_POINT ( 'NONE',  ( 4.893765752498283924E-17, -0.3996062992125986035, -1.338582677165354173 ) ) ;
#70696=CARTESIAN_POINT ( 'NONE',  ( -0.2925321140481932369, 0.2925321140481931259, -0.8838582677165351953 ) ) ;
#70697=CARTESIAN_POINT ( 'NONE',  ( -0.3996062992125985480, -7.340648628747423112E-17, -0.2736220472440945017 ) ) ;
#70699=CARTESIAN_POINT ( 'NONE',  ( 0.1070741851644053527, 0.3996062992125986590, -2.513123359580052174 ) ) ;
#70700=CARTESIAN_POINT ( 'NONE',  ( -0.3917322834645669549, -0.1049643490035306603, -1.547900262467191590 ) ) ;
#70707=CARTESIAN_POINT ( 'NONE',  ( -0.2362204724409447953, -0.4091458600556404646, -1.402230971128609172 ) ) ;
#70710=CARTESIAN_POINT ( 'NONE',  ( 0.1974969037888704704, 0.3420746716998660508, -0.8510498687664042050 ) ) ;
#70717=DIRECTION ( 'NONE',  ( 0.000000000000000000, 0.000000000000000000, 1.000000000000000000 ) ) ;
#70720=CARTESIAN_POINT ( 'NONE',  ( -9.787531504996566615E-17, 0.3996062992125985480, -2.124015748031496287 ) ) ;
#70722=( BOUNDED_CURVE ( )  B_SPLINE_CURVE ( 2, ( #38096, #11622, #31366, #74776, #82726, #30956, #76007, #49902, #29724, #56623, #69277, #70083, #25045 ),
 .UNSPECIFIED., .F., .F. ) 
 B_SPLINE_CURVE_WITH_KNOTS ( ( 3, 2, 2, 2, 2, 2, 3 ),
 ( 0.7625000000000000666, 0.7666666666666668295, 0.7708333333333334814, 0.7750000000000001332, 0.7791666666666667851, 0.7833333333333334370, 0.7875000000000000888 ),
 .UNSPECIFIED. ) 
 CURVE ( )  GEOMETRIC_REPRESENTATION_ITEM ( )  RATIONAL_B_SPLINE_CURVE ( ( 0.9999999999999991118, 0.9659258262890692004, 1.000000000000000000, 0.9659258262890683122, 1.000000000000000000, 0.9659258262890683122, 1.000000000000000000, 0.9659258262890683122, 1.000000000000000000, 0.9659258262890683122, 1.000000000000000000, 0.9659258262890674240, 1.000000000000000888 ) ) 
 REPRESENTATION_ITEM ( '' )  );
#70723=CARTESIAN_POINT ( 'NONE',  ( 0.3392501089628018329, -0.1958661417322834497, -1.759823203903200017 ) ) ;
#70738=CARTESIAN_POINT ( 'NONE',  ( 0.1958661417322836440, -0.3392501089628017219, -1.121391076115485719 ) ) ;
#70759=CARTESIAN_POINT ( 'NONE',  ( -0.3917322834645670104, -7.196005306013484475E-17, -2.551181102362204633 ) ) ;
#70764=CARTESIAN_POINT ( 'NONE',  ( 0.1265901696524989462, 0.4724409448818897572, -0.9383202099737533164 ) ) ;
#70765=CARTESIAN_POINT ( 'NONE',  ( 0.3996062992125986035, 0.1070741851644054776, -0.1246719160104987068 ) ) ;
#70768=CARTESIAN_POINT ( 'NONE',  ( -0.3917322834645669549, -0.1049643490035306603, -1.770341207349081181 ) ) ;
#70772=CARTESIAN_POINT ( 'NONE',  ( 0.4091458600556403535, 0.2362204724409449896, -2.808398950131233640 ) ) ;
#70779=CARTESIAN_POINT ( 'NONE',  ( 0.3392501089628018329, -0.1958661417322834497, -1.129901944060680563 ) ) ;
#70786=CARTESIAN_POINT ( 'NONE',  ( -0.3392501089628019995, 0.1958661417322831999, -2.542670234417010011 ) ) ;
#70794=CARTESIAN_POINT ( 'NONE',  ( 0.1049643490035303689, 0.3917322834645670104, -1.495406824146981117 ) ) ;
#70812=CARTESIAN_POINT ( 'NONE',  ( 0.4724409448818898682, 2.892866454678787531E-17, -0.03740157480314962313 ) ) ;
#70816=CARTESIAN_POINT ( 'NONE',  ( 0.3460692066303959202, -0.1998031496062991630, -2.701443569553806157 ) ) ;
#70823=CARTESIAN_POINT ( 'NONE',  ( -0.3949938075777411073, 0.1058382717557497660, -0.2670603674540682482 ) ) ;
#70830=CARTESIAN_POINT ( 'NONE',  ( 0.2925321140481932369, -0.2925321140481931814, -0.8051181102362205966 ) ) ;
#70832=CARTESIAN_POINT ( 'NONE',  ( 0.2867679344610365999, -0.2867679344610365444, -0.5629921259842519676 ) ) ;
#70847=CARTESIAN_POINT ( 'NONE',  ( -0.4724409448818895907, -0.1265901696524993070, -2.642388451443570041 ) ) ;
#70851=DIRECTION ( 'NONE',  ( 1.000000000000000000, 0.000000000000000000, 0.000000000000000000 ) ) ;
#70865=CARTESIAN_POINT ( 'NONE',  ( 0.2925321140481932369, -0.2925321140481931814, -0.4133858267716534196 ) ) ;
#70866=CARTESIAN_POINT ( 'NONE',  ( 0.3996062992125985480, 2.446882876249141654E-17, -2.872047244094488416 ) ) ;
#70869=VECTOR ( 'NONE', #59831, 39.37007874015748143 ) ;
#70872=CARTESIAN_POINT ( 'NONE',  ( -0.2925321140481932924, 0.2925321140481931814, -2.381889763779527325 ) ) ;
#70873=CARTESIAN_POINT ( 'NONE',  ( -0.2891555358219911054, 0.2891555358219909388, -1.909448818897637956 ) ) ;
#70874=CARTESIAN_POINT ( 'NONE',  ( -0.2867679344610364334, -0.2867679344610367109, -0.3661417322834645827 ) ) ;
#70876=CARTESIAN_POINT ( 'NONE',  ( 0.3917322834645670104, -0.1049643490035303273, -1.048556430446194287 ) ) ;
#70879=CARTESIAN_POINT ( 'NONE',  ( -0.1049643490035306742, 0.3917322834645668994, 0.2283657724747524265 ) ) ;
#70883=CARTESIAN_POINT ( 'NONE',  ( -0.2362204724409447953, -0.4091458600556404646, -2.742782152230971437 ) ) ;
#70884=CARTESIAN_POINT ( 'NONE',  ( 0.3996062992125986035, 0.1070741851644054776, -2.644356955380577912 ) ) ;
#70885=CARTESIAN_POINT ( 'NONE',  ( -0.1049643490035302301, -0.3917322834645671770, -1.328759473262154378 ) ) ;
#70891=CARTESIAN_POINT ( 'NONE',  ( -9.594673741351313045E-17, 0.3917322834645670104, 0.07283464566929125084 ) ) ;
#70899=CARTESIAN_POINT ( 'NONE',  ( -0.1958661417322834220, -0.3392501089628018884, -0.7801837270341208663 ) ) ;
#70900=CARTESIAN_POINT ( 'NONE',  ( -0.3917322834645670104, -7.196005306013484475E-17, -2.078740157480314821 ) ) ;
#70901=CARTESIAN_POINT ( 'NONE',  ( 0.3392501089628018884, -0.1958661417322834220, -2.616797900262466836 ) ) ;
#70903=CARTESIAN_POINT ( 'NONE',  ( 0.2925321140481932369, -0.2925321140481932369, 0.05905511811023619884 ) ) ;
#70906=CARTESIAN_POINT ( 'NONE',  ( 0.2925321140481932369, -0.2925321140481932369, -1.515748031496062742 ) ) ;
#70911=CARTESIAN_POINT ( 'NONE',  ( 0.3917322834645670104, 2.398668435337828261E-17, -0.6751968503937009203 ) ) ;
#70921=CARTESIAN_POINT ( 'NONE',  ( 0.4724409448818897572, -0.1265901696524988906, -2.001312335958005395 ) ) ;
#70925=CARTESIAN_POINT ( 'NONE',  ( 0.4724409448818898682, 0.000000000000000000, -2.755905511811024056 ) ) ;
#70929=CARTESIAN_POINT ( 'NONE',  ( -0.1265901696524986964, -0.4724409448818899238, -2.511154855643044748 ) ) ;
#70933=CARTESIAN_POINT ( 'NONE',  ( 0.3917322834645669549, 2.398668435337827645E-17, -0.8280646737194732321 ) ) ;
#70941=CARTESIAN_POINT ( 'NONE',  ( 0.2867679344610365999, -0.2867679344610365444, -2.610236220472441193 ) ) ;
#70944=CARTESIAN_POINT ( 'NONE',  ( 0.4724409448818898682, 2.892866454678787531E-17, -1.297244094488188670 ) ) ;
#70956=CARTESIAN_POINT ( 'NONE',  ( 0.1070741851644053388, 0.3996062992125986035, -2.432414698162729039 ) ) ;
#70960=CARTESIAN_POINT ( 'NONE',  ( -0.3460692066303957537, -0.1998031496062994405, -1.389107611548556553 ) ) ;
#70966=CARTESIAN_POINT ( 'NONE',  ( 4.893765752498283308E-17, -0.3996062992125985480, -0.4704724409448819422 ) ) ;
#70967=CARTESIAN_POINT ( 'NONE',  ( -9.787531504996567848E-17, 0.3996062992125986035, -0.9448818897637796255 ) ) ;
#70968=CARTESIAN_POINT ( 'NONE',  ( 0.3949938075777409963, 2.418639510665530435E-17, -0.7480314960629920185 ) ) ;
#70974=CARTESIAN_POINT ( 'NONE',  ( -9.674558042662122972E-17, 0.3949938075777409963, -1.336614173228346081 ) ) ;
#70979=CARTESIAN_POINT ( 'NONE',  ( -0.4724409448818899238, 0.1265901696524986686, -1.450131233595800317 ) ) ;
#70988=CARTESIAN_POINT ( 'NONE',  ( 0.1958661417322834497, 0.3392501089628018329, -1.799193282643357428 ) ) ;
#70995=CARTESIAN_POINT ( 'NONE',  ( -0.2867679344610365999, 0.2867679344610364889, -1.271653543307086798 ) ) ;
#70998=CARTESIAN_POINT ( 'NONE',  ( -0.3949938075777411628, 0.1058382717557497937, -2.080052493438320216 ) ) ;
#71003=CARTESIAN_POINT ( 'NONE',  ( -0.2925321140481932924, 0.2925321140481931814, -0.3346456692913385988 ) ) ;
#71007=CARTESIAN_POINT ( 'NONE',  ( -0.1049643490035307020, 0.3917322834645669549, 0.2237532808398949025 ) ) ;
#71010=CARTESIAN_POINT ( 'NONE',  ( -0.3917322834645671215, 0.1049643490035301469, -0.2749343832020998413 ) ) ;
#71016=ORIENTED_EDGE ( 'NONE', *, *, #14771, .T. ) ;
#71017=CARTESIAN_POINT ( 'NONE',  ( 0.1998031496062992463, 0.3460692066303959202, -2.110892388451443225 ) ) ;
#71022=CARTESIAN_POINT ( 'NONE',  ( -0.1265901696524986964, -0.4724409448818899238, -1.017060367454067915 ) ) ;
#71024=CARTESIAN_POINT ( 'NONE',  ( -0.1958661417322834220, -0.3392501089628018884, -0.2152230971128608339 ) ) ;
#71025=CARTESIAN_POINT ( 'NONE',  ( 0.3917322834645670104, -0.04642319063763879206, -1.932137297949608978 ) ) ;
#71029=CARTESIAN_POINT ( 'NONE',  ( -1.157146581871515012E-16, 0.4724409448818898682, -2.753937007874015741 ) ) ;
#71034=CARTESIAN_POINT ( 'NONE',  ( -9.674558042662122972E-17, 0.3949938075777409963, -2.753937007874016185 ) ) ;
#71042=CARTESIAN_POINT ( 'NONE',  ( 4.797336870675656522E-17, -0.3917322834645670104, -1.488188976377952777 ) ) ;
#71046=CARTESIAN_POINT ( 'NONE',  ( 0.2362204724409451007, -0.4091458600556402980, -0.01115485564304462100 ) ) ;
#71058=CARTESIAN_POINT ( 'NONE',  ( 0.3460692066303959202, -0.1998031496062991630, -1.126640419947506633 ) ) ;
#71059=CARTESIAN_POINT ( 'NONE',  ( 0.1049643490035304938, -0.3917322834645669549, -2.689632545931758489 ) ) ;
#71070=CARTESIAN_POINT ( 'NONE',  ( -0.1958661417322836995, 0.3392501089628017219, -2.057105929955067580 ) ) ;
#71077=CARTESIAN_POINT ( 'NONE',  ( -0.1958661417322836718, 0.3392501089628017219, -1.830052493438320216 ) ) ;
#71084=CARTESIAN_POINT ( 'NONE',  ( -0.2925321140481932924, 0.2925321140481931814, -1.279527559055118058 ) ) ;
#71086=CARTESIAN_POINT ( 'NONE',  ( 0.2867679344610366554, -0.2867679344610365999, -0.09516367273721974829 ) ) ;
#71099=CARTESIAN_POINT ( 'NONE',  ( -0.3392501089628017219, -0.1958661417322836718, -0.2020997375328083545 ) ) ;
#71102=CARTESIAN_POINT ( 'NONE',  ( 0.3420746716998660508, -0.1974969037888703871, -0.7349081364829396223 ) ) ;
#71105=DIRECTION ( 'NONE',  ( 1.000000000000000000, 0.000000000000000000, 0.000000000000000000 ) ) ;
#71109=CARTESIAN_POINT ( 'NONE',  ( 0.1958661417322836718, -0.3392501089628017219, -1.820885457514122452 ) ) ;
#71115=CARTESIAN_POINT ( 'NONE',  ( 0.3996062992125986035, 2.446882876249141962E-17, -1.377952755905511806 ) ) ;
#71117=CARTESIAN_POINT ( 'NONE',  ( -9.787531504996566615E-17, 0.3996062992125985480, -0.8641732283464567121 ) ) ;
#71118=CARTESIAN_POINT ( 'NONE',  ( -0.3996062992125984925, -0.1070741851644056858, 0.03477690288713908284 ) ) ;
#71120=CARTESIAN_POINT ( 'NONE',  ( -0.3996062992125986035, -7.340648628747425578E-17, -2.559055118110236560 ) ) ;
#71121=CARTESIAN_POINT ( 'NONE',  ( 0.1049643490035303689, 0.3917322834645670104, -1.967847769028871374 ) ) ;
#71127=CARTESIAN_POINT ( 'NONE',  ( -0.4091458600556402980, -0.2362204724409451284, -1.389107611548556553 ) ) ;
#71130=CARTESIAN_POINT ( 'NONE',  ( -0.1974969037888704149, -0.3420746716998661063, -1.244750656167979086 ) ) ;
#71141=CARTESIAN_POINT ( 'NONE',  ( 0.1070741851644054776, -0.3996062992125984925, -2.051837270341207109 ) ) ;
#71143=EDGE_CURVE ( 'NONE', #82700, #13953, #77805, .T. ) ;
#71144=CARTESIAN_POINT ( 'NONE',  ( 0.2867679344610365999, 0.2867679344610365999, -1.950111917813961426 ) ) ;
#71153=CARTESIAN_POINT ( 'NONE',  ( -0.4091458600556405756, 0.2362204724409446288, -2.388451443569553856 ) ) ;
#71159=CARTESIAN_POINT ( 'NONE',  ( -0.1049643490035302024, -0.3917322834645671215, -1.416666666666666519 ) ) ;
#71168=CARTESIAN_POINT ( 'NONE',  ( 0.000000000000000000, 0.000000000000000000, -2.755905511811024056 ) ) ;
#71179=CARTESIAN_POINT ( 'NONE',  ( 0.3392501089628018329, 0.1958661417322835607, -2.643044619422571628 ) ) ;
#71182=CARTESIAN_POINT ( 'NONE',  ( -1.157146581871515012E-16, 0.4724409448818898682, -0.7874015748031496509 ) ) ;
#71183=CARTESIAN_POINT ( 'NONE',  ( 0.1070741851644053527, 0.3996062992125986590, -0.1509186351706036655 ) ) ;
#71186=CARTESIAN_POINT ( 'NONE',  ( -0.3917322834645671215, 0.1049643490035301469, -1.914698162729658648 ) ) ;
#71187=EDGE_LOOP ( 'NONE', ( #6180, #66437, #65087, #16245 ) ) ;
#71190=CARTESIAN_POINT ( 'NONE',  ( 0.4724409448818897572, -0.1265901696524988906, -2.788713910761154047 ) ) ;
#71197=CARTESIAN_POINT ( 'NONE',  ( 0.3392501089628018329, -0.1958661417322834497, -1.287382259021310427 ) ) ;
#71204=CARTESIAN_POINT ( 'NONE',  ( -0.3917322834645670104, -0.1049643490035307020, -2.562355273787088716 ) ) ;
#71212=CARTESIAN_POINT ( 'NONE',  ( 0.3392501089628018329, 0.1958661417322835607, -1.948162729658792891 ) ) ;
#71216=CARTESIAN_POINT ( 'NONE',  ( -0.08106202739150959735, 0.3841287887292361702, -8.192289201020256726E-18 ) ) ;
#71224=VERTEX_POINT ( 'NONE', #48684 ) ;
#71230=CARTESIAN_POINT ( 'NONE',  ( -0.4724409448818899238, 0.1265901696524986686, -0.4245406824146981672 ) ) ;
#71233=CARTESIAN_POINT ( 'NONE',  ( 0.3949938075777409408, -0.1058382717557499186, -0.3458005249343832910 ) ) ;
#71238=CARTESIAN_POINT ( 'NONE',  ( -0.3949938075777408852, -0.1058382717557502933, -0.1227034120734908501 ) ) ;
#71245=CARTESIAN_POINT ( 'NONE',  ( -0.3996062992125984925, -0.1070741851644056858, -0.9101049868766404316 ) ) ;
#71247=CARTESIAN_POINT ( 'NONE',  ( 0.3917322834645669549, 0.1049643490035304660, -0.7467191601049868455 ) ) ;
#71262=CARTESIAN_POINT ( 'NONE',  ( 0.3458507752293908943, 0.3458507752293908943, -2.576771653543307394 ) ) ;
#71277=CARTESIAN_POINT ( 'NONE',  ( 4.893765752498283924E-17, -0.3996062992125986035, -0.5511811023622047445 ) ) ;
#71283=CARTESIAN_POINT ( 'NONE',  ( 0.3996062992125986035, 2.446882876249141962E-17, -2.637795275590551380 ) ) ;
#71284=CARTESIAN_POINT ( 'NONE',  ( 4.837279021331060870E-17, -0.3949938075777409963, -1.811023622047243986 ) ) ;
#71285=CARTESIAN_POINT ( 'NONE',  ( 0.1049643490035303689, 0.3917322834645670104, -0.4580052493438320216 ) ) ;
#71287=CARTESIAN_POINT ( 'NONE',  ( -0.1049643490035307020, 0.3917322834645669549, -1.101049868766404094 ) ) ;
#71290=CARTESIAN_POINT ( 'NONE',  ( -0.3917322834645669549, -0.1049643490035306603, -0.9829396325459317518 ) ) ;
#71292=CARTESIAN_POINT ( 'NONE',  ( -0.1058382717557497660, -0.3949938075777411073, -2.826115485564304475 ) ) ;
#71298=CARTESIAN_POINT ( 'NONE',  ( -0.2925321140481932924, 0.2925321140481931814, -2.696850393700787052 ) ) ;
#71299=CARTESIAN_POINT ( 'NONE',  ( 0.1958661417322836718, -0.3392501089628017219, -1.033483882710973134 ) ) ;
#71305=CARTESIAN_POINT ( 'NONE',  ( -0.2867679344610365999, 0.2867679344610364889, -0.7342519685039372579 ) ) ;
#71313=CARTESIAN_POINT ( 'NONE',  ( 0.03611438844186872638, -0.3902087894126607392, -1.929133858267717105 ) ) ;
#71314=CARTESIAN_POINT ( 'NONE',  ( 0.3392501089628018884, -0.1958661417322834220, -1.986876640419947604 ) ) ;
#71317=CARTESIAN_POINT ( 'NONE',  ( 0.1998031496062994405, -0.3460692066303958092, 0.06561679790026245240 ) ) ;
#71321=CARTESIAN_POINT ( 'NONE',  ( -1.157146581871515012E-16, 0.4724409448818898682, -2.438976377952756014 ) ) ;
#71323=CARTESIAN_POINT ( 'NONE',  ( -0.4091458600556402980, -0.2362204724409451284, -1.154855643044619518 ) ) ;
#71324=CARTESIAN_POINT ( 'NONE',  ( -0.3392501089628019995, 0.1958661417322832277, -0.8982939632545933195 ) ) ;
#71325=EDGE_CURVE ( 'NONE', #36386, #18415, #54164, .T. ) ;
#71334=CARTESIAN_POINT ( 'NONE',  ( -0.2362204724409451284, 0.4091458600556402425, -2.690288713910760965 ) ) ;
#71340=CARTESIAN_POINT ( 'NONE',  ( 0.2362204724409451007, -0.4091458600556402980, -2.530839895013123453 ) ) ;
#71344=CARTESIAN_POINT ( 'NONE',  ( -0.3917322834645670659, 0.1049643490035301607, -0.9002431514097621879 ) ) ;
#71354=CARTESIAN_POINT ( 'NONE',  ( -0.3917322834645671770, 0.1049643490035302024, -0.02954687483695727160 ) ) ;
#71357=CARTESIAN_POINT ( 'NONE',  ( 0.2362204724409451007, -0.4091458600556402980, -1.270997375328083878 ) ) ;
#71371=CARTESIAN_POINT ( 'NONE',  ( -0.1070741851644056997, 0.3996062992125984925, -2.603018372703412631 ) ) ;
#71375=CARTESIAN_POINT ( 'NONE',  ( 0.1998031496062992463, 0.3460692066303959202, -1.638451443569554078 ) ) ;
#71381=CARTESIAN_POINT ( 'NONE',  ( 0.2925321140481931814, -0.2925321140481931259, -0.9625984251968502381 ) ) ;
#71383=CARTESIAN_POINT ( 'NONE',  ( -0.1998031496062991907, -0.3460692066303959757, -1.167979002624671914 ) ) ;
#71384=CARTESIAN_POINT ( 'NONE',  ( -9.674558042662121740E-17, 0.3949938075777409963, -0.6299212598425196763 ) ) ;
#71390=CARTESIAN_POINT ( 'NONE',  ( 0.1974969037888704704, 0.3420746716998660508, -1.795931758530183942 ) ) ;
#71395=CARTESIAN_POINT ( 'NONE',  ( -0.4724409448818899238, 0.1265901696524986686, -1.765091863517059823 ) ) ;
#71396=CARTESIAN_POINT ( 'NONE',  ( 0.09156050430091122738, 0.3808816823641256732, -2.755905511811024056 ) ) ;
#71404=CARTESIAN_POINT ( 'NONE',  ( -0.3392501089628019439, 0.1958661417322832554, -2.153523991304775009 ) ) ;
#71411=CARTESIAN_POINT ( 'NONE',  ( -0.1958661417322836718, 0.3392501089628017219, 0.05971128608923875758 ) ) ;
#71413=CARTESIAN_POINT ( 'NONE',  ( -0.3917322834645670104, -7.196005306013484475E-17, -1.606299212598425452 ) ) ;
#71416=CARTESIAN_POINT ( 'NONE',  ( -0.3949938075777409408, -0.1058382717557502933, -1.778215223097113107 ) ) ;
#71421=CARTESIAN_POINT ( 'NONE',  ( 0.2925321140481932369, 0.2925321140481932369, -0.4527559055118109965 ) ) ;
#71428=CARTESIAN_POINT ( 'NONE',  ( 0.2867679344610365999, -0.2867679344610365444, -0.1830708661417323746 ) ) ;
#71435=CARTESIAN_POINT ( 'NONE',  ( -0.1070741851644056997, 0.3996062992125984925, -1.973097112860892510 ) ) ;
#71439=CARTESIAN_POINT ( 'NONE',  ( 0.3458507752293908943, 0.3458507752293908943, -0.7677165354330709457 ) ) ;
#71441=CARTESIAN_POINT ( 'NONE',  ( -0.1049643490035307020, 0.3917322834645669549, -0.4711286089238844177 ) ) ;
#71442=CARTESIAN_POINT ( 'NONE',  ( 0.3917322834645670104, 2.398668435337828261E-17, -1.935039370078740273 ) ) ;
#71446=CARTESIAN_POINT ( 'NONE',  ( -0.3996062992125984925, -0.1070741851644056858, 0.1922572178477689464 ) ) ;
#71451=CARTESIAN_POINT ( 'NONE',  ( -0.3420746716998660508, -0.1974969037888706924, -2.491469816272965598 ) ) ;
#71453=CARTESIAN_POINT ( 'NONE',  ( 0.2867679344610366554, 0.2867679344610366554, -0.06496062992125993529 ) ) ;
#71460=CARTESIAN_POINT ( 'NONE',  ( -0.1958661417322834220, -0.3392501089628018884, -1.632545931758530244 ) ) ;
#71463=CARTESIAN_POINT ( 'NONE',  ( 0.1265901696524990294, -0.4724409448818896462, 0.1528871391076115360 ) ) ;
#71476=CARTESIAN_POINT ( 'NONE',  ( 0.3996062992125986035, -0.1070741851644052972, -1.290682414698162583 ) ) ;
#71478=CARTESIAN_POINT ( 'NONE',  ( 0.2867679344610365999, -0.2867679344610365444, -2.860236220472440749 ) ) ;
#71487=CARTESIAN_POINT ( 'NONE',  ( 4.893765752498283924E-17, -0.3996062992125986035, 0.07874015748031494566 ) ) ;
#71488=CARTESIAN_POINT ( 'NONE',  ( -0.1049643490035307158, 0.3917322834645670104, -2.522985195046931306 ) ) ;
#71489=ORIENTED_EDGE ( 'NONE', *, *, #13980, .F. ) ;
#71494=CARTESIAN_POINT ( 'NONE',  ( 0.3392501089628018884, -0.1958661417322834220, -2.236876640419947826 ) ) ;
#71501=CARTESIAN_POINT ( 'NONE',  ( -0.3460692066303958092, -0.1998031496062994683, -1.312335958005249381 ) ) ;
#71503=CARTESIAN_POINT ( 'NONE',  ( -0.1049643490035302301, -0.3917322834645671770, 0.08856336138351518505 ) ) ;
#71516=CARTESIAN_POINT ( 'NONE',  ( 0.1958661417322836440, -0.3392501089628017219, -0.3989501312335957950 ) ) ;
#71519=CARTESIAN_POINT ( 'NONE',  ( -0.3949938075777409408, -0.1058382717557502933, -0.5183727034120736432 ) ) ;
#71528=CARTESIAN_POINT ( 'NONE',  ( 0.000000000000000000, 0.000000000000000000, -2.755905511811024056 ) ) ;
#71533=CARTESIAN_POINT ( 'NONE',  ( -0.3996062992125987146, 0.1070741851644051862, -1.450131233595800317 ) ) ;
#71535=CARTESIAN_POINT ( 'NONE',  ( 0.3996062992125985480, 2.446882876249141654E-17, -0.6673228346456693272 ) ) ;
#71536=CARTESIAN_POINT ( 'NONE',  ( -0.3460692066303957537, -0.1998031496062994405, 0.02821522309711283621 ) ) ;
#71538=CARTESIAN_POINT ( 'NONE',  ( -0.3996062992125986035, -0.1070741851644056997, -2.723097112860892288 ) ) ;
#71540=CARTESIAN_POINT ( 'NONE',  ( -0.3917322834645670104, -7.196005306013484475E-17, -2.171259842519685179 ) ) ;
#71546=CARTESIAN_POINT ( 'NONE',  ( -0.1265901696524986964, -0.4724409448818899238, -1.408792650918635259 ) ) ;
#71549=CARTESIAN_POINT ( 'NONE',  ( 0.3949938075777409408, -0.1058382717557499186, -1.448162729658792669 ) ) ;
#71559=CARTESIAN_POINT ( 'NONE',  ( -0.1070741851644056997, 0.3996062992125984925, -2.288057742782152459 ) ) ;
#71561=CARTESIAN_POINT ( 'NONE',  ( -0.3392501089628019439, 0.1958661417322832554, -1.996043676344145146 ) ) ;
#71573=CARTESIAN_POINT ( 'NONE',  ( -0.1070741851644056997, 0.3996062992125984925, -0.08333333333333335646 ) ) ;
#71575=CARTESIAN_POINT ( 'NONE',  ( -0.3917322834645671215, 0.1049643490035301469, -1.219816272965879023 ) ) ;
#71596=CARTESIAN_POINT ( 'NONE',  ( -0.1049643490035307020, 0.3917322834645669549, -2.360892388451443669 ) ) ;
#71599=CARTESIAN_POINT ( 'NONE',  ( -0.1265901696524986964, -0.4724409448818899238, -0.8595800524934383846 ) ) ;
#71600=CARTESIAN_POINT ( 'NONE',  ( -0.1998031496062991907, -0.3460692066303959757, 0.09186351706036742504 ) ) ;
#71603=CARTESIAN_POINT ( 'NONE',  ( -0.1958661417322834220, -0.3392501089628018884, -1.947506561679789971 ) ) ;
#71615=CARTESIAN_POINT ( 'NONE',  ( 0.1958661417322836162, -0.3392501089628018329, -1.116778584480628389 ) ) ;
#71621=CARTESIAN_POINT ( 'NONE',  ( -0.2867679344610367109, 0.2867679344610365444, -2.378628239666354283 ) ) ;
#71630=CARTESIAN_POINT ( 'NONE',  ( -0.3917322834645670104, -7.196005306013484475E-17, -1.856299212598425230 ) ) ;
#71646=CARTESIAN_POINT ( 'NONE',  ( 0.2362204724409449064, 0.4091458600556404646, -0.2211286089238845010 ) ) ;
#71649=CARTESIAN_POINT ( 'NONE',  ( 0.1058382717557499880, 0.3949938075777409408, -0.07020997375328083545 ) ) ;
#71654=CARTESIAN_POINT ( 'NONE',  ( 0.1974969037888706092, -0.3420746716998660508, -0.1686351706036745279 ) ) ;
#71662=CARTESIAN_POINT ( 'NONE',  ( 0.1070741851644054776, -0.3996062992125984925, -0.7919947506561679784 ) ) ;
#71664=CARTESIAN_POINT ( 'NONE',  ( -0.3392501089628019995, 0.1958661417322832277, -0.6482939632545930975 ) ) ;
#71679=CARTESIAN_POINT ( 'NONE',  ( 0.3996062992125984925, 0.1070741851644054637, 0.1135170603674540285 ) ) ;
#71696=CARTESIAN_POINT ( 'NONE',  ( 0.3460692066303959202, 0.1998031496062993295, -0.9186351706036745002 ) ) ;
#71701=CARTESIAN_POINT ( 'NONE',  ( -0.3996062992125986035, -7.340648628747425578E-17, -2.559055118110236560 ) ) ;
#71702=CARTESIAN_POINT ( 'NONE',  ( 4.837279021331060870E-17, -0.3949938075777409963, -2.125984251968503713 ) ) ;
#71703=CARTESIAN_POINT ( 'NONE',  ( 0.2867679344610365999, 0.2867679344610365999, -0.4448818897637794589 ) ) ;
#71705=CARTESIAN_POINT ( 'NONE',  ( -0.1958661417322834220, -0.3392501089628018884, -1.002624671916010568 ) ) ;
#71707=CARTESIAN_POINT ( 'NONE',  ( 0.3392501089628018329, 0.1958661417322835607, -1.225721784776902634 ) ) ;
#71709=CARTESIAN_POINT ( 'NONE',  ( -0.3917322834645669549, -7.196005306013483243E-17, 0.03807705856399132283 ) ) ;
#71714=CARTESIAN_POINT ( 'NONE',  ( -0.3458507752293909498, 0.3458507752293908388, -0.09645669291338582196 ) ) ;
#71715=CARTESIAN_POINT ( 'NONE',  ( -0.2925321140481930704, -0.2925321140481933480, -2.736220472440944018 ) ) ;
#71716=CARTESIAN_POINT ( 'NONE',  ( 0.3392501089628018329, 0.1958661417322835607, -1.230334276411760186 ) ) ;
#71722=CARTESIAN_POINT ( 'NONE',  ( 0.2867679344610365999, -0.2867679344610365444, -0.4980314960629922405 ) ) ;
#71731=CARTESIAN_POINT ( 'NONE',  ( 0.3692639355350713637, -0.1324727617106734590, -1.929133858267717549 ) ) ;
#71732=CARTESIAN_POINT ( 'NONE',  ( 0.3917322834645670104, 2.398668435337828261E-17, -1.842519685039370136 ) ) ;
#71734=CARTESIAN_POINT ( 'NONE',  ( -0.3996062992125987146, 0.1070741851644051862, 0.1246719160104986790 ) ) ;
#71741=CARTESIAN_POINT ( 'NONE',  ( 0.3392501089628018884, -0.1958661417322834220, -0.9770341207349081403 ) ) ;
#71762=CARTESIAN_POINT ( 'NONE',  ( 0.1049643490035304522, -0.3917322834645668994, -0.9527365897299718833 ) ) ;
#71772=CARTESIAN_POINT ( 'NONE',  ( -0.3917322834645670659, -7.196005306013484475E-17, -0.1935888695876134269 ) ) ;
#71775=CARTESIAN_POINT ( 'NONE',  ( -0.4091458600556405756, 0.2362204724409446288, -1.362860892388451539 ) ) ;
#71792=CARTESIAN_POINT ( 'NONE',  ( -0.1070741851644051862, -0.3996062992125986590, -2.353674540682414218 ) ) ;
#71796=CARTESIAN_POINT ( 'NONE',  ( 0.1070741851644053388, 0.3996062992125986035, -1.802493438320210029 ) ) ;
#71802=CARTESIAN_POINT ( 'NONE',  ( -0.1998031496062994405, 0.3460692066303957537, -1.192257217847769057 ) ) ;
#71803=CARTESIAN_POINT ( 'NONE',  ( -0.3996062992125986035, -7.340648628747425578E-17, -1.456692913385826849 ) ) ;
#71806=CARTESIAN_POINT ( 'NONE',  ( -0.3420746716998659953, -0.1974969037888706647, -0.8398950131233596794 ) ) ;
#71812=CARTESIAN_POINT ( 'NONE',  ( -0.3949938075777411073, 0.1058382717557497660, -1.684383202099737575 ) ) ;
#71814=EDGE_CURVE ( 'NONE', #35562, #70572, #21801, .T. ) ;
#71818=CARTESIAN_POINT ( 'NONE',  ( -0.4091458600556402980, -0.2362204724409451284, -2.099737532808398921 ) ) ;
#71819=CARTESIAN_POINT ( 'NONE',  ( 0.3622863298689343314, -0.1504864506494317244, -2.755905511811024056 ) ) ;
#71825=CARTESIAN_POINT ( 'NONE',  ( 0.3917322834645668994, -0.1049643490035303134, -2.396306143535746447 ) ) ;
#71831=B_SPLINE_CURVE_WITH_KNOTS ( 'NONE', 3,
 ( #60207, #2137, #47149, #65288, #7626, #47566, #72840, #15189, #40846, #9285, #2969, #28215, #53874, #34956, #60619, #24681, #63400, #44431 ),
 .UNSPECIFIED., .F., .F.,
 ( 4, 2, 2, 2, 2, 2, 2, 2, 4 ),
 ( 0.000000000000000000, 2.503579457910189637E-05, 5.007158915820379274E-05, 0.0001001431783164055797, 0.0002002863566328091536, 0.0004005727132656153257, 0.0008011454265312270735, 0.001602290853062450461, 0.003204581706124896151 ),
 .UNSPECIFIED. ) ;
#71832=CARTESIAN_POINT ( 'NONE',  ( 0.3917322834645668994, 0.1049643490035304522, -2.724390133037059236 ) ) ;
#71834=CARTESIAN_POINT ( 'NONE',  ( 0.3392501089628018329, 0.1958661417322835607, -2.013123359580052618 ) ) ;
#71837=CARTESIAN_POINT ( 'NONE',  ( 0.1058382717557499880, 0.3949938075777411073, -2.040682414698163250 ) ) ;
#71842=CARTESIAN_POINT ( 'NONE',  ( -0.2925321140481932924, 0.2925321140481931814, -0.4921259842519684624 ) ) ;
#71850=CARTESIAN_POINT ( 'NONE',  ( 0.2867679344610365999, 0.2867679344610365999, -0.3799212598425197318 ) ) ;
#71861=CARTESIAN_POINT ( 'NONE',  ( -0.2362204724409447953, -0.4091458600556404646, -1.167979002624671914 ) ) ;
#71863=CARTESIAN_POINT ( 'NONE',  ( 0.2867679344610365999, 0.2867679344610365999, -0.1299212598425196485 ) ) ;
#71864=CARTESIAN_POINT ( 'NONE',  ( 0.3917322834645670104, -0.1049643490035303273, -2.243438320209973913 ) ) ;
#71868=CARTESIAN_POINT ( 'NONE',  ( 0.1070741851644054776, -0.3996062992125984925, -0.004593175853018396058 ) ) ;
#71870=EDGE_CURVE ( 'NONE', #21240, #37037, #37721, .T. ) ;
#71874=CARTESIAN_POINT ( 'NONE',  ( -0.3420746716998662729, 0.1974969037888702206, -2.465223097112861250 ) ) ;
#71876=DIRECTION ( 'NONE',  ( 0.000000000000000000, 0.000000000000000000, 1.000000000000000000 ) ) ;
#71881=CARTESIAN_POINT ( 'NONE',  ( 0.2867679344610365999, -0.2867679344610365444, -1.980314960629921073 ) ) ;
#71884=CARTESIAN_POINT ( 'NONE',  ( 0.4091458600556403535, 0.2362204724409449896, -0.05052493438320210251 ) ) ;
#71888=CARTESIAN_POINT ( 'NONE',  ( -0.4724409448818899238, 0.1265901696524986964, -0.7395013123359578389 ) ) ;
#71897=CARTESIAN_POINT ( 'NONE',  ( 0.3460692066303958092, 0.1998031496062993018, -1.310367454068241511 ) ) ;
#71898=CARTESIAN_POINT ( 'NONE',  ( -0.2867679344610364334, -0.2867679344610367109, -2.663385826771653253 ) ) ;
#71908=CARTESIAN_POINT ( 'NONE',  ( 0.2925321140481932369, -0.2925321140481932369, -0.09842519685039373412 ) ) ;
#71909=CARTESIAN_POINT ( 'NONE',  ( 4.797336870675656522E-17, -0.3917322834645670659, -2.437683357776589510 ) ) ;
#71916=CARTESIAN_POINT ( 'NONE',  ( -0.3392501089628019995, 0.1958661417322832277, -2.315616797900262647 ) ) ;
#71921=CARTESIAN_POINT ( 'NONE',  ( 0.2925321140481932369, 0.2925321140481932369, -2.027559055118109743 ) ) ;
#71923=CARTESIAN_POINT ( 'NONE',  ( -0.3996062992125986035, -7.340648628747425578E-17, -1.456692913385826849 ) ) ;
#71924=ORIENTED_EDGE ( 'NONE', *, *, #76134, .T. ) ;
#71925=VECTOR ( 'NONE', #55369, 39.37007874015748143 ) ;
#71926=CARTESIAN_POINT ( 'NONE',  ( 0.3392501089628018884, -0.1958661417322833942, 0.05575496243338393110 ) ) ;
#71927=ORIENTED_EDGE ( 'NONE', *, *, #44019, .F. ) ;
#71937=CARTESIAN_POINT ( 'NONE',  ( -0.3392501089628019995, 0.1958661417322832277, -0.4908136482939632339 ) ) ;
#71939=ORIENTED_EDGE ( 'NONE', *, *, #76134, .F. ) ;
#71940=CARTESIAN_POINT ( 'NONE',  ( -9.674558042662121740E-17, 0.3949938075777409963, -0.7874015748031496509 ) ) ;
#71955=CARTESIAN_POINT ( 'NONE',  ( -0.2925321140481932924, 0.2925321140481931814, -1.437007874015747921 ) ) ;
#71957=CARTESIAN_POINT ( 'NONE',  ( 0.1998031496062992463, 0.3460692066303959202, -0.8510498687664042050 ) ) ;
#71958=CARTESIAN_POINT ( 'NONE',  ( -0.1998031496062994405, 0.3460692066303957537, -0.4048556430446194621 ) ) ;
#71960=CARTESIAN_POINT ( 'NONE',  ( -0.3458507752293906723, -0.3458507752293910609, -0.2165354330708661734 ) ) ;
#71961=CARTESIAN_POINT ( 'NONE',  ( 4.797336870675656522E-17, -0.3917322834645670104, -2.053149606299212948 ) ) ;
#71967=CARTESIAN_POINT ( 'NONE',  ( 0.4724409448818898682, 2.892866454678787531E-17, -1.927165354330708569 ) ) ;
#71971=CARTESIAN_POINT ( 'NONE',  ( 0.2891555358219910499, -0.2891555358219909944, -1.277559055118109965 ) ) ;
#71981=CARTESIAN_POINT ( 'NONE',  ( 0.1998031496062994128, -0.3460692066303957537, -2.215879265091863726 ) ) ;
#71982=CARTESIAN_POINT ( 'NONE',  ( 0.3917322834645668994, -0.1049643490035303134, -1.923865198653856634 ) ) ;
#71995=CARTESIAN_POINT ( 'NONE',  ( 0.3996062992125984925, 0.1070741851644054637, 0.1135170603674540563 ) ) ;
#71997=CARTESIAN_POINT ( 'NONE',  ( 0.1958661417322836440, -0.3392501089628017219, -1.593832020997375531 ) ) ;
#72008=ORIENTED_EDGE ( 'NONE', *, *, #38239, .T. ) ;
#72018=CARTESIAN_POINT ( 'NONE',  ( -0.2867679344610364334, -0.2867679344610367109, -2.413385826771653253 ) ) ;
#72021=CARTESIAN_POINT ( 'NONE',  ( 0.3460692066303959757, -0.1998031496062991907, -0.1049868766404199599 ) ) ;
#72024=CARTESIAN_POINT ( 'NONE',  ( -0.3392501089628017219, -0.1958661417322836718, -1.934383202099737575 ) ) ;
#72035=CARTESIAN_POINT ( 'NONE',  ( -0.1958661417322834497, -0.3392501089628018884, -1.090531865320523153 ) ) ;
#72042=CARTESIAN_POINT ( 'NONE',  ( 0.3392501089628018329, 0.1958661417322835607, -2.647657111057429624 ) ) ;
#72051=CARTESIAN_POINT ( 'NONE',  ( 4.797336870675656522E-17, -0.3917322834645670104, -1.895669291338582640 ) ) ;
#72065=CARTESIAN_POINT ( 'NONE',  ( -0.4724409448818895907, -0.1265901696524993070, -0.2801837270341207553 ) ) ;
#72068=CARTESIAN_POINT ( 'NONE',  ( -0.2891555358219911054, 0.2891555358219909388, -0.09645669291338582196 ) ) ;
#72073=CARTESIAN_POINT ( 'NONE',  ( 0.2891555358219910499, -0.2891555358219909944, -0.1751968503937007815 ) ) ;
#72080=CARTESIAN_POINT ( 'NONE',  ( -0.1998031496062991630, -0.3460692066303959202, -0.9297900262467192478 ) ) ;
#72083=CARTESIAN_POINT ( 'NONE',  ( -0.2867679344610365999, 0.2867679344610364889, -0.4842519685039369248 ) ) ;
#72086=CARTESIAN_POINT ( 'NONE',  ( 0.4724409448818902568, -0.1265901696524981135, -0.5032808398950130435 ) ) ;
#72094=CARTESIAN_POINT ( 'NONE',  ( -0.3965571307776180610, -0.02707642104390632631, -1.220472440944881942 ) ) ;
#72096=CARTESIAN_POINT ( 'NONE',  ( -0.1998031496062994405, 0.3460692066303957537, 0.2250656167979002420 ) ) ;
#72113=CARTESIAN_POINT ( 'NONE',  ( 0.1998031496062994405, -0.3460692066303958092, -0.8792650918635170898 ) ) ;
#72118=CARTESIAN_POINT ( 'NONE',  ( 0.2925321140481932369, 0.2925321140481932369, -2.500000000000000444 ) ) ;
#72119=CARTESIAN_POINT ( 'NONE',  ( -0.3949938075777409408, -0.1058382717557502933, -1.778215223097113107 ) ) ;
#72121=CARTESIAN_POINT ( 'NONE',  ( 0.3917322834645670104, -0.1049643490035303411, -0.4186351706036745557 ) ) ;
#72122=CARTESIAN_POINT ( 'NONE',  ( -9.594673741351313045E-17, 0.3917322834645670104, -0.9370078740157480324 ) ) ;
#72124=CARTESIAN_POINT ( 'NONE',  ( 0.3392501089628018329, 0.1958661417322835607, -0.9107611548556429071 ) ) ;
#72126=CARTESIAN_POINT ( 'NONE',  ( 0.3392501089628018329, 0.1958661417322835052, -0.05378645849637612303 ) ) ;
#72133=CARTESIAN_POINT ( 'NONE',  ( 0.3996062992125986590, -0.1070741851644053111, -2.473753280839894764 ) ) ;
#72134=CARTESIAN_POINT ( 'NONE',  ( 0.1049643490035304799, -0.3917322834645670104, -1.026922202920946825 ) ) ;
#72142=CARTESIAN_POINT ( 'NONE',  ( -0.1958661417322834220, -0.3392501089628018884, -0.4652230971128609727 ) ) ;
#72150=CARTESIAN_POINT ( 'NONE',  ( -0.02733964191563385132, -0.3913445824880820156, -1.929133858267717994 ) ) ;
#72152=CARTESIAN_POINT ( 'NONE',  ( 0.3917322834645670104, 2.398668435337828261E-17, -2.000000000000000000 ) ) ;
#72154=CARTESIAN_POINT ( 'NONE',  ( 0.3996062992125986590, -0.1070741851644053111, -0.5839895013123358458 ) ) ;
#72160=CARTESIAN_POINT ( 'NONE',  ( 0.4724409448818898127, -0.1265901696524988629, -1.213910761154855411 ) ) ;
#72161=CARTESIAN_POINT ( 'NONE',  ( -0.3917322834645669549, -0.1049643490035306603, -1.390419947506561504 ) ) ;
#72171=DIRECTION ( 'NONE',  ( 0.000000000000000000, 0.000000000000000000, 1.000000000000000000 ) ) ;
#72180=CARTESIAN_POINT ( 'NONE',  ( 0.3917322834645668994, 0.1049643490035304522, -0.9921066684701294047 ) ) ;
#72183=CARTESIAN_POINT ( 'NONE',  ( 0.1958661417322836440, -0.3392501089628017219, -1.121391076115485719 ) ) ;
#72190=CARTESIAN_POINT ( 'NONE',  ( 0.2867679344610366554, 0.2867679344610366554, 0.02294656348325270490 ) ) ;
#72194=AXIS2_PLACEMENT_3D ( 'NONE', #24754, #50015, #23938 ) ;
#72197=CARTESIAN_POINT ( 'NONE',  ( -0.4724409448818898682, -8.678599364036362592E-17, -1.690944881889763884 ) ) ;
#72209=PRODUCT ( 'Independent Actuating Lead Screws', 'Independent Actuating Lead Screws', '', ( #29207 ) ) ;
#72214=CARTESIAN_POINT ( 'NONE',  ( -0.1058382717557503072, 0.3949938075777408852, 0.2316272965879264401 ) ) ;
#72220=CARTESIAN_POINT ( 'NONE',  ( 0.1998031496062994128, -0.3460692066303957537, -1.743438320209973913 ) ) ;
#72227=CARTESIAN_POINT ( 'NONE',  ( -9.787531504996567848E-17, 0.3996062992125986035, -1.259842519685039353 ) ) ;
#72228=CARTESIAN_POINT ( 'NONE',  ( -0.1974969037888703871, -0.3420746716998661063, -0.8530183727034120755 ) ) ;
#72233=CARTESIAN_POINT ( 'NONE',  ( -0.3420746716998660508, -0.1974969037888706924, -1.861548556430446588 ) ) ;
#72238=CARTESIAN_POINT ( 'NONE',  ( -0.4724409448818899238, 0.1265901696524986686, -2.080052493438320216 ) ) ;
#72240=ORIENTED_EDGE ( 'NONE', *, *, #38275, .T. ) ;
#72245=CARTESIAN_POINT ( 'NONE',  ( -0.3917322834645669549, -7.196005306013483243E-17, -2.324127665845457713 ) ) ;
#72251=CARTESIAN_POINT ( 'NONE',  ( -0.3392501089628019439, 0.1958661417322832554, -2.783445251147295352 ) ) ;
#72253=CARTESIAN_POINT ( 'NONE',  ( -0.3917322834645669549, -0.1049643490035306603, -1.770341207349081181 ) ) ;
#72256=CARTESIAN_POINT ( 'NONE',  ( 0.1058382717557499880, 0.3949938075777411073, -2.198162729658792891 ) ) ;
#72262=CARTESIAN_POINT ( 'NONE',  ( -0.3996062992125986035, -7.340648628747425578E-17, -0.6692913385826770867 ) ) ;
#72266=CARTESIAN_POINT ( 'NONE',  ( 0.03178304480586199854, -0.3983403474834772418, -9.560572922657961637E-16 ) ) ;
#72269=CARTESIAN_POINT ( 'NONE',  ( -0.3917322834645670104, -7.196005306013484475E-17, -0.4389763779527560139 ) ) ;
#72281=CARTESIAN_POINT ( 'NONE',  ( -0.1265901696524986964, -0.4724409448818899238, -1.332020997375328086 ) ) ;
#72284=CARTESIAN_POINT ( 'NONE',  ( 0.1958661417322834775, 0.3392501089628018884, -0.4514435695538057125 ) ) ;
#72285=CARTESIAN_POINT ( 'NONE',  ( 0.3392501089628018884, -0.1958661417322834220, -2.394356955380577467 ) ) ;
#72288=CARTESIAN_POINT ( 'NONE',  ( -0.2925321140481930149, -0.2925321140481933480, 0.02165354330708658959 ) ) ;
#72293=CARTESIAN_POINT ( 'NONE',  ( -0.1974969037888704149, -0.3420746716998661063, -2.819553805774278388 ) ) ;
#72295=CARTESIAN_POINT ( 'NONE',  ( -9.594673741351313045E-17, 0.3917322834645670104, -0.08464566929133868212 ) ) ;
#72300=CARTESIAN_POINT ( 'NONE',  ( 0.2867679344610365999, 0.2867679344610365999, -1.862204724409449064 ) ) ;
#72304=CARTESIAN_POINT ( 'NONE',  ( -0.1265901696524993347, 0.4724409448818895907, -0.2408136482939632061 ) ) ;
#72314=CARTESIAN_POINT ( 'NONE',  ( 0.1265901696524989184, 0.4724409448818898127, -1.959973753280839892 ) ) ;
#72317=CARTESIAN_POINT ( 'NONE',  ( 0.3460692066303959202, -0.1998031496062991630, -1.599081364829396223 ) ) ;
#72319=CARTESIAN_POINT ( 'NONE',  ( -0.3917322834645669549, -0.1049643490035306603, -2.807742782152229832 ) ) ;
#72327=CARTESIAN_POINT ( 'NONE',  ( 0.1998031496062992740, 0.3460692066303959757, 0.01312335958005248458 ) ) ;
#72328=CARTESIAN_POINT ( 'NONE',  ( -0.1958661417322833942, -0.3392501089628018884, -2.582040313157166977 ) ) ;
#72333=CARTESIAN_POINT ( 'NONE',  ( 0.1049643490035303689, 0.3917322834645670104, -2.597769028871390606 ) ) ;
#72341=CARTESIAN_POINT ( 'NONE',  ( -0.1998031496062991907, -0.3460692066303959757, -1.640419947506561726 ) ) ;
#72342=ORIENTED_EDGE ( 'NONE', *, *, #40988, .F. ) ;
#72343=CARTESIAN_POINT ( 'NONE',  ( 0.3917322834645670104, 0.1049643490035304660, -0.2788907068579546400 ) ) ;
#72356=CARTESIAN_POINT ( 'NONE',  ( 0.3917322834645670104, 2.398668435337828261E-17, -0.5826771653543306728 ) ) ;
#72359=CARTESIAN_POINT ( 'NONE',  ( 0.3949938075777409408, 0.1058382717557500574, -1.069553805774278388 ) ) ;
#72374=CARTESIAN_POINT ( 'NONE',  ( -0.2925321140481930704, -0.2925321140481933480, -1.161417322834645383 ) ) ;
#72376=CARTESIAN_POINT ( 'NONE',  ( -0.2925321140481932369, 0.2925321140481931259, -0.7263779527559056648 ) ) ;
#72377=CARTESIAN_POINT ( 'NONE',  ( -0.3996062992125986590, 0.1070741851644051723, -0.7395013123359580609 ) ) ;
#72379=CARTESIAN_POINT ( 'NONE',  ( -0.4091458600556405756, 0.2362204724409446288, -0.1837270341207349056 ) ) ;
#72380=CARTESIAN_POINT ( 'NONE',  ( -0.1958661417322834220, -0.3392501089628018884, -2.197506561679789971 ) ) ;
#72386=CARTESIAN_POINT ( 'NONE',  ( -0.2362204724409451284, 0.4091458600556402425, -1.822178477690288512 ) ) ;
#72389=CARTESIAN_POINT ( 'NONE',  ( 0.1974969037888706092, -0.3420746716998660508, -1.585958005249344493 ) ) ;
#72400=CARTESIAN_POINT ( 'NONE',  ( 0.3460692066303958092, 0.1998031496062993018, -2.570209973753280863 ) ) ;
#72401=CARTESIAN_POINT ( 'NONE',  ( 4.797336870675655290E-17, -0.3917322834645669549, -1.891056799703724645 ) ) ;
#72412=CARTESIAN_POINT ( 'NONE',  ( -0.3996062992125984925, -0.1070741851644056858, 0.1922572178477690297 ) ) ;
#72414=CARTESIAN_POINT ( 'NONE',  ( 0.3917322834645670104, -0.1049643490035303411, -1.613517060367454237 ) ) ;
#72423=CARTESIAN_POINT ( 'NONE',  ( 0.1070741851644054776, -0.3996062992125984925, -0.9494750656167976199 ) ) ;
#72436=CARTESIAN_POINT ( 'NONE',  ( 0.1958661417322836440, -0.3392501089628017219, -2.288713910761154935 ) ) ;
#72440=CARTESIAN_POINT ( 'NONE',  ( -0.3996062992125987146, 0.1070741851644051862, -0.6627296587926508886 ) ) ;
#72443=CARTESIAN_POINT ( 'NONE',  ( -0.3917322834645670104, -7.196005306013484475E-17, -2.236220472440944906 ) ) ;
#72454=CARTESIAN_POINT ( 'NONE',  ( -0.2867679344610366554, 0.2867679344610365444, -1.044600106790339433 ) ) ;
#72460=CARTESIAN_POINT ( 'NONE',  ( -0.1958661417322836995, 0.3392501089628017219, -2.529546874836956949 ) ) ;
#72469=CARTESIAN_POINT ( 'NONE',  ( -0.3392501089628017219, -0.1958661417322836718, -1.711942257217847763 ) ) ;
#72477=CARTESIAN_POINT ( 'NONE',  ( -0.3460692066303960868, 0.1998031496062990242, -1.916010498687664043 ) ) ;
#72482=CARTESIAN_POINT ( 'NONE',  ( -0.1265901696524986964, -0.4724409448818899238, -0.7788713910761155823 ) ) ;
#72485=CARTESIAN_POINT ( 'NONE',  ( 0.2891555358219910499, -0.2891555358219909944, -0.01771653543307087977 ) ) ;
#72490=CARTESIAN_POINT ( 'NONE',  ( 0.2891555358219910499, 0.2891555358219910499, -0.6870078740157480324 ) ) ;
#72497=CARTESIAN_POINT ( 'NONE',  ( -0.3460692066303957537, -0.1998031496062994405, -1.389107611548556553 ) ) ;
#72499=CARTESIAN_POINT ( 'NONE',  ( -0.3917322834645671215, 0.1049643490035301469, -0.4973753280839895430 ) ) ;
#72513=CARTESIAN_POINT ( 'NONE',  ( 0.3460692066303958092, 0.1998031496062993018, 0.1069553805774277888 ) ) ;
#72532=CARTESIAN_POINT ( 'NONE',  ( 0.3460692066303959757, -0.1998031496062991907, -0.7349081364829396223 ) ) ;
#72533=CARTESIAN_POINT ( 'NONE',  ( 0.3458507752293908943, 0.3458507752293908943, -1.159448818897637734 ) ) ;
#72536=CARTESIAN_POINT ( 'NONE',  ( -0.1998031496062991907, -0.3460692066303959757, -2.585301837270341352 ) ) ;
#72537=CARTESIAN_POINT ( 'NONE',  ( -9.674558042662121740E-17, 0.3949938075777409963, -1.889763779527559029 ) ) ;
#72538=CARTESIAN_POINT ( 'NONE',  ( -0.1049643490035307020, 0.3917322834645669549, -0.6286089238845143923 ) ) ;
#72542=CARTESIAN_POINT ( 'NONE',  ( 0.3917322834645670104, -0.1049643490035303411, -0.8910761154855640909 ) ) ;
#72544=CARTESIAN_POINT ( 'NONE',  ( -0.3392501089628018329, -0.1958661417322836440, 0.02495369898393883651 ) ) ;
#72550=CARTESIAN_POINT ( 'NONE',  ( -0.3996062992125987146, 0.1070741851644051862, -2.395013123359580387 ) ) ;
#72551=CARTESIAN_POINT ( 'NONE',  ( 0.1958661417322834775, 0.3392501089628018884, -1.243457635991812582 ) ) ;
#72556=CARTESIAN_POINT ( 'NONE',  ( -0.1049643490035302024, -0.3917322834645671215, -0.4717847769028871152 ) ) ;
#72564=CARTESIAN_POINT ( 'NONE',  ( 0.06766049032769154425, -0.3859888145975187701, -1.929133858267717549 ) ) ;
#72565=CARTESIAN_POINT ( 'NONE',  ( -9.594673741351313045E-17, 0.3917322834645670104, -1.724409448818897683 ) ) ;
#72567=CARTESIAN_POINT ( 'NONE',  ( 0.2925321140481932369, -0.2925321140481932369, -0.2559055118110236116 ) ) ;
#72574=CARTESIAN_POINT ( 'NONE',  ( 0.2867679344610365999, -0.2867679344610365444, -1.127952755905512028 ) ) ;
#72579=ORIENTED_EDGE ( 'NONE', *, *, #32099, .F. ) ;
#72595=CARTESIAN_POINT ( 'NONE',  ( 0.1049643490035304522, -0.3917322834645668994, -1.267697219651231499 ) ) ;
#72605=CARTESIAN_POINT ( 'NONE',  ( 0.1958661417322836718, -0.3392501089628017219, -0.2460823079078234277 ) ) ;
#72608=CARTESIAN_POINT ( 'NONE',  ( 0.2362204724409449064, 0.4091458600556404646, -1.480971128608923548 ) ) ;
#72622=EDGE_LOOP ( 'NONE', ( #37772, #13780, #37937, #9315 ) ) ;
#72623=CARTESIAN_POINT ( 'NONE',  ( 0.3996062992125985480, 2.446882876249141654E-17, -2.872047244094488416 ) ) ;
#72628=CARTESIAN_POINT ( 'NONE',  ( -0.2925321140481930149, -0.2925321140481933480, -1.710629921259842812 ) ) ;
#72634=CARTESIAN_POINT ( 'NONE',  ( 0.3996062992125986035, 0.1070741851644054776, -1.384514435695537671 ) ) ;
#72635=CARTESIAN_POINT ( 'NONE',  ( 4.837279021331060870E-17, -0.3949938075777409963, -0.7086614173228346081 ) ) ;
#72636=CARTESIAN_POINT ( 'NONE',  ( 0.1049643490035303689, 0.3917322834645670104, -0.1430446194225721279 ) ) ;
#72640=CARTESIAN_POINT ( 'NONE',  ( 0.3949938075777409408, -0.1058382717557499186, -1.920603674540682260 ) ) ;
#72644=CARTESIAN_POINT ( 'NONE',  ( 0.4091458600556404646, -0.2362204724409448231, -1.837270341207349000 ) ) ;
#72645=CARTESIAN_POINT ( 'NONE',  ( 0.3588842212257977726, 0.1584414948821297187, -2.755905511811021835 ) ) ;
#72652=CARTESIAN_POINT ( 'NONE',  ( -0.2867679344610366554, 0.2867679344610365444, -2.461922941436009094 ) ) ;
#72661=CARTESIAN_POINT ( 'NONE',  ( -0.3917322834645669549, -7.196005306013483243E-17, -2.796568610727347082 ) ) ;
#72663=CARTESIAN_POINT ( 'NONE',  ( -9.594673741351313045E-17, 0.3917322834645670104, -1.724409448818897683 ) ) ;
#72666=CARTESIAN_POINT ( 'NONE',  ( -0.1974969037888703871, -0.3420746716998661063, -2.427821522309711266 ) ) ;
#72671=CARTESIAN_POINT ( 'NONE',  ( -0.1070741851644056997, 0.3996062992125986035, -0.7939632545931758489 ) ) ;
#72676=CARTESIAN_POINT ( 'NONE',  ( -0.1958661417322836718, 0.3392501089628017219, -0.09776902887139117537 ) ) ;
#72678=CARTESIAN_POINT ( 'NONE',  ( 0.1958661417322836440, -0.3392501089628017219, -0.6489501312335959060 ) ) ;
#72689=CARTESIAN_POINT ( 'NONE',  ( 0.4724409448818896462, 0.1265901696524990294, -1.069553805774278166 ) ) ;
#72692=CARTESIAN_POINT ( 'NONE',  ( -0.3917322834645670104, -7.196005306013484475E-17, -0.8188976377952754682 ) ) ;
#72693=CARTESIAN_POINT ( 'NONE',  ( -0.1958661417322836718, 0.3392501089628017219, -2.617454068241469756 ) ) ;
#72696=CARTESIAN_POINT ( 'NONE',  ( -0.1070741851644056997, 0.3996062992125984925, -0.2408136482939632061 ) ) ;
#72701=CARTESIAN_POINT ( 'NONE',  ( -0.3392501089628019439, 0.1958661417322832554, 0.05120041814404382302 ) ) ;
#72703=DIRECTION ( 'NONE',  ( 1.000000000000000000, 0.000000000000000000, 0.000000000000000000 ) ) ;
#72708=CARTESIAN_POINT ( 'NONE',  ( 0.3917322834645669549, 0.1049643490035304660, -2.006561679790026531 ) ) ;
#72712=CARTESIAN_POINT ( 'NONE',  ( -0.4724409448818895907, -0.1265901696524993070, -0.4376640419947506744 ) ) ;
#72722=CARTESIAN_POINT ( 'NONE',  ( 0.000000000000000000, 0.000000000000000000, -1.929133858267716661 ) ) ;
#72724=MECHANICAL_DESIGN_GEOMETRIC_PRESENTATION_REPRESENTATION('',(#52567),#27049);
#72726=CARTESIAN_POINT ( 'NONE',  ( -0.2925321140481932369, 0.2925321140481931259, -1.513779527559054872 ) ) ;
#72733=CARTESIAN_POINT ( 'NONE',  ( 0.2925321140481931814, -0.2925321140481931259, -0.01771653543307089365 ) ) ;
#72735=CARTESIAN_POINT ( 'NONE',  ( 0.3460692066303959202, 0.1998031496062993295, -0.1312335958005249603 ) ) ;
#72736=CARTESIAN_POINT ( 'NONE',  ( -9.594673741351313045E-17, 0.3917322834645670659, -2.358943200296274689 ) ) ;
#72741=CARTESIAN_POINT ( 'NONE',  ( 0.1049643490035304938, -0.3917322834645669549, -2.532152230971127960 ) ) ;
#72748=ORIENTED_EDGE ( 'NONE', *, *, #82059, .F. ) ;
#72749=CARTESIAN_POINT ( 'NONE',  ( 0.3392501089628018329, 0.1958661417322835607, -0.4429327016086107571 ) ) ;
#72762=CARTESIAN_POINT ( 'NONE',  ( 0.3917322834645669549, 0.1049643490035304660, -0.7467191601049868455 ) ) ;
#72764=EDGE_LOOP ( 'NONE', ( #6389, #53196, #8058, #1572 ) ) ;
#72765=CARTESIAN_POINT ( 'NONE',  ( 0.2891555358219910499, 0.2891555358219910499, -1.082677165354330784 ) ) ;
#72781=CARTESIAN_POINT ( 'NONE',  ( 0.3460692066303959202, 0.1998031496062993295, -1.548556430446194287 ) ) ;
#72783=CARTESIAN_POINT ( 'NONE',  ( 0.3996062992125984925, 0.1070741851644054637, -0.9888451443569553634 ) ) ;
#72784=CARTESIAN_POINT ( 'NONE',  ( 0.3996062992125984925, 0.1070741851644054637, -0.5164041994750655507 ) ) ;
#72786=CARTESIAN_POINT ( 'NONE',  ( 0.4091458600556403535, 0.2362204724409449896, -0.1312335958005249326 ) ) ;
#72787=CARTESIAN_POINT ( 'NONE',  ( -0.1958661417322836718, 0.3392501089628017219, -2.302493438320210029 ) ) ;
#72793=CARTESIAN_POINT ( 'NONE',  ( 0.1265901696524990294, -0.4724409448818896462, -1.894356955380577023 ) ) ;
#72796=CARTESIAN_POINT ( 'NONE',  ( -0.3949938075777409963, -7.255918531996591613E-17, -1.690944881889764329 ) ) ;
#72807=CARTESIAN_POINT ( 'NONE',  ( 0.1998031496062994128, -0.3460692066303957537, -2.530839895013123453 ) ) ;
#72808=CARTESIAN_POINT ( 'NONE',  ( -0.3392501089628019439, 0.1958661417322832554, -2.153523991304775009 ) ) ;
#72822=CARTESIAN_POINT ( 'NONE',  ( -0.1070741851644051862, -0.3996062992125986590, -0.1489501312335958227 ) ) ;
#72824=CARTESIAN_POINT ( 'NONE',  ( 0.3917322834645669549, 0.1049643490035304660, -1.311679790026246906 ) ) ;
#72833=CARTESIAN_POINT ( 'NONE',  ( 0.3996062992125986035, -0.1070741851644052972, -1.133202099737532720 ) ) ;
#72840=CARTESIAN_POINT ( 'NONE',  ( 0.3979867861068622781, 0.002674255378527819714, -1.220472440944881942 ) ) ;
#72849=CARTESIAN_POINT ( 'NONE',  ( 0.3996062992125986035, 0.1070741851644054776, -0.5971128608923884640 ) ) ;
#72853=CARTESIAN_POINT ( 'NONE',  ( -0.1049643490035307020, 0.3917322834645669549, -2.203412073490814027 ) ) ;
#72860=CARTESIAN_POINT ( 'NONE',  ( 0.2362204724409451007, -0.4091458600556402980, -2.058398950131233640 ) ) ;
#72864=CARTESIAN_POINT ( 'NONE',  ( 0.3917322834645669549, 2.398668435337827645E-17, -1.772946563483252858 ) ) ;
#72871=CARTESIAN_POINT ( 'NONE',  ( 0.2891555358219910499, -0.2891555358219909944, 0.05905511811023616414 ) ) ;
#72880=CARTESIAN_POINT ( 'NONE',  ( 0.1958661417322834775, 0.3392501089628018884, -1.646325459317585338 ) ) ;
#72889=CARTESIAN_POINT ( 'NONE',  ( 0.3996062992125986590, -0.1070741851644053111, -1.843832020997375309 ) ) ;
#72894=CARTESIAN_POINT ( 'NONE',  ( 0.4724409448818897572, -0.1265901696524988906, -0.8182414698162727706 ) ) ;
#72897=CARTESIAN_POINT ( 'NONE',  ( -0.3420746716998662729, 0.1974969037888702206, 0.05446194225721785048 ) ) ;
#72902=CARTESIAN_POINT ( 'NONE',  ( 0.2891555358219910499, 0.2891555358219910499, -0.3720472440944882497 ) ) ;
#72909=CARTESIAN_POINT ( 'NONE',  ( -0.1070741851644056997, 0.3996062992125984925, -1.185695538057742526 ) ) ;
#72911=CARTESIAN_POINT ( 'NONE',  ( -0.3917322834645671215, 0.1049643490035301469, -1.284776902887139194 ) ) ;
#72924=CARTESIAN_POINT ( 'NONE',  ( -0.4724409448818898682, -8.678599364036362592E-17, -2.793307086614173151 ) ) ;
#72941=CARTESIAN_POINT ( 'NONE',  ( 0.1998031496062992740, 0.3460692066303959757, -0.6167979002624671692 ) ) ;
#72945=CARTESIAN_POINT ( 'NONE',  ( -0.1265901696524993347, 0.4724409448818895907, -0.006561679790026246628 ) ) ;
#72946=CARTESIAN_POINT ( 'NONE',  ( 0.1974969037888706369, -0.3420746716998659953, -2.139107611548556331 ) ) ;
#72948=AXIS2_PLACEMENT_3D ( 'NONE', #34502, #41634, #15987 ) ;
#72949=CARTESIAN_POINT ( 'NONE',  ( -0.3917322834645670104, -7.196005306013484475E-17, -0.9763779527559053317 ) ) ;
#72953=CARTESIAN_POINT ( 'NONE',  ( 0.1049643490035303689, 0.3917322834645670104, -1.087926509186351476 ) ) ;
#72955=CARTESIAN_POINT ( 'NONE',  ( 4.797336870675655290E-17, -0.3917322834645669549, -0.1587733351367961454 ) ) ;
#72961=CARTESIAN_POINT ( 'NONE',  ( 0.4724409448818898682, 2.892866454678787531E-17, -1.062992125984252079 ) ) ;
#72962=CARTESIAN_POINT ( 'NONE',  ( -0.1958661417322833942, -0.3392501089628018884, -1.479678108432757933 ) ) ;
#72968=CARTESIAN_POINT ( 'NONE',  ( 0.3392501089628018329, 0.1958661417322835607, -0.3733595800524935338 ) ) ;
#72976=CARTESIAN_POINT ( 'NONE',  ( -0.1265901696524993347, 0.4724409448818896462, -0.5557742782152230721 ) ) ;
#72977=CARTESIAN_POINT ( 'NONE',  ( -0.1958661417322836718, 0.3392501089628017219, -2.209973753280840114 ) ) ;
#72979=CARTESIAN_POINT ( 'NONE',  ( 0.1998031496062994405, -0.3460692066303958092, -0.5643044619422572516 ) ) ;
#72980=VERTEX_POINT ( 'NONE', #23162 ) ;
#72986=CARTESIAN_POINT ( 'NONE',  ( -0.3392501089628019995, 0.1958661417322832277, -1.213254593175852936 ) ) ;
#72987=CARTESIAN_POINT ( 'NONE',  ( -0.1998031496062991630, -0.3460692066303959202, -2.032152230971128848 ) ) ;
#72997=CARTESIAN_POINT ( 'NONE',  ( 0.3460692066303958092, 0.1998031496062993018, -1.940288713910761409 ) ) ;
#72999=CARTESIAN_POINT ( 'NONE',  ( -0.3392501089628017219, -0.1958661417322836718, 0.1128608923884514836 ) ) ;
#73007=CARTESIAN_POINT ( 'NONE',  ( -0.1049643490035301746, -0.3917322834645670659, -1.097093545110549462 ) ) ;
#73017=CARTESIAN_POINT ( 'NONE',  ( -0.1049643490035302301, -0.3917322834645671770, -0.06891695357711476178 ) ) ;
#73021=CARTESIAN_POINT ( 'NONE',  ( -0.4091458600556402980, -0.2362204724409451284, -1.546587926509186639 ) ) ;
#73033=CARTESIAN_POINT ( 'NONE',  ( 0.2017716535433070613, -0.2017716535433070890, -0.3937007874015748254 ) ) ;
#73037=CARTESIAN_POINT ( 'NONE',  ( 0.1070741851644054776, -0.3996062992125984925, -2.839238845144356649 ) ) ;
#73042=CARTESIAN_POINT ( 'NONE',  ( -0.1998031496062991630, -0.3460692066303959202, -1.874671916010498762 ) ) ;
#73047=CARTESIAN_POINT ( 'NONE',  ( -0.1070741851644051862, -0.3996062992125986035, -0.9363517060367454459 ) ) ;
#73048=CARTESIAN_POINT ( 'NONE',  ( 0.3460692066303959757, -0.1998031496062991907, -1.364829396325459188 ) ) ;
#73049=CARTESIAN_POINT ( 'NONE',  ( 0.2891555358219910499, -0.2891555358219909944, -1.043307086614173373 ) ) ;
#73050=CARTESIAN_POINT ( 'NONE',  ( -9.787531504996567848E-17, 0.3996062992125986035, -2.677165354330708347 ) ) ;
#73052=AXIS2_PLACEMENT_3D ( 'NONE', #72722, #15069, #40725 ) ;
#73053=CARTESIAN_POINT ( 'NONE',  ( 0.1049643490035303689, 0.3917322834645670104, -0.3005249343832020470 ) ) ;
#73057=CARTESIAN_POINT ( 'NONE',  ( 0.1058382717557500852, -0.3949938075777408852, -1.736876640419947826 ) ) ;
#73061=CARTESIAN_POINT ( 'NONE',  ( 0.4091458600556403535, 0.2362204724409449896, -1.863517060367454015 ) ) ;
#73062=CARTESIAN_POINT ( 'NONE',  ( 0.3814249188612239272, -0.08989863709124447377, -2.755905511811024500 ) ) ;
#73066=AXIS2_PLACEMENT_3D ( 'NONE', #62390, #28338, #47688 ) ;
#73070=CARTESIAN_POINT ( 'NONE',  ( -0.1958661417322836440, 0.3392501089628016664, -2.612841576606612204 ) ) ;
#73077=CARTESIAN_POINT ( 'NONE',  ( -0.1049643490035301746, -0.3917322834645670659, -2.829377009677478405 ) ) ;
#73079=CARTESIAN_POINT ( 'NONE',  ( -0.3917322834645671215, 0.1049643490035301469, -1.914698162729658648 ) ) ;
#73082=CARTESIAN_POINT ( 'NONE',  ( 0.1058382717557500713, -0.3949938075777409408, -2.290026246719159886 ) ) ;
#73087=CARTESIAN_POINT ( 'NONE',  ( 0.1998031496062994405, -0.3460692066303958092, -0.5643044619422572516 ) ) ;
#73092=CARTESIAN_POINT ( 'NONE',  ( 0.3917322834645670104, 2.398668435337828261E-17, 0.1122047244094487306 ) ) ;
#73103=CARTESIAN_POINT ( 'NONE',  ( -0.2362204724409451284, 0.4091458600556402425, -1.430446194225721834 ) ) ;
#73106=CARTESIAN_POINT ( 'NONE',  ( 0.1958661417322834775, 0.3392501089628018884, -0.7664041994750655507 ) ) ;
#73107=CARTESIAN_POINT ( 'NONE',  ( 0.2867679344610366554, -0.2867679344610365444, -2.387795275590551380 ) ) ;
#73110=CARTESIAN_POINT ( 'NONE',  ( 0.1070741851644054776, -0.3996062992125984925, -0.1620734908136483299 ) ) ;
#73115=CARTESIAN_POINT ( 'NONE',  ( 0.2867679344610365999, 0.2867679344610365999, 0.09713217667422754942 ) ) ;
#73117=CARTESIAN_POINT ( 'NONE',  ( -0.3917322834645671215, 0.1049643490035301469, -0.1174540682414699083 ) ) ;
#73124=CARTESIAN_POINT ( 'NONE',  ( -0.1049643490035302024, -0.3917322834645671215, -1.796587926509185973 ) ) ;
#73128=CARTESIAN_POINT ( 'NONE',  ( 0.3458507752293908943, -0.3458507752293908943, -0.3326771653543306728 ) ) ;
#73141=CARTESIAN_POINT ( 'NONE',  ( -0.1070741851644056997, 0.3996062992125984925, -1.658136482939632117 ) ) ;
#73150=CARTESIAN_POINT ( 'NONE',  ( 0.1070741851644054915, -0.3996062992125986035, -0.2427821522309711322 ) ) ;
#73151=CARTESIAN_POINT ( 'NONE',  ( -0.1049643490035307158, 0.3917322834645670104, -2.365504880086300776 ) ) ;
#73155=CARTESIAN_POINT ( 'NONE',  ( -0.1049643490035307020, 0.3917322834645669549, -2.610892388451443225 ) ) ;
#73161=CARTESIAN_POINT ( 'NONE',  ( -0.2362204724409447953, -0.4091458600556404646, -0.6955380577427822120 ) ) ;
#73165=CARTESIAN_POINT ( 'NONE',  ( 0.2867679344610366554, 0.2867679344610366554, -0.2920140664380071471 ) ) ;
#73179=CARTESIAN_POINT ( 'NONE',  ( 4.797336870675656522E-17, -0.3917322834645670104, -0.7007874015748030150 ) ) ;
#73182=CARTESIAN_POINT ( 'NONE',  ( 0.3949938075777409408, 0.1058382717557500574, -1.227034120734908473 ) ) ;
#73193=CARTESIAN_POINT ( 'NONE',  ( 0.4724409448818898682, 2.892866454678787531E-17, -1.062992125984252079 ) ) ;
#73199=CARTESIAN_POINT ( 'NONE',  ( -0.3460692066303960868, 0.1998031496062990242, -1.601049868766404094 ) ) ;
#73202=CARTESIAN_POINT ( 'NONE',  ( 0.2925321140481932369, 0.2925321140481932369, -1.316929133858267598 ) ) ;
#73203=CARTESIAN_POINT ( 'NONE',  ( -0.1998031496062991630, -0.3460692066303959202, -0.6148293963254594097 ) ) ;
#73205=CARTESIAN_POINT ( 'NONE',  ( -0.2362204724409451284, 0.4091458600556402425, 0.1443569553805774397 ) ) ;
#73206=CARTESIAN_POINT ( 'NONE',  ( -0.3917322834645671215, 0.1049643490035301469, -2.479658792650918375 ) ) ;
#73212=CARTESIAN_POINT ( 'NONE',  ( -0.3458507752293906723, -0.3458507752293910609, -1.868110236220472453 ) ) ;
#73215=CARTESIAN_POINT ( 'NONE',  ( 0.1974969037888706092, -0.3420746716998660508, -1.743438320209973913 ) ) ;
#73225=CARTESIAN_POINT ( 'NONE',  ( 0.3996062992125985480, 2.446882876249141654E-17, -2.399606299212598604 ) ) ;
#73226=CARTESIAN_POINT ( 'NONE',  ( -0.3392501089628018329, -0.1958661417322836440, -2.494731340386139529 ) ) ;
#73235=CARTESIAN_POINT ( 'NONE',  ( 5.785732909357575061E-17, -0.4724409448818898682, -0.8661417322834645827 ) ) ;
#73240=CARTESIAN_POINT ( 'NONE',  ( 0.2925321140481932369, -0.2925321140481931814, -0.4901574803149606474 ) ) ;
#73243=CARTESIAN_POINT ( 'NONE',  ( -0.3392501089628017219, -0.1958661417322836718, -1.711942257217847763 ) ) ;
#73253=CARTESIAN_POINT ( 'NONE',  ( 0.2925321140481932369, -0.2925321140481931814, -0.9625984251968502381 ) ) ;
#73261=CARTESIAN_POINT ( 'NONE',  ( -0.2362204724409447953, -0.4091458600556404646, -2.112860892388451539 ) ) ;
#73269=CARTESIAN_POINT ( 'NONE',  ( 0.1998031496062992740, 0.3460692066303959757, -0.6167979002624671692 ) ) ;
#73272=CARTESIAN_POINT ( 'NONE',  ( 0.3392501089628018329, 0.1958661417322835607, -2.328083989501312345 ) ) ;
#73284=CARTESIAN_POINT ( 'NONE',  ( -0.1049643490035306742, 0.3917322834645668994, -1.503917692092176628 ) ) ;
#73290=CARTESIAN_POINT ( 'NONE',  ( -0.3917322834645670659, -7.196005306013484475E-17, -2.713273908957691827 ) ) ;
#73299=CARTESIAN_POINT ( 'NONE',  ( 4.797336870675656522E-17, -0.3917322834645670104, -2.053149606299212948 ) ) ;
#73307=CARTESIAN_POINT ( 'NONE',  ( 0.2925321140481932369, -0.2925321140481931814, -0.01771653543307087630 ) ) ;
#73309=CARTESIAN_POINT ( 'NONE',  ( -0.3460692066303960868, 0.1998031496062990242, -2.073490813648294129 ) ) ;
#73315=CARTESIAN_POINT ( 'NONE',  ( 0.3458507752293908943, -0.3458507752293908943, -0.8051181102362205966 ) ) ;
#73319=CARTESIAN_POINT ( 'NONE',  ( -0.3420746716998660508, -0.1974969037888706924, -0.4442257217847768724 ) ) ;
#73324=CARTESIAN_POINT ( 'NONE',  ( -0.2891555358219911054, 0.2891555358219909388, -0.4114173228346456046 ) ) ;
#73332=CARTESIAN_POINT ( 'NONE',  ( 0.1998031496062992463, 0.3460692066303959202, -1.323490813648294129 ) ) ;
#73334=CARTESIAN_POINT ( 'NONE',  ( 0.3917322834645669549, 0.1049643490035304660, -1.061679790026246462 ) ) ;
#73345=ADVANCED_FACE ( 'NONE', ( #47028 ), #79463, .T. ) ;
#73346=CARTESIAN_POINT ( 'NONE',  ( 0.4724409448818897017, 0.1265901696524990294, -0.2014435695538057958 ) ) ;
#73362=CARTESIAN_POINT ( 'NONE',  ( 0.3996062992125986035, 2.446882876249141962E-17, -0.9055118110236221041 ) ) ;
#73365=AXIS2_PLACEMENT_3D ( 'NONE', #49371, #16166, #11083 ) ;
#73367=CARTESIAN_POINT ( 'NONE',  ( 0.4724409448818898682, 2.892866454678787531E-17, 0.03937007874015747977 ) ) ;
#73368=CARTESIAN_POINT ( 'NONE',  ( -0.1974969037888703871, -0.3420746716998661063, -2.427821522309711266 ) ) ;
#73371=CARTESIAN_POINT ( 'NONE',  ( 0.1958661417322834775, 0.3392501089628018884, -0.7664041994750655507 ) ) ;
#73377=CARTESIAN_POINT ( 'NONE',  ( -0.3917322834645668994, -0.1049643490035306742, -0.2834452511472947966 ) ) ;
#73384=CARTESIAN_POINT ( 'NONE',  ( 0.1049643490035304799, -0.3917322834645670104, -1.499363147802836860 ) ) ;
#73391=CARTESIAN_POINT ( 'NONE',  ( -0.2867679344610365999, 0.2867679344610364889, -1.049212598425196763 ) ) ;
#73401=CARTESIAN_POINT ( 'NONE',  ( -0.3917322834645671215, 0.1049643490035301469, -2.229658792650918819 ) ) ;
#73407=AXIS2_PLACEMENT_3D ( 'NONE', #7058, #71876, #72703 ) ;
#73413=CARTESIAN_POINT ( 'NONE',  ( 0.3392501089628018329, 0.1958661417322835607, -1.318241469816273215 ) ) ;
#73414=CARTESIAN_POINT ( 'NONE',  ( 0.3996062992125985480, 2.446882876249141654E-17, -2.399606299212598604 ) ) ;
#73422=CARTESIAN_POINT ( 'NONE',  ( -0.2925321140481932369, 0.2925321140481930704, -2.143700787401574104 ) ) ;
#73431=CARTESIAN_POINT ( 'NONE',  ( -0.1049643490035301746, -0.3917322834645670659, -1.412054175031808967 ) ) ;
#73440=CARTESIAN_POINT ( 'NONE',  ( 0.1049643490035303967, 0.3917322834645670659, -0.6200980559393196589 ) ) ;
#73445=CARTESIAN_POINT ( 'NONE',  ( 0.4724409448818898682, 2.892866454678787531E-17, -1.612204724409448842 ) ) ;
#73462=CARTESIAN_POINT ( 'NONE',  ( -0.1998031496062991630, -0.3460692066303959202, -2.819553805774277944 ) ) ;
#73466=VECTOR ( 'NONE', #23410, 39.37007874015748143 ) ;
#73468=CARTESIAN_POINT ( 'NONE',  ( 0.2925321140481932369, 0.2925321140481932369, -2.104330708661417582 ) ) ;
#73476=CARTESIAN_POINT ( 'NONE',  ( 0.3996062992125986035, 0.1070741851644054776, -1.699475065616798064 ) ) ;
#73477=CARTESIAN_POINT ( 'NONE',  ( 0.3420746716998660508, -0.1974969037888703871, -1.207349081364829324 ) ) ;
#73478=CARTESIAN_POINT ( 'NONE',  ( 0.1070741851644054915, -0.3996062992125986035, -2.447506561679789527 ) ) ;
#73479=CARTESIAN_POINT ( 'NONE',  ( -0.4724409448818898682, -8.678599364036362592E-17, -0.6692913385826770867 ) ) ;
#73480=CARTESIAN_POINT ( 'NONE',  ( 0.1049643490035304799, -0.3917322834645669549, -0.07742782152230966164 ) ) ;
#73484=CARTESIAN_POINT ( 'NONE',  ( -0.3949938075777411073, 0.1058382717557497660, -2.156824146981627610 ) ) ;
#73488=CARTESIAN_POINT ( 'NONE',  ( -0.4724409448818899238, 0.1265901696524986686, -1.922572178477689908 ) ) ;
#73498=CARTESIAN_POINT ( 'NONE',  ( -0.1958661417322834497, -0.3392501089628018884, -2.822815329887452318 ) ) ;
#73501=CARTESIAN_POINT ( 'NONE',  ( 0.3458507752293908943, -0.3458507752293908943, -2.460629921259842146 ) ) ;
#73505=CARTESIAN_POINT ( 'NONE',  ( 0.1049643490035304938, -0.3917322834645669549, -0.01246719160104995359 ) ) ;
#73507=CARTESIAN_POINT ( 'NONE',  ( 0.1049643490035303689, 0.3917322834645670104, -2.032808398950130879 ) ) ;
#73510=CARTESIAN_POINT ( 'NONE',  ( 0.3949938075777411073, -0.1058382717557499464, -2.316272965879265122 ) ) ;
#73514=CARTESIAN_POINT ( 'NONE',  ( -0.1998031496062994683, 0.3460692066303958092, -0.9580052493438320216 ) ) ;
#73519=CARTESIAN_POINT ( 'NONE',  ( 0.3392501089628018329, 0.1958661417322835607, -0.05839895013123368173 ) ) ;
#73525=CARTESIAN_POINT ( 'NONE',  ( 0.1958661417322834775, 0.3392501089628018884, 0.02099737532808403431 ) ) ;
#73531=CARTESIAN_POINT ( 'NONE',  ( -0.4724409448818898682, -8.678599364036362592E-17, -1.456692913385826849 ) ) ;
#73533=CARTESIAN_POINT ( 'NONE',  ( -9.594673741351313045E-17, 0.3917322834645670104, -0.7795275590551180578 ) ) ;
#73535=CIRCLE ( 'NONE', #29116, 0.4724409448818898682 ) ;
#73536=CARTESIAN_POINT ( 'NONE',  ( -0.3917322834645671215, 0.1049643490035301469, -2.322178477690288290 ) ) ;
#73540=CARTESIAN_POINT ( 'NONE',  ( 0.1998031496062992463, 0.3460692066303959202, -0.2211286089238845565 ) ) ;
#73545=CARTESIAN_POINT ( 'NONE',  ( 4.797336870675655290E-17, -0.3917322834645669549, -0.1587733351367961454 ) ) ;
#73547=CARTESIAN_POINT ( 'NONE',  ( 0.3917322834645670104, 2.398668435337828261E-17, -0.3602362204724410266 ) ) ;
#73552=CARTESIAN_POINT ( 'NONE',  ( -0.3917322834645669549, -0.1049643490035306603, -2.400262467191600635 ) ) ;
#73555=CARTESIAN_POINT ( 'NONE',  ( -0.2362204724409447953, -0.4091458600556404646, -0.4573490813648293796 ) ) ;
#73565=CARTESIAN_POINT ( 'NONE',  ( -0.1998031496062991630, -0.3460692066303959202, -1.559711286089238591 ) ) ;
#73573=CARTESIAN_POINT ( 'NONE',  ( -0.2925321140481932369, 0.2925321140481930704, -0.2539370078740156855 ) ) ;
#73574=CARTESIAN_POINT ( 'NONE',  ( -0.1998031496062991907, -0.3460692066303959757, -0.3805774278215223183 ) ) ;
#73575=CARTESIAN_POINT ( 'NONE',  ( 0.1049643490035304799, -0.3917322834645670104, -2.759205667487876656 ) ) ;
#73580=CARTESIAN_POINT ( 'NONE',  ( -0.3420746716998660508, -0.1974969037888706924, -1.074146981627296826 ) ) ;
#73587=CARTESIAN_POINT ( 'NONE',  ( 0.2362204724409451007, -0.4091458600556402980, -0.7217847769028871152 ) ) ;
#73592=CARTESIAN_POINT ( 'NONE',  ( 0.2867679344610366554, 0.2867679344610366554, -0.4494943813986370107 ) ) ;
#73606=CARTESIAN_POINT ( 'NONE',  ( 0.1958661417322834775, 0.3392501089628018884, -0.4514435695538057125 ) ) ;
#73609=CARTESIAN_POINT ( 'NONE',  ( 0.2891555358219910499, 0.2891555358219910499, -0.9251968503937008093 ) ) ;
#73619=CARTESIAN_POINT ( 'NONE',  ( 0.2362204724409451007, -0.4091458600556402980, -1.036745406824147064 ) ) ;
#73625=CARTESIAN_POINT ( 'NONE',  ( 0.1070741851644054915, -0.3996062992125986035, -1.502624671916010346 ) ) ;
#73627=ORIENTED_EDGE ( 'NONE', *, *, #13177, .F. ) ;
#73628=CARTESIAN_POINT ( 'NONE',  ( 0.3996062992125984925, 0.1070741851644054637, -1.146325459317585116 ) ) ;
#73629=CARTESIAN_POINT ( 'NONE',  ( -0.1070741851644051862, -0.3996062992125986590, -0.6213910761154856077 ) ) ;
#73632=CARTESIAN_POINT ( 'NONE',  ( -0.3458507752293909498, 0.3458507752293907833, 0.1377952755905511861 ) ) ;
#73633=CARTESIAN_POINT ( 'NONE',  ( 0.1958661417322834775, 0.3392501089628018884, -2.591207349081364519 ) ) ;
#73639=CARTESIAN_POINT ( 'NONE',  ( 0.2362204724409449064, 0.4091458600556404646, -2.110892388451443225 ) ) ;
#73642=CARTESIAN_POINT ( 'NONE',  ( -0.1058382717557497660, -0.3949938075777411073, -1.723753280839894986 ) ) ;
#73651=CARTESIAN_POINT ( 'NONE',  ( 0.3996062992125986035, -0.1070741851644052972, -2.393044619422572072 ) ) ;
#73652=AXIS2_PLACEMENT_3D ( 'NONE', #82958, #40, #18571 ) ;
#73653=CARTESIAN_POINT ( 'NONE',  ( -0.3917322834645670659, 0.1049643490035301607, -2.317565986055430738 ) ) ;
#73663=CARTESIAN_POINT ( 'NONE',  ( 0.4724409448818898127, -0.1265901696524988629, -0.8989501312335956840 ) ) ;
#73666=CARTESIAN_POINT ( 'NONE',  ( 0.1998031496062994128, -0.3460692066303957537, -0.3261154855643044748 ) ) ;
#73668=CARTESIAN_POINT ( 'NONE',  ( 0.3392501089628018329, 0.1958661417322835607, -1.790682414698162805 ) ) ;
#73678=CARTESIAN_POINT ( 'NONE',  ( 0.1998031496062992463, 0.3460692066303959202, -1.008530183727034180 ) ) ;
#73692=CARTESIAN_POINT ( 'NONE',  ( 0.1070741851644053527, 0.3996062992125986590, -0.4658792650918635592 ) ) ;
#73695=CARTESIAN_POINT ( 'NONE',  ( 0.3392501089628018329, 0.1958661417322835607, -2.013123359580052618 ) ) ;
#73696=ORIENTED_EDGE ( 'NONE', *, *, #47963, .T. ) ;
#73705=CARTESIAN_POINT ( 'NONE',  ( -0.3917322834645668994, -0.1049643490035306742, -1.543287770832334038 ) ) ;
#73711=CARTESIAN_POINT ( 'NONE',  ( -9.594673741351313045E-17, 0.3917322834645670659, -2.831384145178164058 ) ) ;
#73720=CARTESIAN_POINT ( 'NONE',  ( 0.3917322834645670104, 0.1049643490035304660, -1.223772596621734321 ) ) ;
#73722=CARTESIAN_POINT ( 'NONE',  ( 0.1049643490035304938, -0.3917322834645669549, -2.059711286089238591 ) ) ;
#73730=CARTESIAN_POINT ( 'NONE',  ( -0.3460692066303957537, -0.1998031496062994405, 0.02821522309711285356 ) ) ;
#73733=CARTESIAN_POINT ( 'NONE',  ( 0.3996062992125986035, 2.446882876249141962E-17, -1.692913385826771533 ) ) ;
#73739=CARTESIAN_POINT ( 'NONE',  ( 0.3458507752293908943, -0.3458507752293908943, -0.4901574803149606474 ) ) ;
#73742=CARTESIAN_POINT ( 'NONE',  ( -0.1058382717557497660, -0.3949938075777411073, -0.4639107611548556331 ) ) ;
#73747=CARTESIAN_POINT ( 'NONE',  ( 0.3949938075777408852, 0.1058382717557500435, -0.5164041994750657727 ) ) ;
#73754=CARTESIAN_POINT ( 'NONE',  ( 0.3996062992125986035, -0.1070741851644052972, -1.290682414698162805 ) ) ;
#73757=CARTESIAN_POINT ( 'NONE',  ( 0.1049643490035303689, 0.3917322834645670104, -0.9304461942257216123 ) ) ;
#73784=CARTESIAN_POINT ( 'NONE',  ( -0.1998031496062991907, -0.3460692066303959757, -1.167979002624671914 ) ) ;
#73788=CARTESIAN_POINT ( 'NONE',  ( -1.157146581871515012E-16, 0.4724409448818898682, 0.1574803149606299191 ) ) ;
#73789=CARTESIAN_POINT ( 'NONE',  ( 0.1058382717557499880, 0.3949938075777411073, -2.198162729658792891 ) ) ;
#73792=CARTESIAN_POINT ( 'NONE',  ( -0.3392501089628019995, 0.1958661417322832277, -0.9632545931758529356 ) ) ;
#73799=CARTESIAN_POINT ( 'NONE',  ( 0.2867679344610365999, 0.2867679344610365999, -0.2178284532470323442 ) ) ;
#73805=CARTESIAN_POINT ( 'NONE',  ( -0.3458507752293909498, 0.3458507752293908388, -0.01968503937007873988 ) ) ;
#73806=CARTESIAN_POINT ( 'NONE',  ( 0.1265901696524989184, 0.4724409448818898127, -1.095800524934382958 ) ) ;
#73807=CARTESIAN_POINT ( 'NONE',  ( -0.1049643490035307158, 0.3917322834645670104, -1.578103305283151681 ) ) ;
#73813=CARTESIAN_POINT ( 'NONE',  ( 0.2867679344610365999, -0.2867679344610365444, -1.127952755905512028 ) ) ;
#73822=CARTESIAN_POINT ( 'NONE',  ( 0.1958661417322836440, -0.3392501089628017219, -2.446194225721784576 ) ) ;
#73831=CARTESIAN_POINT ( 'NONE',  ( 0.1958661417322836440, -0.3392501089628017219, -1.436351706036745446 ) ) ;
#73832=CARTESIAN_POINT ( 'NONE',  ( 0.1998031496062994128, -0.3460692066303957537, -2.215879265091863726 ) ) ;
#73841=CARTESIAN_POINT ( 'NONE',  ( 0.1998031496062992463, 0.3460692066303959202, -1.953412073490813805 ) ) ;
#73850=CARTESIAN_POINT ( 'NONE',  ( -0.1049643490035306742, 0.3917322834645668994, -1.188957062170916679 ) ) ;
#73859=CARTESIAN_POINT ( 'NONE',  ( -0.2867679344610365444, -0.2867679344610367664, -0.5282345388789521090 ) ) ;
#73862=CARTESIAN_POINT ( 'NONE',  ( 0.4724409448818897572, -0.1265901696524988906, -2.078083989501312345 ) ) ;
#73884=CARTESIAN_POINT ( 'NONE',  ( 0.3996062992125986035, -0.1070741851644052972, -2.078083989501312345 ) ) ;
#73889=CARTESIAN_POINT ( 'NONE',  ( 0.2925321140481932369, 0.2925321140481932369, -1.870078740157480546 ) ) ;
#73890=CARTESIAN_POINT ( 'NONE',  ( -0.3949938075777409408, -0.1058382717557502933, -0.9908136482939633449 ) ) ;
#73891=CARTESIAN_POINT ( 'NONE',  ( 0.3460692066303959202, 0.1998031496062993295, -2.650918635170603554 ) ) ;
#73893=CARTESIAN_POINT ( 'NONE',  ( -0.2867679344610366554, 0.2867679344610365444, -0.01181102362204719883 ) ) ;
#73897=CARTESIAN_POINT ( 'NONE',  ( 0.1058382717557499880, 0.3949938075777409408, -2.274934383202099841 ) ) ;
#73901=CARTESIAN_POINT ( 'NONE',  ( 0.3458507752293908943, 0.3458507752293908943, -2.500000000000000444 ) ) ;
#73902=CARTESIAN_POINT ( 'NONE',  ( 0.3996062992125986035, 0.1070741851644054776, -1.541994750656167978 ) ) ;
#73911=CARTESIAN_POINT ( 'NONE',  ( -0.1049643490035307020, 0.3917322834645669549, 0.2237532808398949025 ) ) ;
#73918=CARTESIAN_POINT ( 'NONE',  ( -0.2867679344610365999, 0.2867679344610364889, -0.1043307086614174151 ) ) ;
#73920=CARTESIAN_POINT ( 'NONE',  ( 0.2867679344610365999, 0.2867679344610365999, -2.177165354330708347 ) ) ;
#73923=CARTESIAN_POINT ( 'NONE',  ( 0.1974969037888704704, 0.3420746716998660508, -2.191601049868766360 ) ) ;
#73924=ORIENTED_EDGE ( 'NONE', *, *, #20205, .T. ) ;
#73927=CARTESIAN_POINT ( 'NONE',  ( -0.2925321140481930704, -0.2925321140481933480, -1.161417322834645383 ) ) ;
#73928=DIRECTION ( 'NONE',  ( 1.000000000000000000, 0.000000000000000000, 0.000000000000000000 ) ) ;
#73932=CARTESIAN_POINT ( 'NONE',  ( 0.2867679344610365999, -0.2867679344610365444, -0.1830708661417323746 ) ) ;
#73938=CARTESIAN_POINT ( 'NONE',  ( 4.797336870675656522E-17, -0.3917322834645670104, -0.07086614173228342195 ) ) ;
#73942=CARTESIAN_POINT ( 'NONE',  ( -0.2362204724409451284, 0.4091458600556402425, -1.587926509186351698 ) ) ;
#73944=CARTESIAN_POINT ( 'NONE',  ( -0.3917322834645669549, -0.1049643490035306603, -0.8254593175853015552 ) ) ;
#73949=CARTESIAN_POINT ( 'NONE',  ( 0.2362204724409451007, -0.4091458600556402980, -1.981627296587926690 ) ) ;
#73952=CARTESIAN_POINT ( 'NONE',  ( 0.3392501089628018329, -0.1958661417322834497, -0.02753973933627114692 ) ) ;
#73954=CARTESIAN_POINT ( 'NONE',  ( 0.1958661417322836440, -0.3392501089628017219, -0.3339895013123360679 ) ) ;
#73960=CARTESIAN_POINT ( 'NONE',  ( -0.1958661417322834220, -0.3392501089628018884, -2.262467191601049699 ) ) ;
#73963=CARTESIAN_POINT ( 'NONE',  ( -0.2362204724409451284, 0.4091458600556402425, -0.2473753280839895152 ) ) ;
#73965=EDGE_CURVE ( 'NONE', #21217, #34363, #46590, .T. ) ;
#73974=CARTESIAN_POINT ( 'NONE',  ( 0.3460692066303958092, 0.1998031496062993018, -1.625328083989501460 ) ) ;
#73983=CARTESIAN_POINT ( 'NONE',  ( 0.2925321140481931814, 0.2925321140481931814, -0.3720472440944882497 ) ) ;
#73984=CARTESIAN_POINT ( 'NONE',  ( -0.3460692066303960868, 0.1998031496062990242, -0.3412073490813647969 ) ) ;
#73985=CARTESIAN_POINT ( 'NONE',  ( -0.3949938075777409963, -7.255918531996591613E-17, 0.1181102362204723977 ) ) ;
#73991=CARTESIAN_POINT ( 'NONE',  ( 4.837279021331061486E-17, -0.3949938075777409963, -1.100393700787401619 ) ) ;
#73996=CARTESIAN_POINT ( 'NONE',  ( 0.2362204724409449064, 0.4091458600556404646, -1.089238845144356871 ) ) ;
#73997=CARTESIAN_POINT ( 'NONE',  ( 0.3460692066303959202, 0.1998031496062993295, -2.335958005249343827 ) ) ;
#74000=CARTESIAN_POINT ( 'NONE',  ( -0.3917322834645671770, 0.1049643490035302024, -0.1870271897975872011 ) ) ;
#74011=CARTESIAN_POINT ( 'NONE',  ( 0.1958661417322836440, -0.3392501089628017219, -1.028871391076115360 ) ) ;
#74014=CARTESIAN_POINT ( 'NONE',  ( -0.3420746716998661618, 0.1974969037888702206, -0.9711286089238846397 ) ) ;
#74029=ORIENTED_EDGE ( 'NONE', *, *, #20687, .T. ) ;
#74030=CARTESIAN_POINT ( 'NONE',  ( -9.787531504996567848E-17, 0.3996062992125986035, -1.574803149606299302 ) ) ;
#74033=CARTESIAN_POINT ( 'NONE',  ( -0.3996062992125984925, -0.1070741851644056858, -1.225065616797899937 ) ) ;
#74037=CARTESIAN_POINT ( 'NONE',  ( 0.1265901696524989462, 0.4724409448818897572, -0.6233595800524933672 ) ) ;
#74038=CARTESIAN_POINT ( 'NONE',  ( 0.3917322834645669549, 0.1049643490035304660, -2.414041994750655729 ) ) ;
#74044=CARTESIAN_POINT ( 'NONE',  ( 5.785732909357575061E-17, -0.4724409448818898682, -2.202755905511811108 ) ) ;
#74047=CARTESIAN_POINT ( 'NONE',  ( 0.1974969037888704704, 0.3420746716998660508, -1.795931758530183942 ) ) ;
#74059=CARTESIAN_POINT ( 'NONE',  ( -0.3917322834645670659, 0.1049643490035301607, -2.475046301016061268 ) ) ;
#74073=CARTESIAN_POINT ( 'NONE',  ( 0.3996062992125984925, 0.1070741851644054637, -0.2014435695538057958 ) ) ;
#74075=CARTESIAN_POINT ( 'NONE',  ( -0.3392501089628019995, 0.1958661417322832277, -2.000656167979002920 ) ) ;
#74080=CARTESIAN_POINT ( 'NONE',  ( 0.4724409448818898682, 0.000000000000000000, -2.755905511811024056 ) ) ;
#74084=CARTESIAN_POINT ( 'NONE',  ( -0.1070741851644051862, -0.3996062992125986590, -1.093832020997375087 ) ) ;
#74090=B_SPLINE_CURVE_WITH_KNOTS ( 'NONE', 3,
 ( #33433, #14506, #53179, #34262, #53599, #13661, #27523, #15328, #21215, #66672, #46870, #32586, #58249, #52348, #78477, #59094, #614, #72150, #19968, #45619, #71313, #26270, #72564, #52768, #8591, #2278, #39313, #46457, #33004, #40159, #78055, #66252, #46036, #59508, #8176, #71731, #33842, #14086 ),
 .UNSPECIFIED., .F., .F.,
 ( 4, 2, 2, 2, 2, 2, 2, 2, 2, 2, 2, 2, 2, 2, 2, 2, 2, 2, 4 ),
 ( 9.146428360655323264E-14, 0.003207193274670050703, 0.004810789911959344189, 0.006414386549248637243, 0.007216184867893282034, 0.008017983186537928561, 0.009621579823827219879, 0.01042337814247186814, 0.01122517646111651467, 0.01282877309840580599, 0.01363057141705045078, 0.01443236973569509730, 0.01603596637298438862, 0.01763956301027367821, 0.01924315964756296779, 0.02084675628485226778, 0.02245035292214156084, 0.02405394955943085736, 0.02565754619672015041 ),
 .UNSPECIFIED. ) ;
#74093=CARTESIAN_POINT ( 'NONE',  ( -0.1049643490035302024, -0.3917322834645671215, -1.416666666666666519 ) ) ;
#74098=CARTESIAN_POINT ( 'NONE',  ( 0.1070741851644054637, -0.3996062992125984925, -2.209317585301837639 ) ) ;
#74100=CARTESIAN_POINT ( 'NONE',  ( 0.3996062992125986590, -0.1070741851644053111, -0.4265091863517060933 ) ) ;
#74101=EDGE_LOOP ( 'NONE', ( #80526, #36736, #7533, #12114 ) ) ;
#74103=CARTESIAN_POINT ( 'NONE',  ( 0.1958661417322834775, 0.3392501089628018884, -2.026246719160105236 ) ) ;
#74113=CARTESIAN_POINT ( 'NONE',  ( -0.1049643490035301746, -0.3917322834645670659, -1.412054175031808967 ) ) ;
#74117=CARTESIAN_POINT ( 'NONE',  ( 0.3917322834645670104, -0.1049643490035303411, -2.873359580052493811 ) ) ;
#74120=CARTESIAN_POINT ( 'NONE',  ( -0.3420746716998661618, 0.1974969037888702206, 0.1312335958005248771 ) ) ;
#74129=CARTESIAN_POINT ( 'NONE',  ( 0.1958661417322834775, 0.3392501089628018884, -1.085977321031183163 ) ) ;
#74131=CARTESIAN_POINT ( 'NONE',  ( 0.3917322834645670104, -0.1049643490035303411, -2.400918635170603554 ) ) ;
#74138=CARTESIAN_POINT ( 'NONE',  ( -0.3996062992125985480, -7.340648628747423112E-17, 0.04133858267716534335 ) ) ;
#74140=CARTESIAN_POINT ( 'NONE',  ( -9.787531504996567848E-17, 0.3996062992125986035, -1.889763779527559251 ) ) ;
#74145=CARTESIAN_POINT ( 'NONE',  ( -0.4724409448818898682, -8.678599364036362592E-17, -0.9035433070866141225 ) ) ;
#74148=CARTESIAN_POINT ( 'NONE',  ( -0.3949938075777408852, -0.1058382717557502933, -0.7526246719160105680 ) ) ;
#74153=CARTESIAN_POINT ( 'NONE',  ( -0.3949938075777409963, -7.255918531996591613E-17, -0.2736220472440945017 ) ) ;
#74161=CARTESIAN_POINT ( 'NONE',  ( 0.1070741851644053388, 0.3996062992125986035, -1.330052493438320438 ) ) ;
#74164=CARTESIAN_POINT ( 'NONE',  ( 0.1958661417322836440, -0.3392501089628017219, -1.028871391076115360 ) ) ;
#74190=DIRECTION ( 'NONE',  ( 8.462065736472231082E-17, -1.000000000000000000, 0.000000000000000000 ) ) ;
#74196=CARTESIAN_POINT ( 'NONE',  ( 0.4091458600556404646, -0.2362204724409448231, -0.1049868766404199460 ) ) ;
#74197=CARTESIAN_POINT ( 'NONE',  ( 4.837279021331060870E-17, -0.3949938075777409963, -2.440944881889763884 ) ) ;
#74200=CARTESIAN_POINT ( 'NONE',  ( 0.2867679344610365999, -0.2867679344610365444, -1.035433070866141447 ) ) ;
#74202=CARTESIAN_POINT ( 'NONE',  ( -0.1265901696524986964, -0.4724409448818899238, -2.434383202099737353 ) ) ;
#74209=CARTESIAN_POINT ( 'NONE',  ( -0.2867679344610366554, 0.2867679344610365444, -0.4146788469478197015 ) ) ;
#74212=ADVANCED_FACE ( 'NONE', ( #51147 ), #19175, .T. ) ;
#74217=CARTESIAN_POINT ( 'NONE',  ( -0.3917322834645670659, -7.196005306013484475E-17, -1.453431389272652696 ) ) ;
#74223=CARTESIAN_POINT ( 'NONE',  ( 0.1049643490035304938, -0.3917322834645669549, -0.9573490813648293241 ) ) ;
#74233=CARTESIAN_POINT ( 'NONE',  ( -0.3917322834645671215, 0.1049643490035301469, -2.544619422572177658 ) ) ;
#74240=CARTESIAN_POINT ( 'NONE',  ( 0.3392501089628018884, -0.1958661417322834220, -0.6620734908136483021 ) ) ;
#74242=CARTESIAN_POINT ( 'NONE',  ( 0.3963884504522703911, 0.02578378529929774635, -1.929133858267716883 ) ) ;
#74243=CARTESIAN_POINT ( 'NONE',  ( 0.1049643490035303689, 0.3917322834645670104, -1.495406824146981117 ) ) ;
#74244=CARTESIAN_POINT ( 'NONE',  ( -0.1998031496062994405, 0.3460692066303957537, -2.609580052493438274 ) ) ;
#74253=CARTESIAN_POINT ( 'NONE',  ( -0.1998031496062994405, 0.3460692066303957537, -1.979658792650918597 ) ) ;
#74263=CARTESIAN_POINT ( 'NONE',  ( -0.1049643490035306742, 0.3917322834645668994, -1.503917692092176628 ) ) ;
#74271=CARTESIAN_POINT ( 'NONE',  ( 0.3392501089628018329, 0.1958661417322835607, -0.6004130165692406207 ) ) ;
#74273=CARTESIAN_POINT ( 'NONE',  ( 0.3808816823641231752, -0.09156050430092187165, -1.929133858267716661 ) ) ;
#74275=CARTESIAN_POINT ( 'NONE',  ( -0.1265901696524993347, 0.4724409448818895907, -2.130577427821522374 ) ) ;
#74295=CARTESIAN_POINT ( 'NONE',  ( -0.3460692066303957537, -0.1998031496062994405, -2.176509186351706315 ) ) ;
#74300=CARTESIAN_POINT ( 'NONE',  ( -9.787531504996567848E-17, 0.3996062992125986035, -1.574803149606299302 ) ) ;
#74301=CARTESIAN_POINT ( 'NONE',  ( -9.674558042662121740E-17, 0.3949938075777409963, -1.259842519685039353 ) ) ;
#74302=CARTESIAN_POINT ( 'NONE',  ( -0.2925321140481930704, -0.2925321140481933480, -2.421259842519684735 ) ) ;
#74304=CARTESIAN_POINT ( 'NONE',  ( -0.3392501089628019995, 0.1958661417322832277, -0.01837270341207344546 ) ) ;
#74308=CARTESIAN_POINT ( 'NONE',  ( -0.2891555358219909388, -0.2891555358219912164, -2.183070866141731958 ) ) ;
#74312=CARTESIAN_POINT ( 'NONE',  ( -0.3458507752293906723, -0.3458507752293910609, -2.263779527559055094 ) ) ;
#74313=CARTESIAN_POINT ( 'NONE',  ( -0.1998031496062991907, -0.3460692066303959757, -1.955380577427821454 ) ) ;
#74321=CARTESIAN_POINT ( 'NONE',  ( 0.3917322834645670104, -0.1049643490035303411, 0.1187664041994749703 ) ) ;
#74324=CARTESIAN_POINT ( 'NONE',  ( -0.1265901696524986964, -0.4724409448818899238, -2.434383202099737353 ) ) ;
#74328=CARTESIAN_POINT ( 'NONE',  ( 0.1049643490035303689, 0.3917322834645670104, -0.2355643044619422921 ) ) ;
#74330=CARTESIAN_POINT ( 'NONE',  ( -0.2867679344610364334, -0.2867679344610367109, -2.255905511811023612 ) ) ;
#74333=CARTESIAN_POINT ( 'NONE',  ( -0.2891555358219908833, -0.2891555358219912164, -2.578740157480315265 ) ) ;
#74337=CARTESIAN_POINT ( 'NONE',  ( 4.893765752498283924E-17, -0.3996062992125986035, -1.181102362204724310 ) ) ;
#74343=CARTESIAN_POINT ( 'NONE',  ( -0.3917322834645669549, -0.1049643490035306603, 0.02690288713910752097 ) ) ;
#74351=CARTESIAN_POINT ( 'NONE',  ( -0.3917322834645669549, -0.1049643490035306603, -0.1955380577427821009 ) ) ;
#74354=FACE_OUTER_BOUND ( 'NONE', #61676, .T. ) ;
#74355=SHAPE_REPRESENTATION_RELATIONSHIP ( 'NONE' , 'NONE' ,  #33107, #79614 ) ;
#74356=CARTESIAN_POINT ( 'NONE',  ( 0.4091458600556403535, 0.2362204724409449896, -1.706036745406824151 ) ) ;
#74358=CARTESIAN_POINT ( 'NONE',  ( 0.3392501089628018329, 0.1958661417322835607, -0.5958005249343831800 ) ) ;
#74363=CARTESIAN_POINT ( 'NONE',  ( 0.1265901696524990572, -0.4724409448818897017, -1.975065616797900159 ) ) ;
#74366=CARTESIAN_POINT ( 'NONE',  ( 0.3917322834645668994, -0.1049643490035303134, 0.1233788958343325359 ) ) ;
#74368=CARTESIAN_POINT ( 'NONE',  ( 0.1958661417322834775, 0.3392501089628018884, -0.2290026246719160941 ) ) ;
#74373=CARTESIAN_POINT ( 'NONE',  ( 0.3392501089628018329, 0.1958661417322835607, -2.485564304461941987 ) ) ;
#74377=CARTESIAN_POINT ( 'NONE',  ( 0.4724409448818898682, 2.892866454678787531E-17, -0.8248031496062991907 ) ) ;
#74388=CARTESIAN_POINT ( 'NONE',  ( -0.3460692066303957537, -0.1998031496062994405, -2.176509186351706315 ) ) ;
#74397=CARTESIAN_POINT ( 'NONE',  ( 0.2925321140481931814, 0.2925321140481931814, -0.2145669291338582751 ) ) ;
#74398=CARTESIAN_POINT ( 'NONE',  ( -0.1070741851644056997, 0.3996062992125986035, -0.4790026246719158998 ) ) ;
#74400=CARTESIAN_POINT ( 'NONE',  ( 0.2891555358219910499, -0.2891555358219909944, 0.05905511811023616414 ) ) ;
#74401=CARTESIAN_POINT ( 'NONE',  ( 0.02963302784745480353, -0.3970677821444032474, -8.612909436665150641E-17 ) ) ;
#74404=CARTESIAN_POINT ( 'NONE',  ( -9.787531504996567848E-17, 0.3996062992125986035, -1.920830620545185230E-17 ) ) ;
#74406=CARTESIAN_POINT ( 'NONE',  ( 0.3420746716998660508, 0.1974969037888705814, -0.9954068241469814504 ) ) ;
#74411=CARTESIAN_POINT ( 'NONE',  ( -0.4724409448818895907, -0.1265901696524993070, -0.9908136482939633449 ) ) ;
#74412=CARTESIAN_POINT ( 'NONE',  ( -0.3460692066303960868, 0.1998031496062990242, -2.230971128608923770 ) ) ;
#74415=CARTESIAN_POINT ( 'NONE',  ( 0.3392501089628018884, -0.1958661417322833942, -0.8891269273303956666 ) ) ;
#74426=CARTESIAN_POINT ( 'NONE',  ( 0.1049643490035303689, 0.3917322834645670104, -1.087926509186351476 ) ) ;
#74429=CARTESIAN_POINT ( 'NONE',  ( 0.3420746716998659953, 0.1974969037888705536, -1.391076115485564424 ) ) ;
#74447=CARTESIAN_POINT ( 'NONE',  ( 0.3996062992125986590, -0.1070741851644053111, -1.843832020997375309 ) ) ;
#74450=CARTESIAN_POINT ( 'NONE',  ( -0.3996062992125984925, -0.1070741851644056858, -1.067585301837270517 ) ) ;
#74454=CARTESIAN_POINT ( 'NONE',  ( 0.4724409448818897572, -0.1265901696524988906, -0.4265091863517060933 ) ) ;
#74456=CARTESIAN_POINT ( 'NONE',  ( -0.1958661417322834220, -0.3392501089628018884, -2.354986876640420057 ) ) ;
#74462=CARTESIAN_POINT ( 'NONE',  ( 0.4724409448818896462, 0.1265901696524990294, -2.406167979002624246 ) ) ;
#74465=CARTESIAN_POINT ( 'NONE',  ( 0.2891555358219910499, 0.2891555358219910499, -1.946850393700787496 ) ) ;
#74475=CARTESIAN_POINT ( 'NONE',  ( 0.1049643490035303689, 0.3917322834645668994, -2.593156537236534387 ) ) ;
#74489=CARTESIAN_POINT ( 'NONE',  ( -0.3996062992125985480, -7.340648628747423112E-17, -0.4311023622047244208 ) ) ;
#74491=CARTESIAN_POINT ( 'NONE',  ( -0.1958661417322834220, -0.3392501089628018884, -1.882545931758530244 ) ) ;
#74500=CARTESIAN_POINT ( 'NONE',  ( -0.3996062992125985480, -7.340648628747423112E-17, -1.375984251968504157 ) ) ;
#74508=CARTESIAN_POINT ( 'NONE',  ( 0.1958661417322836440, -0.3392501089628017219, -1.751312335958005395 ) ) ;
#74509=CARTESIAN_POINT ( 'NONE',  ( 0.4724409448818898682, 2.892866454678787531E-17, -2.165354330708661568 ) ) ;
#74512=CARTESIAN_POINT ( 'NONE',  ( 4.797336870675656522E-17, -0.3917322834645670104, -2.748031496062991685 ) ) ;
#74513=CARTESIAN_POINT ( 'NONE',  ( 0.1998031496062992463, 0.3460692066303959202, -2.425853018372703396 ) ) ;
#74515=CARTESIAN_POINT ( 'NONE',  ( -0.3460692066303958092, -0.1998031496062994683, -0.8398950131233595684 ) ) ;
#74519=CARTESIAN_POINT ( 'NONE',  ( -0.1049643490035307020, 0.3917322834645669549, -2.833333333333333037 ) ) ;
#74523=APPLICATION_CONTEXT ( 'automotive_design' ) ;
#74530=CARTESIAN_POINT ( 'NONE',  ( -0.1049643490035301746, -0.3917322834645670659, -1.569534489992439497 ) ) ;
#74534=CARTESIAN_POINT ( 'NONE',  ( -0.3917322834645671215, 0.1049643490035301469, -2.794619422572177658 ) ) ;
#74537=CARTESIAN_POINT ( 'NONE',  ( 0.3917322834645670104, 0.1049643490035304660, -2.798575746228034067 ) ) ;
#74544=EDGE_CURVE ( 'NONE', #51716, #37370, #3118, .T. ) ;
#74546=CARTESIAN_POINT ( 'NONE',  ( -0.3917322834645670104, -0.1049643490035307020, -1.459993069062679005 ) ) ;
#74548=CARTESIAN_POINT ( 'NONE',  ( -0.1958661417322834220, -0.3392501089628018884, -2.040026246719160330 ) ) ;
#74553=CARTESIAN_POINT ( 'NONE',  ( 0.2925321140481932369, 0.2925321140481932369, -0.6102362204724409711 ) ) ;
#74555=CARTESIAN_POINT ( 'NONE',  ( 0.3996062992125985480, 2.446882876249141654E-17, -0.03740157480314962313 ) ) ;
#74557=CARTESIAN_POINT ( 'NONE',  ( -0.2925321140481930704, -0.2925321140481933480, -2.263779527559055094 ) ) ;
#74562=CARTESIAN_POINT ( 'NONE',  ( -0.4724409448818899238, 0.1265901696524986686, -1.054461942257217899 ) ) ;
#74565=CARTESIAN_POINT ( 'NONE',  ( 0.3949938075777409963, 2.418639510665530743E-17, -0.6673228346456693272 ) ) ;
#74579=CARTESIAN_POINT ( 'NONE',  ( 0.3460692066303958092, 0.1998031496062993018, -1.940288713910761409 ) ) ;
#74581=CARTESIAN_POINT ( 'NONE',  ( 0.2867679344610365999, 0.2867679344610365999, -1.232283464566929387 ) ) ;
#74583=CARTESIAN_POINT ( 'NONE',  ( -0.3165741174739065689, -0.2316922116739008053, -4.446769521226833214E-17 ) ) ;
#74597=CARTESIAN_POINT ( 'NONE',  ( 0.4091458600556404646, -0.2362204724409448231, -0.3392388451443569819 ) ) ;
#74604=CARTESIAN_POINT ( 'NONE',  ( -0.2867679344610367109, 0.2867679344610365444, -2.221147924705723753 ) ) ;
#74615=CARTESIAN_POINT ( 'NONE',  ( -0.1265901696524986964, -0.4724409448818899238, 0.08530183727034119923 ) ) ;
#74616=CARTESIAN_POINT ( 'NONE',  ( 0.3420746716998660508, -0.1974969037888703871, -2.152230971128608950 ) ) ;
#74619=CARTESIAN_POINT ( 'NONE',  ( -0.1049643490035302024, -0.3917322834645671215, -0.8517060367454066805 ) ) ;
#74621=CARTESIAN_POINT ( 'NONE',  ( -0.4724409448818898682, -8.678599364036362592E-17, -2.559055118110236560 ) ) ;
#74627=CARTESIAN_POINT ( 'NONE',  ( -0.1049643490035301746, -0.3917322834645670659, -0.3096919703073997554 ) ) ;
#74631=EDGE_CURVE ( 'NONE', #59707, #80266, #70268, .T. ) ;
#74634=CARTESIAN_POINT ( 'NONE',  ( -0.1070741851644051862, -0.3996062992125987146, -2.906824146981627610 ) ) ;
#74635=CARTESIAN_POINT ( 'NONE',  ( -0.1958661417322836995, 0.3392501089628017219, -1.742145300033807631 ) ) ;
#74642=CARTESIAN_POINT ( 'NONE',  ( 0.3917322834645670104, 2.398668435337828261E-17, -1.147637795275590733 ) ) ;
#74652=CARTESIAN_POINT ( 'NONE',  ( -0.2867679344610365999, 0.2867679344610364889, -2.374015748031496287 ) ) ;
#74659=CARTESIAN_POINT ( 'NONE',  ( 0.3917322834645670104, 2.398668435337828261E-17, -0.8326771653543307838 ) ) ;
#74660=CARTESIAN_POINT ( 'NONE',  ( 0.4724409448818897572, -0.1265901696524988906, -0.03083989501312336262 ) ) ;
#74662=CARTESIAN_POINT ( 'NONE',  ( 0.2925321140481932369, 0.2925321140481932369, -2.261811023622047223 ) ) ;
#74679=CARTESIAN_POINT ( 'NONE',  ( 0.1049643490035303689, 0.3917322834645668994, -1.805754962433383737 ) ) ;
#74688=CARTESIAN_POINT ( 'NONE',  ( 0.1958661417322836718, -0.3392501089628017219, -0.4035626228684533467 ) ) ;
#74691=CARTESIAN_POINT ( 'NONE',  ( -0.4091458600556402980, -0.2362204724409451284, -2.176509186351706315 ) ) ;
#74712=CARTESIAN_POINT ( 'NONE',  ( 0.1998031496062992463, 0.3460692066303959202, -2.110892388451443669 ) ) ;
#74717=CARTESIAN_POINT ( 'NONE',  ( 0.3996062992125986035, 2.446882876249141962E-17, -1.850393700787401619 ) ) ;
#74718=CARTESIAN_POINT ( 'NONE',  ( 0.2891555358219910499, 0.2891555358219910499, -1.082677165354330784 ) ) ;
#74719=CARTESIAN_POINT ( 'NONE',  ( -0.3460692066303960868, 0.1998031496062990242, -2.545931758530183497 ) ) ;
#74721=CARTESIAN_POINT ( 'NONE',  ( 0.1958661417322834775, 0.3392501089628018884, -0.4514435695538057125 ) ) ;
#74725=CARTESIAN_POINT ( 'NONE',  ( -0.1058382717557497660, -0.3949938075777411073, -2.353674540682414218 ) ) ;
#74728=CARTESIAN_POINT ( 'NONE',  ( -0.1265901696524986964, -0.4724409448818899238, -2.434383202099737353 ) ) ;
#74729=CARTESIAN_POINT ( 'NONE',  ( 0.1998031496062994405, -0.3460692066303958092, -1.824146981627296604 ) ) ;
#74736=CARTESIAN_POINT ( 'NONE',  ( -9.594673741351310580E-17, 0.3917322834645669549, -2.757198531987190115 ) ) ;
#74743=CARTESIAN_POINT ( 'NONE',  ( 0.1049643490035304938, -0.3917322834645669549, -0.1699475065616798397 ) ) ;
#74745=( BOUNDED_CURVE ( )  B_SPLINE_CURVE ( 2, ( #82157, #56042, #49730, #31611, #25289, #18985, #24877, #50139, #75429, #69515, #11864, #5532, #18583 ),
 .UNSPECIFIED., .F., .F. ) 
 B_SPLINE_CURVE_WITH_KNOTS ( ( 3, 2, 2, 2, 2, 2, 3 ),
 ( 0.2125000000000000222, 0.2166666666666667018, 0.2208333333333333537, 0.2250000000000000333, 0.2291666666666666852, 0.2333333333333333648, 0.2375000000000000167 ),
 .UNSPECIFIED. ) 
 CURVE ( )  GEOMETRIC_REPRESENTATION_ITEM ( )  RATIONAL_B_SPLINE_CURVE ( ( 0.9999999999999997780, 0.9659258262890685343, 1.000000000000000000, 0.9659258262890683122, 1.000000000000000000, 0.9659258262890683122, 1.000000000000000000, 0.9659258262890683122, 1.000000000000000000, 0.9659258262890683122, 1.000000000000000000, 0.9659258262890680902, 1.000000000000000222 ) ) 
 REPRESENTATION_ITEM ( '' )  );
#74746=CARTESIAN_POINT ( 'NONE',  ( -9.594673741351313045E-17, 0.3917322834645670104, -2.196850393700787496 ) ) ;
#74749=CARTESIAN_POINT ( 'NONE',  ( 4.837279021331060870E-17, -0.3949938075777409963, -2.598425196850393970 ) ) ;
#74754=CARTESIAN_POINT ( 'NONE',  ( -0.3996062992125986035, -7.340648628747425578E-17, -1.141732283464566899 ) ) ;
#74759=CARTESIAN_POINT ( 'NONE',  ( 0.3917322834645669549, 0.1049643490035304660, -0.5242782152230972548 ) ) ;
#74765=CARTESIAN_POINT ( 'NONE',  ( 0.3917322834645670104, -0.1049643490035303411, -0.1036745406824146343 ) ) ;
#74767=ADVANCED_FACE ( 'NONE', ( #1915 ), #78107, .T. ) ;
#74770=CARTESIAN_POINT ( 'NONE',  ( -0.2362204724409447953, -0.4091458600556404646, -1.482939632545931863 ) ) ;
#74772=EDGE_CURVE ( 'NONE', #83292, #47997, #39368, .T. ) ;
#74776=CARTESIAN_POINT ( 'NONE',  ( -0.3458507752293906723, -0.3458507752293910609, -2.263779527559055094 ) ) ;
#74780=CARTESIAN_POINT ( 'NONE',  ( 0.1049643490035303689, 0.3917322834645668994, -0.2309518128270847681 ) ) ;
#74782=CARTESIAN_POINT ( 'NONE',  ( 4.797336870675656522E-17, -0.3917322834645670104, -0.3208661417322835607 ) ) ;
#74787=CARTESIAN_POINT ( 'NONE',  ( -0.1958661417322836718, 0.3392501089628017219, -2.524934383202099397 ) ) ;
#74792=CARTESIAN_POINT ( 'NONE',  ( 0.4724409448818897572, -0.1265901696524988906, -0.6607611548556431291 ) ) ;
#74805=CARTESIAN_POINT ( 'NONE',  ( -0.3460692066303957537, -0.1998031496062994405, -1.861548556430446144 ) ) ;
#74815=CARTESIAN_POINT ( 'NONE',  ( -0.3996062992125984925, -0.1070741851644056719, -0.1227034120734908362 ) ) ;
#74816=CARTESIAN_POINT ( 'NONE',  ( -0.1070741851644056997, 0.3996062992125986035, -0.6364829396325458744 ) ) ;
#74817=CARTESIAN_POINT ( 'NONE',  ( -0.3917322834645670104, -0.1049643490035307020, -2.877315903708348444 ) ) ;
#74823=CARTESIAN_POINT ( 'NONE',  ( 0.3420746716998660508, 0.1974969037888705814, -0.8379265091863515869 ) ) ;
#74828=CARTESIAN_POINT ( 'NONE',  ( -0.3458507752293906723, -0.3458507752293910609, -1.003937007874015741 ) ) ;
#74829=CARTESIAN_POINT ( 'NONE',  ( 0.1070741851644053666, 0.3996062992125986035, -2.198162729658792447 ) ) ;
#74832=ORIENTED_EDGE ( 'NONE', *, *, #55159, .F. ) ;
#74833=CARTESIAN_POINT ( 'NONE',  ( 4.797336870675656522E-17, -0.3917322834645670659, -0.7053998932096606778 ) ) ;
#74845=CARTESIAN_POINT ( 'NONE',  ( 0.1958661417322834775, 0.3392501089628018884, -1.238845144356955252 ) ) ;
#74847=ORIENTED_EDGE ( 'NONE', *, *, #33021, .F. ) ;
#74848=CARTESIAN_POINT ( 'NONE',  ( 4.837279021331060870E-17, -0.3949938075777409963, -1.653543307086614123 ) ) ;
#74861=CARTESIAN_POINT ( 'NONE',  ( -0.3392501089628019995, 0.1958661417322832277, 0.2040682414698161695 ) ) ;
#74866=CARTESIAN_POINT ( 'NONE',  ( 0.3460692066303959757, -0.1998031496062991907, -1.994750656167979086 ) ) ;
#74869=CARTESIAN_POINT ( 'NONE',  ( 4.893765752498283308E-17, -0.3996062992125985480, -1.572834645669291431 ) ) ;
#74873=CARTESIAN_POINT ( 'NONE',  ( 0.4724409448818896462, 0.1265901696524990294, -0.5971128608923884640 ) ) ;
#74875=CARTESIAN_POINT ( 'NONE',  ( 0.3917322834645670104, -0.1049643490035303411, -2.400918635170603554 ) ) ;
#74881=CARTESIAN_POINT ( 'NONE',  ( -0.1265901696524993347, 0.4724409448818895907, -2.288057742782152015 ) ) ;
#74883=CARTESIAN_POINT ( 'NONE',  ( -0.1058382717557503072, 0.3949938075777408852, -2.130577427821521930 ) ) ;
#74903=CARTESIAN_POINT ( 'NONE',  ( 0.1070741851644053388, 0.3996062992125986035, -0.8576115485564304031 ) ) ;
#74905=CARTESIAN_POINT ( 'NONE',  ( 0.1049643490035303689, 0.3917322834645670104, -1.967847769028871374 ) ) ;
#74917=CARTESIAN_POINT ( 'NONE',  ( 0.2925321140481932369, 0.2925321140481932369, -1.474409448818897905 ) ) ;
#74925=CARTESIAN_POINT ( 'NONE',  ( -0.3917322834645671215, 0.1049643490035301469, -1.692257217847769057 ) ) ;
#74930=CARTESIAN_POINT ( 'NONE',  ( 0.3460692066303958092, 0.1998031496062993018, -2.255249343832021136 ) ) ;
#74932=CARTESIAN_POINT ( 'NONE',  ( 0.2925321140481932369, 0.2925321140481932369, -0.7677165354330709457 ) ) ;
#74935=CARTESIAN_POINT ( 'NONE',  ( -0.3917322834645671215, 0.1049643490035301469, -2.544619422572177658 ) ) ;
#74936=ORIENTED_EDGE ( 'NONE', *, *, #2885, .F. ) ;
#74945=CARTESIAN_POINT ( 'NONE',  ( 0.1049643490035303689, 0.3917322834645668994, -1.805754962433383737 ) ) ;
#74948=CARTESIAN_POINT ( 'NONE',  ( -0.1049643490035302024, -0.3917322834645671215, 0.09317585301837273681 ) ) ;
#74951=CARTESIAN_POINT ( 'NONE',  ( -0.1058382717557503211, 0.3949938075777409408, -0.1640419947506562559 ) ) ;
#74953=ORIENTED_EDGE ( 'NONE', *, *, #35152, .T. ) ;
#74959=CARTESIAN_POINT ( 'NONE',  ( 0.1049643490035303967, 0.3917322834645670659, -1.407499630742469199 ) ) ;
#74961=CARTESIAN_POINT ( 'NONE',  ( 0.1958661417322836440, -0.3392501089628017219, -2.853674540682414662 ) ) ;
#74966=CARTESIAN_POINT ( 'NONE',  ( 0.2925321140481932369, -0.2925321140481932369, -0.8858267716535430658 ) ) ;
#74968=CARTESIAN_POINT ( 'NONE',  ( -0.3996062992125985480, -7.340648628747423112E-17, -0.1161417322834645827 ) ) ;
#74970=CARTESIAN_POINT ( 'NONE',  ( -0.1070741851644056997, 0.3996062992125986035, -2.368766404199475151 ) ) ;
#74976=CARTESIAN_POINT ( 'NONE',  ( -0.2362204724409447953, -0.4091458600556404646, -1.244750656167979086 ) ) ;
#74979=CARTESIAN_POINT ( 'NONE',  ( 0.3949938075777409408, -0.1058382717557499186, -0.6607611548556431291 ) ) ;
#74992=CARTESIAN_POINT ( 'NONE',  ( -0.1070741851644056997, 0.3996062992125984925, -1.658136482939632339 ) ) ;
#74994=CARTESIAN_POINT ( 'NONE',  ( -0.3917322834645669549, -0.1049643490035306603, -1.455380577427821676 ) ) ;
#74996=CARTESIAN_POINT ( 'NONE',  ( -0.1906283239483360925, -0.3428707098288028554, -2.110585413283057979E-17 ) ) ;
#75016=CARTESIAN_POINT ( 'NONE',  ( 0.1958661417322834775, 0.3392501089628018884, -2.030859210794962344 ) ) ;
#75024=CARTESIAN_POINT ( 'NONE',  ( -0.3917322834645670104, -7.196005306013484475E-17, -2.078740157480314821 ) ) ;
#75028=CARTESIAN_POINT ( 'NONE',  ( -0.1265901696524993347, 0.4724409448818895907, -0.1640419947506561726 ) ) ;
#75029=CARTESIAN_POINT ( 'NONE',  ( -0.1974969037888706647, 0.3420746716998658843, -2.847769028871391495 ) ) ;
#75032=CARTESIAN_POINT ( 'NONE',  ( -0.2867679344610364334, -0.2867679344610367109, -1.468503937007874294 ) ) ;
#75034=CARTESIAN_POINT ( 'NONE',  ( -0.3458507752293906723, -0.3458507752293910609, -2.578740157480315265 ) ) ;
#75039=CARTESIAN_POINT ( 'NONE',  ( -0.1958661417322834497, -0.3392501089628018884, -0.9330515503598931781 ) ) ;
#75044=FACE_OUTER_BOUND ( 'NONE', #6282, .T. ) ;
#75046=CARTESIAN_POINT ( 'NONE',  ( -0.1049643490035302301, -0.3917322834645671770, -2.116161048065303696 ) ) ;
#75052=CARTESIAN_POINT ( 'NONE',  ( 0.3392501089628018329, 0.1958661417322835607, -0.8458005249343831800 ) ) ;
#75061=CARTESIAN_POINT ( 'NONE',  ( 0.3392501089628018884, -0.1958661417322834220, -2.774278215223096922 ) ) ;
#75068=CARTESIAN_POINT ( 'NONE',  ( 0.3917322834645670104, 2.398668435337828261E-17, -0.9901574803149607584 ) ) ;
#75069=CARTESIAN_POINT ( 'NONE',  ( -0.4724409448818899238, 0.1265901696524986686, 0.2053805774278214813 ) ) ;
#75071=CARTESIAN_POINT ( 'NONE',  ( 0.3996062992125986035, -0.1070741851644052972, -2.235564304461942431 ) ) ;
#75080=CARTESIAN_POINT ( 'NONE',  ( -0.2925321140481930149, -0.2925321140481933480, -0.2933070866141732069 ) ) ;
#75082=CARTESIAN_POINT ( 'NONE',  ( -0.1958661417322834220, -0.3392501089628018884, -0.05774278215223092176 ) ) ;
#75089=CARTESIAN_POINT ( 'NONE',  ( 0.3917322834645669549, 2.398668435337827645E-17, -1.615466248522622550 ) ) ;
#75098=CARTESIAN_POINT ( 'NONE',  ( 0.1049643490035304799, -0.3917322834645670104, -0.3970009430784271487 ) ) ;
#75103=CARTESIAN_POINT ( 'NONE',  ( -0.4091458600556405756, 0.2362204724409446288, -1.992782152230971437 ) ) ;
#75107=( BOUNDED_CURVE ( )  B_SPLINE_CURVE ( 2, ( #65434, #1449, #65843, #27106, #21626, #51931, #79308, #72976, #27941, #47287, #78894, #7336, #39738 ),
 .UNSPECIFIED., .F., .F. ) 
 B_SPLINE_CURVE_WITH_KNOTS ( ( 3, 2, 2, 2, 2, 2, 3 ),
 ( 0.2375000000000000167, 0.2416666666666666963, 0.2458333333333333204, 0.2500000000000000000, 0.2541666666666666519, 0.2583333333333333037, 0.2624999999999999556 ),
 .UNSPECIFIED. ) 
 CURVE ( )  GEOMETRIC_REPRESENTATION_ITEM ( )  RATIONAL_B_SPLINE_CURVE ( ( 0.9999999999999997780, 0.9659258262890685343, 1.000000000000000000, 0.9659258262890683122, 1.000000000000000000, 0.9659258262890683122, 1.000000000000000000, 0.9659258262890683122, 1.000000000000000000, 0.9659258262890683122, 1.000000000000000000, 0.9659258262890687563, 0.9999999999999995559 ) ) 
 REPRESENTATION_ITEM ( '' )  );
#75114=EDGE_CURVE ( 'NONE', #54535, #7865, #67539, .T. ) ;
#75125=CARTESIAN_POINT ( 'NONE',  ( 0.2925321140481932369, 0.2925321140481932369, -2.261811023622047223 ) ) ;
#75130=CARTESIAN_POINT ( 'NONE',  ( 0.3460692066303959757, -0.1998031496062991907, -1.837270341207349000 ) ) ;
#75131=CARTESIAN_POINT ( 'NONE',  ( 0.2891555358219910499, 0.2891555358219910499, -1.712598425196850682 ) ) ;
#75134=CARTESIAN_POINT ( 'NONE',  ( -0.3392501089628019995, 0.1958661417322832277, -0.6482939632545930975 ) ) ;
#75138=CARTESIAN_POINT ( 'NONE',  ( -0.3949938075777411073, 0.1058382717557497660, -1.999343832020997747 ) ) ;
#75142=CARTESIAN_POINT ( 'NONE',  ( -0.4724409448818899238, 0.1265901696524986686, -2.395013123359580387 ) ) ;
#75143=CARTESIAN_POINT ( 'NONE',  ( -9.787531504996567848E-17, 0.3996062992125986035, -1.732283464566929165 ) ) ;
#75144=CARTESIAN_POINT ( 'NONE',  ( 0.4724409448818897017, 0.1265901696524990294, -2.721128608923884862 ) ) ;
#75150=CARTESIAN_POINT ( 'NONE',  ( 0.2867679344610365999, -0.2867679344610365999, -2.855623728837584085 ) ) ;
#75157=CARTESIAN_POINT ( 'NONE',  ( -0.3392501089628019995, 0.1958661417322832277, -0.2683727034120735877 ) ) ;
#75159=CARTESIAN_POINT ( 'NONE',  ( 4.797336870675656522E-17, -0.3917322834645670104, -2.118110236220472675 ) ) ;
#75162=CARTESIAN_POINT ( 'NONE',  ( -0.3949938075777411628, 0.1058382717557497937, -2.709973753280840114 ) ) ;
#75166=CARTESIAN_POINT ( 'NONE',  ( 0.3996062992125986035, 2.446882876249141962E-17, -1.220472440944881942 ) ) ;
#75168=CARTESIAN_POINT ( 'NONE',  ( 0.3458507752293908943, -0.3458507752293908943, -0.8051181102362204856 ) ) ;
#75171=CARTESIAN_POINT ( 'NONE',  ( 0.1958661417322836440, -0.3392501089628017219, -0.4914698162729659869 ) ) ;
#75177=CARTESIAN_POINT ( 'NONE',  ( 0.2867679344610365999, -0.2867679344610365444, -0.09055118110236216877 ) ) ;
#75181=CARTESIAN_POINT ( 'NONE',  ( -0.2362204724409451284, 0.4091458600556402425, -1.745406824146981561 ) ) ;
#75183=CARTESIAN_POINT ( 'NONE',  ( 0.2362204724409449064, 0.4091458600556404646, -0.9317585301837270073 ) ) ;
#75187=CARTESIAN_POINT ( 'NONE',  ( -0.3458507752293906723, -0.3458507752293910609, -1.948818897637795144 ) ) ;
#75191=CARTESIAN_POINT ( 'NONE',  ( 0.3917322834645668994, 0.1049643490035304522, -0.5196657235882398140 ) ) ;
#75193=CARTESIAN_POINT ( 'NONE',  ( 0.2867679344610366554, 0.2867679344610366554, -0.5374015748031496509 ) ) ;
#75198=CARTESIAN_POINT ( 'NONE',  ( 0.3917322834645670104, -0.1049643490035303411, -2.308398950131233640 ) ) ;
#75201=CARTESIAN_POINT ( 'NONE',  ( -0.4091458600556405756, 0.2362204724409446288, -0.8904199475065617264 ) ) ;
#75209=CARTESIAN_POINT ( 'NONE',  ( -0.4724409448818898682, -8.678599364036362592E-17, -0.3543307086614173040 ) ) ;
#75211=ORIENTED_EDGE ( 'NONE', *, *, #47963, .F. ) ;
#75212=CARTESIAN_POINT ( 'NONE',  ( 0.3996062992125984925, 0.1070741851644054637, -1.776246719160104570 ) ) ;
#75220=CARTESIAN_POINT ( 'NONE',  ( -0.2925321140481930149, -0.2925321140481933480, -0.4507874015748031815 ) ) ;
#75221=CARTESIAN_POINT ( 'NONE',  ( -0.3460692066303958092, -0.1998031496062994683, -0.6824146981627295938 ) ) ;
#75222=CARTESIAN_POINT ( 'NONE',  ( 0.2891555358219910499, 0.2891555358219910499, -0.2952755905511811885 ) ) ;
#75228=CARTESIAN_POINT ( 'NONE',  ( -9.674558042662122972E-17, 0.3949938075777409963, -0.8641732283464566011 ) ) ;
#75230=( BOUNDED_CURVE ( )  B_SPLINE_CURVE ( 2, ( #45990, #79681, #47658, #14038, #59465, #1406, #2232, #78432, #8961, #39695, #53968, #65386, #1816 ),
 .UNSPECIFIED., .F., .F. ) 
 B_SPLINE_CURVE_WITH_KNOTS ( ( 3, 2, 2, 2, 2, 2, 3 ),
 ( 0.6875000000000000000, 0.6916666666666666519, 0.6958333333333333037, 0.6999999999999999556, 0.7041666666666666075, 0.7083333333333332593, 0.7124999999999999112 ),
 .UNSPECIFIED. ) 
 CURVE ( )  GEOMETRIC_REPRESENTATION_ITEM ( )  RATIONAL_B_SPLINE_CURVE ( ( 1.000000000000000000, 0.9659258262890683122, 1.000000000000000000, 0.9659258262890683122, 1.000000000000000000, 0.9659258262890683122, 1.000000000000000000, 0.9659258262890683122, 1.000000000000000000, 0.9659258262890683122, 1.000000000000000000, 0.9659258262890692004, 0.9999999999999991118 ) ) 
 REPRESENTATION_ITEM ( '' )  );
#75234=CARTESIAN_POINT ( 'NONE',  ( 0.3458507752293908943, -0.3458507752293908943, -1.358267716535433101 ) ) ;
#75235=CARTESIAN_POINT ( 'NONE',  ( -0.3996062992125986035, -7.340648628747425578E-17, -2.401574803149606474 ) ) ;
#75237=ORIENTED_EDGE ( 'NONE', *, *, #71143, .F. ) ;
#75238=CARTESIAN_POINT ( 'NONE',  ( 0.1049643490035303967, 0.3917322834645670659, -0.7775783708999494115 ) ) ;
#75250=CARTESIAN_POINT ( 'NONE',  ( -0.1958661417322834220, -0.3392501089628018884, -1.160104986876640210 ) ) ;
#75253=CARTESIAN_POINT ( 'NONE',  ( -0.1974969037888703871, -0.3420746716998661063, -1.482939632545931863 ) ) ;
#75258=CARTESIAN_POINT ( 'NONE',  ( -0.1998031496062991907, -0.3460692066303959757, 0.09186351706036742504 ) ) ;
#75266=CARTESIAN_POINT ( 'NONE',  ( 0.2867679344610365999, -0.2867679344610365444, 0.1318897637795274913 ) ) ;
#75272=CARTESIAN_POINT ( 'NONE',  ( -0.1070741851644051862, -0.3996062992125987146, -2.119422572178477626 ) ) ;
#75275=CARTESIAN_POINT ( 'NONE',  ( 0.1998031496062992463, 0.3460692066303959202, -1.480971128608923548 ) ) ;
#75279=CARTESIAN_POINT ( 'NONE',  ( 0.4091458600556403535, 0.2362204724409449896, -0.6036745406824146620 ) ) ;
#75281=CARTESIAN_POINT ( 'NONE',  ( 0.3392501089628018884, -0.1958661417322834220, -2.866797900262466836 ) ) ;
#75287=CARTESIAN_POINT ( 'NONE',  ( 0.1265901696524990294, -0.4724409448818896462, -2.366797900262467280 ) ) ;
#75289=CARTESIAN_POINT ( 'NONE',  ( -0.3949938075777408852, -0.1058382717557502933, -2.169947506561679784 ) ) ;
#75295=CARTESIAN_POINT ( 'NONE',  ( -0.2362204724409447953, -0.4091458600556404646, -2.189632545931758489 ) ) ;
#75309=CARTESIAN_POINT ( 'NONE',  ( -0.2925321140481932369, 0.2925321140481931259, -0.7263779527559056648 ) ) ;
#75310=CARTESIAN_POINT ( 'NONE',  ( -0.3917322834645669549, -0.1049643490035306603, -2.335301837270341352 ) ) ;
#75326=CARTESIAN_POINT ( 'NONE',  ( 0.1958661417322836440, -0.3392501089628017219, -1.436351706036745446 ) ) ;
#75327=CARTESIAN_POINT ( 'NONE',  ( -0.06766049032609942893, 0.3859888145977988794, -1.220472440944881498 ) ) ;
#75330=CARTESIAN_POINT ( 'NONE',  ( -0.2362204724409451284, 0.4091458600556402425, -0.4855643044619422644 ) ) ;
#75331=CARTESIAN_POINT ( 'NONE',  ( -0.1998031496062991630, -0.3460692066303959202, -2.189632545931758489 ) ) ;
#75333=CARTESIAN_POINT ( 'NONE',  ( -0.1070741851644051862, -0.3996062992125987146, -1.017060367454067915 ) ) ;
#75336=CARTESIAN_POINT ( 'NONE',  ( 0.1049643490035304938, -0.3917322834645669549, -2.754593175853017328 ) ) ;
#75348=CARTESIAN_POINT ( 'NONE',  ( 0.2867679344610365999, -0.2867679344610365444, -2.702755905511810663 ) ) ;
#75351=CARTESIAN_POINT ( 'NONE',  ( -9.674558042662121740E-17, 0.3949938075777409963, -0.1574803149606300023 ) ) ;
#75359=CARTESIAN_POINT ( 'NONE',  ( -0.1958661417322836995, 0.3392501089628017219, -1.269704355151917818 ) ) ;
#75361=CARTESIAN_POINT ( 'NONE',  ( -0.1049643490035302024, -0.3917322834645671215, -2.676509186351705871 ) ) ;
#75367=CARTESIAN_POINT ( 'NONE',  ( -0.3460692066303960868, 0.1998031496062990242, -0.6561679790026246906 ) ) ;
#75369=CARTESIAN_POINT ( 'NONE',  ( -0.3996062992125984925, -0.1070741851644056858, -0.1227034120734908362 ) ) ;
#75372=CARTESIAN_POINT ( 'NONE',  ( -0.1998031496062991907, -0.3460692066303959757, -2.112860892388451539 ) ) ;
#75376=CARTESIAN_POINT ( 'NONE',  ( -0.4724409448818895907, -0.1265901696524993070, -1.067585301837270517 ) ) ;
#75380=CARTESIAN_POINT ( 'NONE',  ( -0.2891555358219909388, -0.2891555358219912164, -0.9232283464566930498 ) ) ;
#75382=CARTESIAN_POINT ( 'NONE',  ( -0.2362204724409447953, -0.4091458600556404646, -1.087270341207349000 ) ) ;
#75384=EDGE_CURVE ( 'NONE', #32899, #52886, #48588, .T. ) ;
#75394=DIRECTION ( 'NONE',  ( 0.000000000000000000, 0.000000000000000000, 1.000000000000000000 ) ) ;
#75395=CARTESIAN_POINT ( 'NONE',  ( -0.3460692066303960313, 0.1998031496062989965, -1.677821522309711488 ) ) ;
#75397=CARTESIAN_POINT ( 'NONE',  ( 0.2867679344610365999, 0.2867679344610365999, -1.547244094488189115 ) ) ;
#75412=CARTESIAN_POINT ( 'NONE',  ( 0.3392501089628018329, 0.1958661417322835607, -1.160761154855643129 ) ) ;
#75429=CARTESIAN_POINT ( 'NONE',  ( 0.2362204724409451007, -0.4091458600556402980, -0.5643044619422572516 ) ) ;
#75431=CARTESIAN_POINT ( 'NONE',  ( 0.2925321140481932369, -0.2925321140481931814, -1.200787401574802793 ) ) ;
#75433=CARTESIAN_POINT ( 'NONE',  ( -0.1049643490035301885, -0.3917322834645671215, -2.111548556430446144 ) ) ;
#75437=CARTESIAN_POINT ( 'NONE',  ( 5.785732909357575061E-17, -0.4724409448818898682, -0.2362204724409449064 ) ) ;
#75438=CARTESIAN_POINT ( 'NONE',  ( -0.1058382717557497937, -0.3949938075777411628, -2.749343832020997969 ) ) ;
#75441=CARTESIAN_POINT ( 'NONE',  ( 0.3392501089628018884, -0.1958661417322834220, -1.199475065616797842 ) ) ;
#75443=CARTESIAN_POINT ( 'NONE',  ( 0.2362204724409449064, 0.4091458600556404646, -2.664041994750656173 ) ) ;
#75450=CARTESIAN_POINT ( 'NONE',  ( -0.3917322834645668994, -0.1049643490035306742, -0.7558861960291846094 ) ) ;
#75458=CARTESIAN_POINT ( 'NONE',  ( 0.3392501089628018329, 0.1958661417322835607, -1.860255536254279862 ) ) ;
#75464=CARTESIAN_POINT ( 'NONE',  ( 0.3917322834645670104, 2.398668435337828261E-17, -1.462598425196850460 ) ) ;
#75474=CARTESIAN_POINT ( 'NONE',  ( -0.3917322834645670104, -7.196005306013484475E-17, -2.708661417322834275 ) ) ;
#75481=CARTESIAN_POINT ( 'NONE',  ( -0.1958661417322836718, 0.3392501089628017219, -0.7276902887139108378 ) ) ;
#75482=CARTESIAN_POINT ( 'NONE',  ( 0.4724409448818896462, 0.1265901696524990294, 0.1135170603674540563 ) ) ;
#75485=CARTESIAN_POINT ( 'NONE',  ( -0.3996062992125984925, -0.1070741851644056858, -2.799868766404198794 ) ) ;
#75495=CARTESIAN_POINT ( 'NONE',  ( 0.3996062992125986035, -0.1070741851644052972, -0.3458005249343831244 ) ) ;
#75497=CARTESIAN_POINT ( 'NONE',  ( 0.1958661417322834775, 0.3392501089628018884, -0.1364829396325459021 ) ) ;
#75500=FACE_OUTER_BOUND ( 'NONE', #38254, .T. ) ;
#75504=CARTESIAN_POINT ( 'NONE',  ( -0.1049643490035306742, 0.3917322834645668994, -1.661398007052806269 ) ) ;
#75513=CARTESIAN_POINT ( 'NONE',  ( 0.2867679344610366554, -0.2867679344610365999, -0.8825652475403695796 ) ) ;
#75517=CARTESIAN_POINT ( 'NONE',  ( 0.4091458600556404646, -0.2362204724409448231, -2.071522309711285814 ) ) ;
#75531=ORIENTED_EDGE ( 'NONE', *, *, #15762, .F. ) ;
#75535=CARTESIAN_POINT ( 'NONE',  ( 0.2925321140481932369, -0.2925321140481931814, -0.09842519685039372024 ) ) ;
#75536=CARTESIAN_POINT ( 'NONE',  ( 0.1070741851644053388, 0.3996062992125986035, -2.432414698162729039 ) ) ;
#75541=CARTESIAN_POINT ( 'NONE',  ( 0.3460692066303959757, -0.1998031496062991907, -2.309711286089239035 ) ) ;
#75542=CARTESIAN_POINT ( 'NONE',  ( -0.3949938075777411628, 0.1058382717557497937, -1.607611548556430847 ) ) ;
#75545=CARTESIAN_POINT ( 'NONE',  ( 0.2867679344610366554, 0.2867679344610366554, -0.6023622047244093780 ) ) ;
#75550=CARTESIAN_POINT ( 'NONE',  ( 0.1974969037888706092, -0.3420746716998660508, -2.688320209973753094 ) ) ;
#75554=CARTESIAN_POINT ( 'NONE',  ( 0.3458507752293908943, -0.3458507752293908943, -2.933070866141732402 ) ) ;
#75555=CARTESIAN_POINT ( 'NONE',  ( -0.3460692066303960868, 0.1998031496062990242, -2.230971128608923770 ) ) ;
#75562=CARTESIAN_POINT ( 'NONE',  ( -0.3392501089628017219, -0.1958661417322836718, -0.1371391076115486551 ) ) ;
#75569=CARTESIAN_POINT ( 'NONE',  ( 0.1049643490035303689, 0.3917322834645670104, -0.3930446194225722945 ) ) ;
#75571=CARTESIAN_POINT ( 'NONE',  ( 0.2867679344610365999, -0.2867679344610365444, -1.507874015748031260 ) ) ;
#75572=CARTESIAN_POINT ( 'NONE',  ( -0.1958661417322834220, -0.3392501089628018884, -2.577427821522309426 ) ) ;
#75574=ORIENTED_EDGE ( 'NONE', *, *, #48087, .F. ) ;
#75575=CARTESIAN_POINT ( 'NONE',  ( 0.2891555358219910499, -0.2891555358219909944, -2.618110236220472675 ) ) ;
#75576=ORIENTED_EDGE ( 'NONE', *, *, #6890, .F. ) ;
#75579=CARTESIAN_POINT ( 'NONE',  ( -0.3996062992125986035, -0.1070741851644056997, -1.305774278215223072 ) ) ;
#75584=CARTESIAN_POINT ( 'NONE',  ( -0.1049643490035302024, -0.3917322834645671215, -0.3143044619422573072 ) ) ;
#75594=CARTESIAN_POINT ( 'NONE',  ( 0.2362204724409451007, -0.4091458600556402980, -1.824146981627296604 ) ) ;
#75604=CARTESIAN_POINT ( 'NONE',  ( -0.2867679344610366554, 0.2867679344610365444, -0.4146788469478197015 ) ) ;
#75606=CARTESIAN_POINT ( 'NONE',  ( 0.1958661417322836440, -0.3392501089628017219, -0.8064304461942258806 ) ) ;
#75612=CARTESIAN_POINT ( 'NONE',  ( 4.797336870675656522E-17, -0.3917322834645670104, -2.748031496062991685 ) ) ;
#75615=CARTESIAN_POINT ( 'NONE',  ( 0.3458507752293908943, 0.3458507752293908943, -0.8444881889763780070 ) ) ;
#75627=CARTESIAN_POINT ( 'NONE',  ( -0.2925321140481932369, 0.2925321140481931259, -1.986220472440944906 ) ) ;
#75635=CARTESIAN_POINT ( 'NONE',  ( 0.1070741851644053527, 0.3996062992125985480, -0.8576115485564304031 ) ) ;
#75636=CARTESIAN_POINT ( 'NONE',  ( 0.1998031496062994405, -0.3460692066303958092, -1.036745406824147064 ) ) ;
#75637=CARTESIAN_POINT ( 'NONE',  ( -0.3949938075777409963, -7.255918531996591613E-17, -0.03937007874015754222 ) ) ;
#75643=CARTESIAN_POINT ( 'NONE',  ( -0.1974969037888704149, -0.3420746716998661063, -1.402230971128609172 ) ) ;
#75648=CARTESIAN_POINT ( 'NONE',  ( -0.2362204724409447953, -0.4091458600556404646, -1.167979002624671914 ) ) ;
#75649=CARTESIAN_POINT ( 'NONE',  ( -0.3996062992125986590, 0.1070741851644051862, -2.709973753280840114 ) ) ;
#75651=ORIENTED_EDGE ( 'NONE', *, *, #9813, .F. ) ;
#75652=CARTESIAN_POINT ( 'NONE',  ( -9.594673741351313045E-17, 0.3917322834645670659, -0.9416203656506056952 ) ) ;
#75663=CARTESIAN_POINT ( 'NONE',  ( -0.1049643490035302024, -0.3917322834645671215, -1.009186351706036433 ) ) ;
#75666=CARTESIAN_POINT ( 'NONE',  ( -0.3949938075777409408, -0.1058382717557502933, -1.620734908136483243 ) ) ;
#75671=CARTESIAN_POINT ( 'NONE',  ( -0.3460692066303960868, 0.1998031496062990242, -0.02624671916010499692 ) ) ;
#75674=CARTESIAN_POINT ( 'NONE',  ( 0.3996062992125986035, 2.446882876249141962E-17, -1.220472440944881942 ) ) ;
#75678=CARTESIAN_POINT ( 'NONE',  ( -0.2867679344610364334, -0.2867679344610367109, -0.1437007874015748810 ) ) ;
#75684=CARTESIAN_POINT ( 'NONE',  ( -0.3460692066303960868, 0.1998031496062990242, -2.230971128608923770 ) ) ;
#75687=CARTESIAN_POINT ( 'NONE',  ( 0.3460692066303958092, 0.1998031496062993018, -1.782808398950131101 ) ) ;
#75688=CARTESIAN_POINT ( 'NONE',  ( -0.03143970413924313673, 0.3977953519386766557, -2.755905511811078679 ) ) ;
#75691=CARTESIAN_POINT ( 'NONE',  ( -0.4091458600556405756, 0.2362204724409446288, -0.3412073490813647969 ) ) ;
#75693=CARTESIAN_POINT ( 'NONE',  ( 0.1958661417322836440, -0.3392501089628017219, -2.853674540682414662 ) ) ;
#75699=CARTESIAN_POINT ( 'NONE',  ( 0.4091458600556403535, 0.2362204724409449896, -2.255249343832020692 ) ) ;
#75701=CARTESIAN_POINT ( 'NONE',  ( -0.1058382717557503072, 0.3949938075777408852, -2.288057742782152459 ) ) ;
#75708=CARTESIAN_POINT ( 'NONE',  ( 0.4724409448818898682, 2.892866454678787531E-17, -2.242125984251968518 ) ) ;
#75713=CARTESIAN_POINT ( 'NONE',  ( -1.157146581871515012E-16, 0.4724409448818898682, -1.021653543307086576 ) ) ;
#75724=CARTESIAN_POINT ( 'NONE',  ( -0.3460692066303957537, -0.1998031496062994405, -0.7591863517060367661 ) ) ;
#75725=CARTESIAN_POINT ( 'NONE',  ( 0.1958661417322834775, 0.3392501089628018884, -2.433727034120734878 ) ) ;
#75734=CARTESIAN_POINT ( 'NONE',  ( -1.157146581871515012E-16, 0.4724409448818898682, -2.204724409448818978 ) ) ;
#75740=CARTESIAN_POINT ( 'NONE',  ( -0.3917322834645671215, 0.1049643490035301469, -1.377296587926508664 ) ) ;
#75744=DIRECTION ( 'NONE',  ( -0.000000000000000000, -0.000000000000000000, 1.000000000000000000 ) ) ;
#75745=CARTESIAN_POINT ( 'NONE',  ( 0.1998031496062994128, -0.3460692066303957537, -2.373359580052493367 ) ) ;
#75748=CARTESIAN_POINT ( 'NONE',  ( 0.1998031496062994405, -0.3460692066303958092, -1.036745406824147064 ) ) ;
#75750=CARTESIAN_POINT ( 'NONE',  ( -0.1958661417322836718, 0.3392501089628017219, -2.524934383202099397 ) ) ;
#75762=CARTESIAN_POINT ( 'NONE',  ( 0.2867679344610365999, 0.2867679344610365999, -2.742125984251967630 ) ) ;
#75765=CARTESIAN_POINT ( 'NONE',  ( 4.837279021331060870E-17, -0.3949938075777409963, -0.07874015748031501505 ) ) ;
#75766=ORIENTED_EDGE ( 'NONE', *, *, #57587, .F. ) ;
#75773=CARTESIAN_POINT ( 'NONE',  ( -0.3917322834645671770, 0.1049643490035302024, -1.604350024443256695 ) ) ;
#75775=CARTESIAN_POINT ( 'NONE',  ( -0.3392501089628019995, 0.1958661417322832277, -2.630577427821522374 ) ) ;
#75780=CARTESIAN_POINT ( 'NONE',  ( 0.1070741851644053527, 0.3996062992125986590, -0.9383202099737533164 ) ) ;
#75782=CARTESIAN_POINT ( 'NONE',  ( -0.3996062992125986590, 0.1070741851644051723, -0.2670603674540683037 ) ) ;
#75784=CARTESIAN_POINT ( 'NONE',  ( 4.893765752498283924E-17, -0.3996062992125986035, -2.440944881889763884 ) ) ;
#75785=CARTESIAN_POINT ( 'NONE',  ( 0.3392501089628018884, -0.1958661417322834220, -1.764435695538057791 ) ) ;
#75789=CARTESIAN_POINT ( 'NONE',  ( 0.4091458600556404646, -0.2362204724409448231, -1.126640419947506633 ) ) ;
#75792=CARTESIAN_POINT ( 'NONE',  ( 0.1974969037888706092, -0.3420746716998660508, -1.113517060367454015 ) ) ;
#75804=CARTESIAN_POINT ( 'NONE',  ( -0.3996062992125986590, 0.1070741851644051723, -1.684383202099737575 ) ) ;
#75821=CARTESIAN_POINT ( 'NONE',  ( -0.1958661417322836718, 0.3392501089628017219, -0.8851706036745407014 ) ) ;
#75840=CARTESIAN_POINT ( 'NONE',  ( 0.3392501089628018329, 0.1958661417322835607, -2.013123359580052618 ) ) ;
#75843=CARTESIAN_POINT ( 'NONE',  ( -0.4091458600556405756, 0.2362204724409446288, -0.4986876640419947715 ) ) ;
#75844=CARTESIAN_POINT ( 'NONE',  ( -0.1058382717557503211, 0.3949938075777409408, -2.841207349081365408 ) ) ;
#75847=CARTESIAN_POINT ( 'NONE',  ( -0.3917322834645670104, -7.196005306013484475E-17, -1.291338582677165503 ) ) ;
#75849=CARTESIAN_POINT ( 'NONE',  ( 0.1265901696524990294, -0.4724409448818896462, -2.290026246719159442 ) ) ;
#75856=CARTESIAN_POINT ( 'NONE',  ( 0.3392501089628018329, 0.1958661417322835052, -0.8411880332995258502 ) ) ;
#75863=CARTESIAN_POINT ( 'NONE',  ( 0.3917322834645670659, 2.398668435337828261E-17, -2.162092806595487637 ) ) ;
#75870=CARTESIAN_POINT ( 'NONE',  ( -0.3392501089628019995, 0.1958661417322832277, -1.528215223097112885 ) ) ;
#75881=CARTESIAN_POINT ( 'NONE',  ( 0.3917322834645670104, -0.1049643490035303411, -2.780839895013122565 ) ) ;
#75887=FACE_OUTER_BOUND ( 'NONE', #24789, .T. ) ;
#75888=CARTESIAN_POINT ( 'NONE',  ( 0.1049643490035303689, 0.3917322834645670104, -1.337926509186352142 ) ) ;
#75889=CARTESIAN_POINT ( 'NONE',  ( 5.785732909357575061E-17, -0.4724409448818898682, 0.1594488188976377896 ) ) ;
#75892=CARTESIAN_POINT ( 'NONE',  ( 0.3996062992125986035, -0.1070741851644052972, -2.865485564304462329 ) ) ;
#75901=CARTESIAN_POINT ( 'NONE',  ( 0.1070741851644054776, -0.3996062992125984925, -0.6345144356955381149 ) ) ;
#75904=CARTESIAN_POINT ( 'NONE',  ( 0.1049643490035304938, -0.3917322834645669549, -0.3923884514435695414 ) ) ;
#75919=CARTESIAN_POINT ( 'NONE',  ( -0.3917322834645670104, -0.1049643490035307020, -0.8300718092201594400 ) ) ;
#75923=CARTESIAN_POINT ( 'NONE',  ( 0.4724409448818896462, 0.1265901696524990294, -2.563648293963254776 ) ) ;
#75943=CARTESIAN_POINT ( 'NONE',  ( 0.1070741851644053388, 0.3996062992125986035, -2.589895013123359568 ) ) ;
#75949=CARTESIAN_POINT ( 'NONE',  ( 0.3996062992125986035, 0.1070741851644054776, -2.329396325459317296 ) ) ;
#75951=CARTESIAN_POINT ( 'NONE',  ( -0.1974969037888706647, 0.3420746716998658843, -1.587926509186351920 ) ) ;
#75953=CARTESIAN_POINT ( 'NONE',  ( -0.3458507752293909498, 0.3458507752293908388, -2.539370078740157410 ) ) ;
#75954=CARTESIAN_POINT ( 'NONE',  ( -0.3917322834645671215, 0.1049643490035301469, -0.4973753280839894875 ) ) ;
#75959=CARTESIAN_POINT ( 'NONE',  ( -0.3420746716998662729, 0.1974969037888702206, -2.465223097112861250 ) ) ;
#75964=CARTESIAN_POINT ( 'NONE',  ( -0.3460692066303960868, 0.1998031496062990242, -2.073490813648294129 ) ) ;
#75970=CARTESIAN_POINT ( 'NONE',  ( -0.3392501089628019995, 0.1958661417322832277, -0.1108923884514436548 ) ) ;
#75977=CARTESIAN_POINT ( 'NONE',  ( 0.1958661417322836440, -0.3392501089628017219, -0.6489501312335959060 ) ) ;
#75978=CARTESIAN_POINT ( 'NONE',  ( -0.1958661417322834220, -0.3392501089628018884, -1.632545931758530244 ) ) ;
#75979=CARTESIAN_POINT ( 'NONE',  ( -0.1958661417322836718, 0.3392501089628017219, -2.524934383202099397 ) ) ;
#75982=CARTESIAN_POINT ( 'NONE',  ( 0.1974969037888704704, 0.3420746716998660508, -2.506561679790026087 ) ) ;
#75986=CARTESIAN_POINT ( 'NONE',  ( -0.2925321140481930704, -0.2925321140481933480, -1.476377952755905554 ) ) ;
#75991=CARTESIAN_POINT ( 'NONE',  ( 0.1049643490035303689, 0.3917322834645670104, -0.3930446194225722945 ) ) ;
#76001=CARTESIAN_POINT ( 'NONE',  ( -0.3458507752293906723, -0.3458507752293910609, -1.948818897637795144 ) ) ;
#76007=CARTESIAN_POINT ( 'NONE',  ( 5.785732909357575061E-17, -0.4724409448818898682, -2.283464566929133799 ) ) ;
#76011=CARTESIAN_POINT ( 'NONE',  ( -0.3917322834645668994, -0.1049643490035306742, -0.5984058810685547458 ) ) ;
#76013=CARTESIAN_POINT ( 'NONE',  ( 0.2867679344610366554, -0.2867679344610365444, -0.8129921259842519676 ) ) ;
#76018=CARTESIAN_POINT ( 'NONE',  ( 0.2867679344610365999, 0.2867679344610365999, -2.649606299212598604 ) ) ;
#76022=CARTESIAN_POINT ( 'NONE',  ( 0.4091458600556403535, 0.2362204724409449896, -0.8379265091863516979 ) ) ;
#76034=CARTESIAN_POINT ( 'NONE',  ( -0.3996062992125985480, -7.340648628747423112E-17, -2.163385826771653697 ) ) ;
#76040=CARTESIAN_POINT ( 'NONE',  ( 0.1265901696524990572, -0.4724409448818897017, -0.08530183727034119923 ) ) ;
#76042=CARTESIAN_POINT ( 'NONE',  ( 0.1998031496062992463, 0.3460692066303959202, -0.5360892388451443669 ) ) ;
#76044=CARTESIAN_POINT ( 'NONE',  ( -0.3460692066303958092, -0.1998031496062994683, -0.9973753280839895430 ) ) ;
#76045=CARTESIAN_POINT ( 'NONE',  ( -0.3420746716998659953, -0.1974969037888706647, -0.05249343832021002854 ) ) ;
#76051=CARTESIAN_POINT ( 'NONE',  ( -0.1058382717557497660, -0.3949938075777411073, -1.408792650918635259 ) ) ;
#76056=CARTESIAN_POINT ( 'NONE',  ( 5.785732909357575061E-17, -0.4724409448818898682, -1.811023622047244208 ) ) ;
#76057=CARTESIAN_POINT ( 'NONE',  ( 0.1998031496062992740, 0.3460692066303959757, -2.664041994750656173 ) ) ;
#76071=CARTESIAN_POINT ( 'NONE',  ( 0.3917322834645669549, 0.1049643490035304660, -1.534120734908136052 ) ) ;
#76074=CARTESIAN_POINT ( 'NONE',  ( -0.2891555358219911054, 0.2891555358219909388, -1.594488188976378007 ) ) ;
#76079=CARTESIAN_POINT ( 'NONE',  ( 0.1998031496062992740, 0.3460692066303959757, -0.1443569553805774397 ) ) ;
#76086=CARTESIAN_POINT ( 'NONE',  ( 0.3392501089628018329, 0.1958661417322835607, 0.09908136482939623735 ) ) ;
#76092=CARTESIAN_POINT ( 'NONE',  ( -0.3996062992125986035, -7.340648628747425578E-17, -1.929133858267716439 ) ) ;
#76095=CARTESIAN_POINT ( 'NONE',  ( 0.3460692066303959202, -0.1998031496062991630, -1.756561679790026309 ) ) ;
#76099=CARTESIAN_POINT ( 'NONE',  ( 0.4724409448818897572, -0.1265901696524988906, -0.8989501312335956840 ) ) ;
#76101=CARTESIAN_POINT ( 'NONE',  ( 0.1049643490035303689, 0.3917322834645670104, -2.755249343832020248 ) ) ;
#76104=CARTESIAN_POINT ( 'NONE',  ( 0.3917322834645670104, -0.1049643490035303273, -2.085958005249343827 ) ) ;
#76110=CARTESIAN_POINT ( 'NONE',  ( 0.1998031496062994128, -0.3460692066303957537, 0.1463254593175852825 ) ) ;
#76112=CARTESIAN_POINT ( 'NONE',  ( -0.2891555358219909388, -0.2891555358219912164, -2.183070866141731958 ) ) ;
#76117=CARTESIAN_POINT ( 'NONE',  ( -0.4724409448818880364, -0.1265901696525023323, -2.169947506561679784 ) ) ;
#76133=CARTESIAN_POINT ( 'NONE',  ( 0.3996062992125984925, 0.1070741851644054637, -0.5164041994750655507 ) ) ;
#76134=EDGE_CURVE ( 'NONE', #6583, #50887, #47615, .T. ) ;
#76135=CARTESIAN_POINT ( 'NONE',  ( 0.3917322834645670104, -0.1049643490035303411, -2.400918635170603554 ) ) ;
#76144=CARTESIAN_POINT ( 'NONE',  ( -0.4724409448818898682, -8.678599364036362592E-17, -0.6692913385826770867 ) ) ;
#76151=CARTESIAN_POINT ( 'NONE',  ( -0.2867679344610364334, -0.2867679344610367109, -1.875984251968503935 ) ) ;
#76152=CARTESIAN_POINT ( 'NONE',  ( 0.02733964191757773388, 0.3913445824879502322, -1.220472440944881498 ) ) ;
#76155=CARTESIAN_POINT ( 'NONE',  ( 0.4091458600556403535, 0.2362204724409449896, -0.4461942257217847430 ) ) ;
#76158=CARTESIAN_POINT ( 'NONE',  ( -0.01591673448991381273, 0.3996062992125985480, -2.754912411187758536 ) ) ;
#76161=CARTESIAN_POINT ( 'NONE',  ( 0.1070741851644053527, 0.3996062992125986590, -1.095800524934382958 ) ) ;
#76163=CARTESIAN_POINT ( 'NONE',  ( 0.1958661417322834775, 0.3392501089628018884, -2.813648293963254776 ) ) ;
#76175=CARTESIAN_POINT ( 'NONE',  ( -0.1049643490035302024, -0.3917322834645671215, -0.2217847769028870319 ) ) ;
#76178=CARTESIAN_POINT ( 'NONE',  ( 0.1058382717557499880, 0.3949938075777411073, 0.006561679790026190250 ) ) ;
#76185=CARTESIAN_POINT ( 'NONE',  ( -0.1958661417322836995, 0.3392501089628017219, -1.742145300033807631 ) ) ;
#76187=CARTESIAN_POINT ( 'NONE',  ( -9.594673741351313045E-17, 0.3917322834645670104, -2.604330708661416693 ) ) ;
#76192=CARTESIAN_POINT ( 'NONE',  ( -0.2925321140481932924, 0.2925321140481931814, -0.6496062992125984925 ) ) ;
#76194=CARTESIAN_POINT ( 'NONE',  ( 0.2925321140481932369, 0.2925321140481932369, -0.2145669291338583029 ) ) ;
#76196=CARTESIAN_POINT ( 'NONE',  ( 0.3996062992125986035, 0.1070741851644054776, -2.486876640419947382 ) ) ;
#76197=CARTESIAN_POINT ( 'NONE',  ( -0.3917322834645669549, -0.1049643490035306603, -1.862860892388451761 ) ) ;
#76202=CARTESIAN_POINT ( 'NONE',  ( -0.4091458600556405756, 0.2362204724409446288, -1.677821522309711266 ) ) ;
#76205=CARTESIAN_POINT ( 'NONE',  ( -0.1058382717557497660, -0.3949938075777411073, -0.7788713910761156933 ) ) ;
#76208=CARTESIAN_POINT ( 'NONE',  ( -0.4724409448818888135, -0.1265901696525008335, -1.067585301837270517 ) ) ;
#76217=CARTESIAN_POINT ( 'NONE',  ( -0.1070741851644051862, -0.3996062992125986590, -1.881233595800524849 ) ) ;
#76234=CARTESIAN_POINT ( 'NONE',  ( 0.1049643490035304938, -0.3917322834645669549, -0.9573490813648293241 ) ) ;
#76237=FACE_OUTER_BOUND ( 'NONE', #29398, .T. ) ;
#76249=CARTESIAN_POINT ( 'NONE',  ( -0.4709442531824371558, -0.03757601356356778805, -1.220472440944882164 ) ) ;
#76253=CARTESIAN_POINT ( 'NONE',  ( 0.3917322834645670104, 2.398668435337828261E-17, -2.000000000000000000 ) ) ;
#76256=CARTESIAN_POINT ( 'NONE',  ( 0.2362204724409449064, 0.4091458600556404646, -0.1443569553805774397 ) ) ;
#76257=CARTESIAN_POINT ( 'NONE',  ( -0.3949938075777411628, 0.1058382717557497937, -2.709973753280840114 ) ) ;
#76260=CARTESIAN_POINT ( 'NONE',  ( -0.3917322834645671215, 0.1049643490035301469, -1.442257217847769057 ) ) ;
#76262=CARTESIAN_POINT ( 'NONE',  ( -0.3458507752293906723, -0.3458507752293910609, -2.736220472440944018 ) ) ;
#76270=CARTESIAN_POINT ( 'NONE',  ( -0.3917322834645668994, -0.1049643490035306742, -0.9133665109898146950 ) ) ;
#76277=CARTESIAN_POINT ( 'NONE',  ( -0.4724409448818898682, -8.678599364036362592E-17, -1.141732283464566899 ) ) ;
#76279=CARTESIAN_POINT ( 'NONE',  ( 4.797336870675656522E-17, -0.3917322834645670659, -1.965242412894699919 ) ) ;
#76287=CARTESIAN_POINT ( 'NONE',  ( -0.3917322834645669549, -0.1049643490035306603, -1.547900262467191590 ) ) ;
#76292=CARTESIAN_POINT ( 'NONE',  ( -0.0008564280371856086574, 0.3986795681651738033, 7.618016766297077184E-18 ) ) ;
#76297=CARTESIAN_POINT ( 'NONE',  ( 0.1049643490035303689, 0.3917322834645670104, -2.662729658792650778 ) ) ;
#76305=CARTESIAN_POINT ( 'NONE',  ( 4.797336870675656522E-17, -0.3917322834645670104, -1.108267716535433101 ) ) ;
#76306=CARTESIAN_POINT ( 'NONE',  ( -0.4091458600556402980, -0.2362204724409451284, 0.02821522309711285356 ) ) ;
#76307=CARTESIAN_POINT ( 'NONE',  ( -0.1070741851644051862, -0.3996062992125986590, -2.668635170603674833 ) ) ;
#76317=CARTESIAN_POINT ( 'NONE',  ( 0.3996062992125986035, -0.1070741851644052972, -0.6607611548556431291 ) ) ;
#76319=CARTESIAN_POINT ( 'NONE',  ( 0.3917322834645670104, 2.398668435337828261E-17, -0.2677165354330708347 ) ) ;
#76333=CARTESIAN_POINT ( 'NONE',  ( 0.3392501089628018884, -0.1958661417322833942, -1.046607242291025752 ) ) ;
#76337=CARTESIAN_POINT ( 'NONE',  ( -0.2362204724409451284, 0.4091458600556402425, -2.452099737532808188 ) ) ;
#76356=CARTESIAN_POINT ( 'NONE',  ( 0.3996062992125986035, -0.1070741851644053111, -0.4265091863517060378 ) ) ;
#76357=CARTESIAN_POINT ( 'NONE',  ( 0.1070741851644053388, 0.3996062992125986035, -2.747375328083988766 ) ) ;
#76362=CARTESIAN_POINT ( 'NONE',  ( -0.3996062992125986035, -7.340648628747425578E-17, -2.244094488188976388 ) ) ;
#76363=CARTESIAN_POINT ( 'NONE',  ( -9.674558042662121740E-17, 0.3949938075777409963, -1.417322834645669216 ) ) ;
#76366=CARTESIAN_POINT ( 'NONE',  ( -0.1958661417322834220, -0.3392501089628018884, -0.6876640419947506189 ) ) ;
#76369=CARTESIAN_POINT ( 'NONE',  ( 0.3420746716998660508, -0.1974969037888704149, -2.386482939632546429 ) ) ;
#76374=CARTESIAN_POINT ( 'NONE',  ( 0.1070741851644054915, -0.3996062992125986035, -1.975065616797900381 ) ) ;
#76380=CARTESIAN_POINT ( 'NONE',  ( 0.1958661417322834775, 0.3392501089628018884, -0.2290026246719160941 ) ) ;
#76387=CARTESIAN_POINT ( 'NONE',  ( -0.3917322834645669549, -0.1049643490035306603, -0.4455380577427821565 ) ) ;
#76388=CARTESIAN_POINT ( 'NONE',  ( -0.2867679344610364334, -0.2867679344610367109, -1.468503937007874294 ) ) ;
#76389=CARTESIAN_POINT ( 'NONE',  ( -0.3392501089628019995, 0.1958661417322832277, -2.695538057742782101 ) ) ;
#76391=CARTESIAN_POINT ( 'NONE',  ( -0.3996062992125986035, -7.340648628747425578E-17, 0.1181102362204724254 ) ) ;
#76396=CARTESIAN_POINT ( 'NONE',  ( 0.3460692066303959757, -0.1998031496062991907, -1.364829396325459188 ) ) ;
#76398=CARTESIAN_POINT ( 'NONE',  ( -0.3996062992125986035, -1.273259842764937629E-12, -1.929133858267794599 ) ) ;
#76401=CARTESIAN_POINT ( 'NONE',  ( -0.3917322834645670104, -7.196005306013484475E-17, -0.4389763779527560139 ) ) ;
#76411=CARTESIAN_POINT ( 'NONE',  ( 0.4091458600556403535, 0.2362204724409449896, -2.178477690288713742 ) ) ;
#76422=CARTESIAN_POINT ( 'NONE',  ( 4.797336870675655290E-17, -0.3917322834645669549, -0.4737339650580559280 ) ) ;
#76424=CARTESIAN_POINT ( 'NONE',  ( 4.797336870675656522E-17, -0.3917322834645670104, -0.6358267716535433989 ) ) ;
#76425=EDGE_CURVE ( 'NONE', #42415, #28644, #13702, .T. ) ;
#76430=CARTESIAN_POINT ( 'NONE',  ( 0.1049643490035304938, -0.3917322834645669549, -2.597112860892388131 ) ) ;
#76433=CARTESIAN_POINT ( 'NONE',  ( -0.2362204724409451284, 0.4091458600556402425, -1.192257217847769057 ) ) ;
#76446=CARTESIAN_POINT ( 'NONE',  ( 0.3996062992125985480, 2.446882876249141654E-17, -2.399606299212598604 ) ) ;
#76447=( BOUNDED_CURVE ( )  B_SPLINE_CURVE ( 2, ( #34399, #15050, #33153, #8729, #59229, #20108, #21763, #27245, #47009, #2421, #33982, #71453, #41126, #28078, #72295, #52904, #14641, #59643, #27662, #73117, #2000, #53328, #79037, #21356, #79444, #15469, #32726, #58394, #26415, #13802, #39459, #58822, #1179, #26830, #47841, #49082, #74368, #41539, #29730, #4473, #17133, #60892, #23832, #42765, #36459, #60480, #54984, #2831, #80692, #35228, #74782, #34822, #73954, #23005, #28492, #62133, #73547, #49500, #9558, #3660, #15890, #30141, #54152, #61302, #42352, #79866, #36054, #16711, #29323, #41943, #22184, #67639, #23415, #67227, #68461, #48671, #3242, #28907, #54570, #55804, #81098, #10799, #68050, #75193, #80284, #22597, #17537, #16300, #48258, #10397, #9971, #81510, #35642, #61726, #66817, #4063, #55392, #9150, #76424, #63777, #19158, #24236, #50315, #51131, #25464, #70089, #17945, #82732, #30962, #62965, #5303, #18753, #57452, #69283, #38519, #49909, #57037, #76825, #11629, #12443, #63367, #43581, #18355, #32206, #75606, #76013, #44808, #70503, #38102, #37290, #25051, #56629, #82330, #24648, #44397, #83145, #43998, #12862, #5701, #6117, #31789, #64202, #6536, #50726, #77246, #57863, #69692, #12035, #231, #25882, #37692, #51543, #31373, #30561, #43169, #68865, #11214, #36873, #62551, #81925, #4887, #56227, #21249, #40604, #66287, #53632, #39771, #13281, #46073, #7369, #8211, #65466, #72183, #7800, #59958, #19576, #8626, #34297, #2313, #33039, #6950, #65034, #78089, #1484, #59127, #32621, #33465, #1073, #20835 ),
 .UNSPECIFIED., .F., .F. ) 
 B_SPLINE_CURVE_WITH_KNOTS ( ( 3, 2, 2, 2, 2, 2, 2, 2, 2, 2, 2, 2, 2, 2, 2, 2, 2, 2, 2, 2, 2, 2, 2, 2, 2, 2, 2, 2, 2, 2, 2, 2, 2, 2, 2, 2, 2, 2, 2, 2, 2, 2, 2, 2, 2, 2, 2, 2, 2, 2, 2, 2, 2, 2, 2, 2, 2, 2, 2, 2, 2, 2, 2, 2, 2, 2, 2, 2, 2, 2, 2, 2, 2, 2, 2, 2, 2, 2, 2, 2, 2, 2, 2, 2, 2, 2, 2, 2, 2, 2, 2, 2, 2, 2, 3 ),
 ( 0.07312148491320361043, 0.07499999999999999722, 0.07916666666666666297, 0.08333333333333332871, 0.08749999999999999445, 0.09166666666666666019, 0.09583333333333333981, 0.1000000000000000056, 0.1041666666666666713, 0.1083333333333333370, 0.1125000000000000028, 0.1166666666666666685, 0.1208333333333333204, 0.1250000000000000000, 0.1291666666666666796, 0.1333333333333333315, 0.1375000000000000111, 0.1416666666666666630, 0.1458333333333333426, 0.1499999999999999944, 0.1541666666666666741, 0.1583333333333333259, 0.1625000000000000056, 0.1666666666666666297, 0.1708333333333333370, 0.1749999999999999889, 0.1791666666666666685, 0.1833333333333333204, 0.1875000000000000000, 0.1916666666666666796, 0.1958333333333333592, 0.2000000000000000111, 0.2041666666666666630, 0.2083333333333333426, 0.2124999999999999944, 0.2166666666666666741, 0.2208333333333333259, 0.2250000000000000056, 0.2291666666666666574, 0.2333333333333333370, 0.2374999999999999889, 0.2416666666666666685, 0.2458333333333332926, 0.2500000000000000000, 0.2541666666666666519, 0.2583333333333333592, 0.2624999999999999556, 0.2666666666666666630, 0.2708333333333333148, 0.2750000000000000222, 0.2791666666666666741, 0.2833333333333333259, 0.2874999999999999778, 0.2916666666666667407, 0.2958333333333333370, 0.2999999999999999889, 0.3041666666666666408, 0.3083333333333333481, 0.3125000000000000000, 0.3166666666666666519, 0.3208333333333334147, 0.3249999999999999556, 0.3291666666666666075, 0.3333333333333332593, 0.3375000000000000222, 0.3416666666666666741, 0.3458333333333333259, 0.3499999999999999778, 0.3541666666666666297, 0.3583333333333332815, 0.3624999999999999334, 0.3666666666666665853, 0.3708333333333333481, 0.3750000000000000000, 0.3791666666666666519, 0.3833333333333333037, 0.3874999999999999556, 0.3916666666666666075, 0.3958333333333332593, 0.4000000000000000222, 0.4041666666666666741, 0.4083333333333333259, 0.4124999999999999778, 0.4166666666666666297, 0.4208333333333333925, 0.4249999999999999334, 0.4291666666666665853, 0.4333333333333333481, 0.4375000000000000000, 0.4416666666666666519, 0.4458333333333333037, 0.4499999999999999556, 0.4541666666666666075, 0.4583333333333333703, 0.4606214849132036493 ),
 .UNSPECIFIED. ) 
 CURVE ( )  GEOMETRIC_REPRESENTATION_ITEM ( )  RATIONAL_B_SPLINE_CURVE ( ( 0.9831275833774530959, 0.9846378761473345564, 1.000000000000000000, 0.9659258262890683122, 1.000000000000000000, 0.9659258262890683122, 1.000000000000000000, 0.9659258262890683122, 1.000000000000000000, 0.9659258262890683122, 1.000000000000000000, 0.9659258262890683122, 1.000000000000000000, 0.9659258262890683122, 1.000000000000000000, 0.9659258262890683122, 1.000000000000000000, 0.9659258262890683122, 1.000000000000000000, 0.9659258262890683122, 1.000000000000000000, 0.9659258262890683122, 1.000000000000000000, 0.9659258262890683122, 1.000000000000000000, 0.9659258262890683122, 1.000000000000000000, 0.9659258262890683122, 1.000000000000000000, 0.9659258262890683122, 1.000000000000000000, 0.9659258262890683122, 1.000000000000000000, 0.9659258262890683122, 1.000000000000000000, 0.9659258262890683122, 1.000000000000000000, 0.9659258262890683122, 1.000000000000000000, 0.9659258262890683122, 1.000000000000000000, 0.9659258262890683122, 1.000000000000000000, 0.9659258262890683122, 1.000000000000000000, 0.9659258262890683122, 1.000000000000000000, 0.9659258262890683122, 1.000000000000000000, 0.9659258262890683122, 1.000000000000000000, 0.9659258262890683122, 1.000000000000000000, 0.9659258262890683122, 1.000000000000000000, 0.9659258262890683122, 1.000000000000000000, 0.9659258262890683122, 1.000000000000000000, 0.9659258262890683122, 1.000000000000000000, 0.9659258262890683122, 1.000000000000000000, 0.9659258262890683122, 1.000000000000000000, 0.9659258262890683122, 1.000000000000000000, 0.9659258262890683122, 1.000000000000000000, 0.9659258262890683122, 1.000000000000000000, 0.9659258262890683122, 1.000000000000000000, 0.9659258262890683122, 1.000000000000000000, 0.9659258262890683122, 1.000000000000000000, 0.9659258262890683122, 1.000000000000000000, 0.9659258262890683122, 1.000000000000000000, 0.9659258262890683122, 1.000000000000000000, 0.9659258262890683122, 1.000000000000000000, 0.9659258262890683122, 1.000000000000000000, 0.9659258262890683122, 1.000000000000000000, 0.9659258262890683122, 1.000000000000000000, 0.9659258262890683122, 1.000000000000000000, 0.9659258262890683122, 1.000000000000000000, 0.9659258262890683122, 1.000000000000000000, 0.9659258262890683122, 1.000000000000000000, 0.9659258262890683122, 1.000000000000000000, 0.9659258262890683122, 1.000000000000000000, 0.9659258262890683122, 1.000000000000000000, 0.9659258262890683122, 1.000000000000000000, 0.9659258262890683122, 1.000000000000000000, 0.9659258262890683122, 1.000000000000000000, 0.9659258262890683122, 1.000000000000000000, 0.9659258262890683122, 1.000000000000000000, 0.9659258262890683122, 1.000000000000000000, 0.9659258262890683122, 1.000000000000000000, 0.9659258262890683122, 1.000000000000000000, 0.9659258262890683122, 1.000000000000000000, 0.9659258262890683122, 1.000000000000000000, 0.9659258262890683122, 1.000000000000000000, 0.9659258262890683122, 1.000000000000000000, 0.9659258262890683122, 1.000000000000000000, 0.9659258262890683122, 1.000000000000000000, 0.9659258262890683122, 1.000000000000000000, 0.9659258262890683122, 1.000000000000000000, 0.9659258262890683122, 1.000000000000000000, 0.9659258262890683122, 1.000000000000000000, 0.9659258262890683122, 1.000000000000000000, 0.9659258262890683122, 1.000000000000000000, 0.9659258262890683122, 1.000000000000000000, 0.9659258262890683122, 1.000000000000000000, 0.9659258262890683122, 1.000000000000000000, 0.9659258262890683122, 1.000000000000000000, 0.9659258262890683122, 1.000000000000000000, 0.9659258262890683122, 1.000000000000000000, 0.9659258262890683122, 1.000000000000000000, 0.9659258262890683122, 1.000000000000000000, 0.9659258262890683122, 1.000000000000000000, 0.9659258262890683122, 1.000000000000000000, 0.9659258262890683122, 1.000000000000000000, 0.9659258262890683122, 1.000000000000000000, 0.9659258262890683122, 1.000000000000000000, 0.9659258262890683122, 1.000000000000000000, 0.9659258262890683122, 1.000000000000000000, 0.9659258262890683122, 1.000000000000000000, 0.9659258262890683122, 1.000000000000000000, 0.9659258262890683122, 1.000000000000000000, 0.9659258262890683122, 1.000000000000000000, 0.9659258262890683122, 1.000000000000000000, 0.9659258262890683122, 1.000000000000000000, 0.9812879501417335337, 0.9831275833774533179 ) ) 
 REPRESENTATION_ITEM ( '' )  );
#76451=CARTESIAN_POINT ( 'NONE',  ( -0.1998031496062994405, 0.3460692066303957537, -1.507217847769029007 ) ) ;
#76457=CARTESIAN_POINT ( 'NONE',  ( 0.3996062992125984925, 0.1070741851644054499, -0.6738845144356955252 ) ) ;
#76458=CARTESIAN_POINT ( 'NONE',  ( -0.3996062992125987146, 0.1070741851644051862, -1.135170603674540590 ) ) ;
#76460=CARTESIAN_POINT ( 'NONE',  ( 0.2891555358219910499, 0.2891555358219910499, -0.4527559055118110520 ) ) ;
#76466=CARTESIAN_POINT ( 'NONE',  ( -0.1974969037888706924, 0.3420746716998658843, -1.507217847769029007 ) ) ;
#76471=CARTESIAN_POINT ( 'NONE',  ( 0.4091458600556403535, 0.2362204724409449896, -1.706036745406824151 ) ) ;
#76472=CARTESIAN_POINT ( 'NONE',  ( 0.2925321140481932369, 0.2925321140481932369, -2.657480314960630086 ) ) ;
#76479=CARTESIAN_POINT ( 'NONE',  ( -0.1049643490035301746, -0.3917322834645670659, -2.041975434874328865 ) ) ;
#76485=CARTESIAN_POINT ( 'NONE',  ( -0.1049643490035302024, -0.3917322834645671215, -1.481627296587926690 ) ) ;
#76488=CARTESIAN_POINT ( 'NONE',  ( 0.3949938075777409408, 0.1058382717557500574, -2.014435695538057569 ) ) ;
#76493=CARTESIAN_POINT ( 'NONE',  ( 0.3996062992125986035, 0.1070741851644054776, -0.1246719160104987068 ) ) ;
#76500=CARTESIAN_POINT ( 'NONE',  ( 0.3917322834645669549, 0.1049643490035304660, 0.1056430446194224632 ) ) ;
#76507=CARTESIAN_POINT ( 'NONE',  ( 0.3996062992125986035, -0.1070741851644052972, -1.448162729658792669 ) ) ;
#76512=CARTESIAN_POINT ( 'NONE',  ( -1.157146581871515012E-16, 0.4724409448818898682, -0.9448818897637796255 ) ) ;
#76514=CARTESIAN_POINT ( 'NONE',  ( -0.3917322834645671215, 0.1049643490035301469, -2.794619422572177658 ) ) ;
#76516=CARTESIAN_POINT ( 'NONE',  ( -0.3392501089628019995, 0.1958661417322832277, -2.000656167979002920 ) ) ;
#76520=CARTESIAN_POINT ( 'NONE',  ( 0.3458507752293908943, 0.3458507752293908943, -2.734251968503936148 ) ) ;
#76524=CARTESIAN_POINT ( 'NONE',  ( 0.1974969037888704704, 0.3420746716998660508, -2.268372703412073754 ) ) ;
#76533=CARTESIAN_POINT ( 'NONE',  ( -0.4091458600556405756, 0.2362204724409446288, -0.1030183727034120617 ) ) ;
#76545=CARTESIAN_POINT ( 'NONE',  ( 0.3460692066303958092, 0.1998031496062993018, -0.5229658792650918597 ) ) ;
#76546=CARTESIAN_POINT ( 'NONE',  ( 0.3392501089628018884, -0.1958661417322834220, -2.079396325459317740 ) ) ;
#76556=CARTESIAN_POINT ( 'NONE',  ( 0.1049643490035304799, -0.3917322834645670104, -2.286764722605985956 ) ) ;
#76562=CARTESIAN_POINT ( 'NONE',  ( 0.3392501089628018329, 0.1958661417322835607, -1.790682414698162805 ) ) ;
#76569=CARTESIAN_POINT ( 'NONE',  ( 0.3996062992125986590, -0.1070741851644053111, -1.528871391076114916 ) ) ;
#76571=CARTESIAN_POINT ( 'NONE',  ( 0.3917322834645670659, -0.1049643490035303273, 0.04919328264335768447 ) ) ;
#76583=CARTESIAN_POINT ( 'NONE',  ( -0.1049643490035302024, -0.3917322834645671215, -0.06430446194225715451 ) ) ;
#76586=CARTESIAN_POINT ( 'NONE',  ( -0.1974969037888703871, -0.3420746716998661063, -0.06561679790026252179 ) ) ;
#76593=CARTESIAN_POINT ( 'NONE',  ( 0.1049643490035304799, -0.3917322834645670104, -1.814323777724096809 ) ) ;
#76595=CARTESIAN_POINT ( 'NONE',  ( -0.1958661417322834220, -0.3392501089628018884, -2.669947506561679784 ) ) ;
#76599=CARTESIAN_POINT ( 'NONE',  ( -0.2925321140481930704, -0.2925321140481933480, -1.003937007874015741 ) ) ;
#76601=CARTESIAN_POINT ( 'NONE',  ( 0.3460692066303958092, 0.1998031496062993018, -0.5229658792650918597 ) ) ;
#76602=CARTESIAN_POINT ( 'NONE',  ( 0.3460692066303959202, -0.1998031496062991630, -0.1817585301837270351 ) ) ;
#76604=CARTESIAN_POINT ( 'NONE',  ( 0.3996062992125986590, -0.1070741851644053111, -2.788713910761154047 ) ) ;
#76606=CARTESIAN_POINT ( 'NONE',  ( 0.3392501089628018884, -0.1958661417322834220, -1.606955380577427928 ) ) ;
#76611=CARTESIAN_POINT ( 'NONE',  ( 0.4091458600556403535, 0.2362204724409449896, -1.310367454068241511 ) ) ;
#76614=CARTESIAN_POINT ( 'NONE',  ( 0.2891555358219910499, 0.2891555358219910499, -1.001968503937007871 ) ) ;
#76620=CARTESIAN_POINT ( 'NONE',  ( 0.4724409448818898682, 0.000000000000000000, -2.755905511811024056 ) ) ;
#76623=CARTESIAN_POINT ( 'NONE',  ( -0.3996062992125985480, -7.340648628747423112E-17, -2.005905511811023612 ) ) ;
#76626=DIRECTION ( 'NONE',  ( 0.000000000000000000, 0.000000000000000000, 1.000000000000000000 ) ) ;
#76637=CARTESIAN_POINT ( 'NONE',  ( -0.2867679344610364334, -0.2867679344610367109, -1.088582677165354173 ) ) ;
#76656=CARTESIAN_POINT ( 'NONE',  ( -0.3917322834645669549, -0.1049643490035306603, -2.085301837270341352 ) ) ;
#76659=CARTESIAN_POINT ( 'NONE',  ( 0.4724409448818896462, 0.1265901696524990294, -0.4396325459317584339 ) ) ;
#76660=CARTESIAN_POINT ( 'NONE',  ( -0.3460692066303958092, -0.1998031496062994683, -0.05249343832020999384 ) ) ;
#76663=CARTESIAN_POINT ( 'NONE',  ( 0.1049643490035303689, 0.3917322834645670104, -1.560367454068241511 ) ) ;
#76665=CARTESIAN_POINT ( 'NONE',  ( -0.1265901696524993347, 0.4724409448818895907, -2.841207349081364963 ) ) ;
#76673=CARTESIAN_POINT ( 'NONE',  ( -0.1958661417322836440, 0.3392501089628016664, -0.7230777970790532860 ) ) ;
#76680=CARTESIAN_POINT ( 'NONE',  ( -0.2867679344610367109, 0.2867679344610365444, -1.906187294784464026 ) ) ;
#76687=CARTESIAN_POINT ( 'NONE',  ( 0.3917322834645670104, 2.398668435337828261E-17, -1.305118110236220375 ) ) ;
#76694=CARTESIAN_POINT ( 'NONE',  ( 0.4091458600556404646, -0.2362204724409448231, -0.9691601049868766582 ) ) ;
#76696=CARTESIAN_POINT ( 'NONE',  ( 0.2867679344610365999, -0.2867679344610365444, -2.925196850393700920 ) ) ;
#76704=CARTESIAN_POINT ( 'NONE',  ( 0.3917322834645669549, 0.1049643490035304660, -1.311679790026246906 ) ) ;
#76705=CARTESIAN_POINT ( 'NONE',  ( -0.3458507752293906723, -0.3458507752293910609, -0.2933070866141732069 ) ) ;
#76708=CARTESIAN_POINT ( 'NONE',  ( -9.674558042662122972E-17, 0.3949938075777409963, 0.2381889763779528046 ) ) ;
#76713=CARTESIAN_POINT ( 'NONE',  ( -0.1058382717557503072, 0.3949938075777408852, -0.08333333333333334259 ) ) ;
#76717=CARTESIAN_POINT ( 'NONE',  ( -0.1958661417322834220, -0.3392501089628018884, -2.669947506561679784 ) ) ;
#76721=CARTESIAN_POINT ( 'NONE',  ( 0.1070741851644054776, -0.3996062992125984925, -1.106955380577427706 ) ) ;
#76723=CARTESIAN_POINT ( 'NONE',  ( 0.3917322834645670104, -0.1049643490035303411, -0.1036745406824146343 ) ) ;
#76738=CARTESIAN_POINT ( 'NONE',  ( 0.3392501089628018329, 0.1958661417322835607, -0.7578933315298707063 ) ) ;
#76742=CARTESIAN_POINT ( 'NONE',  ( -0.2362204724409447953, -0.4091458600556404646, -2.504593175853018661 ) ) ;
#76760=CARTESIAN_POINT ( 'NONE',  ( -0.3996062992125986590, 0.1070741851644051862, -0.5052493438320209140 ) ) ;
#76761=CARTESIAN_POINT ( 'NONE',  ( -0.2925321140481932369, 0.2925321140481931259, -2.616141732283464805 ) ) ;
#76766=CARTESIAN_POINT ( 'NONE',  ( -9.787531504996567848E-17, 0.3996062992125986035, -2.204724409448818978 ) ) ;
#76767=CARTESIAN_POINT ( 'NONE',  ( 0.1058382717557499880, 0.3949938075777411073, -1.410761154855643351 ) ) ;
#76768=CARTESIAN_POINT ( 'NONE',  ( 0.2925321140481932369, 0.2925321140481932369, -2.814960629921259727 ) ) ;
#76769=CARTESIAN_POINT ( 'NONE',  ( -0.1958661417322836718, 0.3392501089628017219, -1.107611548556430403 ) ) ;
#76772=CARTESIAN_POINT ( 'NONE',  ( -0.2891555358219911054, 0.2891555358219909388, -2.616141732283464805 ) ) ;
#76776=CARTESIAN_POINT ( 'NONE',  ( 0.3458507752293908943, 0.3458507752293908943, -0.05708661417322836301 ) ) ;
#76777=CARTESIAN_POINT ( 'NONE',  ( -0.3460692066303958092, -0.1998031496062994683, -2.099737532808398921 ) ) ;
#76783=CARTESIAN_POINT ( 'NONE',  ( -0.3917322834645669549, -0.1049643490035306603, -0.1305774278215224293 ) ) ;
#76792=CARTESIAN_POINT ( 'NONE',  ( -0.1049643490035307020, 0.3917322834645669549, -0.5636482939632546652 ) ) ;
#76793=CARTESIAN_POINT ( 'NONE',  ( -0.3392501089628019995, 0.1958661417322832277, -1.435695538057742970 ) ) ;
#76794=CARTESIAN_POINT ( 'NONE',  ( -9.594673741351313045E-17, 0.3917322834645670104, -2.669291338582676865 ) ) ;
#76796=CARTESIAN_POINT ( 'NONE',  ( 0.3460692066303959202, 0.1998031496062993295, 0.02624671916010496570 ) ) ;
#76800=CARTESIAN_POINT ( 'NONE',  ( 0.1070741851644053527, 0.3996062992125986590, -1.410761154855643129 ) ) ;
#76804=CARTESIAN_POINT ( 'NONE',  ( 0.3893108287682404134, -0.05073257145186561845, -1.929133858267715773 ) ) ;
#76805=CARTESIAN_POINT ( 'NONE',  ( -0.2867679344610364334, -0.2867679344610367109, -0.7736220472440945573 ) ) ;
#76813=CARTESIAN_POINT ( 'NONE',  ( 0.3458507752293908943, -0.3458507752293908943, -2.145669291338581974 ) ) ;
#76814=CARTESIAN_POINT ( 'NONE',  ( 0.2362204724409449064, 0.4091458600556404646, -2.664041994750656173 ) ) ;
#76823=CARTESIAN_POINT ( 'NONE',  ( -0.3917322834645668994, -0.1049643490035306742, -0.9133665109898146950 ) ) ;
#76825=CARTESIAN_POINT ( 'NONE',  ( -0.3917322834645669549, -0.1049643490035306603, -0.7604986876640419391 ) ) ;
#76831=CARTESIAN_POINT ( 'NONE',  ( 0.1958661417322834775, 0.3392501089628018884, -2.656167979002624691 ) ) ;
#76834=CARTESIAN_POINT ( 'NONE',  ( -0.3458507752293909498, 0.3458507752293907833, -1.198818897637795367 ) ) ;
#76841=DIRECTION ( 'NONE',  ( 1.000000000000000000, 0.000000000000000000, 0.000000000000000000 ) ) ;
#76846=CARTESIAN_POINT ( 'NONE',  ( -0.1998031496062991630, -0.3460692066303959202, -2.347112860892388575 ) ) ;
#76851=CARTESIAN_POINT ( 'NONE',  ( -0.2925321140481932369, 0.2925321140481931259, -1.198818897637795367 ) ) ;
#76858=CARTESIAN_POINT ( 'NONE',  ( -0.2925321140481932369, 0.2925321140481930704, -0.5688976377952755792 ) ) ;
#76859=CARTESIAN_POINT ( 'NONE',  ( -0.3996062992125986035, -7.340648628747425578E-17, -0.9842519685039369248 ) ) ;
#76860=CARTESIAN_POINT ( 'NONE',  ( 0.3949938075777409408, 0.1058382717557500574, -0.2821522309711286813 ) ) ;
#76866=CARTESIAN_POINT ( 'NONE',  ( -0.4724409448818896462, -0.1265901696524993070, -2.327427821522309426 ) ) ;
#76867=CARTESIAN_POINT ( 'NONE',  ( 0.1058382717557499880, 0.3949938075777409408, -1.172572178477690574 ) ) ;
#76872=CARTESIAN_POINT ( 'NONE',  ( -0.1265901696524993347, 0.4724409448818895907, -1.581364829396325389 ) ) ;
#76874=DIRECTION ( 'NONE',  ( 0.000000000000000000, 0.000000000000000000, 1.000000000000000000 ) ) ;
#76882=CARTESIAN_POINT ( 'NONE',  ( 4.797336870675655290E-17, -0.3917322834645669549, -1.891056799703724645 ) ) ;
#76883=CARTESIAN_POINT ( 'NONE',  ( 0.3460692066303959202, -0.1998031496062991630, -2.858923884514435798 ) ) ;
#76889=CARTESIAN_POINT ( 'NONE',  ( 0.2867679344610365999, 0.2867679344610365999, -1.389763779527558807 ) ) ;
#76892=CARTESIAN_POINT ( 'NONE',  ( -0.3949938075777409963, -7.255918531996591613E-17, -1.771653543307086576 ) ) ;
#76897=CARTESIAN_POINT ( 'NONE',  ( 0.2925321140481932369, -0.2925321140481932369, -0.2559055118110235560 ) ) ;
#76904=CARTESIAN_POINT ( 'NONE',  ( 0.1958661417322836440, -0.3392501089628017219, -0.4914698162729659869 ) ) ;
#76909=ORIENTED_EDGE ( 'NONE', *, *, #4894, .T. ) ;
#76911=CARTESIAN_POINT ( 'NONE',  ( -0.1070741851644051862, -0.3996062992125986590, -1.881233595800524849 ) ) ;
#76917=CARTESIAN_POINT ( 'NONE',  ( -0.2362204724409447953, -0.4091458600556404646, -1.010498687664042050 ) ) ;
#76920=CARTESIAN_POINT ( 'NONE',  ( 0.1958661417322834775, 0.3392501089628018884, 0.02099737532808403431 ) ) ;
#76921=CARTESIAN_POINT ( 'NONE',  ( 0.1049643490035304799, -0.3917322834645669549, -2.059711286089238591 ) ) ;
#76925=CARTESIAN_POINT ( 'NONE',  ( 0.4091458600556403535, 0.2362204724409449896, -2.570209973753280863 ) ) ;
#76928=EDGE_CURVE ( 'NONE', #34363, #64782, #55097, .T. ) ;
#76930=CARTESIAN_POINT ( 'NONE',  ( 0.1058382717557500852, -0.3949938075777408852, -2.681758530183727451 ) ) ;
#76937=CARTESIAN_POINT ( 'NONE',  ( 0.2867679344610365999, 0.2867679344610365999, -1.389763779527558807 ) ) ;
#76942=CARTESIAN_POINT ( 'NONE',  ( 0.1265901696524989462, 0.4724409448818897572, -0.07020997375328083545 ) ) ;
#76954=CARTESIAN_POINT ( 'NONE',  ( 0.3460692066303959202, -0.1998031496062991630, -0.9691601049868766582 ) ) ;
#76955=CARTESIAN_POINT ( 'NONE',  ( 0.3917322834645670104, -0.1049643490035303411, -2.085958005249344271 ) ) ;
#76966=CARTESIAN_POINT ( 'NONE',  ( -0.1958661417322836995, 0.3392501089628017219, -1.899625614994437495 ) ) ;
#76972=CARTESIAN_POINT ( 'NONE',  ( 4.797336870675656522E-17, -0.3917322834645670104, -2.053149606299212948 ) ) ;
#76980=CARTESIAN_POINT ( 'NONE',  ( -0.3996062992125986035, -7.340648628747425578E-17, -1.299212598425196985 ) ) ;
#76982=CARTESIAN_POINT ( 'NONE',  ( 0.2867679344610366554, -0.2867679344610365999, 0.06231664222341019160 ) ) ;
#76996=CARTESIAN_POINT ( 'NONE',  ( 0.3917322834645670104, 2.398668435337828261E-17, -0.2677165354330708347 ) ) ;
#76999=CARTESIAN_POINT ( 'NONE',  ( 0.3949938075777411073, -0.1058382717557499464, -0.4265091863517062043 ) ) ;
#77000=ORIENTED_EDGE ( 'NONE', *, *, #66685, .T. ) ;
#77006=CARTESIAN_POINT ( 'NONE',  ( -0.3917322834645670659, -7.196005306013484475E-17, -1.768392019193912423 ) ) ;
#77010=AXIS2_PLACEMENT_3D ( 'NONE', #13714, #34316, #47757 ) ;
#77013=CARTESIAN_POINT ( 'NONE',  ( 0.2925321140481932369, -0.2925321140481932369, -1.358267716535433101 ) ) ;
#77015=CARTESIAN_POINT ( 'NONE',  ( -0.3460692066303960313, 0.1998031496062989965, -0.7329396325459317518 ) ) ;
#77016=CARTESIAN_POINT ( 'NONE',  ( 0.3996062992125986035, -0.1070741851644052972, -0.1883202099737532609 ) ) ;
#77018=CARTESIAN_POINT ( 'NONE',  ( -0.1070741851644051862, -0.3996062992125987146, -2.591863517060367439 ) ) ;
#77019=CARTESIAN_POINT ( 'NONE',  ( -0.2867679344610365999, 0.2867679344610364889, -1.679133858267716661 ) ) ;
#77025=CARTESIAN_POINT ( 'NONE',  ( -0.1265901696524993347, 0.4724409448818895907, -1.500656167979002031 ) ) ;
#77029=CARTESIAN_POINT ( 'NONE',  ( 0.2891555358219910499, 0.2891555358219910499, -1.159448818897637956 ) ) ;
#77038=CARTESIAN_POINT ( 'NONE',  ( 0.1070741851644054776, -0.3996062992125984925, -2.209317585301837639 ) ) ;
#77040=CARTESIAN_POINT ( 'NONE',  ( -0.2867679344610364334, -0.2867679344610368219, -1.713891445373016520 ) ) ;
#77051=CARTESIAN_POINT ( 'NONE',  ( -0.2925321140481930149, -0.2925321140481933480, 0.1791338582677165503 ) ) ;
#77053=CARTESIAN_POINT ( 'NONE',  ( -0.3392501089628019995, 0.1958661417322832277, -1.055774278215223294 ) ) ;
#77062=CARTESIAN_POINT ( 'NONE',  ( 0.4724409448818915891, -0.1265901696524958653, -2.631233595800525293 ) ) ;
#77073=CARTESIAN_POINT ( 'NONE',  ( 0.1958661417322836440, -0.3392501089628017219, -2.603674540682414218 ) ) ;
#77076=CARTESIAN_POINT ( 'NONE',  ( 0.4724409448818896462, 0.1265901696524990294, -0.5971128608923884640 ) ) ;
#77078=CARTESIAN_POINT ( 'NONE',  ( 0.1998031496062992740, 0.3460692066303959757, 0.01312335958005247417 ) ) ;
#77082=CARTESIAN_POINT ( 'NONE',  ( -0.3392501089628019995, 0.1958661417322832277, -1.593175853018372612 ) ) ;
#77085=CARTESIAN_POINT ( 'NONE',  ( 0.4724409448818897572, -0.1265901696524988906, -2.946194225721785465 ) ) ;
#77092=CARTESIAN_POINT ( 'NONE',  ( -0.3917322834645669549, -7.196005306013483243E-17, -1.064285146160418360 ) ) ;
#77099=CARTESIAN_POINT ( 'NONE',  ( 0.3392501089628018884, -0.1958661417322833942, -2.463930076936694746 ) ) ;
#77107=CARTESIAN_POINT ( 'NONE',  ( 0.1049643490035304938, -0.3917322834645669549, -1.429790026246719359 ) ) ;
#77122=CARTESIAN_POINT ( 'NONE',  ( -0.3917322834645671215, 0.1049643490035301469, -1.219816272965879023 ) ) ;
#77123=CARTESIAN_POINT ( 'NONE',  ( -0.3458507752293909498, 0.3458507752293907833, -0.2539370078740156855 ) ) ;
#77126=CARTESIAN_POINT ( 'NONE',  ( 0.3420746716998660508, 0.1974969037888705814, 0.1069553805774278443 ) ) ;
#77132=CARTESIAN_POINT ( 'NONE',  ( -0.3420746716998662729, 0.1974969037888702206, -0.2604986876640420501 ) ) ;
#77139=CARTESIAN_POINT ( 'NONE',  ( -0.1070741851644056997, 0.3996062992125984925, -0.8707349081364830212 ) ) ;
#77141=CARTESIAN_POINT ( 'NONE',  ( 0.2867679344610365999, 0.2867679344610365999, -0.7598425196850391306 ) ) ;
#77158=CARTESIAN_POINT ( 'NONE',  ( 0.3458507752293908943, -0.3458507752293908943, -2.379921259842520342 ) ) ;
#77175=CARTESIAN_POINT ( 'NONE',  ( 0.3996062992125985480, 0.1070741851644054637, -0.2821522309711286258 ) ) ;
#77176=CARTESIAN_POINT ( 'NONE',  ( 0.3996062992125986035, -0.1070741851644052972, -2.865485564304462329 ) ) ;
#77181=CARTESIAN_POINT ( 'NONE',  ( -9.787531504996567848E-17, 0.3996062992125986035, -2.362204724409448620 ) ) ;
#77182=CARTESIAN_POINT ( 'NONE',  ( -0.2891555358219911054, 0.2891555358219909388, -2.066929133858268042 ) ) ;
#77183=CARTESIAN_POINT ( 'NONE',  ( 0.3392501089628018329, 0.1958661417322835607, -0.4383202099737532609 ) ) ;
#77185=CARTESIAN_POINT ( 'NONE',  ( 0.2867679344610366554, -0.2867679344610365444, -1.035433070866141447 ) ) ;
#77188=CARTESIAN_POINT ( 'NONE',  ( 0.3949938075777409408, -0.1058382717557499186, -2.550524934383202158 ) ) ;
#77192=CARTESIAN_POINT ( 'NONE',  ( -0.4724409448818895907, -0.1265901696524993070, -2.880577427821522374 ) ) ;
#77193=CARTESIAN_POINT ( 'NONE',  ( -0.3996062992125986035, -0.1070741851644056997, -2.093175853018372834 ) ) ;
#77194=CARTESIAN_POINT ( 'NONE',  ( 0.3392501089628018884, -0.1958661417322833942, -0.7316466123697656920 ) ) ;
#77202=CARTESIAN_POINT ( 'NONE',  ( -0.1049643490035302024, -0.3917322834645671215, -0.3143044619422573072 ) ) ;
#77210=CARTESIAN_POINT ( 'NONE',  ( -0.2867679344610364334, -0.2867679344610367109, -0.7736220472440945573 ) ) ;
#77211=CARTESIAN_POINT ( 'NONE',  ( 0.1049643490035303689, 0.3917322834645670104, -2.032808398950130879 ) ) ;
#77212=CARTESIAN_POINT ( 'NONE',  ( -0.2867679344610364334, -0.2867679344610367109, -2.885826771653543066 ) ) ;
#77214=CARTESIAN_POINT ( 'NONE',  ( 0.1974969037888706369, -0.3420746716998659953, -2.926509186351706315 ) ) ;
#77218=CARTESIAN_POINT ( 'NONE',  ( -0.3460692066303958092, -0.1998031496062994683, -1.312335958005249381 ) ) ;
#77220=CARTESIAN_POINT ( 'NONE',  ( 0.4724409448818898682, 2.892866454678787531E-17, -0.7480314960629921295 ) ) ;
#77223=CARTESIAN_POINT ( 'NONE',  ( 4.797336870675656522E-17, -0.3917322834645670104, -0.9507874015748032370 ) ) ;
#77232=CARTESIAN_POINT ( 'NONE',  ( -0.1265901696524986964, -0.4724409448818899238, -2.119422572178477626 ) ) ;
#77243=CARTESIAN_POINT ( 'NONE',  ( 4.797336870675655290E-17, -0.3917322834645669549, -0.7886945949793155997 ) ) ;
#77246=CARTESIAN_POINT ( 'NONE',  ( -0.1958661417322834220, -0.3392501089628018884, -0.9376640419947508409 ) ) ;
#77252=CARTESIAN_POINT ( 'NONE',  ( -0.3917322834645669549, -0.1049643490035306603, -2.557742782152230721 ) ) ;
#77255=CARTESIAN_POINT ( 'NONE',  ( 0.4091458600556404646, -0.2362204724409448231, -1.126640419947506633 ) ) ;
#77268=CARTESIAN_POINT ( 'NONE',  ( 0.3996062992125985480, 2.446882876249141654E-17, -2.557086614173228689 ) ) ;
#77272=CARTESIAN_POINT ( 'NONE',  ( -0.1998031496062994405, 0.3460692066303957537, -1.192257217847769057 ) ) ;
#77278=CARTESIAN_POINT ( 'NONE',  ( -0.1998031496062991630, -0.3460692066303959202, -0.4573490813648293796 ) ) ;
#77279=CARTESIAN_POINT ( 'NONE',  ( -9.787531504996567848E-17, 0.3996062992125986035, -0.7874015748031496509 ) ) ;
#77280=CARTESIAN_POINT ( 'NONE',  ( 0.1058382717557500713, -0.3949938075777409408, -0.5577427821522310536 ) ) ;
#77286=CARTESIAN_POINT ( 'NONE',  ( -0.1058382717557503072, 0.3949938075777408852, -1.185695538057742748 ) ) ;
#77291=CARTESIAN_POINT ( 'NONE',  ( 0.3458507752293908943, 0.3458507752293908943, -1.397637795275590067 ) ) ;
#77292=CARTESIAN_POINT ( 'NONE',  ( -9.787531504996567848E-17, 0.3996062992125986035, -2.677165354330708347 ) ) ;
#77293=( BOUNDED_CURVE ( )  B_SPLINE_CURVE ( 2, ( #67368, #10121, #76155, #56366, #49637, #62272, #37837, #18085, #75330, #11777, #12179, #24785, #61863 ),
 .UNSPECIFIED., .F., .F. ) 
 B_SPLINE_CURVE_WITH_KNOTS ( ( 3, 2, 2, 2, 2, 2, 3 ),
 ( 0.1875000000000000000, 0.1916666666666666796, 0.1958333333333333315, 0.2000000000000000111, 0.2041666666666666907, 0.2083333333333333703, 0.2125000000000000222 ),
 .UNSPECIFIED. ) 
 CURVE ( )  GEOMETRIC_REPRESENTATION_ITEM ( )  RATIONAL_B_SPLINE_CURVE ( ( 1.000000000000000000, 0.9659258262890683122, 1.000000000000000000, 0.9659258262890683122, 1.000000000000000000, 0.9659258262890683122, 1.000000000000000000, 0.9659258262890683122, 1.000000000000000000, 0.9659258262890683122, 1.000000000000000000, 0.9659258262890680902, 1.000000000000000222 ) ) 
 REPRESENTATION_ITEM ( '' )  );
#77300=CARTESIAN_POINT ( 'NONE',  ( -0.3392501089628018329, -0.1958661417322836440, -2.022290395504250160 ) ) ;
#77309=CARTESIAN_POINT ( 'NONE',  ( -0.1049643490035302024, -0.3917322834645671215, -1.639107611548556109 ) ) ;
#77312=CARTESIAN_POINT ( 'NONE',  ( 0.3949938075777409408, 0.1058382717557500574, -1.856955380577427928 ) ) ;
#77317=CARTESIAN_POINT ( 'NONE',  ( -0.2925321140481930704, -0.2925321140481933480, -0.2165354330708661734 ) ) ;
#77324=CARTESIAN_POINT ( 'NONE',  ( 0.1049643490035304938, -0.3917322834645669549, -0.1699475065616798397 ) ) ;
#77331=CARTESIAN_POINT ( 'NONE',  ( 4.893765752498283308E-17, -0.3996062992125985480, -2.045275590551181022 ) ) ;
#77336=CARTESIAN_POINT ( 'NONE',  ( 0.3458507752293908943, 0.3458507752293908943, -0.9251968503937008093 ) ) ;
#77339=CARTESIAN_POINT ( 'NONE',  ( -0.3392501089628019995, 0.1958661417322832277, -0.1758530183727033402 ) ) ;
#77340=CARTESIAN_POINT ( 'NONE',  ( -0.4724409448818898682, -8.678599364036362592E-17, -0.7460629921259841479 ) ) ;
#77344=CARTESIAN_POINT ( 'NONE',  ( -0.1265901696524986964, -0.4724409448818899238, -2.668635170603674833 ) ) ;
#77348=CARTESIAN_POINT ( 'NONE',  ( 0.1058382717557499880, 0.3949938075777409408, -2.747375328083990098 ) ) ;
#77355=PRODUCT_DEFINITION_CONTEXT ( 'detailed design', #74523, 'design' ) ;
#77357=CARTESIAN_POINT ( 'NONE',  ( 0.3392501089628018329, 0.1958661417322835607, -1.383202099737532942 ) ) ;
#77360=CARTESIAN_POINT ( 'NONE',  ( -0.1265901696524993347, 0.4724409448818895907, -0.08333333333333335646 ) ) ;
#77372=CARTESIAN_POINT ( 'NONE',  ( 0.1998031496062994128, -0.3460692066303957537, -0.9560367454068241511 ) ) ;
#77373=CARTESIAN_POINT ( 'NONE',  ( -0.2867679344610365999, 0.2867679344610364889, -2.466535433070865757 ) ) ;
#77383=CARTESIAN_POINT ( 'NONE',  ( -0.4724409448818898682, 5.785732909357575061E-17, -2.755905511811024056 ) ) ;
#77384=CARTESIAN_POINT ( 'NONE',  ( 0.1958661417322836718, -0.3392501089628017219, -2.135846087435382401 ) ) ;
#77391=CARTESIAN_POINT ( 'NONE',  ( 4.797336870675656522E-17, -0.3917322834645670104, -1.895669291338582640 ) ) ;
#77395=FACE_OUTER_BOUND ( 'NONE', #51934, .T. ) ;
#77398=CARTESIAN_POINT ( 'NONE',  ( 0.1998031496062994405, -0.3460692066303958092, -1.194225721784776928 ) ) ;
#77400=CARTESIAN_POINT ( 'NONE',  ( 0.1958661417322836718, -0.3392501089628017219, -0.08860199294719349472 ) ) ;
#77401=ORIENTED_EDGE ( 'NONE', *, *, #78409, .F. ) ;
#77413=CARTESIAN_POINT ( 'NONE',  ( 0.3392501089628018329, 0.1958661417322835607, -0.2808398950131232863 ) ) ;
#77416=CARTESIAN_POINT ( 'NONE',  ( -0.3949938075777411628, 0.1058382717557497937, -0.6627296587926508886 ) ) ;
#77425=CARTESIAN_POINT ( 'NONE',  ( -0.3917322834645670104, -0.1049643490035307020, -1.774953698983938954 ) ) ;
#77431=CARTESIAN_POINT ( 'NONE',  ( -9.787531504996567848E-17, 0.3996062992125986035, -1.259842519685039353 ) ) ;
#77433=CARTESIAN_POINT ( 'NONE',  ( 0.3460692066303958092, 0.1998031496062993018, -0.6804461942257218343 ) ) ;
#77434=CARTESIAN_POINT ( 'NONE',  ( -0.3996062992125986590, 0.1070741851644051723, 0.04790026246719156916 ) ) ;
#77436=CARTESIAN_POINT ( 'NONE',  ( -0.1998031496062991907, -0.3460692066303959757, -2.742782152230971437 ) ) ;
#77438=CARTESIAN_POINT ( 'NONE',  ( 0.1049643490035303689, 0.3917322834645670104, -2.125328083989501682 ) ) ;
#77445=CARTESIAN_POINT ( 'NONE',  ( 0.4724409448818896462, 0.1265901696524990294, -1.618766404199474929 ) ) ;
#77448=CARTESIAN_POINT ( 'NONE',  ( -0.3420746716998660508, -0.1974969037888706924, -1.389107611548556553 ) ) ;
#77458=CARTESIAN_POINT ( 'NONE',  ( 0.3996062992125984925, 0.1070741851644054637, -2.091207349081364963 ) ) ;
#77460=CARTESIAN_POINT ( 'NONE',  ( 0.1958661417322834497, 0.3392501089628018329, -1.956673597603987957 ) ) ;
#77469=CARTESIAN_POINT ( 'NONE',  ( -0.3458507752293909498, 0.3458507752293908388, -2.381889763779527769 ) ) ;
#77473=CARTESIAN_POINT ( 'NONE',  ( -0.2925321140481932369, 0.2925321140481931259, 0.2185039370078740162 ) ) ;
#77476=CARTESIAN_POINT ( 'NONE',  ( -0.3392501089628017219, -0.1958661417322836718, -1.396981627296587813 ) ) ;
#77497=CARTESIAN_POINT ( 'NONE',  ( -0.3392501089628019995, 0.1958661417322832277, -2.538057742782152015 ) ) ;
#77501=CARTESIAN_POINT ( 'NONE',  ( 0.3458507752293908943, -0.3458507752293908943, -0.8858267716535430658 ) ) ;
#77502=CARTESIAN_POINT ( 'NONE',  ( -0.3996062992125986035, -0.1070741851644056997, 0.1115485564304461580 ) ) ;
#77505=CARTESIAN_POINT ( 'NONE',  ( -0.1049643490035307020, 0.3917322834645669549, -1.888451443569553412 ) ) ;
#77509=CARTESIAN_POINT ( 'NONE',  ( 5.785732909357575061E-17, -0.4724409448818898682, -2.755905511811023612 ) ) ;
#77516=CARTESIAN_POINT ( 'NONE',  ( -0.2867679344610366554, 0.2867679344610365444, -1.202080421750969741 ) ) ;
#77523=CARTESIAN_POINT ( 'NONE',  ( -0.1049643490035302301, -0.3917322834645671770, -2.273641363025933781 ) ) ;
#77525=ORIENTED_EDGE ( 'NONE', *, *, #81282, .T. ) ;
#77532=CARTESIAN_POINT ( 'NONE',  ( 4.797336870675656522E-17, -0.3917322834645670104, -1.738188976377952777 ) ) ;
#77550=CARTESIAN_POINT ( 'NONE',  ( 0.1265901696524990572, -0.4724409448818897017, -0.4002624671916010235 ) ) ;
#77551=CARTESIAN_POINT ( 'NONE',  ( 0.4724409448818898682, 2.892866454678787531E-17, -0.1948818897637795422 ) ) ;
#77554=CARTESIAN_POINT ( 'NONE',  ( 0.3949938075777409408, -0.1058382717557499186, -0.1883202099737532886 ) ) ;
#77559=CARTESIAN_POINT ( 'NONE',  ( -0.3949938075777408852, -0.1058382717557502933, 0.03477690288713909672 ) ) ;
#77566=CARTESIAN_POINT ( 'NONE',  ( -0.1998031496062991630, -0.3460692066303959202, -0.7723097112860892732 ) ) ;
#77568=CARTESIAN_POINT ( 'NONE',  ( -0.3917322834645671215, 0.1049643490035301469, -0.8123359580052491591 ) ) ;
#77570=CARTESIAN_POINT ( 'NONE',  ( -0.1265901696524986964, -0.4724409448818899238, -0.4639107611548556331 ) ) ;
#77584=CARTESIAN_POINT ( 'NONE',  ( -0.2362204724409447953, -0.4091458600556404646, -2.662073490813648746 ) ) ;
#77601=CARTESIAN_POINT ( 'NONE',  ( -0.3996062992125986590, 0.1070741851644051862, -0.1902887139107611592 ) ) ;
#77607=CARTESIAN_POINT ( 'NONE',  ( -0.1998031496062991907, -0.3460692066303959757, -2.427821522309711266 ) ) ;
#77608=CARTESIAN_POINT ( 'NONE',  ( 0.3420746716998659953, 0.1974969037888705536, -1.863517060367453793 ) ) ;
#77609=CARTESIAN_POINT ( 'NONE',  ( -0.3392501089628019995, 0.1958661417322832277, -0.6482939632545930975 ) ) ;
#77611=CARTESIAN_POINT ( 'NONE',  ( 0.3392501089628018884, -0.1958661417322834220, -0.8845144356955378928 ) ) ;
#77613=CARTESIAN_POINT ( 'NONE',  ( 0.1958661417322836440, -0.3392501089628017219, -1.028871391076115360 ) ) ;
#77615=CARTESIAN_POINT ( 'NONE',  ( 0.3917322834645669549, 2.398668435337827645E-17, 0.1168172160443062824 ) ) ;
#77621=CARTESIAN_POINT ( 'NONE',  ( 0.1070741851644053527, 0.3996062992125986590, -2.670603674540682260 ) ) ;
#77622=CARTESIAN_POINT ( 'NONE',  ( 4.797336870675656522E-17, -0.3917322834645670659, -1.177840838091550602 ) ) ;
#77628=CARTESIAN_POINT ( 'NONE',  ( -9.594673741351313045E-17, 0.3917322834645670104, -0.7145669291338584417 ) ) ;
#77637=CARTESIAN_POINT ( 'NONE',  ( -0.1958661417322836718, 0.3392501089628017219, -1.737532808398950079 ) ) ;
#77640=CARTESIAN_POINT ( 'NONE',  ( -0.1070741851644056997, 0.3996062992125986035, 0.1509186351706036100 ) ) ;
#77644=CARTESIAN_POINT ( 'NONE',  ( -0.4091458600556405756, 0.2362204724409446288, -2.465223097112860806 ) ) ;
#77647=CARTESIAN_POINT ( 'NONE',  ( 0.1049643490035304938, -0.3917322834645669549, -0.7998687664041995715 ) ) ;
#77667=CARTESIAN_POINT ( 'NONE',  ( 0.2867679344610365999, 0.2867679344610365999, -0.8477497130895521593 ) ) ;
#77671=CARTESIAN_POINT ( 'NONE',  ( -0.1265901696524993347, 0.4724409448818896462, -0.7939632545931758489 ) ) ;
#77677=CARTESIAN_POINT ( 'NONE',  ( 0.3917322834645670104, 0.1049643490035304660, -0.1214103918973247487 ) ) ;
#77680=CARTESIAN_POINT ( 'NONE',  ( -0.4724409448818895907, -0.1265901696524993070, -1.225065616797899937 ) ) ;
#77694=CARTESIAN_POINT ( 'NONE',  ( 0.3460692066303958092, 0.1998031496062993018, -2.412729658792650778 ) ) ;
#77698=CARTESIAN_POINT ( 'NONE',  ( 0.3996062992125985480, 2.446882876249141654E-17, -1.612204724409448842 ) ) ;
#77704=CARTESIAN_POINT ( 'NONE',  ( 0.3996062992125984925, 0.1070741851644054499, -0.9888451443569553634 ) ) ;
#77705=CARTESIAN_POINT ( 'NONE',  ( 0.2925321140481932369, -0.2925321140481932369, -1.200787401574803015 ) ) ;
#77706=CARTESIAN_POINT ( 'NONE',  ( 0.1974969037888706369, -0.3420746716998659953, -0.5643044619422573627 ) ) ;
#77712=CARTESIAN_POINT ( 'NONE',  ( -0.1058382717557497660, -0.3949938075777411073, -1.881233595800524849 ) ) ;
#77717=CARTESIAN_POINT ( 'NONE',  ( -0.3458507752293909498, 0.3458507752293907833, -1.751968503937007648 ) ) ;
#77726=CARTESIAN_POINT ( 'NONE',  ( -9.594673741351310580E-17, 0.3917322834645669549, -2.127277272144670217 ) ) ;
#77733=CARTESIAN_POINT ( 'NONE',  ( 0.2867679344610365999, -0.2867679344610365444, -1.507874015748031260 ) ) ;
#77736=CARTESIAN_POINT ( 'NONE',  ( -0.3420746716998659953, -0.1974969037888706647, -1.942257217847769279 ) ) ;
#77741=CARTESIAN_POINT ( 'NONE',  ( 0.2925321140481932369, -0.2925321140481932369, -0.7283464566929134243 ) ) ;
#77749=CARTESIAN_POINT ( 'NONE',  ( 0.3392501089628018884, -0.1958661417322834220, -0.1896325459317586282 ) ) ;
#77754=ORIENTED_EDGE ( 'NONE', *, *, #68913, .T. ) ;
#77756=CARTESIAN_POINT ( 'NONE',  ( -0.2925321140481932369, 0.2925321140481931259, -1.986220472440944906 ) ) ;
#77759=PLANE ( 'NONE',  #37961 ) ;
#77761=CARTESIAN_POINT ( 'NONE',  ( 0.4724409448818896462, 0.1265901696524990294, -0.7545931758530182165 ) ) ;
#77763=CARTESIAN_POINT ( 'NONE',  ( 0.3917322834645670104, -0.1049643490035303411, -0.4186351706036745557 ) ) ;
#77768=CARTESIAN_POINT ( 'NONE',  ( -0.3460692066303960313, 0.1998031496062989965, 0.2119422572178477349 ) ) ;
#77773=CARTESIAN_POINT ( 'NONE',  ( -0.3949938075777411073, 0.1058382717557497660, -2.786745406824147064 ) ) ;
#77780=CARTESIAN_POINT ( 'NONE',  ( -0.3917322834645670104, -7.196005306013484475E-17, -1.606299212598425452 ) ) ;
#77783=B_SPLINE_CURVE_WITH_KNOTS ( 'NONE', 3,
 ( #33017, #59519, #46882, #53611, #8604, #58687, #46051, #21227, #34275, #21639, #26284, #59936, #51945, #52362, #39328, #27118, #33446, #1462 ),
 .UNSPECIFIED., .F., .F.,
 ( 4, 2, 2, 2, 2, 2, 2, 2, 4 ),
 ( 5.794108576630504547E-15, 2.503579458505735792E-05, 5.007158916432061067E-05, 0.0001001431783228451036, 0.0002002863566398940896, 0.0004005727132739911127, 0.0008011454265421859722, 0.001602290853078575149, 0.003204581706151352419 ),
 .UNSPECIFIED. ) ;
#77784=CARTESIAN_POINT ( 'NONE',  ( 0.1265901696524989462, 0.4724409448818897572, 0.08727034120734905587 ) ) ;
#77788=CARTESIAN_POINT ( 'NONE',  ( -0.1265901696524993347, 0.4724409448818896462, -0.7132545931758530466 ) ) ;
#77798=CARTESIAN_POINT ( 'NONE',  ( -0.3996062992125984925, -0.1070741851644056858, -1.067585301837270517 ) ) ;
#77799=CARTESIAN_POINT ( 'NONE',  ( 0.2867679344610365999, 0.2867679344610365999, -2.742125984251967630 ) ) ;
#77805=( BOUNDED_CURVE ( )  B_SPLINE_CURVE ( 2, ( #19696, #46612, #1192, #13815, #58834, #8329, #27677, #77788, #20121, #79051, #46192, #71888, #27257 ),
 .UNSPECIFIED., .F., .F. ) 
 B_SPLINE_CURVE_WITH_KNOTS ( ( 3, 2, 2, 2, 2, 2, 3 ),
 ( 0.2875000000000000333, 0.2916666666666667407, 0.2958333333333333925, 0.3000000000000000444, 0.3041666666666666408, 0.3083333333333333481, 0.3125000000000000000 ),
 .UNSPECIFIED. ) 
 CURVE ( )  GEOMETRIC_REPRESENTATION_ITEM ( )  RATIONAL_B_SPLINE_CURVE ( ( 0.9999999999999995559, 0.9659258262890687563, 1.000000000000000000, 0.9659258262890683122, 1.000000000000000000, 0.9659258262890683122, 1.000000000000000000, 0.9659258262890683122, 1.000000000000000000, 0.9659258262890683122, 1.000000000000000000, 0.9659258262890683122, 1.000000000000000000 ) ) 
 REPRESENTATION_ITEM ( '' )  );
#77809=LINE ( 'NONE', #77383, #17924 ) ;
#77810=CARTESIAN_POINT ( 'NONE',  ( -0.1049643490035302301, -0.3917322834645671770, -2.431121677986564311 ) ) ;
#77812=CARTESIAN_POINT ( 'NONE',  ( 0.006307039255732630779, -0.3948371832379766189, -2.032323646524576638E-15 ) ) ;
#77816=CARTESIAN_POINT ( 'NONE',  ( 0.2867679344610365999, 0.2867679344610365999, -1.954724409448818978 ) ) ;
#77824=CARTESIAN_POINT ( 'NONE',  ( -0.3996062992125987146, 0.1070741851644051862, -1.292650918635170454 ) ) ;
#77826=CARTESIAN_POINT ( 'NONE',  ( -0.1958661417322833942, -0.3392501089628018884, -0.06235527378708850127 ) ) ;
#77838=CARTESIAN_POINT ( 'NONE',  ( 0.3917322834645670104, 2.398668435337828261E-17, -0.1102362204724409017 ) ) ;
#77841=CARTESIAN_POINT ( 'NONE',  ( -0.1974969037888703871, -0.3420746716998661063, -0.6955380577427822120 ) ) ;
#77855=CARTESIAN_POINT ( 'NONE',  ( 0.2925321140481932369, -0.2925321140481932369, -1.200787401574803015 ) ) ;
#77857=CARTESIAN_POINT ( 'NONE',  ( 0.1070741851644053388, 0.3996062992125986035, -0.8576115485564304031 ) ) ;
#77858=CARTESIAN_POINT ( 'NONE',  ( 0.3996062992125985480, 2.446882876249141654E-17, -0.03740157480314963701 ) ) ;
#77860=CARTESIAN_POINT ( 'NONE',  ( 0.2925321140481932369, 0.2925321140481932369, -2.500000000000000444 ) ) ;
#77861=CARTESIAN_POINT ( 'NONE',  ( -9.594673741351313045E-17, 0.3917322834645670104, -1.974409448818897683 ) ) ;
#77867=CARTESIAN_POINT ( 'NONE',  ( -0.1265901696524993347, 0.4724409448818895907, -1.658136482939632117 ) ) ;
#77870=CARTESIAN_POINT ( 'NONE',  ( 0.3949938075777409963, 2.418639510665530743E-17, -1.297244094488188892 ) ) ;
#77873=CARTESIAN_POINT ( 'NONE',  ( -0.4724409448818898682, -8.678599364036362592E-17, -0.8267716535433070613 ) ) ;
#77880=CARTESIAN_POINT ( 'NONE',  ( 0.3996062992125986035, -0.1070741851644052972, -2.235564304461942431 ) ) ;
#77882=CARTESIAN_POINT ( 'NONE',  ( 0.1958661417322834497, 0.3392501089628018329, -2.114153912564617599 ) ) ;
#77896=CARTESIAN_POINT ( 'NONE',  ( 0.1998031496062992463, 0.3460692066303959202, 0.09383202099737532331 ) ) ;
#77898=CARTESIAN_POINT ( 'NONE',  ( 0.3917322834645669549, 0.1049643490035304660, -1.469160104986876769 ) ) ;
#77919=CARTESIAN_POINT ( 'NONE',  ( -0.1958661417322834220, -0.3392501089628018884, -2.262467191601049699 ) ) ;
#77922=CARTESIAN_POINT ( 'NONE',  ( 0.2362204724409451007, -0.4091458600556402980, -0.5643044619422572516 ) ) ;
#77923=CARTESIAN_POINT ( 'NONE',  ( 0.1998031496062994405, -0.3460692066303958092, 0.06561679790026245240 ) ) ;
#77926=CARTESIAN_POINT ( 'NONE',  ( -0.3917322834645671215, 0.1049643490035301469, -1.599737532808399143 ) ) ;
#77930=CARTESIAN_POINT ( 'NONE',  ( -1.157146581871515012E-16, 0.4724409448818898682, -2.677165354330708347 ) ) ;
#77937=CARTESIAN_POINT ( 'NONE',  ( 0.3917322834645668994, 0.1049643490035304522, -0.9921066684701294047 ) ) ;
#77944=CARTESIAN_POINT ( 'NONE',  ( -0.3392501089628019995, 0.1958661417322831999, -2.385189919456379926 ) ) ;
#77953=CARTESIAN_POINT ( 'NONE',  ( -0.3917322834645671215, 0.1049643490035301469, -1.692257217847769057 ) ) ;
#77964=ORIENTED_EDGE ( 'NONE', *, *, #6890, .T. ) ;
#77969=CARTESIAN_POINT ( 'NONE',  ( 0.4091458600556404646, -0.2362204724409448231, -0.3392388451443569819 ) ) ;
#77972=CARTESIAN_POINT ( 'NONE',  ( 0.3420746716998660508, -0.1974969037888704149, -0.02427821522309712640 ) ) ;
#77977=CARTESIAN_POINT ( 'NONE',  ( -9.674558042662122972E-17, 0.3949938075777409963, 0.08070866141732281618 ) ) ;
#77985=CARTESIAN_POINT ( 'NONE',  ( 0.3996062992125986035, -0.1070741851644052972, -0.8182414698162727706 ) ) ;
#77987=CARTESIAN_POINT ( 'NONE',  ( -0.3917322834645670104, -7.196005306013484475E-17, -0.8188976377952754682 ) ) ;
#78001=CARTESIAN_POINT ( 'NONE',  ( -0.3970677821444029698, -0.02963302784745281207, -1.220472440944882386 ) ) ;
#78003=CARTESIAN_POINT ( 'NONE',  ( 0.1998031496062994128, -0.3460692066303957537, 0.1463254593175852825 ) ) ;
#78020=CARTESIAN_POINT ( 'NONE',  ( 4.893765752498283924E-17, -0.3996062992125986035, -0.3937007874015748254 ) ) ;
#78021=CARTESIAN_POINT ( 'NONE',  ( 0.4091458600556403535, 0.2362204724409449896, -1.152887139107611425 ) ) ;
#78025=CARTESIAN_POINT ( 'NONE',  ( 0.2925321140481932369, -0.2925321140481932369, -2.618110236220472675 ) ) ;
#78026=CARTESIAN_POINT ( 'NONE',  ( -0.1974969037888703871, -0.3420746716998661063, -2.112860892388451539 ) ) ;
#78027=CARTESIAN_POINT ( 'NONE',  ( -0.1049643490035307020, 0.3917322834645669549, -0.4711286089238844177 ) ) ;
#78029=CARTESIAN_POINT ( 'NONE',  ( -9.594673741351313045E-17, 0.3917322834645670104, -1.094488188976378007 ) ) ;
#78031=CARTESIAN_POINT ( 'NONE',  ( -0.3392501089628019995, 0.1958661417322832277, -1.120734908136482799 ) ) ;
#78033=CARTESIAN_POINT ( 'NONE',  ( 0.1049643490035304522, -0.3917322834645668994, -0.007854699966192403571 ) ) ;
#78039=CARTESIAN_POINT ( 'NONE',  ( -0.1070741851644056997, 0.3996062992125986035, -2.526246719160104792 ) ) ;
#78040=CARTESIAN_POINT ( 'NONE',  ( -0.3392501089628017219, -0.1958661417322836995, -1.309074433892075451 ) ) ;
#78043=EDGE_CURVE ( 'NONE', #58583, #15221, #56214, .T. ) ;
#78047=CARTESIAN_POINT ( 'NONE',  ( -0.3917322834645670104, -7.196005306013484475E-17, -0.5964566929133858775 ) ) ;
#78055=CARTESIAN_POINT ( 'NONE',  ( 0.2798680777852625701, -0.2749078412849261244, -1.929133858267715773 ) ) ;
#78056=CARTESIAN_POINT ( 'NONE',  ( -0.2867679344610364334, -0.2867679344610367109, -2.098425196850393526 ) ) ;
#78058=CARTESIAN_POINT ( 'NONE',  ( -0.3996062992125987146, 0.1070741851644051862, -0.1902887139107611592 ) ) ;
#78062=CARTESIAN_POINT ( 'NONE',  ( -0.3458507752293909498, 0.3458507752293908388, -2.458661417322834719 ) ) ;
#78065=CARTESIAN_POINT ( 'NONE',  ( 4.797336870675656522E-17, -0.3917322834645670104, -0.7933070866141732624 ) ) ;
#78075=CARTESIAN_POINT ( 'NONE',  ( 0.4724409448818880919, 0.1265901696525020825, -2.644356955380577467 ) ) ;
#78085=CARTESIAN_POINT ( 'NONE',  ( 0.3392501089628018329, 0.1958661417322835052, -0.8411880332995258502 ) ) ;
#78089=CARTESIAN_POINT ( 'NONE',  ( -9.594673741351313045E-17, 0.3917322834645670104, -1.187007874015748143 ) ) ;
#78095=CARTESIAN_POINT ( 'NONE',  ( -0.1049643490035302301, -0.3917322834645671770, 0.08856336138351518505 ) ) ;
#78098=CARTESIAN_POINT ( 'NONE',  ( -0.2362204724409451284, 0.4091458600556402425, -1.349737532808398921 ) ) ;
#78107=CYLINDRICAL_SURFACE ( 'NONE', #77010, 0.4724409448818898682 ) ;
#78113=CARTESIAN_POINT ( 'NONE',  ( 0.1998031496062994128, -0.3460692066303957537, -2.373359580052493367 ) ) ;
#78117=CARTESIAN_POINT ( 'NONE',  ( 0.1070741851644054776, -0.3996062992125984925, -1.894356955380577023 ) ) ;
#78123=CARTESIAN_POINT ( 'NONE',  ( 0.1070741851644053527, 0.3996062992125985480, -1.172572178477690352 ) ) ;
#78124=CARTESIAN_POINT ( 'NONE',  ( -0.2925321140481932924, 0.2925321140481931814, -1.279527559055118058 ) ) ;
#78125=CARTESIAN_POINT ( 'NONE',  ( -9.674558042662121740E-17, 0.3949938075777409963, -0.7874015748031496509 ) ) ;
#78129=COLOUR_RGB ( '', 0.31764706, 0.68627451, 0.89019608) ;
#78132=CARTESIAN_POINT ( 'NONE',  ( 0.2891555358219910499, 0.2891555358219910499, -1.946850393700787496 ) ) ;
#78137=CARTESIAN_POINT ( 'NONE',  ( 0.4724409448818898682, 2.892866454678787531E-17, -2.165354330708661568 ) ) ;
#78139=VERTEX_POINT ( 'NONE', #79465 ) ;
#78145=CARTESIAN_POINT ( 'NONE',  ( 0.3392501089628018329, 0.1958661417322835052, -2.258510867945195066 ) ) ;
#78146=CARTESIAN_POINT ( 'NONE',  ( 0.1998031496062994128, -0.3460692066303957537, -2.845800524934383624 ) ) ;
#78152=CARTESIAN_POINT ( 'NONE',  ( -0.3392501089628018329, -0.1958661417322836440, -2.652211655346770502 ) ) ;
#78154=CARTESIAN_POINT ( 'NONE',  ( -0.2867679344610364334, -0.2867679344610367109, -1.783464566929133577 ) ) ;
#78157=CARTESIAN_POINT ( 'NONE',  ( 0.3420746716998660508, -0.1974969037888703871, -1.994750656167979086 ) ) ;
#78162=CARTESIAN_POINT ( 'NONE',  ( 0.3460692066303959757, -0.1998031496062991907, -0.7349081364829396223 ) ) ;
#78170=CARTESIAN_POINT ( 'NONE',  ( -0.3392501089628017219, -0.1958661417322836718, -0.2946194225721785465 ) ) ;
#78177=CARTESIAN_POINT ( 'NONE',  ( 0.1998031496062992463, 0.3460692066303959202, -1.953412073490813805 ) ) ;
#78180=DIRECTION ( 'NONE',  ( 0.000000000000000000, 0.000000000000000000, 1.000000000000000000 ) ) ;
#78182=CARTESIAN_POINT ( 'NONE',  ( 0.2362204724409449064, 0.4091458600556404646, -1.089238845144356871 ) ) ;
#78184=CARTESIAN_POINT ( 'NONE',  ( -0.3917322834645670104, -7.196005306013484475E-17, -0.1889763779527558474 ) ) ;
#78185=CARTESIAN_POINT ( 'NONE',  ( 0.3917322834645670104, -0.1049643490035303273, -2.558398950131233196 ) ) ;
#78189=CARTESIAN_POINT ( 'NONE',  ( -0.2925321140481932369, 0.2925321140481931259, 0.06102362204724406242 ) ) ;
#78194=CARTESIAN_POINT ( 'NONE',  ( 0.3949938075777409408, -0.1058382717557499186, -2.550524934383202158 ) ) ;
#78202=CARTESIAN_POINT ( 'NONE',  ( -0.3392501089628017219, -0.1958661417322836718, -1.934383202099737575 ) ) ;
#78205=CARTESIAN_POINT ( 'NONE',  ( 0.3458507752293908943, -0.3458507752293908943, -0.01771653543307087630 ) ) ;
#78218=CARTESIAN_POINT ( 'NONE',  ( 0.1998031496062994128, -0.3460692066303957537, -1.270997375328083878 ) ) ;
#78219=CARTESIAN_POINT ( 'NONE',  ( 0.3392501089628018329, 0.1958661417322835607, -2.578083989501311901 ) ) ;
#78228=CARTESIAN_POINT ( 'NONE',  ( 4.893765752498283924E-17, -0.3996062992125986035, -0.07874015748031498729 ) ) ;
#78229=CARTESIAN_POINT ( 'NONE',  ( 0.2867679344610366554, 0.2867679344610366554, -2.339258160926195984 ) ) ;
#78236=CARTESIAN_POINT ( 'NONE',  ( 0.3917322834645670104, 2.398668435337828261E-17, -2.407480314960630086 ) ) ;
#78242=CARTESIAN_POINT ( 'NONE',  ( 0.3460692066303959757, -0.1998031496062991907, -1.994750656167979086 ) ) ;
#78244=CARTESIAN_POINT ( 'NONE',  ( 0.3996062992125986035, 2.446882876249141962E-17, -1.220472440944881942 ) ) ;
#78246=CARTESIAN_POINT ( 'NONE',  ( 0.2867679344610366554, 0.2867679344610366554, -0.1345337514773772281 ) ) ;
#78258=CARTESIAN_POINT ( 'NONE',  ( -0.1049643490035302024, -0.3917322834645671215, -0.6942257217847765949 ) ) ;
#78261=CARTESIAN_POINT ( 'NONE',  ( -9.674558042662121740E-17, 0.3949938075777409963, -0.4724409448818898127 ) ) ;
#78276=CARTESIAN_POINT ( 'NONE',  ( -0.1070741851644051862, -0.3996062992125987146, -1.332020997375328086 ) ) ;
#78278=CARTESIAN_POINT ( 'NONE',  ( -0.1998031496062991630, -0.3460692066303959202, -0.9297900262467192478 ) ) ;
#78279=CARTESIAN_POINT ( 'NONE',  ( 0.3996062992125985480, 2.446882876249141654E-17, -0.3523622047244094335 ) ) ;
#78282=CARTESIAN_POINT ( 'NONE',  ( -0.4724409448818898682, -8.678599364036362592E-17, -0.1968503937007874127 ) ) ;
#78283=CARTESIAN_POINT ( 'NONE',  ( 0.3392501089628018884, -0.1958661417322834220, -2.236876640419947826 ) ) ;
#78289=CARTESIAN_POINT ( 'NONE',  ( 0.4724409448818898682, 2.892866454678787531E-17, -2.084645669291338432 ) ) ;
#78292=CARTESIAN_POINT ( 'NONE',  ( 0.1974969037888706092, -0.3420746716998660508, -1.428477690288714186 ) ) ;
#78302=CARTESIAN_POINT ( 'NONE',  ( 0.1998031496062994128, -0.3460692066303957537, -2.058398950131233640 ) ) ;
#78303=CARTESIAN_POINT ( 'NONE',  ( 0.1958661417322834497, 0.3392501089628018329, -2.271634227525247685 ) ) ;
#78315=AXIS2_PLACEMENT_3D ( 'NONE', #22830, #74190, #16536 ) ;
#78317=CARTESIAN_POINT ( 'NONE',  ( -0.3460692066303957537, -0.1998031496062994405, 0.1856955380577427484 ) ) ;
#78319=CARTESIAN_POINT ( 'NONE',  ( -0.2867679344610365999, 0.2867679344610364889, -1.206692913385826627 ) ) ;
#78341=CARTESIAN_POINT ( 'NONE',  ( -0.2867679344610366554, 0.2867679344610365444, -2.374015748031496287 ) ) ;
#78344=CARTESIAN_POINT ( 'NONE',  ( 0.3996062992125986035, 0.1070741851644054776, 0.03280839895013121232 ) ) ;
#78347=CARTESIAN_POINT ( 'NONE',  ( -0.1958661417322836718, 0.3392501089628017219, -1.895013123359580165 ) ) ;
#78359=CARTESIAN_POINT ( 'NONE',  ( -0.1049643490035306742, 0.3917322834645668994, -1.188957062170916679 ) ) ;
#78365=CARTESIAN_POINT ( 'NONE',  ( 0.2867679344610366554, -0.2867679344610365999, -2.299888082186038574 ) ) ;
#78374=CARTESIAN_POINT ( 'NONE',  ( -0.3917322834645670104, -7.196005306013484475E-17, -1.698818897637795367 ) ) ;
#78389=CARTESIAN_POINT ( 'NONE',  ( 5.785732909357575061E-17, -0.4724409448818898682, -0.1555118110236220763 ) ) ;
#78392=CARTESIAN_POINT ( 'NONE',  ( 0.3949938075777408852, 0.1058382717557500435, -0.2014435695538058235 ) ) ;
#78397=CARTESIAN_POINT ( 'NONE',  ( -0.1058382717557503072, 0.3949938075777408852, 0.07414698162729657649 ) ) ;
#78405=CARTESIAN_POINT ( 'NONE',  ( 0.3996062992125985480, 2.446882876249141654E-17, -0.8248031496062991907 ) ) ;
#78408=CARTESIAN_POINT ( 'NONE',  ( -0.1049643490035307020, 0.3917322834645669549, -0.4711286089238844177 ) ) ;
#78409=EDGE_CURVE ( 'NONE', #63931, #25317, #69017, .T. ) ;
#78425=CARTESIAN_POINT ( 'NONE',  ( -0.4724409448818899238, 0.1265901696524986686, -2.786745406824146620 ) ) ;
#78432=CARTESIAN_POINT ( 'NONE',  ( -0.1265901696524993347, 0.4724409448818896462, -2.053805774278214979 ) ) ;
#78442=CARTESIAN_POINT ( 'NONE',  ( -0.3460692066303958092, -0.1998031496062994683, -0.6824146981627295938 ) ) ;
#78447=CARTESIAN_POINT ( 'NONE',  ( -9.787531504996567848E-17, 0.3996062992125986035, -2.677165354330708347 ) ) ;
#78448=CARTESIAN_POINT ( 'NONE',  ( -9.674558042662121740E-17, 0.3949938075777409963, -1.732283464566929165 ) ) ;
#78449=CARTESIAN_POINT ( 'NONE',  ( 0.1958661417322836440, -0.3392501089628017219, -0.7139107611548556331 ) ) ;
#78450=CARTESIAN_POINT ( 'NONE',  ( -0.3392501089628019995, 0.1958661417322832277, -0.9632545931758529356 ) ) ;
#78452=CARTESIAN_POINT ( 'NONE',  ( -0.3917322834645670104, -7.196005306013484475E-17, -1.291338582677165503 ) ) ;
#78454=CARTESIAN_POINT ( 'NONE',  ( 0.3917322834645669549, 2.398668435337827645E-17, -0.04066309891632365059 ) ) ;
#78461=CARTESIAN_POINT ( 'NONE',  ( -0.1998031496062991907, -0.3460692066303959757, -2.585301837270341352 ) ) ;
#78462=CARTESIAN_POINT ( 'NONE',  ( -0.3917322834645670104, -0.1049643490035307020, -1.302512754102049142 ) ) ;
#78468=CARTESIAN_POINT ( 'NONE',  ( 0.1049643490035303689, 0.3917322834645670104, -0.3930446194225722945 ) ) ;
#78477=CARTESIAN_POINT ( 'NONE',  ( -0.08989863708912321227, -0.3814249188617225839, -1.929133858267717105 ) ) ;
#78478=CARTESIAN_POINT ( 'NONE',  ( 0.3917322834645670104, -0.1049643490035303411, -1.835958005249343827 ) ) ;
#78479=ORIENTED_EDGE ( 'NONE', *, *, #38792, .T. ) ;
#78480=CARTESIAN_POINT ( 'NONE',  ( -0.1998031496062991907, -0.3460692066303959757, -0.5380577427821522374 ) ) ;
#78487=CARTESIAN_POINT ( 'NONE',  ( -0.2362204724409447953, -0.4091458600556404646, -1.167979002624671914 ) ) ;
#78488=CARTESIAN_POINT ( 'NONE',  ( -0.3917322834645670104, -7.196005306013484475E-17, -0.7539370078740157410 ) ) ;
#78509=CARTESIAN_POINT ( 'NONE',  ( 0.3917322834645669549, 2.398668435337827645E-17, -0.9855449886801030956 ) ) ;
#78512=CARTESIAN_POINT ( 'NONE',  ( -0.2362204724409451284, 0.4091458600556402425, -0.8005249343832020470 ) ) ;
#78518=CARTESIAN_POINT ( 'NONE',  ( 0.2867679344610366554, -0.2867679344610365999, -0.2526439876978496257 ) ) ;
#78521=CARTESIAN_POINT ( 'NONE',  ( -0.1265901696524986964, -0.4724409448818899238, -1.566272965879265344 ) ) ;
#78538=CARTESIAN_POINT ( 'NONE',  ( 0.3460692066303959202, -0.1998031496062991630, -2.858923884514435798 ) ) ;
#78543=CARTESIAN_POINT ( 'NONE',  ( 0.1998031496062992463, 0.3460692066303959202, -1.795931758530183719 ) ) ;
#78549=CARTESIAN_POINT ( 'NONE',  ( -0.1070741851644051862, -0.3996062992125987146, -1.489501312335957950 ) ) ;
#78551=CARTESIAN_POINT ( 'NONE',  ( -0.3949938075777411628, 0.1058382717557497937, -0.8202099737532810853 ) ) ;
#78556=CARTESIAN_POINT ( 'NONE',  ( -0.3949938075777408852, -0.1058382717557502933, -1.540026246719160108 ) ) ;
#78561=CARTESIAN_POINT ( 'NONE',  ( -0.1265901696524993347, 0.4724409448818895907, -1.896325459317584894 ) ) ;
#78562=CARTESIAN_POINT ( 'NONE',  ( 0.3089825338612027239, -0.2417350488526308905, -2.755905511811024944 ) ) ;
#78568=CARTESIAN_POINT ( 'NONE',  ( 0.1958661417322834497, 0.3392501089628018329, -2.429114542485877770 ) ) ;
#78569=CARTESIAN_POINT ( 'NONE',  ( -0.3460692066303957537, -0.1998031496062994405, -2.806430446194225770 ) ) ;
#78574=CARTESIAN_POINT ( 'NONE',  ( 0.3392501089628018329, -0.1958661417322834497, -2.862185408627609728 ) ) ;
#78576=CARTESIAN_POINT ( 'NONE',  ( -0.2867679344610365999, 0.2867679344610364889, -1.901574803149606252 ) ) ;
#78579=CARTESIAN_POINT ( 'NONE',  ( -0.3949938075777409963, -7.255918531996591613E-17, -2.086614173228346303 ) ) ;
#78584=CARTESIAN_POINT ( 'NONE',  ( -0.3996062992125986035, -0.1070741851644056997, -0.5183727034120735322 ) ) ;
#78592=CARTESIAN_POINT ( 'NONE',  ( 0.3392501089628018329, 0.1958661417322835607, -0.2158792650918636147 ) ) ;
#78604=CARTESIAN_POINT ( 'NONE',  ( -0.1265901696524993347, 0.4724409448818895907, -1.266404199475065440 ) ) ;
#78606=CARTESIAN_POINT ( 'NONE',  ( -0.3392501089628017219, -0.1958661417322836718, -0.3595800524934382736 ) ) ;
#78607=CARTESIAN_POINT ( 'NONE',  ( 0.3392501089628018884, -0.1958661417322834220, -2.236876640419947826 ) ) ;
#78610=CARTESIAN_POINT ( 'NONE',  ( 0.3996062992125985480, 2.446882876249141654E-17, -0.1948818897637795700 ) ) ;
#78616=CARTESIAN_POINT ( 'NONE',  ( 0.3420746716998660508, -0.1974969037888704149, -2.858923884514436242 ) ) ;
#78623=CARTESIAN_POINT ( 'NONE',  ( 0.3392501089628018329, 0.1958661417322835607, -2.013123359580052618 ) ) ;
#78626=CARTESIAN_POINT ( 'NONE',  ( -0.4091458600556402980, -0.2362204724409451284, -0.2867454068241469534 ) ) ;
#78635=DIRECTION ( 'NONE',  ( 0.000000000000000000, 0.000000000000000000, 1.000000000000000000 ) ) ;
#78637=CARTESIAN_POINT ( 'NONE',  ( 0.4709442531824356015, 0.03757601356358733491, -1.929133858267717549 ) ) ;
#78640=CARTESIAN_POINT ( 'NONE',  ( 0.1998031496062994128, -0.3460692066303957537, -1.585958005249344049 ) ) ;
#78641=CARTESIAN_POINT ( 'NONE',  ( -0.3392501089628017219, -0.1958661417322836718, -2.499343832020997080 ) ) ;
#78648=CARTESIAN_POINT ( 'NONE',  ( 0.000000000000000000, 0.000000000000000000, -2.755905511811024056 ) ) ;
#78650=CARTESIAN_POINT ( 'NONE',  ( -0.3460692066303958092, -0.1998031496062994683, -0.05249343832020997996 ) ) ;
#78651=CARTESIAN_POINT ( 'NONE',  ( 0.1958661417322834775, 0.3392501089628018884, -2.345819840716222515 ) ) ;
#78652=CARTESIAN_POINT ( 'NONE',  ( -0.3949938075777409408, -0.1058382717557502933, -0.6758530183727035068 ) ) ;
#78657=CARTESIAN_POINT ( 'NONE',  ( -0.1049643490035302024, -0.3917322834645671215, -2.204068241469816503 ) ) ;
#78662=CARTESIAN_POINT ( 'NONE',  ( -0.3460692066303958092, -0.1998031496062994683, -2.099737532808398921 ) ) ;
#78664=CARTESIAN_POINT ( 'NONE',  ( -0.1998031496062991907, -0.3460692066303959757, -1.797900262467191590 ) ) ;
#78667=CARTESIAN_POINT ( 'NONE',  ( -0.1958661417322836995, 0.3392501089628017219, -0.3248224653881383595 ) ) ;
#78679=CARTESIAN_POINT ( 'NONE',  ( 0.1049643490035303689, 0.3917322834645670104, -0.7729658792650916377 ) ) ;
#78682=CARTESIAN_POINT ( 'NONE',  ( -0.3420746716998659953, -0.1974969037888706647, -0.6824146981627297048 ) ) ;
#78697=CARTESIAN_POINT ( 'NONE',  ( 0.3996062992125986035, 2.446882876249141962E-17, -1.220472440944881942 ) ) ;
#78699=CARTESIAN_POINT ( 'NONE',  ( -0.3996062992125984925, -0.1070741851644056858, -0.7526246719160103460 ) ) ;
#78700=CARTESIAN_POINT ( 'NONE',  ( -0.1070741851644056997, 0.3996062992125984925, -0.7132545931758530466 ) ) ;
#78702=CARTESIAN_POINT ( 'NONE',  ( -0.3458507752293906723, -0.3458507752293910609, -0.05905511811023620578 ) ) ;
#78703=CARTESIAN_POINT ( 'NONE',  ( -0.1958661417322834220, -0.3392501089628018884, -2.040026246719160330 ) ) ;
#78709=CARTESIAN_POINT ( 'NONE',  ( 0.3458507752293908943, 0.3458507752293908943, -1.946850393700787274 ) ) ;
#78712=CARTESIAN_POINT ( 'NONE',  ( 0.3420746716998660508, -0.1974969037888704149, -1.441601049868766804 ) ) ;
#78722=CARTESIAN_POINT ( 'NONE',  ( 0.3460692066303958092, 0.1998031496062993018, -2.727690288713910949 ) ) ;
#78723=EDGE_CURVE ( 'NONE', #21899, #40183, #24977, .T. ) ;
#78724=CARTESIAN_POINT ( 'NONE',  ( -0.3392501089628018329, -0.1958661417322836440, -1.864810080543620074 ) ) ;
#78734=CARTESIAN_POINT ( 'NONE',  ( 0.4724409448818880919, 0.1265901696525020825, -2.329396325459317740 ) ) ;
#78739=CARTESIAN_POINT ( 'NONE',  ( -0.3917322834645671215, 0.1049643490035301469, -1.534776902887139194 ) ) ;
#78748=CARTESIAN_POINT ( 'NONE',  ( -9.787531504996566615E-17, 0.3996062992125985480, -0.8641732283464567121 ) ) ;
#78760=CARTESIAN_POINT ( 'NONE',  ( -0.1958661417322836718, 0.3392501089628017219, -2.367454068241469756 ) ) ;
#78764=CARTESIAN_POINT ( 'NONE',  ( -0.1998031496062994683, 0.3460692066303958092, -0.6430446194225721834 ) ) ;
#78767=CARTESIAN_POINT ( 'NONE',  ( -0.3917322834645670104, -7.196005306013484475E-17, -1.606299212598425452 ) ) ;
#78778=CARTESIAN_POINT ( 'NONE',  ( 0.3917322834645669549, 2.398668435337827645E-17, -0.9855449886801030956 ) ) ;
#78784=CARTESIAN_POINT ( 'NONE',  ( 0.3392501089628018884, -0.1958661417322833942, -2.306449761976065105 ) ) ;
#78794=CARTESIAN_POINT ( 'NONE',  ( -0.3392501089628019995, 0.1958661417322832277, -1.843175853018372834 ) ) ;
#78798=CARTESIAN_POINT ( 'NONE',  ( -0.03178304480585582292, 0.3983403474834776858, -2.755905511811024500 ) ) ;
#78802=CARTESIAN_POINT ( 'NONE',  ( 0.3460692066303959202, 0.1998031496062993295, -2.020997375328084100 ) ) ;
#78807=CARTESIAN_POINT ( 'NONE',  ( -0.2362204724409447953, -0.4091458600556404646, -0.7723097112860892732 ) ) ;
#78810=CARTESIAN_POINT ( 'NONE',  ( -0.1058382717557497660, -0.3949938075777411073, -0.1489501312335957950 ) ) ;
#78815=CARTESIAN_POINT ( 'NONE',  ( 0.3949938075777409408, -0.1058382717557499186, -0.6607611548556431291 ) ) ;
#78822=CARTESIAN_POINT ( 'NONE',  ( -0.1070741851644051862, -0.3996062992125986590, -1.251312335958005395 ) ) ;
#78825=CARTESIAN_POINT ( 'NONE',  ( -0.1958661417322836718, 0.3392501089628017219, -0.4776902887139107268 ) ) ;
#78840=CARTESIAN_POINT ( 'NONE',  ( -0.4091458600556405756, 0.2362204724409446288, -2.780183727034120977 ) ) ;
#78858=CARTESIAN_POINT ( 'NONE',  ( -0.3996062992125985480, -0.1070741851644057135, -0.9908136482939633449 ) ) ;
#78862=CARTESIAN_POINT ( 'NONE',  ( 0.1070741851644053527, 0.3996062992125986590, -2.513123359580052174 ) ) ;
#78863=CARTESIAN_POINT ( 'NONE',  ( 4.837279021331060870E-17, -0.3949938075777409963, -1.968503937007873850 ) ) ;
#78864=CARTESIAN_POINT ( 'NONE',  ( -0.1049643490035302024, -0.3917322834645671215, -0.5367454068241469534 ) ) ;
#78867=CARTESIAN_POINT ( 'NONE',  ( -9.594673741351313045E-17, 0.3917322834645670104, -0.9370078740157480324 ) ) ;
#78870=CARTESIAN_POINT ( 'NONE',  ( -9.594673741351310580E-17, 0.3917322834645669549, -0.08003317765648111648 ) ) ;
#78876=CARTESIAN_POINT ( 'NONE',  ( -0.2362204724409451284, 0.4091458600556402425, -0.08989501312335958227 ) ) ;
#78878=CARTESIAN_POINT ( 'NONE',  ( 0.3460692066303959202, 0.1998031496062993295, -2.493438320209973469 ) ) ;
#78879=CARTESIAN_POINT ( 'NONE',  ( -0.1958661417322836995, 0.3392501089628017219, -1.112224040191287955 ) ) ;
#78886=CARTESIAN_POINT ( 'NONE',  ( 4.797336870675656522E-17, -0.3917322834645670104, -0.4783464566929135353 ) ) ;
#78894=CARTESIAN_POINT ( 'NONE',  ( -0.4091458600556405756, 0.2362204724409446288, -0.5754593175853018883 ) ) ;
#78895=CARTESIAN_POINT ( 'NONE',  ( -9.594673741351313045E-17, 0.3917322834645670104, -1.881889763779527769 ) ) ;
#78897=CARTESIAN_POINT ( 'NONE',  ( -0.1998031496062994683, 0.3460692066303958092, -0.3280839895013123453 ) ) ;
#78904=CARTESIAN_POINT ( 'NONE',  ( 0.3917322834645670104, 2.398668435337828261E-17, -1.147637795275590733 ) ) ;
#78914=DIRECTION ( 'NONE',  ( 1.000000000000000000, 0.000000000000000000, 0.000000000000000000 ) ) ;
#78924=CARTESIAN_POINT ( 'NONE',  ( -0.1049643490035306742, 0.3917322834645668994, -1.031476747210287037 ) ) ;
#78933=CARTESIAN_POINT ( 'NONE',  ( -0.3917322834645670104, -0.1049643490035307020, -0.04267023441700976139 ) ) ;
#78941=CARTESIAN_POINT ( 'NONE',  ( -0.2362204724409451284, 0.4091458600556402425, -1.664698162729658426 ) ) ;
#78942=AXIS2_PLACEMENT_3D ( 'NONE', #37482, #81299, #61919 ) ;
#78957=CARTESIAN_POINT ( 'NONE',  ( 0.2925321140481932369, -0.2925321140481931814, -2.694881889763780070 ) ) ;
#78962=CARTESIAN_POINT ( 'NONE',  ( -0.1998031496062994405, 0.3460692066303957537, -1.979658792650918597 ) ) ;
#78967=CARTESIAN_POINT ( 'NONE',  ( -0.2925321140481930149, -0.2925321140481933480, -1.080708661417322691 ) ) ;
#78968=CARTESIAN_POINT ( 'NONE',  ( 0.2925321140481932369, 0.2925321140481932369, -1.555118110236220597 ) ) ;
#78969=CARTESIAN_POINT ( 'NONE',  ( 0.1058382717557500713, -0.3949938075777409408, -0.8727034120734908917 ) ) ;
#78970=CARTESIAN_POINT ( 'NONE',  ( 0.3917322834645670104, -0.1049643490035303273, -0.2611548556430445256 ) ) ;
#78974=CARTESIAN_POINT ( 'NONE',  ( 0.2891555358219910499, -0.2891555358219909944, -1.750000000000000000 ) ) ;
#78978=CARTESIAN_POINT ( 'NONE',  ( -0.2362204724409451284, 0.4091458600556402425, -1.902887139107611647 ) ) ;
#78979=CARTESIAN_POINT ( 'NONE',  ( 0.3796925558546759838, 0.09865214182459616787, -2.755905511811022279 ) ) ;
#78987=CARTESIAN_POINT ( 'NONE',  ( -0.2867679344610366554, 0.2867679344610365444, -2.304442626475378564 ) ) ;
#78994=CARTESIAN_POINT ( 'NONE',  ( 0.1958661417322834775, 0.3392501089628018884, 0.08595800524934374409 ) ) ;
#78996=CARTESIAN_POINT ( 'NONE',  ( 0.3392501089628018884, -0.1958661417322834220, -1.671916010498687655 ) ) ;
#78999=CARTESIAN_POINT ( 'NONE',  ( 0.1974969037888704704, 0.3420746716998660508, -2.349081364829396446 ) ) ;
#79005=CARTESIAN_POINT ( 'NONE',  ( -0.3460692066303958092, -0.1998031496062994683, -0.5249343832020997302 ) ) ;
#79010=CARTESIAN_POINT ( 'NONE',  ( 4.797336870675656522E-17, -0.3917322834645670104, 0.1515748031496061965 ) ) ;
#79012=CARTESIAN_POINT ( 'NONE',  ( -0.3917322834645670104, -7.196005306013484475E-17, -0.7539370078740157410 ) ) ;
#79018=CARTESIAN_POINT ( 'NONE',  ( -0.1958661417322836718, 0.3392501089628017219, 0.1522309711286089495 ) ) ;
#79024=CARTESIAN_POINT ( 'NONE',  ( -0.4724409448818899238, 0.1265901696524986686, -1.292650918635170454 ) ) ;
#79025=LINE ( 'NONE', #80271, #14318 ) ;
#79026=CARTESIAN_POINT ( 'NONE',  ( -0.1958661417322834220, -0.3392501089628018884, -0.3727034120734908362 ) ) ;
#79027=CARTESIAN_POINT ( 'NONE',  ( -0.1958661417322836718, 0.3392501089628017219, -2.302493438320210029 ) ) ;
#79030=CARTESIAN_POINT ( 'NONE',  ( 0.3996062992125986035, -0.1070741851644052972, 0.1266404199475064940 ) ) ;
#79035=CARTESIAN_POINT ( 'NONE',  ( -9.594673741351310580E-17, 0.3917322834645669549, 0.07744713730414881647 ) ) ;
#79037=CARTESIAN_POINT ( 'NONE',  ( -0.3392501089628017219, -0.1958661417322836718, -0.1371391076115486551 ) ) ;
#79042=CARTESIAN_POINT ( 'NONE',  ( -0.3917322834645671215, 0.1049643490035301469, -1.914698162729658648 ) ) ;
#79047=CARTESIAN_POINT ( 'NONE',  ( -0.4724409448818899238, 0.1265901696524986686, -0.4245406824146981672 ) ) ;
#79051=CARTESIAN_POINT ( 'NONE',  ( -0.3458507752293909498, 0.3458507752293908388, -0.7263779527559055538 ) ) ;
#79060=CARTESIAN_POINT ( 'NONE',  ( 0.3460692066303959202, -0.1998031496062991630, -1.441601049868766582 ) ) ;
#79071=CARTESIAN_POINT ( 'NONE',  ( -0.3996062992125986035, -0.1070741851644056997, -0.04593175853018373334 ) ) ;
#79072=CARTESIAN_POINT ( 'NONE',  ( 0.2867679344610366554, 0.2867679344610366554, -2.654218790847456155 ) ) ;
#79077=CARTESIAN_POINT ( 'NONE',  ( -0.2867679344610364334, -0.2867679344610367109, -2.348425196850393970 ) ) ;
#79085=CARTESIAN_POINT ( 'NONE',  ( -0.2867679344610365444, -0.2867679344610367664, -0.3707542239183220789 ) ) ;
#79098=CARTESIAN_POINT ( 'NONE',  ( 4.797336870675656522E-17, -0.3917322834645670104, -0.5433070866141732624 ) ) ;
#79101=CARTESIAN_POINT ( 'NONE',  ( 0.2891555358219910499, -0.2891555358219909944, -1.043307086614173373 ) ) ;
#79118=CARTESIAN_POINT ( 'NONE',  ( 0.3996062992125986590, -0.1070741851644053111, -1.686351706036745446 ) ) ;
#79120=CARTESIAN_POINT ( 'NONE',  ( -9.787531504996566615E-17, 0.3996062992125985480, -1.021653543307086576 ) ) ;
#79121=CARTESIAN_POINT ( 'NONE',  ( -0.3460692066303960313, 0.1998031496062989965, -0.4179790026246719137 ) ) ;
#79123=CARTESIAN_POINT ( 'NONE',  ( 0.2362204724409451007, -0.4091458600556402980, -0.09186351706036745279 ) ) ;
#79124=CARTESIAN_POINT ( 'NONE',  ( 0.1958661417322834775, 0.3392501089628018884, -2.276246719160105236 ) ) ;
#79130=CARTESIAN_POINT ( 'NONE',  ( -1.157146581871515012E-16, 0.4724409448818898682, -1.966535433070865979 ) ) ;
#79133=CARTESIAN_POINT ( 'NONE',  ( 0.2891555358219910499, 0.2891555358219910499, -1.316929133858267598 ) ) ;
#79143=CARTESIAN_POINT ( 'NONE',  ( -0.2925321140481930149, -0.2925321140481933480, -2.655511811023622215 ) ) ;
#79144=CARTESIAN_POINT ( 'NONE',  ( 0.2867679344610365999, -0.2867679344610365999, -2.068222154034434546 ) ) ;
#79156=CARTESIAN_POINT ( 'NONE',  ( -0.3996062992125986590, 0.1070741851644051723, -0.2670603674540683037 ) ) ;
#79158=CARTESIAN_POINT ( 'NONE',  ( -0.2867679344610365999, 0.2867679344610364889, -1.364173228346456268 ) ) ;
#79167=CARTESIAN_POINT ( 'NONE',  ( 0.3460692066303959202, -0.1998031496062991630, -1.126640419947506633 ) ) ;
#79173=B_SPLINE_CURVE_WITH_KNOTS ( 'NONE', 1,
 ( #82986, #25306 ),
 .UNSPECIFIED., .F., .F.,
 ( 2, 2 ),
 ( 0.000000000000000000, 0.001849999999999997480 ),
 .UNSPECIFIED. ) ;
#79184=CARTESIAN_POINT ( 'NONE',  ( 0.3996062992125986035, 0.1070741851644054776, -0.2821522309711286258 ) ) ;
#79187=CARTESIAN_POINT ( 'NONE',  ( 0.1049643490035303689, 0.3917322834645670104, -2.347769028871391050 ) ) ;
#79194=CARTESIAN_POINT ( 'NONE',  ( 0.4091458600556404646, -0.2362204724409448231, -2.071522309711285814 ) ) ;
#79198=CARTESIAN_POINT ( 'NONE',  ( 0.3392501089628018329, -0.1958661417322834497, -1.759823203903200017 ) ) ;
#79204=CARTESIAN_POINT ( 'NONE',  ( 0.1049643490035304799, -0.3917322834645670104, -2.759205667487876656 ) ) ;
#79206=VERTEX_POINT ( 'NONE', #33713 ) ;
#79213=CARTESIAN_POINT ( 'NONE',  ( 0.3917322834645670104, -0.1049643490035303411, -1.770997375328083656 ) ) ;
#79222=CARTESIAN_POINT ( 'NONE',  ( 0.2925321140481932369, -0.2925321140481932369, -1.830708661417322913 ) ) ;
#79227=CARTESIAN_POINT ( 'NONE',  ( -0.4091458600556405756, 0.2362204724409446288, -0.5754593175853018883 ) ) ;
#79231=CARTESIAN_POINT ( 'NONE',  ( -0.3420746716998662729, 0.1974969037888702206, -0.2604986876640420501 ) ) ;
#79236=CARTESIAN_POINT ( 'NONE',  ( 0.1974969037888706092, -0.3420746716998660508, -0.3261154855643044748 ) ) ;
#79243=CARTESIAN_POINT ( 'NONE',  ( -0.3460692066303957537, -0.1998031496062994405, -1.231627296587926690 ) ) ;
#79245=CARTESIAN_POINT ( 'NONE',  ( -0.1958661417322836718, 0.3392501089628017219, -1.265091863517060489 ) ) ;
#79258=CARTESIAN_POINT ( 'NONE',  ( 0.3458507752293908943, -0.3458507752293908943, -2.852362204724409711 ) ) ;
#79275=CARTESIAN_POINT ( 'NONE',  ( 0.2925321140481932369, 0.2925321140481932369, -0.7677165354330708347 ) ) ;
#79276=CARTESIAN_POINT ( 'NONE',  ( -0.4724409448818898682, 5.785732909357575061E-17, -2.755905511811024056 ) ) ;
#79279=CARTESIAN_POINT ( 'NONE',  ( -0.3460692066303958092, -0.1998031496062994683, -2.729658792650918375 ) ) ;
#79280=CARTESIAN_POINT ( 'NONE',  ( -0.1058382717557503211, 0.3949938075777409408, -2.211286089238845065 ) ) ;
#79282=CARTESIAN_POINT ( 'NONE',  ( 0.2867679344610365999, 0.2867679344610365999, -1.074803149606299080 ) ) ;
#79285=CARTESIAN_POINT ( 'NONE',  ( 0.3917322834645669549, 0.1049643490035304660, -1.219160104986876325 ) ) ;
#79287=CARTESIAN_POINT ( 'NONE',  ( -0.2867679344610366554, 0.2867679344610365444, 0.05776209793407005577 ) ) ;
#79294=CARTESIAN_POINT ( 'NONE',  ( -0.3392501089628019995, 0.1958661417322831999, -1.125347399771340573 ) ) ;
#79300=CARTESIAN_POINT ( 'NONE',  ( 0.3392501089628018329, 0.1958661417322835607, -0.5308398950131234528 ) ) ;
#79308=CARTESIAN_POINT ( 'NONE',  ( -1.157146581871515012E-16, 0.4724409448818898682, -0.5492125984251968740 ) ) ;
#79309=CARTESIAN_POINT ( 'NONE',  ( -0.1049643490035302024, -0.3917322834645671215, -2.269028871391075786 ) ) ;
#79311=CARTESIAN_POINT ( 'NONE',  ( -0.3460692066303960868, 0.1998031496062990242, -0.4986876640419947715 ) ) ;
#79318=CARTESIAN_POINT ( 'NONE',  ( 0.2867679344610365999, -0.2867679344610365444, -1.442913385826771755 ) ) ;
#79337=CARTESIAN_POINT ( 'NONE',  ( -0.1958661417322834497, -0.3392501089628018884, -1.248012180281152794 ) ) ;
#79346=CARTESIAN_POINT ( 'NONE',  ( -0.3917322834645670659, -7.196005306013484475E-17, 0.1213717603336463974 ) ) ;
#79349=EDGE_CURVE ( 'NONE', #37370, #51716, #66391, .T. ) ;
#79350=CARTESIAN_POINT ( 'NONE',  ( -0.1265901696524986964, -0.4724409448818899238, -0.2296587926509186250 ) ) ;
#79351=CARTESIAN_POINT ( 'NONE',  ( 0.2362204724409451007, -0.4091458600556402980, -1.585958005249344049 ) ) ;
#79366=CARTESIAN_POINT ( 'NONE',  ( -0.2925321140481932369, 0.2925321140481931259, -2.773622047244094002 ) ) ;
#79371=CARTESIAN_POINT ( 'NONE',  ( -0.3996062992125985480, -7.340648628747423112E-17, -1.848425196850393748 ) ) ;
#79376=CARTESIAN_POINT ( 'NONE',  ( -0.3460692066303960313, 0.1998031496062989965, -0.8904199475065617264 ) ) ;
#79377=CARTESIAN_POINT ( 'NONE',  ( 0.1070741851644054915, -0.3996062992125986035, -1.187664041994750619 ) ) ;
#79378=CARTESIAN_POINT ( 'NONE',  ( -0.3949938075777411628, 0.1058382717557497937, -1.135170603674540812 ) ) ;
#79379=CARTESIAN_POINT ( 'NONE',  ( -0.2925321140481932924, 0.2925321140481931814, -2.539370078740157410 ) ) ;
#79380=CARTESIAN_POINT ( 'NONE',  ( 0.3917322834645669549, 0.1049643490035304660, -0.2742782152230970327 ) ) ;
#79384=CARTESIAN_POINT ( 'NONE',  ( 0.3949938075777409408, -0.1058382717557499186, -1.605643044619423199 ) ) ;
#79388=CARTESIAN_POINT ( 'NONE',  ( -0.4091458600556405756, 0.2362204724409446288, -2.230971128608923770 ) ) ;
#79396=CARTESIAN_POINT ( 'NONE',  ( 0.2867679344610365999, 0.2867679344610365999, -2.265072547735221153 ) ) ;
#79404=CARTESIAN_POINT ( 'NONE',  ( -0.1958661417322836440, 0.3392501089628016664, -2.770321891567242734 ) ) ;
#79406=CARTESIAN_POINT ( 'NONE',  ( 0.2867679344610365999, 0.2867679344610365999, -1.862204724409449064 ) ) ;
#79409=CARTESIAN_POINT ( 'NONE',  ( -0.1058382717557503211, 0.3949938075777409408, -2.368766404199475595 ) ) ;
#79414=CARTESIAN_POINT ( 'NONE',  ( 0.1998031496062994405, -0.3460692066303958092, -0.7217847769028871152 ) ) ;
#79417=CARTESIAN_POINT ( 'NONE',  ( 0.1011035889004530536, -0.3790285851608820034, -2.755905511811024944 ) ) ;
#79418=CARTESIAN_POINT ( 'NONE',  ( 0.3917322834645670104, 2.398668435337828261E-17, -0.04527559055118119541 ) ) ;
#79424=CARTESIAN_POINT ( 'NONE',  ( -0.3392501089628019995, 0.1958661417322832277, -0.01837270341207344546 ) ) ;
#79430=CARTESIAN_POINT ( 'NONE',  ( 0.4724409448818898682, 2.892866454678787531E-17, -1.377952755905511806 ) ) ;
#79433=CARTESIAN_POINT ( 'NONE',  ( 0.1049643490035303689, 0.3917322834645670104, -0.6154855643044617741 ) ) ;
#79434=CARTESIAN_POINT ( 'NONE',  ( -9.594673741351313045E-17, 0.3917322834645670104, -2.446850393700787496 ) ) ;
#79437=CARTESIAN_POINT ( 'NONE',  ( -0.1998031496062994405, 0.3460692066303957537, -0.08989501312335959615 ) ) ;
#79442=CARTESIAN_POINT ( 'NONE',  ( 0.1958661417322834497, 0.3392501089628018329, -0.06690981807642862322 ) ) ;
#79444=CARTESIAN_POINT ( 'NONE',  ( -0.1958661417322834220, -0.3392501089628018884, -0.1502624671916011345 ) ) ;
#79449=CARTESIAN_POINT ( 'NONE',  ( -0.1049643490035302024, -0.3917322834645671215, -2.111548556430446144 ) ) ;
#79454=CARTESIAN_POINT ( 'NONE',  ( 0.4724409448818896462, 0.1265901696524990294, -0.5164041994750655507 ) ) ;
#79463=CYLINDRICAL_SURFACE ( 'NONE', #34468, 0.4724409448818898682 ) ;
#79465=CARTESIAN_POINT ( 'NONE',  ( 0.4724409448818898682, 0.000000000000000000, 0.000000000000000000 ) ) ;
#79468=CARTESIAN_POINT ( 'NONE',  ( 0.1070741851644054776, -0.3996062992125984925, -1.579396325459317296 ) ) ;
#79477=CARTESIAN_POINT ( 'NONE',  ( 0.1070741851644053527, 0.3996062992125986590, -0.1509186351706036655 ) ) ;
#79478=CARTESIAN_POINT ( 'NONE',  ( -0.2867679344610365444, -0.2867679344610367664, -2.417998318406511249 ) ) ;
#79485=CARTESIAN_POINT ( 'NONE',  ( 0.2867679344610365999, 0.2867679344610365999, -2.584645669291338876 ) ) ;
#79490=CARTESIAN_POINT ( 'NONE',  ( 0.4724409448818897572, -0.1265901696524988906, -0.8989501312335956840 ) ) ;
#79491=CARTESIAN_POINT ( 'NONE',  ( -0.3996062992125986590, 0.1070741851644051862, -2.080052493438320216 ) ) ;
#79494=CARTESIAN_POINT ( 'NONE',  ( -0.1049643490035307158, 0.3917322834645670104, -0.1607804706374822146 ) ) ;
#79508=CARTESIAN_POINT ( 'NONE',  ( 0.3917322834645670104, -0.1049643490035303411, -0.4186351706036745557 ) ) ;
#79511=CARTESIAN_POINT ( 'NONE',  ( -0.1974969037888703871, -0.3420746716998661063, -1.167979002624671914 ) ) ;
#79522=CARTESIAN_POINT ( 'NONE',  ( 0.3458507752293908943, -0.3458507752293908943, -1.043307086614173151 ) ) ;
#79529=CARTESIAN_POINT ( 'NONE',  ( 0.3996062992125986590, -0.1070741851644053111, -1.528871391076114916 ) ) ;
#79532=CARTESIAN_POINT ( 'NONE',  ( -0.3460692066303957537, -0.1998031496062994405, -1.074146981627296604 ) ) ;
#79533=CARTESIAN_POINT ( 'NONE',  ( 0.3460692066303958092, 0.1998031496062993018, -0.5229658792650918597 ) ) ;
#79535=CARTESIAN_POINT ( 'NONE',  ( 5.785732909357575061E-17, -0.4724409448818898682, 0.07874015748031495954 ) ) ;
#79537=CARTESIAN_POINT ( 'NONE',  ( 0.3392501089628018329, 0.1958661417322835607, -2.420603674540682260 ) ) ;
#79543=CARTESIAN_POINT ( 'NONE',  ( 0.2362204724409449064, 0.4091458600556404646, -1.953412073490813805 ) ) ;
#79546=CARTESIAN_POINT ( 'NONE',  ( 0.3949938075777409963, 2.418639510665530743E-17, -1.769685039370078927 ) ) ;
#79556=CARTESIAN_POINT ( 'NONE',  ( -9.787531504996566615E-17, 0.3996062992125985480, -2.596456692913385655 ) ) ;
#79557=CARTESIAN_POINT ( 'NONE',  ( 0.1049643490035304522, -0.3917322834645668994, -2.370059424375641211 ) ) ;
#79569=CARTESIAN_POINT ( 'NONE',  ( -0.1998031496062994405, 0.3460692066303957537, -0.4048556430446194621 ) ) ;
#79571=CARTESIAN_POINT ( 'NONE',  ( -0.3917322834645669549, -0.1049643490035306603, -2.020341207349081181 ) ) ;
#79581=CARTESIAN_POINT ( 'NONE',  ( -0.3996062992125984925, -0.1070741851644056858, -0.9101049868766404316 ) ) ;
#79594=CARTESIAN_POINT ( 'NONE',  ( -0.1958661417322834220, -0.3392501089628018884, -2.734908136482939511 ) ) ;
#79598=CARTESIAN_POINT ( 'NONE',  ( 0.2925321140481932369, 0.2925321140481932369, -0.4527559055118109965 ) ) ;
#79601=CARTESIAN_POINT ( 'NONE',  ( 0.1049643490035304938, -0.3917322834645669549, -2.124671916010498762 ) ) ;
#79608=CARTESIAN_POINT ( 'NONE',  ( 0.000000000000000000, 0.000000000000000000, -2.755905511811024056 ) ) ;
#79612=CARTESIAN_POINT ( 'NONE',  ( 0.3917322834645669549, 2.398668435337827645E-17, -1.457985933561992686 ) ) ;
#79614=ADVANCED_BREP_SHAPE_REPRESENTATION ( '', ( #31714, #22098 ), #649 ) ;
#79619=CARTESIAN_POINT ( 'NONE',  ( -0.3917322834645670104, -0.1049643490035307020, -2.719835588747718802 ) ) ;
#79628=CARTESIAN_POINT ( 'NONE',  ( 0.2867679344610365999, -0.2867679344610365444, -2.072834645669291209 ) ) ;
#79635=FACE_OUTER_BOUND ( 'NONE', #16162, .T. ) ;
#79637=CARTESIAN_POINT ( 'NONE',  ( -0.2925321140481932924, 0.2925321140481931814, -2.066929133858267154 ) ) ;
#79643=CARTESIAN_POINT ( 'NONE',  ( -1.157146581871515012E-16, 0.4724409448818898682, -0.8641732283464567121 ) ) ;
#79646=CARTESIAN_POINT ( 'NONE',  ( 0.3949938075777408852, 0.1058382717557500435, -0.3589238845144356871 ) ) ;
#79651=CARTESIAN_POINT ( 'NONE',  ( 0.3949938075777409963, 2.418639510665530743E-17, -0.5098425196850394636 ) ) ;
#79659=CARTESIAN_POINT ( 'NONE',  ( -9.787531504996566615E-17, 0.3996062992125985480, -1.336614173228346525 ) ) ;
#79661=CARTESIAN_POINT ( 'NONE',  ( 4.797336870675656522E-17, -0.3917322834645670104, -1.015748031496062964 ) ) ;
#79663=CARTESIAN_POINT ( 'NONE',  ( -0.3496712940256294089, -0.1778467755331540612, -5.947530023412595687E-17 ) ) ;
#79671=( BOUNDED_CURVE ( )  B_SPLINE_CURVE ( 1, ( #72266, #39853 ),
 .UNSPECIFIED., .F., .F. ) 
 B_SPLINE_CURVE_WITH_KNOTS ( ( 2, 2 ),
 ( 0.000000000000000000, 0.001849999999999997480 ),
 .UNSPECIFIED. ) 
 CURVE ( )  GEOMETRIC_REPRESENTATION_ITEM ( )  RATIONAL_B_SPLINE_CURVE ( ( 0.9911642120908024101, 0.9911642120908024101 ) ) 
 REPRESENTATION_ITEM ( '' )  );
#79672=CARTESIAN_POINT ( 'NONE',  ( -0.4091458600556405756, 0.2362204724409446288, -0.2604986876640419946 ) ) ;
#79681=CARTESIAN_POINT ( 'NONE',  ( 0.4724409448818897017, 0.1265901696524990294, -2.014435695538057125 ) ) ;
#79691=CARTESIAN_POINT ( 'NONE',  ( 0.3996062992125985480, 0.1070741851644054637, -0.7545931758530182165 ) ) ;
#79692=LINE ( 'NONE', #79276, #65072 ) ;
#79695=CARTESIAN_POINT ( 'NONE',  ( 0.4724409448818897572, -0.1265901696524988906, 0.04593175853018372640 ) ) ;
#79696=CARTESIAN_POINT ( 'NONE',  ( -0.3420746716998659953, -0.1974969037888706647, -2.257217847769029007 ) ) ;
#79700=CARTESIAN_POINT ( 'NONE',  ( 0.3392501089628018884, -0.1958661417322834220, -1.041994750656167756 ) ) ;
#79706=CARTESIAN_POINT ( 'NONE',  ( 0.3917322834645668994, -0.1049643490035303134, -0.5065423640081871959 ) ) ;
#79713=CARTESIAN_POINT ( 'NONE',  ( 0.1049643490035304799, -0.3917322834645670104, -1.814323777724096809 ) ) ;
#79719=CARTESIAN_POINT ( 'NONE',  ( 0.2867679344610365999, -0.2867679344610365444, -0.9704724409448820532 ) ) ;
#79728=CARTESIAN_POINT ( 'NONE',  ( 4.797336870675656522E-17, -0.3917322834645670104, -2.433070866141732402 ) ) ;
#79735=DIRECTION ( 'NONE',  ( 0.000000000000000000, 0.000000000000000000, 1.000000000000000000 ) ) ;
#79736=CARTESIAN_POINT ( 'NONE',  ( -0.3917322834645669549, -0.1049643490035306603, -1.232939632545931863 ) ) ;
#79737=CARTESIAN_POINT ( 'NONE',  ( -0.2925321140481930149, -0.2925321140481933480, -2.183070866141731958 ) ) ;
#79747=CARTESIAN_POINT ( 'NONE',  ( -0.3996062992125984925, -0.1070741851644056719, -2.012467191601049699 ) ) ;
#79756=CARTESIAN_POINT ( 'NONE',  ( -9.594673741351310580E-17, 0.3917322834645669549, -1.182395382380890592 ) ) ;
#79766=CARTESIAN_POINT ( 'NONE',  ( 0.3917322834645670659, -0.1049643490035303273, -0.5807279771991620265 ) ) ;
#79769=CARTESIAN_POINT ( 'NONE',  ( -0.3458507752293906723, -0.3458507752293910609, -0.2165354330708661734 ) ) ;
#79770=CARTESIAN_POINT ( 'NONE',  ( 0.1265901696524990294, -0.4724409448818896462, -1.579396325459317296 ) ) ;
#79781=DIRECTION ( 'NONE',  ( 0.000000000000000000, 0.000000000000000000, 1.000000000000000000 ) ) ;
#79784=DIRECTION ( 'NONE',  ( 1.000000000000000000, 0.000000000000000000, 0.000000000000000000 ) ) ;
#79788=CARTESIAN_POINT ( 'NONE',  ( -0.2925321140481930149, -0.2925321140481933480, -2.812992125984251857 ) ) ;
#79793=CARTESIAN_POINT ( 'NONE',  ( -9.787531504996566615E-17, 0.3996062992125985480, -2.281496062992125928 ) ) ;
#79799=CARTESIAN_POINT ( 'NONE',  ( 0.2925321140481932369, -0.2925321140481932369, -1.988188976377952777 ) ) ;
#79800=CARTESIAN_POINT ( 'NONE',  ( 0.2891555358219910499, 0.2891555358219910499, -0.9251968503937008093 ) ) ;
#79801=CARTESIAN_POINT ( 'NONE',  ( -0.1998031496062991907, -0.3460692066303959757, -2.585301837270341352 ) ) ;
#79802=CARTESIAN_POINT ( 'NONE',  ( 0.3458507752293908943, 0.3458507752293908943, -0.6102362204724408601 ) ) ;
#79803=CARTESIAN_POINT ( 'NONE',  ( -0.3392501089628017219, -0.1958661417322836718, -0.3595800524934382736 ) ) ;
#79807=CARTESIAN_POINT ( 'NONE',  ( 4.837279021331061486E-17, -0.3949938075777409963, -2.045275590551181022 ) ) ;
#79811=CARTESIAN_POINT ( 'NONE',  ( -0.3458507752293906723, -0.3458507752293910609, -2.106299212598425452 ) ) ;
#79812=DIRECTION ( 'NONE',  ( -0.000000000000000000, -1.000000000000000000, -0.000000000000000000 ) ) ;
#79820=CARTESIAN_POINT ( 'NONE',  ( 0.3392501089628018329, -0.1958661417322834497, -2.232264148785090274 ) ) ;
#79827=CARTESIAN_POINT ( 'NONE',  ( -0.2867679344610364334, -0.2867679344610367109, 0.01377952755905502598 ) ) ;
#79829=CARTESIAN_POINT ( 'NONE',  ( 0.2867679344610365999, -0.2867679344610365444, -1.980314960629921073 ) ) ;
#79832=CARTESIAN_POINT ( 'NONE',  ( -0.3949938075777409408, -0.1058382717557502933, -2.250656167979002920 ) ) ;
#79836=CARTESIAN_POINT ( 'NONE',  ( 0.1070741851644054915, -0.3996062992125986035, -0.8727034120734907807 ) ) ;
#79841=CARTESIAN_POINT ( 'NONE',  ( 0.3917322834645669549, 0.1049643490035304660, 0.1056430446194224632 ) ) ;
#79852=CARTESIAN_POINT ( 'NONE',  ( 0.1265901696524989462, 0.4724409448818897572, -1.095800524934382958 ) ) ;
#79853=CARTESIAN_POINT ( 'NONE',  ( 0.2952755905511810774, 0.000000000000000000, -1.929133858267716661 ) ) ;
#79855=CARTESIAN_POINT ( 'NONE',  ( 0.1958661417322834775, 0.3392501089628018884, -0.6089238845144356871 ) ) ;
#79856=CARTESIAN_POINT ( 'NONE',  ( -0.3917322834645670104, -7.196005306013484475E-17, -2.486220472440944906 ) ) ;
#79859=CARTESIAN_POINT ( 'NONE',  ( -0.2925321140481932369, 0.2925321140481931259, -0.09645669291338584972 ) ) ;
#79864=CARTESIAN_POINT ( 'NONE',  ( -0.1049643490035301746, -0.3917322834645670659, -0.1522116553467698086 ) ) ;
#79866=CARTESIAN_POINT ( 'NONE',  ( -0.2867679344610366554, 0.2867679344610365444, -0.4192913385826772532 ) ) ;
#79872=CARTESIAN_POINT ( 'NONE',  ( -0.2867679344610364334, -0.2867679344610367109, -1.783464566929133577 ) ) ;
#79875=CARTESIAN_POINT ( 'NONE',  ( -0.1265901696524993347, 0.4724409448818895907, -0.5557742782152230721 ) ) ;
#79886=CARTESIAN_POINT ( 'NONE',  ( -0.3460692066303960313, 0.1998031496062989965, -1.520341207349081181 ) ) ;
#79894=CARTESIAN_POINT ( 'NONE',  ( -0.1070741851644051862, -0.3996062992125986035, -0.3064304461942256586 ) ) ;
#79895=CARTESIAN_POINT ( 'NONE',  ( -0.2925321140481932924, 0.2925321140481931814, -0.1771653543307086520 ) ) ;
#79896=CARTESIAN_POINT ( 'NONE',  ( -9.674558042662121740E-17, 0.3949938075777409963, 0.1574803149606298636 ) ) ;
#79900=DIRECTION ( 'NONE',  ( -1.000000000000000000, 0.000000000000000000, 0.000000000000000000 ) ) ;
#79903=CARTESIAN_POINT ( 'NONE',  ( 0.3917322834645670104, -0.1049643490035303411, -2.243438320209974357 ) ) ;
#79909=CARTESIAN_POINT ( 'NONE',  ( 5.785732909357575061E-17, -0.4724409448818898682, -0.8661417322834645827 ) ) ;
#79910=CARTESIAN_POINT ( 'NONE',  ( -0.1998031496062994683, 0.3460692066303958092, -2.060367454068241511 ) ) ;
#79913=CARTESIAN_POINT ( 'NONE',  ( 0.3392501089628018884, -0.1958661417322833942, -0.4166859824485057984 ) ) ;
#79928=CARTESIAN_POINT ( 'NONE',  ( 0.2867679344610365999, 0.2867679344610365999, -0.4448818897637794589 ) ) ;
#79931=CARTESIAN_POINT ( 'NONE',  ( -0.3949938075777409408, -0.1058382717557502933, -0.8333333333333334814 ) ) ;
#79942=CARTESIAN_POINT ( 'NONE',  ( 0.3458507752293908943, 0.3458507752293908943, -0.3720472440944882497 ) ) ;
#79949=CARTESIAN_POINT ( 'NONE',  ( -0.1070741851644051862, -0.3996062992125987146, -1.804461942257217677 ) ) ;
#79952=CARTESIAN_POINT ( 'NONE',  ( -0.1998031496062994405, 0.3460692066303957537, -1.349737532808398921 ) ) ;
#79953=CARTESIAN_POINT ( 'NONE',  ( -0.3460692066303960313, 0.1998031496062989965, -0.5754593175853018883 ) ) ;
#79956=CARTESIAN_POINT ( 'NONE',  ( -0.1265901696524993347, 0.4724409448818895907, -0.1640419947506561726 ) ) ;
#79957=CARTESIAN_POINT ( 'NONE',  ( -0.1958661417322836718, 0.3392501089628017219, -2.459973753280839670 ) ) ;
#79963=CARTESIAN_POINT ( 'NONE',  ( 5.785732909357575061E-17, -0.4724409448818898682, -1.730314960629921517 ) ) ;
#79966=CARTESIAN_POINT ( 'NONE',  ( 0.2891555358219910499, 0.2891555358219910499, -1.631889763779527991 ) ) ;
#79975=CARTESIAN_POINT ( 'NONE',  ( 4.893765752498283308E-17, -0.3996062992125985480, -2.675196850393700920 ) ) ;
#79976=CARTESIAN_POINT ( 'NONE',  ( -0.1049643490035306742, 0.3917322834645668994, -2.291319266895325946 ) ) ;
#79990=CARTESIAN_POINT ( 'NONE',  ( 0.3996062992125985480, 2.446882876249141654E-17, -0.3523622047244094335 ) ) ;
#79992=CARTESIAN_POINT ( 'NONE',  ( -9.594673741351313045E-17, 0.3917322834645670104, -1.974409448818897683 ) ) ;
#80002=CARTESIAN_POINT ( 'NONE',  ( -0.1998031496062994405, 0.3460692066303957537, -1.034776902887139194 ) ) ;
#80012=CARTESIAN_POINT ( 'NONE',  ( -0.3917322834645670104, -7.196005306013484475E-17, -2.708661417322834275 ) ) ;
#80014=CARTESIAN_POINT ( 'NONE',  ( -0.3996062992125987146, 0.1070741851644051862, -0.3477690288713909950 ) ) ;
#80017=CARTESIAN_POINT ( 'NONE',  ( -0.1049643490035307020, 0.3917322834645669549, -2.360892388451444113 ) ) ;
#80027=CARTESIAN_POINT ( 'NONE',  ( 0.3392501089628018329, 0.1958661417322835052, -1.628589608102675390 ) ) ;
#80033=CARTESIAN_POINT ( 'NONE',  ( 0.3392501089628018884, -0.1958661417322833942, -2.778890706857954473 ) ) ;
#80042=CARTESIAN_POINT ( 'NONE',  ( 0.2867679344610366554, -0.2867679344610365999, -1.355006192422259170 ) ) ;
#80044=CARTESIAN_POINT ( 'NONE',  ( 0.2867679344610365999, -0.2867679344610365444, -2.387795275590551380 ) ) ;
#80051=CARTESIAN_POINT ( 'NONE',  ( -0.1070741851644056997, 0.3996062992125984925, 0.2316272965879264956 ) ) ;
#80053=CARTESIAN_POINT ( 'NONE',  ( -0.3460692066303958092, -0.1998031496062994683, -1.942257217847769057 ) ) ;
#80059=CARTESIAN_POINT ( 'NONE',  ( -0.4724409448818895907, -0.1265901696524993070, -0.7526246719160103460 ) ) ;
#80063=CARTESIAN_POINT ( 'NONE',  ( -0.3420746716998662729, 0.1974969037888702206, -0.5754593175853018883 ) ) ;
#80069=CARTESIAN_POINT ( 'NONE',  ( -0.2891555358219909388, -0.2891555358219912164, -0.4507874015748032925 ) ) ;
#80076=CARTESIAN_POINT ( 'NONE',  ( 0.1070741851644053388, 0.3996062992125986035, -1.172572178477690352 ) ) ;
#80078=CARTESIAN_POINT ( 'NONE',  ( 4.797336870675656522E-17, -0.3917322834645670104, -1.173228346456692828 ) ) ;
#80080=CARTESIAN_POINT ( 'NONE',  ( -0.2263583204867699317, -0.3204081651523066343, -2.110585413283051508E-17 ) ) ;
#80106=CARTESIAN_POINT ( 'NONE',  ( 0.3460692066303959202, 0.1998031496062993295, -0.6036745406824146620 ) ) ;
#80111=CARTESIAN_POINT ( 'NONE',  ( -0.2362204724409451284, 0.4091458600556402425, -0.01312335958005249326 ) ) ;
#80112=CARTESIAN_POINT ( 'NONE',  ( -0.3949938075777409408, -0.1058382717557502933, -2.250656167979002920 ) ) ;
#80115=CARTESIAN_POINT ( 'NONE',  ( 0.1049643490035303689, 0.3917322834645670104, -0.7729658792650916377 ) ) ;
#80122=CARTESIAN_POINT ( 'NONE',  ( 0.3917322834645668994, 0.1049643490035304522, -0.2047050936669798094 ) ) ;
#80127=PLANE ( 'NONE',  #50214 ) ;
#80129=CARTESIAN_POINT ( 'NONE',  ( -0.2867679344610365444, -0.2867679344610367664, -1.473116428642731401 ) ) ;
#80135=CARTESIAN_POINT ( 'NONE',  ( 4.797336870675656522E-17, -0.3917322834645670104, -0.7933070866141732624 ) ) ;
#80144=CARTESIAN_POINT ( 'NONE',  ( 0.3917322834645670104, -0.1049643490035303411, -2.150918635170603554 ) ) ;
#80155=CARTESIAN_POINT ( 'NONE',  ( 0.3392501089628018884, -0.1958661417322834220, -1.291994750656167978 ) ) ;
#80157=CARTESIAN_POINT ( 'NONE',  ( 0.1070741851644053388, 0.3996062992125986035, -2.432414698162729039 ) ) ;
#80168=( BOUNDED_CURVE ( )  B_SPLINE_CURVE ( 2, ( #42166, #73346, #3464, #67861, #60290, #3878, #16102, #16521, #80500, #2640, #79672, #15693, #10198 ),
 .UNSPECIFIED., .F., .F. ) 
 B_SPLINE_CURVE_WITH_KNOTS ( ( 3, 2, 2, 2, 2, 2, 3 ),
 ( 0.1375000000000000111, 0.1416666666666666630, 0.1458333333333333426, 0.1499999999999999944, 0.1541666666666666741, 0.1583333333333333259, 0.1625000000000000056 ),
 .UNSPECIFIED. ) 
 CURVE ( )  GEOMETRIC_REPRESENTATION_ITEM ( )  RATIONAL_B_SPLINE_CURVE ( ( 1.000000000000000000, 0.9659258262890683122, 1.000000000000000000, 0.9659258262890683122, 1.000000000000000000, 0.9659258262890683122, 1.000000000000000000, 0.9659258262890683122, 1.000000000000000000, 0.9659258262890683122, 1.000000000000000000, 0.9659258262890683122, 1.000000000000000000 ) ) 
 REPRESENTATION_ITEM ( '' )  );
#80177=CARTESIAN_POINT ( 'NONE',  ( -0.2867679344610366554, 0.2867679344610365444, -1.359560736711598938 ) ) ;
#80186=CARTESIAN_POINT ( 'NONE',  ( 0.1958661417322836718, -0.3392501089628017219, -0.5610429378290832103 ) ) ;
#80188=CARTESIAN_POINT ( 'NONE',  ( -0.4724409448818898682, -8.678599364036362592E-17, -0.1968503937007874127 ) ) ;
#80189=CARTESIAN_POINT ( 'NONE',  ( -0.1265901696524993347, 0.4724409448818895907, -1.500656167979002031 ) ) ;
#80209=CARTESIAN_POINT ( 'NONE',  ( 0.3460692066303958092, 0.1998031496062993018, -2.412729658792650778 ) ) ;
#80215=CARTESIAN_POINT ( 'NONE',  ( 0.1998031496062992740, 0.3460692066303959757, -1.719160104986876769 ) ) ;
#80216=CARTESIAN_POINT ( 'NONE',  ( -0.1058382717557503211, 0.3949938075777409408, -1.266404199475065440 ) ) ;
#80217=CARTESIAN_POINT ( 'NONE',  ( -0.1070741851644051862, -0.3996062992125987146, -2.591863517060367439 ) ) ;
#80219=CARTESIAN_POINT ( 'NONE',  ( 0.1958661417322834775, 0.3392501089628018884, -0.2939632545931757934 ) ) ;
#80223=CARTESIAN_POINT ( 'NONE',  ( -0.3420746716998662729, 0.1974969037888702206, -1.992782152230971882 ) ) ;
#80227=CARTESIAN_POINT ( 'NONE',  ( 0.3458507752293908943, 0.3458507752293908943, -2.342519685039369914 ) ) ;
#80228=CARTESIAN_POINT ( 'NONE',  ( -0.2925321140481932924, 0.2925321140481931814, -1.594488188976378229 ) ) ;
#80237=CARTESIAN_POINT ( 'NONE',  ( -0.2867679344610364334, -0.2867679344610368219, -2.816253650097426231 ) ) ;
#80244=CARTESIAN_POINT ( 'NONE',  ( 0.2867679344610365999, -0.2867679344610365444, -0.02559055118110245899 ) ) ;
#80247=CARTESIAN_POINT ( 'NONE',  ( 0.1958661417322834775, 0.3392501089628018884, -2.183727034120734878 ) ) ;
#80250=CARTESIAN_POINT ( 'NONE',  ( 0.3949938075777409963, 2.418639510665530435E-17, -2.322834645669291209 ) ) ;
#80254=CARTESIAN_POINT ( 'NONE',  ( -0.3996062992125986035, -0.1070741851644056997, -0.9908136482939633449 ) ) ;
#80257=CARTESIAN_POINT ( 'NONE',  ( -0.4724409448818898682, 5.785732909357575061E-17, -2.755905511811024056 ) ) ;
#80259=CARTESIAN_POINT ( 'NONE',  ( 0.1049643490035303689, 0.3917322834645670104, 0.07939632545931750440 ) ) ;
#80266=VERTEX_POINT ( 'NONE', #61696 ) ;
#80269=AXIS2_PLACEMENT_3D ( 'NONE', #78648, #60512, #46211 ) ;
#80270=CARTESIAN_POINT ( 'NONE',  ( -0.1265901696524993347, 0.4724409448818895907, -1.896325459317584894 ) ) ;
#80271=CARTESIAN_POINT ( 'NONE',  ( -0.2017716535433071445, -0.2017716535433071445, -0.3937007874015748254 ) ) ;
#80272=CARTESIAN_POINT ( 'NONE',  ( 0.1958661417322836440, -0.3392501089628017219, -0.8713910761154854967 ) ) ;
#80277=VECTOR ( 'NONE', #59923, 39.37007874015748143 ) ;
#80279=CARTESIAN_POINT ( 'NONE',  ( -0.4091458600556402980, -0.2362204724409451284, -1.942257217847769057 ) ) ;
#80282=CARTESIAN_POINT ( 'NONE',  ( 0.1049643490035304522, -0.3917322834645668994, 0.1496256149944375224 ) ) ;
#80284=CARTESIAN_POINT ( 'NONE',  ( 0.1958661417322834775, 0.3392501089628018884, -0.5439632545931759600 ) ) ;
#80289=CARTESIAN_POINT ( 'NONE',  ( -0.1049643490035307020, 0.3917322834645669549, -2.203412073490814027 ) ) ;
#80292=CARTESIAN_POINT ( 'NONE',  ( 0.4724409448818896462, 0.1265901696524990294, -0.2014435695538057958 ) ) ;
#80300=CARTESIAN_POINT ( 'NONE',  ( -0.1265901696524993347, 0.4724409448818896462, -1.973097112860892510 ) ) ;
#80302=CARTESIAN_POINT ( 'NONE',  ( 0.3996062992125985480, 2.446882876249141654E-17, -1.769685039370078927 ) ) ;
#80311=CARTESIAN_POINT ( 'NONE',  ( 0.1998031496062994128, -0.3460692066303957537, -0.3261154855643044748 ) ) ;
#80312=CARTESIAN_POINT ( 'NONE',  ( -0.3996062992125986035, -7.340648628747425578E-17, -0.3543307086614173040 ) ) ;
#80313=CARTESIAN_POINT ( 'NONE',  ( -0.3392501089628017219, -0.1958661417322836995, -2.883877583498374531 ) ) ;
#80318=CARTESIAN_POINT ( 'NONE',  ( -0.3420746716998660508, -0.1974969037888706924, -0.7591863517060368771 ) ) ;
#80324=CARTESIAN_POINT ( 'NONE',  ( -0.3458507752293909498, 0.3458507752293907833, -1.122047244094488194 ) ) ;
#80326=CARTESIAN_POINT ( 'NONE',  ( 0.2925321140481932369, -0.2925321140481931814, -2.145669291338582418 ) ) ;
#80329=CARTESIAN_POINT ( 'NONE',  ( 0.3392501089628018884, -0.1958661417322833942, -0.5741662974091357174 ) ) ;
#80342=CARTESIAN_POINT ( 'NONE',  ( -0.1958661417322836718, 0.3392501089628017219, -1.107611548556430403 ) ) ;
#80345=CARTESIAN_POINT ( 'NONE',  ( -0.1974969037888706647, 0.3420746716998658843, -1.115485564304461885 ) ) ;
#80355=CARTESIAN_POINT ( 'NONE',  ( -0.1265901696524993347, 0.4724409448818896462, -0.3982939632545931530 ) ) ;
#80356=CARTESIAN_POINT ( 'NONE',  ( -0.3458507752293906723, -0.3458507752293910609, -0.6082677165354329896 ) ) ;
#80361=CARTESIAN_POINT ( 'NONE',  ( -0.3996062992125986035, -0.1070741851644056997, -1.620734908136482799 ) ) ;
#80364=CARTESIAN_POINT ( 'NONE',  ( 0.2925321140481932369, -0.2925321140481931814, -1.120078740157480324 ) ) ;
#80368=CARTESIAN_POINT ( 'NONE',  ( 0.3458507752293908943, 0.3458507752293908943, -0.4527559055118109965 ) ) ;
#80369=CARTESIAN_POINT ( 'NONE',  ( -0.3917322834645670104, -7.196005306013484475E-17, -2.486220472440944906 ) ) ;
#80375=CARTESIAN_POINT ( 'NONE',  ( 0.4724409448818898682, 2.892866454678787531E-17, -2.399606299212598604 ) ) ;
#80378=CARTESIAN_POINT ( 'NONE',  ( -0.1974969037888704149, -0.3420746716998661063, -1.874671916010499428 ) ) ;
#80390=CARTESIAN_POINT ( 'NONE',  ( -0.1958661417322836440, 0.3392501089628016664, -2.455361261645982562 ) ) ;
#80403=CARTESIAN_POINT ( 'NONE',  ( -0.3996062992125986590, 0.1070741851644051723, -0.1095800524934383152 ) ) ;
#80405=CARTESIAN_POINT ( 'NONE',  ( -0.1958661417322836718, 0.3392501089628017219, -1.987532808398950079 ) ) ;
#80414=CARTESIAN_POINT ( 'NONE',  ( -0.3460692066303957537, -0.1998031496062994405, -0.7591863517060367661 ) ) ;
#80416=CARTESIAN_POINT ( 'NONE',  ( 0.2362204724409449064, 0.4091458600556404646, -2.583333333333333481 ) ) ;
#80423=CARTESIAN_POINT ( 'NONE',  ( -0.3392501089628019995, 0.1958661417322832277, -1.370734908136483021 ) ) ;
#80428=CARTESIAN_POINT ( 'NONE',  ( 0.1070741851644053527, 0.3996062992125985480, -2.274934383202099397 ) ) ;
#80430=CARTESIAN_POINT ( 'NONE',  ( 0.2925321140481932369, -0.2925321140481932369, -0.5708661417322833387 ) ) ;
#80433=CARTESIAN_POINT ( 'NONE',  ( 0.3392501089628018329, 0.1958661417322835607, -2.170603674540682260 ) ) ;
#80443=CARTESIAN_POINT ( 'NONE',  ( 0.1049643490035304522, -0.3917322834645668994, -1.582657849572491449 ) ) ;
#80449=CARTESIAN_POINT ( 'NONE',  ( 0.2867679344610366554, -0.2867679344610365999, -2.772329027067928386 ) ) ;
#80458=CARTESIAN_POINT ( 'NONE',  ( 0.1049643490035304799, -0.3917322834645670104, -1.341882832842206774 ) ) ;
#80460=CARTESIAN_POINT ( 'NONE',  ( -0.1958661417322836718, 0.3392501089628017219, -2.302493438320210029 ) ) ;
#80466=CARTESIAN_POINT ( 'NONE',  ( -0.3460692066303960313, 0.1998031496062989965, -0.1030183727034120617 ) ) ;
#80468=CARTESIAN_POINT ( 'NONE',  ( 0.1998031496062992740, 0.3460692066303959757, -1.876640419947506411 ) ) ;
#80473=CARTESIAN_POINT ( 'NONE',  ( 0.1265901696524989462, 0.4724409448818897572, -0.5426509186351704539 ) ) ;
#80476=CARTESIAN_POINT ( 'NONE',  ( -0.2891555358219911054, 0.2891555358219909388, -0.4114173228346456046 ) ) ;
#80480=CARTESIAN_POINT ( 'NONE',  ( 0.3949938075777409963, 2.418639510665530743E-17, -0.6673228346456693272 ) ) ;
#80488=CARTESIAN_POINT ( 'NONE',  ( -9.787531504996566615E-17, 0.3996062992125985480, -1.494094488188976610 ) ) ;
#80490=CARTESIAN_POINT ( 'NONE',  ( 0.1958661417322836440, -0.3392501089628017219, -1.186351706036745446 ) ) ;
#80491=DIRECTION ( 'NONE',  ( 0.000000000000000000, 0.000000000000000000, 1.000000000000000000 ) ) ;
#80500=CARTESIAN_POINT ( 'NONE',  ( -0.2362204724409451284, 0.4091458600556402425, -0.2473753280839895152 ) ) ;
#80505=CARTESIAN_POINT ( 'NONE',  ( 0.4724409448818898682, 2.892866454678787531E-17, -0.3523622047244094335 ) ) ;
#80515=PLANE ( 'NONE',  #78315 ) ;
#80517=CARTESIAN_POINT ( 'NONE',  ( -0.2925321140481932369, 0.2925321140481931814, -1.122047244094488194 ) ) ;
#80523=( BOUNDED_CURVE ( )  B_SPLINE_CURVE ( 2, ( #53359, #21385, #47040, #72733, #15079, #40737, #54602, #23860, #43198, #49109, #4090, #17565, #29758, #11243, #62579, #61332, #29351, #48699, #68080, #74815, #4921, #47869, #67255, #16329, #41973, #55421, #62162, #81128, #17160, #30170, #35257, #3686, #55010, #74397, #60921, #10424, #4503, #54181, #15918, #73573, #9588, #35668, #3272, #80718, #23445, #68893, #36903, #79894, #42793, #28933, #80311, #16741, #67666, #22626, #48286, #10003, #41566, #73983, #23033, #55833, #81541, #68488, #22212, #42381, #36082, #61753, #49527, #10827, #36487, #75220, #77278, #63809, #70966, #38963, #37723, #5732, #25083, #44428, #51162, #64647, #70537, #43610, #76042, #18387, #6148, #38552, #31822, #76858, #6566, #11662, #63397, #57482, #50757, #30589, #5332, #69312, #49937, #56255, #62993, #32238, #37321, #30990, #12893, #76457, #19190, #83176, #82359, #25496, #44839, #64232, #70122, #18784, #56658, #57896, #12065, #82762, #31403, #263, #57068, #25916, #24677, #50345, #19608, #12473, #81951, #24264, #51575, #38135, #45270, #44028, #13311, #75635, #17973, #69721, #40228, #59162, #79376, #26338, #53669, #47358, #2353, #21695, #53255, #73047, #15396, #8661, #59997, #71381, #1520, #46526, #51999, #77704, #20034, #33500, #66322, #14981, #27596, #45685, #26759, #33079, #34332, #33912, #41058, #6984, #32653, #78967, #13731, #39385, #52836, #52414, #58746, #7409, #46109, #65070, #1108, #682, #40640, #28009, #58319, #78123, #21287, #20456, #71802, #14155, #39811, #1932, #65910, #65501, #8247 ),
 .UNSPECIFIED., .F., .F. ) 
 B_SPLINE_CURVE_WITH_KNOTS ( ( 3, 2, 2, 2, 2, 2, 2, 2, 2, 2, 2, 2, 2, 2, 2, 2, 2, 2, 2, 2, 2, 2, 2, 2, 2, 2, 2, 2, 2, 2, 2, 2, 2, 2, 2, 2, 2, 2, 2, 2, 2, 2, 2, 2, 2, 2, 2, 2, 2, 2, 2, 2, 2, 2, 2, 2, 2, 2, 2, 2, 2, 2, 2, 2, 2, 2, 2, 2, 2, 2, 2, 2, 2, 2, 2, 2, 2, 2, 2, 2, 2, 2, 2, 2, 2, 2, 2, 2, 2, 2, 2, 2, 2, 2, 3 ),
 ( 0.07563788552403453991, 0.07916666666666666297, 0.08333333333333332871, 0.08749999999999999445, 0.09166666666666666019, 0.09583333333333333981, 0.1000000000000000056, 0.1041666666666666713, 0.1083333333333333370, 0.1125000000000000028, 0.1166666666666666685, 0.1208333333333333343, 0.1250000000000000000, 0.1291666666666666796, 0.1333333333333333315, 0.1375000000000000111, 0.1416666666666666630, 0.1458333333333333426, 0.1499999999999999944, 0.1541666666666666741, 0.1583333333333333259, 0.1625000000000000333, 0.1666666666666666574, 0.1708333333333333370, 0.1749999999999999889, 0.1791666666666666685, 0.1833333333333333204, 0.1875000000000000000, 0.1916666666666666796, 0.1958333333333333315, 0.2000000000000000111, 0.2041666666666666630, 0.2083333333333333703, 0.2125000000000000222, 0.2166666666666666741, 0.2208333333333333259, 0.2250000000000000333, 0.2291666666666666852, 0.2333333333333333370, 0.2374999999999999889, 0.2416666666666666408, 0.2458333333333333481, 0.2500000000000000000, 0.2541666666666666519, 0.2583333333333333037, 0.2625000000000000111, 0.2666666666666666630, 0.2708333333333333148, 0.2750000000000000222, 0.2791666666666666741, 0.2833333333333333259, 0.2874999999999999778, 0.2916666666666666852, 0.2958333333333333370, 0.2999999999999999889, 0.3041666666666666408, 0.3083333333333333481, 0.3125000000000000000, 0.3166666666666666519, 0.3208333333333333592, 0.3250000000000000111, 0.3291666666666666630, 0.3333333333333333148, 0.3375000000000000222, 0.3416666666666666741, 0.3458333333333333259, 0.3499999999999999778, 0.3541666666666666852, 0.3583333333333333370, 0.3624999999999999889, 0.3666666666666666408, 0.3708333333333333481, 0.3750000000000000000, 0.3791666666666666519, 0.3833333333333333592, 0.3875000000000000111, 0.3916666666666666630, 0.3958333333333333148, 0.4000000000000000222, 0.4041666666666666741, 0.4083333333333333259, 0.4124999999999999778, 0.4166666666666667407, 0.4208333333333333370, 0.4249999999999999889, 0.4291666666666666963, 0.4333333333333333481, 0.4375000000000000000, 0.4416666666666665964, 0.4458333333333333592, 0.4500000000000000666, 0.4541666666666666630, 0.4583333333333333148, 0.4625000000000000222, 0.4631378855240345094 ),
 .UNSPECIFIED. ) 
 CURVE ( )  GEOMETRIC_REPRESENTATION_ITEM ( )  RATIONAL_B_SPLINE_CURVE ( ( 0.9911642120907997455, 0.9711423276059423237, 1.000000000000000000, 0.9659258262890683122, 1.000000000000000000, 0.9659258262890683122, 1.000000000000000000, 0.9659258262890683122, 1.000000000000000000, 0.9659258262890683122, 1.000000000000000000, 0.9659258262890683122, 1.000000000000000000, 0.9659258262890683122, 1.000000000000000000, 0.9659258262890683122, 1.000000000000000000, 0.9659258262890683122, 1.000000000000000000, 0.9659258262890683122, 1.000000000000000000, 0.9659258262890683122, 1.000000000000000000, 0.9659258262890683122, 1.000000000000000000, 0.9659258262890683122, 1.000000000000000000, 0.9659258262890683122, 1.000000000000000000, 0.9659258262890683122, 1.000000000000000000, 0.9659258262890683122, 1.000000000000000000, 0.9659258262890683122, 1.000000000000000000, 0.9659258262890683122, 1.000000000000000000, 0.9659258262890683122, 1.000000000000000000, 0.9659258262890683122, 1.000000000000000000, 0.9659258262890683122, 1.000000000000000000, 0.9659258262890683122, 1.000000000000000000, 0.9659258262890683122, 1.000000000000000000, 0.9659258262890683122, 1.000000000000000000, 0.9659258262890683122, 1.000000000000000000, 0.9659258262890683122, 1.000000000000000000, 0.9659258262890683122, 1.000000000000000000, 0.9659258262890683122, 1.000000000000000000, 0.9659258262890683122, 1.000000000000000000, 0.9659258262890683122, 1.000000000000000000, 0.9659258262890683122, 1.000000000000000000, 0.9659258262890683122, 1.000000000000000000, 0.9659258262890683122, 1.000000000000000000, 0.9659258262890683122, 1.000000000000000000, 0.9659258262890683122, 1.000000000000000000, 0.9659258262890683122, 1.000000000000000000, 0.9659258262890683122, 1.000000000000000000, 0.9659258262890683122, 1.000000000000000000, 0.9659258262890683122, 1.000000000000000000, 0.9659258262890683122, 1.000000000000000000, 0.9659258262890683122, 1.000000000000000000, 0.9659258262890683122, 1.000000000000000000, 0.9659258262890683122, 1.000000000000000000, 0.9659258262890683122, 1.000000000000000000, 0.9659258262890683122, 1.000000000000000000, 0.9659258262890683122, 1.000000000000000000, 0.9659258262890683122, 1.000000000000000000, 0.9659258262890683122, 1.000000000000000000, 0.9659258262890683122, 1.000000000000000000, 0.9659258262890683122, 1.000000000000000000, 0.9659258262890683122, 1.000000000000000000, 0.9659258262890683122, 1.000000000000000000, 0.9659258262890683122, 1.000000000000000000, 0.9659258262890683122, 1.000000000000000000, 0.9659258262890683122, 1.000000000000000000, 0.9659258262890683122, 1.000000000000000000, 0.9659258262890683122, 1.000000000000000000, 0.9659258262890683122, 1.000000000000000000, 0.9659258262890683122, 1.000000000000000000, 0.9659258262890683122, 1.000000000000000000, 0.9659258262890683122, 1.000000000000000000, 0.9659258262890683122, 1.000000000000000000, 0.9659258262890683122, 1.000000000000000000, 0.9659258262890683122, 1.000000000000000000, 0.9659258262890683122, 1.000000000000000000, 0.9659258262890683122, 1.000000000000000000, 0.9659258262890683122, 1.000000000000000000, 0.9659258262890683122, 1.000000000000000000, 0.9659258262890683122, 1.000000000000000000, 0.9659258262890683122, 1.000000000000000000, 0.9659258262890683122, 1.000000000000000000, 0.9659258262890683122, 1.000000000000000000, 0.9659258262890683122, 1.000000000000000000, 0.9659258262890683122, 1.000000000000000000, 0.9659258262890683122, 1.000000000000000000, 0.9659258262890683122, 1.000000000000000000, 0.9659258262890683122, 1.000000000000000000, 0.9659258262890683122, 1.000000000000000000, 0.9659258262890683122, 1.000000000000000000, 0.9659258262890683122, 1.000000000000000000, 0.9659258262890683122, 1.000000000000000000, 0.9659258262890683122, 1.000000000000000000, 0.9659258262890683122, 1.000000000000000000, 0.9659258262890683122, 1.000000000000000000, 0.9659258262890683122, 1.000000000000000000, 0.9659258262890683122, 1.000000000000000000, 0.9659258262890683122, 1.000000000000000000, 0.9659258262890683122, 1.000000000000000000, 0.9659258262890683122, 1.000000000000000000, 0.9659258262890683122, 1.000000000000000000, 0.9659258262890683122, 1.000000000000000000, 0.9659258262890683122, 1.000000000000000000, 0.9659258262890683122, 1.000000000000000000, 0.9947834986831268766, 0.9911642120908008557 ) ) 
 REPRESENTATION_ITEM ( '' )  );
#80524=CARTESIAN_POINT ( 'NONE',  ( -0.4724409448818895907, -0.1265901696524993070, -0.04593175853018372640 ) ) ;
#80525=CARTESIAN_POINT ( 'NONE',  ( -0.1974969037888703871, -0.3420746716998661063, -2.270341207349081181 ) ) ;
#80526=ORIENTED_EDGE ( 'NONE', *, *, #47459, .T. ) ;
#80528=CARTESIAN_POINT ( 'NONE',  ( -0.2867679344610365999, 0.2867679344610364889, -0.7992125984251968740 ) ) ;
#80530=CARTESIAN_POINT ( 'NONE',  ( -0.3458507752293909498, 0.3458507752293907833, -2.381889763779527325 ) ) ;
#80537=CARTESIAN_POINT ( 'NONE',  ( 0.1049643490035303689, 0.3917322834645668994, -0.3884321277877147427 ) ) ;
#80542=DIRECTION ( 'NONE',  ( 0.000000000000000000, 0.000000000000000000, -1.000000000000000000 ) ) ;
#80544=CARTESIAN_POINT ( 'NONE',  ( -0.2867679344610367109, 0.2867679344610365444, -1.748706979823833718 ) ) ;
#80550=CARTESIAN_POINT ( 'NONE',  ( -0.3917322834645671215, 0.1049643490035301469, -0.9048556430446195176 ) ) ;
#80558=CARTESIAN_POINT ( 'NONE',  ( 0.4724409448818898682, 2.892866454678787531E-17, -1.220472440944881942 ) ) ;
#80560=CARTESIAN_POINT ( 'NONE',  ( -0.2867679344610365999, 0.2867679344610364889, -2.531496062992125484 ) ) ;
#80567=CARTESIAN_POINT ( 'NONE',  ( -0.1958661417322834220, -0.3392501089628018884, -0.9376640419947508409 ) ) ;
#80570=CARTESIAN_POINT ( 'NONE',  ( -0.1958661417322834220, -0.3392501089628018884, -1.725065616797900381 ) ) ;
#80572=CARTESIAN_POINT ( 'NONE',  ( 0.2925321140481932369, -0.2925321140481931814, -2.379921259842520342 ) ) ;
#80581=CARTESIAN_POINT ( 'NONE',  ( -0.2925321140481930149, -0.2925321140481933480, -2.183070866141731958 ) ) ;
#80584=CARTESIAN_POINT ( 'NONE',  ( -0.1049643490035307020, 0.3917322834645669549, 0.001312335958005294862 ) ) ;
#80590=CARTESIAN_POINT ( 'NONE',  ( 0.1958661417322836162, -0.3392501089628018329, -1.274258899441258031 ) ) ;
#80598=CARTESIAN_POINT ( 'NONE',  ( -0.3392501089628019995, 0.1958661417322831999, -0.4954261399288207857 ) ) ;
#80601=CARTESIAN_POINT ( 'NONE',  ( -1.157146581871515012E-16, 0.4724409448818898682, -1.966535433070865979 ) ) ;
#80621=CARTESIAN_POINT ( 'NONE',  ( -0.3996062992125985480, -7.340648628747423112E-17, -2.163385826771653697 ) ) ;
#80627=CARTESIAN_POINT ( 'NONE',  ( -0.2925321140481930704, -0.2925321140481933480, -1.633858267716534973 ) ) ;
#80628=CARTESIAN_POINT ( 'NONE',  ( 0.3949938075777411073, -0.1058382717557499464, -1.056430446194225770 ) ) ;
#80629=CARTESIAN_POINT ( 'NONE',  ( -0.1998031496062994683, 0.3460692066303958092, -2.375328083989501238 ) ) ;
#80631=CARTESIAN_POINT ( 'NONE',  ( -0.1208384647389192101, 0.3726288332213502641, 1.112018681666451222E-17 ) ) ;
#80635=CARTESIAN_POINT ( 'NONE',  ( 0.2891555358219910499, 0.2891555358219910499, -2.261811023622047667 ) ) ;
#80639=CARTESIAN_POINT ( 'NONE',  ( 0.1265901696524990294, -0.4724409448818896462, -2.447506561679789527 ) ) ;
#80640=CARTESIAN_POINT ( 'NONE',  ( -0.3460692066303958092, -0.1998031496062994683, -1.942257217847769057 ) ) ;
#80641=CARTESIAN_POINT ( 'NONE',  ( 0.4724409448818898682, 2.892866454678787531E-17, -2.714566929133858331 ) ) ;
#80647=CARTESIAN_POINT ( 'NONE',  ( 0.3917322834645669549, 2.398668435337827645E-17, -2.717828453247031817 ) ) ;
#80654=CARTESIAN_POINT ( 'NONE',  ( 4.797336870675656522E-17, -0.3917322834645670104, -0.1633858267716536417 ) ) ;
#80656=( BOUNDED_CURVE ( )  B_SPLINE_CURVE ( 2, ( #63152, #76208, #44189, #749, #75382, #39453, #65141, #7477, #62749, #36648, #56821, #56000, #32721 ),
 .UNSPECIFIED., .F., .F. ) 
 B_SPLINE_CURVE_WITH_KNOTS ( ( 3, 2, 2, 2, 2, 2, 3 ),
 ( 0.4125000000000000333, 0.4166666666666667407, 0.4208333333333333925, 0.4250000000000000444, 0.4291666666666666408, 0.4333333333333333481, 0.4375000000000000000 ),
 .UNSPECIFIED. ) 
 CURVE ( )  GEOMETRIC_REPRESENTATION_ITEM ( )  RATIONAL_B_SPLINE_CURVE ( ( 0.9999999999999995559, 0.9659258262890687563, 1.000000000000000000, 0.9659258262890683122, 1.000000000000000000, 0.9659258262890683122, 1.000000000000000000, 0.9659258262890683122, 1.000000000000000000, 0.9659258262890683122, 1.000000000000000000, 0.9659258262890683122, 1.000000000000000000 ) ) 
 REPRESENTATION_ITEM ( '' )  );
#80657=CARTESIAN_POINT ( 'NONE',  ( 0.3392501089628018329, 0.1958661417322835607, -2.170603674540682260 ) ) ;
#80659=EDGE_LOOP ( 'NONE', ( #13000, #59794, #59565, #75574 ) ) ;
#80660=CARTESIAN_POINT ( 'NONE',  ( -0.1058382717557503211, 0.3949938075777409408, -2.526246719160105236 ) ) ;
#80664=CARTESIAN_POINT ( 'NONE',  ( 0.3460692066303959202, 0.1998031496062993295, -0.9186351706036745002 ) ) ;
#80669=CARTESIAN_POINT ( 'NONE',  ( 0.1958661417322836440, -0.3392501089628017219, -0.01902887139107619849 ) ) ;
#80679=CARTESIAN_POINT ( 'NONE',  ( -0.2362204724409447953, -0.4091458600556404646, -1.640419947506561726 ) ) ;
#80681=CARTESIAN_POINT ( 'NONE',  ( 0.1049643490035303689, 0.3917322834645670104, -0.7729658792650916377 ) ) ;
#80690=CARTESIAN_POINT ( 'NONE',  ( 0.2867679344610365999, -0.2867679344610365999, -0.02097805954624490030 ) ) ;
#80692=CARTESIAN_POINT ( 'NONE',  ( -0.1958661417322834220, -0.3392501089628018884, -0.3077427821522311091 ) ) ;
#80697=CARTESIAN_POINT ( 'NONE',  ( -0.2867679344610365999, 0.2867679344610364889, -2.374015748031496287 ) ) ;
#80700=CARTESIAN_POINT ( 'NONE',  ( 0.3458507752293908943, -0.3458507752293908943, -0.6476377952755905110 ) ) ;
#80710=CARTESIAN_POINT ( 'NONE',  ( -0.3996062992125986590, 0.1070741851644051723, -1.999343832020997525 ) ) ;
#80718=CARTESIAN_POINT ( 'NONE',  ( -0.3996062992125984925, -0.1070741851644056719, -0.2801837270341207553 ) ) ;
#80720=CARTESIAN_POINT ( 'NONE',  ( 0.1070741851644053527, 0.3996062992125986590, -0.4658792650918635592 ) ) ;
#80721=CARTESIAN_POINT ( 'NONE',  ( 0.2867679344610366554, -0.2867679344610365999, -2.772329027067928386 ) ) ;
#80727=CARTESIAN_POINT ( 'NONE',  ( 0.1974969037888706092, -0.3420746716998660508, -0.7985564304461942875 ) ) ;
#80732=CARTESIAN_POINT ( 'NONE',  ( 0.1265901696524989462, 0.4724409448818897572, -1.253280839895013044 ) ) ;
#80733=CARTESIAN_POINT ( 'NONE',  ( 0.1070741851644054915, -0.3996062992125985480, -2.447506561679789527 ) ) ;
#80736=CARTESIAN_POINT ( 'NONE',  ( -0.3917322834645670659, -7.196005306013484475E-17, -0.6660298144695031564 ) ) ;
#80737=ORIENTED_EDGE ( 'NONE', *, *, #13177, .T. ) ;
#80747=CARTESIAN_POINT ( 'NONE',  ( 0.3917322834645669549, 0.1049643490035304660, -1.219160104986876325 ) ) ;
#80750=CARTESIAN_POINT ( 'NONE',  ( 0.3949938075777409408, 0.1058382717557500574, -0.9120734908136481911 ) ) ;
#80766=CARTESIAN_POINT ( 'NONE',  ( -0.3460692066303958092, -0.1998031496062994683, -1.784776902887138972 ) ) ;
#80769=CARTESIAN_POINT ( 'NONE',  ( 0.1998031496062994128, -0.3460692066303957537, -1.270997375328083878 ) ) ;
#80773=CARTESIAN_POINT ( 'NONE',  ( 0.3458507752293908943, -0.3458507752293908943, -0.4133858267716534196 ) ) ;
#80774=CARTESIAN_POINT ( 'NONE',  ( 4.797336870675656522E-17, -0.3917322834645670104, -2.525590551181102317 ) ) ;
#80780=CARTESIAN_POINT ( 'NONE',  ( -0.4724409448818899238, 0.1265901696524986686, -2.156824146981627166 ) ) ;
#80782=CARTESIAN_POINT ( 'NONE',  ( -0.2891555358219909388, -0.2891555358219912164, -1.868110236220472009 ) ) ;
#80793=CARTESIAN_POINT ( 'NONE',  ( -9.594673741351310580E-17, 0.3917322834645669549, -2.442237902065930388 ) ) ;
#80797=CARTESIAN_POINT ( 'NONE',  ( -0.3458507752293909498, 0.3458507752293908388, -1.041338582677165281 ) ) ;
#80807=CARTESIAN_POINT ( 'NONE',  ( -9.787531504996566615E-17, 0.3996062992125985480, -0.3917322834645669549 ) ) ;
#80810=CARTESIAN_POINT ( 'NONE',  ( 0.1049643490035304938, -0.3917322834645669549, -1.902230971128608727 ) ) ;
#80819=CARTESIAN_POINT ( 'NONE',  ( 0.3460692066303958092, 0.1998031496062993018, -1.467847769028871596 ) ) ;
#80826=CARTESIAN_POINT ( 'NONE',  ( 0.1958661417322836440, -0.3392501089628017219, -1.593832020997375531 ) ) ;
#80827=CARTESIAN_POINT ( 'NONE',  ( -0.3458507752293906723, -0.3458507752293910609, -2.106299212598425008 ) ) ;
#80830=CARTESIAN_POINT ( 'NONE',  ( 0.4724409448818898682, 2.892866454678787531E-17, -2.637795275590551380 ) ) ;
#80831=CARTESIAN_POINT ( 'NONE',  ( 0.1998031496062994128, -0.3460692066303957537, -2.530839895013123453 ) ) ;
#80834=CARTESIAN_POINT ( 'NONE',  ( 0.3996062992125986590, -0.1070741851644053111, -0.7414698162729659314 ) ) ;
#80837=CARTESIAN_POINT ( 'NONE',  ( 0.2867679344610365999, 0.2867679344610365999, -2.807086614173227357 ) ) ;
#80848=CARTESIAN_POINT ( 'NONE',  ( -0.1049643490035301746, -0.3917322834645670659, -1.727014804953068916 ) ) ;
#80852=CARTESIAN_POINT ( 'NONE',  ( 0.3392501089628018329, 0.1958661417322835607, -2.735564304461941987 ) ) ;
#80855=CARTESIAN_POINT ( 'NONE',  ( -0.3917322834645671770, 0.1049643490035302024, -2.706712229167666184 ) ) ;
#80863=CARTESIAN_POINT ( 'NONE',  ( -0.3917322834645670659, -7.196005306013484475E-17, -1.453431389272652696 ) ) ;
#80865=CARTESIAN_POINT ( 'NONE',  ( 0.3917322834645670104, 2.398668435337828261E-17, -2.092519685039370358 ) ) ;
#80870=CARTESIAN_POINT ( 'NONE',  ( 0.2925321140481932369, -0.2925321140481932369, -0.5708661417322833387 ) ) ;
#80872=CARTESIAN_POINT ( 'NONE',  ( 4.893765752498283308E-17, -0.3996062992125985480, 0.001968503937007862279 ) ) ;
#80874=CARTESIAN_POINT ( 'NONE',  ( 0.1070741851644054915, -0.3996062992125986035, -2.132545931758530244 ) ) ;
#80879=CARTESIAN_POINT ( 'NONE',  ( 0.4724409448818897572, -0.1265901696524988906, -0.9757217847769029673 ) ) ;
#80882=CARTESIAN_POINT ( 'NONE',  ( 0.2891555358219910499, 0.2891555358219910499, -0.5295275590551180578 ) ) ;
#80895=CARTESIAN_POINT ( 'NONE',  ( 0.3996062992125985480, 2.446882876249141654E-17, -1.927165354330708791 ) ) ;
#80897=CARTESIAN_POINT ( 'NONE',  ( 0.3917322834645669549, 0.1049643490035304660, -1.219160104986876325 ) ) ;
#80919=CARTESIAN_POINT ( 'NONE',  ( 0.3917322834645670659, 2.398668435337828261E-17, -2.162092806595487637 ) ) ;
#80929=CARTESIAN_POINT ( 'NONE',  ( -0.1998031496062994683, 0.3460692066303958092, -2.847769028871391050 ) ) ;
#80930=CARTESIAN_POINT ( 'NONE',  ( -0.3949938075777409963, -7.255918531996591613E-17, -2.401574803149606474 ) ) ;
#80933=CARTESIAN_POINT ( 'NONE',  ( 0.3917322834645670104, 2.398668435337828261E-17, -0.8976377952755905110 ) ) ;
#80935=CARTESIAN_POINT ( 'NONE',  ( 0.4091458600556404646, -0.2362204724409448231, -2.309711286089239035 ) ) ;
#80942=CARTESIAN_POINT ( 'NONE',  ( 0.2867679344610365999, -0.2867679344610365999, -0.1784583745068747673 ) ) ;
#80948=CARTESIAN_POINT ( 'NONE',  ( 0.2017716535433070613, -0.2017716535433070890, -0.3937007874015748254 ) ) ;
#80949=CARTESIAN_POINT ( 'NONE',  ( 0.3996062992125986590, -0.1070741851644053111, -2.946194225721785465 ) ) ;
#80950=CARTESIAN_POINT ( 'NONE',  ( -0.3917322834645670104, -0.1049643490035307020, -1.617473384023309091 ) ) ;
#80956=CARTESIAN_POINT ( 'NONE',  ( -9.594673741351313045E-17, 0.3917322834645670104, -1.029527559055118280 ) ) ;
#80967=CARTESIAN_POINT ( 'NONE',  ( 0.3917322834645669549, 0.1049643490035304660, -2.479002624671915900 ) ) ;
#80975=CARTESIAN_POINT ( 'NONE',  ( -0.1958661417322834220, -0.3392501089628018884, -0.7801837270341208663 ) ) ;
#80977=FACE_OUTER_BOUND ( 'NONE', #60428, .T. ) ;
#80979=CARTESIAN_POINT ( 'NONE',  ( -0.1070741851644051862, -0.3996062992125986590, -2.353674540682414218 ) ) ;
#80997=CARTESIAN_POINT ( 'NONE',  ( 4.797336870675655290E-17, -0.3917322834645669549, -1.576096169782465140 ) ) ;
#81006=CARTESIAN_POINT ( 'NONE',  ( -0.3392501089628017219, -0.1958661417322836995, -0.3641925441282957698 ) ) ;
#81009=CARTESIAN_POINT ( 'NONE',  ( -0.1265901696524986964, -0.4724409448818899238, -1.881233595800524849 ) ) ;
#81032=CARTESIAN_POINT ( 'NONE',  ( 0.3996062992125984925, 0.1070741851644054637, -2.248687664041995049 ) ) ;
#81037=CARTESIAN_POINT ( 'NONE',  ( -0.1070741851644056997, 0.3996062992125986035, -1.581364829396325389 ) ) ;
#81038=CARTESIAN_POINT ( 'NONE',  ( 0.3420746716998660508, -0.1974969037888703871, -0.8923884514435694859 ) ) ;
#81039=CARTESIAN_POINT ( 'NONE',  ( -0.3460692066303958092, -0.1998031496062994683, -2.572178477690288734 ) ) ;
#81041=CARTESIAN_POINT ( 'NONE',  ( 0.3392501089628018329, 0.1958661417322835607, -0.7532808398950130435 ) ) ;
#81045=CARTESIAN_POINT ( 'NONE',  ( 0.1974969037888706092, -0.3420746716998660508, -2.058398950131233640 ) ) ;
#81049=CARTESIAN_POINT ( 'NONE',  ( -0.1265901696524993347, 0.4724409448818895907, -2.368766404199475151 ) ) ;
#81050=CARTESIAN_POINT ( 'NONE',  ( 4.893765752498283924E-17, -0.3996062992125986035, -1.811023622047244208 ) ) ;
#81055=CARTESIAN_POINT ( 'NONE',  ( -0.3917322834645668994, -0.1049643490035306742, -2.645649975556744415 ) ) ;
#81062=CARTESIAN_POINT ( 'NONE',  ( 0.3917322834645670104, 2.398668435337828261E-17, -0.04527559055118119541 ) ) ;
#81064=CARTESIAN_POINT ( 'NONE',  ( 0.3392501089628018329, 0.1958661417322835607, -2.328083989501312345 ) ) ;
#81066=VERTEX_POINT ( 'NONE', #37968 ) ;
#81067=CARTESIAN_POINT ( 'NONE',  ( -0.3420746716998661618, 0.1974969037888702206, -2.545931758530183497 ) ) ;
#81071=CARTESIAN_POINT ( 'NONE',  ( 0.3996062992125986035, 2.446882876249141962E-17, -1.062992125984252079 ) ) ;
#81073=CARTESIAN_POINT ( 'NONE',  ( 0.1265901696524990572, -0.4724409448818897017, -0.7919947506561678674 ) ) ;
#81076=CARTESIAN_POINT ( 'NONE',  ( 0.1049643490035303689, 0.3917322834645670104, -0.2355643044619422921 ) ) ;
#81083=CARTESIAN_POINT ( 'NONE',  ( -0.1958661417322836718, 0.3392501089628017219, -0.1627296587926508609 ) ) ;
#81087=CARTESIAN_POINT ( 'NONE',  ( 0.1265901696524990294, -0.4724409448818896462, -1.660104986876640210 ) ) ;
#81089=CARTESIAN_POINT ( 'NONE',  ( 0.3392501089628018884, -0.1958661417322834220, -2.709317585301837195 ) ) ;
#81096=CARTESIAN_POINT ( 'NONE',  ( 0.3917322834645668994, 0.1049643490035304522, -0.2047050936669798094 ) ) ;
#81098=CARTESIAN_POINT ( 'NONE',  ( 0.3917322834645670104, 2.398668435337828261E-17, -0.5177165354330709457 ) ) ;
#81104=CARTESIAN_POINT ( 'NONE',  ( -0.3392501089628017219, -0.1958661417322836718, -2.406824146981627166 ) ) ;
#81108=CARTESIAN_POINT ( 'NONE',  ( 0.2362204724409449064, 0.4091458600556404646, -0.6935695538057742304 ) ) ;
#81115=DIRECTION ( 'NONE',  ( 0.000000000000000000, 0.000000000000000000, 1.000000000000000000 ) ) ;
#81119=ORIENTED_EDGE ( 'NONE', *, *, #20687, .F. ) ;
#81120=CARTESIAN_POINT ( 'NONE',  ( 0.3460692066303959202, -0.1998031496062991630, -1.914041994750656395 ) ) ;
#81128=CARTESIAN_POINT ( 'NONE',  ( 0.2925321140481931814, -0.2925321140481931259, -0.1751968503937008370 ) ) ;
#81129=CARTESIAN_POINT ( 'NONE',  ( 0.3460692066303959757, -0.1998031496062991907, -0.5774278215223097588 ) ) ;
#81131=CARTESIAN_POINT ( 'NONE',  ( 0.3392501089628018329, 0.1958661417322835607, -2.805137426018059710 ) ) ;
#81136=CARTESIAN_POINT ( 'NONE',  ( 0.3949938075777409963, 2.418639510665530743E-17, -0.8248031496062994128 ) ) ;
#81142=CARTESIAN_POINT ( 'NONE',  ( -0.1265901696524993347, 0.4724409448818895907, -1.266404199475065440 ) ) ;
#81143=CARTESIAN_POINT ( 'NONE',  ( -0.1998031496062991907, -0.3460692066303959757, -2.270341207349081181 ) ) ;
#81145=ORIENTED_EDGE ( 'NONE', *, *, #49585, .F. ) ;
#81146=CARTESIAN_POINT ( 'NONE',  ( 0.2867679344610366554, 0.2867679344610366554, -0.7644550113198971264 ) ) ;
#81157=CARTESIAN_POINT ( 'NONE',  ( 0.1049643490035304938, -0.3917322834645669549, -1.179790026246718915 ) ) ;
#81160=CARTESIAN_POINT ( 'NONE',  ( 0.3949938075777409408, 0.1058382717557500574, -1.541994750656168200 ) ) ;
#81164=CARTESIAN_POINT ( 'NONE',  ( 4.893765752498283924E-17, -0.3996062992125986035, 0.07874015748031494566 ) ) ;
#81170=CARTESIAN_POINT ( 'NONE',  ( 0.4724409448818897017, 0.1265901696524990294, -0.3589238845144357426 ) ) ;
#81171=CARTESIAN_POINT ( 'NONE',  ( -0.3917322834645670104, -7.196005306013484475E-17, -0.1240157480314961758 ) ) ;
#81177=CARTESIAN_POINT ( 'NONE',  ( 0.1998031496062992740, 0.3460692066303959757, -2.191601049868766360 ) ) ;
#81179=ORIENTED_EDGE ( 'NONE', *, *, #71143, .T. ) ;
#81180=CARTESIAN_POINT ( 'NONE',  ( -0.3460692066303957537, -0.1998031496062994405, -1.546587926509186639 ) ) ;
#81184=CARTESIAN_POINT ( 'NONE',  ( 0.3458507752293908943, -0.3458507752293908943, -0.5708661417322833387 ) ) ;
#81186=CARTESIAN_POINT ( 'NONE',  ( 0.3917322834645670104, 2.398668435337828261E-17, -2.407480314960630086 ) ) ;
#81192=CARTESIAN_POINT ( 'NONE',  ( -0.2362204724409447953, -0.4091458600556404646, -2.504593175853018661 ) ) ;
#81196=CARTESIAN_POINT ( 'NONE',  ( 0.3420746716998660508, 0.1974969037888705814, -1.625328083989501460 ) ) ;
#81217=CARTESIAN_POINT ( 'NONE',  ( 0.1070741851644053388, 0.3996062992125986035, -0.5426509186351704539 ) ) ;
#81218=CARTESIAN_POINT ( 'NONE',  ( 0.3917322834645670104, 2.398668435337828261E-17, -1.935039370078740273 ) ) ;
#81227=CARTESIAN_POINT ( 'NONE',  ( -0.3996062992125984925, -0.1070741851644056858, -1.540026246719160108 ) ) ;
#81235=CARTESIAN_POINT ( 'NONE',  ( 0.3917322834645670104, -0.1049643490035303411, -1.770997375328083656 ) ) ;
#81240=CARTESIAN_POINT ( 'NONE',  ( -0.1998031496062991630, -0.3460692066303959202, -2.347112860892388575 ) ) ;
#81242=CARTESIAN_POINT ( 'NONE',  ( -0.3996062992125986035, -7.340648628747425578E-17, -0.9842519685039369248 ) ) ;
#81246=CARTESIAN_POINT ( 'NONE',  ( 0.3917322834645669549, 0.1049643490035304660, -2.636482939632545985 ) ) ;
#81256=CARTESIAN_POINT ( 'NONE',  ( -0.1958661417322834497, -0.3392501089628018884, -2.192894070044932420 ) ) ;
#81259=CARTESIAN_POINT ( 'NONE',  ( -0.2867679344610364334, -0.2867679344610367109, -2.663385826771653253 ) ) ;
#81262=CARTESIAN_POINT ( 'NONE',  ( 0.1058382717557500713, -0.3949938075777409408, -0.08530183727034125474 ) ) ;
#81270=CARTESIAN_POINT ( 'NONE',  ( -0.3392501089628017219, -0.1958661417322836995, -1.466554748852705092 ) ) ;
#81272=CARTESIAN_POINT ( 'NONE',  ( -0.2867679344610364334, -0.2867679344610367109, -2.033464566929133355 ) ) ;
#81277=CARTESIAN_POINT ( 'NONE',  ( 0.2925321140481932369, -0.2925321140481932369, -0.4133858267716534196 ) ) ;
#81279=CARTESIAN_POINT ( 'NONE',  ( -0.1998031496062994405, 0.3460692066303957537, -0.2473753280839895152 ) ) ;
#81281=CARTESIAN_POINT ( 'NONE',  ( 0.1998031496062992740, 0.3460692066303959757, -2.349081364829396446 ) ) ;
#81282=EDGE_CURVE ( 'NONE', #65725, #60134, #61548, .T. ) ;
#81288=CARTESIAN_POINT ( 'NONE',  ( 0.4724409448818898682, 2.892866454678787531E-17, -1.139763779527559029 ) ) ;
#81291=EDGE_CURVE ( 'NONE', #57445, #53885, #53010, .T. ) ;
#81292=CARTESIAN_POINT ( 'NONE',  ( -0.3949938075777411073, 0.1058382717557497660, -0.7395013123359579499 ) ) ;
#81299=DIRECTION ( 'NONE',  ( 0.000000000000000000, 0.000000000000000000, 1.000000000000000000 ) ) ;
#81306=CARTESIAN_POINT ( 'NONE',  ( 0.3460692066303959202, -0.1998031496062991630, -1.599081364829396446 ) ) ;
#81308=CARTESIAN_POINT ( 'NONE',  ( 0.3392501089628018329, 0.1958661417322835607, -1.698162729658792891 ) ) ;
#81310=CARTESIAN_POINT ( 'NONE',  ( -0.3922539627124310702, 0.006303098004691234414, -4.648478490738284608E-18 ) ) ;
#81330=CARTESIAN_POINT ( 'NONE',  ( -0.3917322834645670659, -7.196005306013484475E-17, -2.240832964075802458 ) ) ;
#81337=CARTESIAN_POINT ( 'NONE',  ( -0.3996062992125986590, 0.1070741851644051862, -1.135170603674540590 ) ) ;
#81338=CARTESIAN_POINT ( 'NONE',  ( 0.3392501089628018329, 0.1958661417322835607, -2.170603674540682260 ) ) ;
#81341=CARTESIAN_POINT ( 'NONE',  ( 0.2362204724409451007, -0.4091458600556402980, -0.09186351706036745279 ) ) ;
#81342=CARTESIAN_POINT ( 'NONE',  ( -9.674558042662121740E-17, 0.3949938075777409963, -2.834645669291338432 ) ) ;
#81345=CARTESIAN_POINT ( 'NONE',  ( 0.3392501089628018329, 0.1958661417322835607, -1.225721784776902634 ) ) ;
#81348=CARTESIAN_POINT ( 'NONE',  ( 0.1265901696524989462, 0.4724409448818897572, -2.513123359580052174 ) ) ;
#81355=CARTESIAN_POINT ( 'NONE',  ( 0.1958661417322836162, -0.3392501089628018329, -0.1718966947168485970 ) ) ;
#81361=FACE_OUTER_BOUND ( 'NONE', #62276, .T. ) ;
#81362=CARTESIAN_POINT ( 'NONE',  ( 0.3392501089628018329, 0.1958661417322835607, -1.545294906333020135 ) ) ;
#81368=CARTESIAN_POINT ( 'NONE',  ( 0.3392501089628018329, 0.1958661417322835607, -1.003280839895013266 ) ) ;
#81378=CARTESIAN_POINT ( 'NONE',  ( -0.1049643490035302024, -0.3917322834645671215, -2.583989501312335513 ) ) ;
#81385=CARTESIAN_POINT ( 'NONE',  ( 0.1958661417322834775, 0.3392501089628018884, -0.8589238845144357981 ) ) ;
#81388=CARTESIAN_POINT ( 'NONE',  ( 0.3460692066303959202, -0.1998031496062991630, -2.543963254593176071 ) ) ;
#81398=CARTESIAN_POINT ( 'NONE',  ( -0.3996062992125984925, -0.1070741851644056858, -0.5951443569553805935 ) ) ;
#81407=CARTESIAN_POINT ( 'NONE',  ( 0.3392501089628018329, -0.1958661417322834497, -1.444862573981940512 ) ) ;
#81417=CARTESIAN_POINT ( 'NONE',  ( -0.2867679344610365444, -0.2867679344610367664, -0.3707542239183220789 ) ) ;
#81421=CARTESIAN_POINT ( 'NONE',  ( 0.1265901696524990294, -0.4724409448818896462, -2.209317585301837195 ) ) ;
#81443=CARTESIAN_POINT ( 'NONE',  ( 0.1998031496062992463, 0.3460692066303959202, -2.425853018372703396 ) ) ;
#81448=CARTESIAN_POINT ( 'NONE',  ( 4.893765752498283924E-17, -0.3996062992125986035, -1.811023622047244208 ) ) ;
#81449=CARTESIAN_POINT ( 'NONE',  ( 0.3949938075777409963, 2.418639510665530435E-17, -1.692913385826771533 ) ) ;
#81452=CARTESIAN_POINT ( 'NONE',  ( -0.2867679344610364334, -0.2867679344610367109, -0.5236220472440944462 ) ) ;
#81456=CARTESIAN_POINT ( 'NONE',  ( -0.3420746716998660508, -0.1974969037888706924, -2.019028871391076230 ) ) ;
#81460=CARTESIAN_POINT ( 'NONE',  ( -1.157146581871515012E-16, 0.4724409448818898682, -2.362204724409448620 ) ) ;
#81461=CARTESIAN_POINT ( 'NONE',  ( 0.3460692066303959757, -0.1998031496062991907, -1.837270341207349000 ) ) ;
#81467=CARTESIAN_POINT ( 'NONE',  ( 0.3917322834645668994, 0.1049643490035304522, -2.724390133037059236 ) ) ;
#81474=CARTESIAN_POINT ( 'NONE',  ( 0.3392501089628018329, 0.1958661417322835607, -0.2158792650918636147 ) ) ;
#81476=CARTESIAN_POINT ( 'NONE',  ( 0.1958661417322834775, 0.3392501089628018884, -2.498687664041994605 ) ) ;
#81479=CARTESIAN_POINT ( 'NONE',  ( 0.1058382717557500713, -0.3949938075777409408, -2.762467191601050587 ) ) ;
#81484=CARTESIAN_POINT ( 'NONE',  ( -0.3996062992125986035, -7.340648628747425578E-17, -0.8267716535433070613 ) ) ;
#81489=CARTESIAN_POINT ( 'NONE',  ( -0.1958661417322836718, 0.3392501089628017219, -0.2552493438320210806 ) ) ;
#81495=CARTESIAN_POINT ( 'NONE',  ( -0.1049643490035307020, 0.3917322834645669549, -0.3136482939632545541 ) ) ;
#81499=CARTESIAN_POINT ( 'NONE',  ( -0.1265901696524986964, -0.4724409448818899238, -1.646981627296587591 ) ) ;
#81501=CARTESIAN_POINT ( 'NONE',  ( 0.2867679344610366554, 0.2867679344610366554, -2.742125984251967630 ) ) ;
#81508=CARTESIAN_POINT ( 'NONE',  ( -0.1958661417322836440, 0.3392501089628016664, -0.2506368521971635843 ) ) ;
#81510=CARTESIAN_POINT ( 'NONE',  ( -0.3917322834645671215, 0.1049643490035301469, -0.5898950131233596794 ) ) ;
#81516=CARTESIAN_POINT ( 'NONE',  ( -0.2867679344610365999, 0.2867679344610364889, -2.216535433070866201 ) ) ;
#81521=CARTESIAN_POINT ( 'NONE',  ( 0.4091458600556404646, -0.2362204724409448231, -0.9691601049868766582 ) ) ;
#81532=CARTESIAN_POINT ( 'NONE',  ( -0.2925321140481932369, 0.2925321140481931259, -1.828740157480315265 ) ) ;
#81535=VECTOR ( 'NONE', #81603, 39.37007874015748143 ) ;
#81541=CARTESIAN_POINT ( 'NONE',  ( -9.787531504996566615E-17, 0.3996062992125985480, -0.3917322834645669549 ) ) ;
#81542=CARTESIAN_POINT ( 'NONE',  ( 0.1998031496062994405, -0.3460692066303958092, -0.4068241469816273326 ) ) ;
#81543=CARTESIAN_POINT ( 'NONE',  ( 0.3917322834645670659, 2.398668435337828261E-17, -2.949494381398636733 ) ) ;
#81548=CARTESIAN_POINT ( 'NONE',  ( 0.4724409448818898127, -0.1265901696524988629, -2.393044619422572072 ) ) ;
#81549=CARTESIAN_POINT ( 'NONE',  ( 0.1974969037888706092, -0.3420746716998660508, -0.9560367454068241511 ) ) ;
#81554=CARTESIAN_POINT ( 'NONE',  ( 0.1265901696524990294, -0.4724409448818896462, -1.345144356955380704 ) ) ;
#81555=CARTESIAN_POINT ( 'NONE',  ( -0.3996062992125986590, 0.1070741851644051862, -2.395013123359579943 ) ) ;
#81559=CARTESIAN_POINT ( 'NONE',  ( 0.1049643490035304799, -0.3917322834645670104, -0.7119615729996870979 ) ) ;
#81565=ADVANCED_FACE ( 'NONE', ( #2181 ), #1767, .T. ) ;
#81571=CARTESIAN_POINT ( 'NONE',  ( -0.2867679344610364334, -0.2867679344610367109, -0.8385826771653541734 ) ) ;
#81574=CARTESIAN_POINT ( 'NONE',  ( -0.3420746716998661618, 0.1974969037888702206, -1.601049868766404094 ) ) ;
#81581=CARTESIAN_POINT ( 'NONE',  ( -0.3996062992125986035, -7.340648628747425578E-17, 0.1181102362204724254 ) ) ;
#81588=CARTESIAN_POINT ( 'NONE',  ( -0.1958661417322836718, 0.3392501089628017219, 0.2171916010498686767 ) ) ;
#81594=CARTESIAN_POINT ( 'NONE',  ( -0.3460692066303958092, -0.1998031496062994683, -1.942257217847769057 ) ) ;
#81597=CARTESIAN_POINT ( 'NONE',  ( 0.3996062992125986035, -0.1070741851644052972, -1.605643044619422977 ) ) ;
#81601=CARTESIAN_POINT ( 'NONE',  ( -0.4724409448818898682, -8.678599364036362592E-17, -0.5118110236220472231 ) ) ;
#81603=DIRECTION ( 'NONE',  ( -0.000000000000000000, -0.000000000000000000, 1.000000000000000000 ) ) ;
#81604=CARTESIAN_POINT ( 'NONE',  ( -0.1049643490035307020, 0.3917322834645669549, 0.1587926509186352031 ) ) ;
#81611=CARTESIAN_POINT ( 'NONE',  ( -0.3458507752293909498, 0.3458507752293907833, -2.301181102362204633 ) ) ;
#81614=CARTESIAN_POINT ( 'NONE',  ( 0.2891555358219910499, -0.2891555358219909944, -2.222440944881889813 ) ) ;
#81627=CYLINDRICAL_SURFACE ( 'NONE', #72194, 0.4724409448818898682 ) ;
#81629=FACE_OUTER_BOUND ( 'NONE', #57535, .T. ) ;
#81637=CARTESIAN_POINT ( 'NONE',  ( -0.3996062992125984925, -0.1070741851644056858, -0.5951443569553805935 ) ) ;
#81639=CARTESIAN_POINT ( 'NONE',  ( 0.1049643490035304938, -0.3917322834645669549, -2.217191601049868677 ) ) ;
#81649=CARTESIAN_POINT ( 'NONE',  ( -0.2362204724409451284, 0.4091458600556402425, -2.609580052493438274 ) ) ;
#81655=CARTESIAN_POINT ( 'NONE',  ( -0.2867679344610365999, 0.2867679344610364889, -1.364173228346456268 ) ) ;
#81656=CARTESIAN_POINT ( 'NONE',  ( 0.08989863709126331981, 0.3814249188612193198, -1.220472440944881942 ) ) ;
#81660=CARTESIAN_POINT ( 'NONE',  ( -0.3996062992125985480, -7.340648628747423112E-17, -2.478346456692913868 ) ) ;
#81663=CARTESIAN_POINT ( 'NONE',  ( -0.1070741851644056997, 0.3996062992125986035, -0.9514435695538056015 ) ) ;
#81666=CARTESIAN_POINT ( 'NONE',  ( -0.3392501089628019995, 0.1958661417322832277, -2.695538057742782101 ) ) ;
#81676=CARTESIAN_POINT ( 'NONE',  ( -0.2867679344610366554, 0.2867679344610365444, -1.989481996554119059 ) ) ;
#81679=CARTESIAN_POINT ( 'NONE',  ( 0.1958661417322834775, 0.3392501089628018884, 0.02099737532808403431 ) ) ;
#81682=CARTESIAN_POINT ( 'NONE',  ( 0.3949938075777409408, 0.1058382717557500574, -0.1246719160104987345 ) ) ;
#81690=CARTESIAN_POINT ( 'NONE',  ( -0.2867679344610365444, -0.2867679344610367664, -1.158155798721471896 ) ) ;
#81692=CARTESIAN_POINT ( 'NONE',  ( -0.2867679344610365999, 0.2867679344610364889, -2.466535433070865757 ) ) ;
#81697=CARTESIAN_POINT ( 'NONE',  ( -0.1998031496062994683, 0.3460692066303958092, -0.8005249343832020470 ) ) ;
#81699=CARTESIAN_POINT ( 'NONE',  ( 0.3460692066303958092, 0.1998031496062993018, -0.3654855643044619407 ) ) ;
#81701=CARTESIAN_POINT ( 'NONE',  ( -0.1070741851644051862, -0.3996062992125987146, -2.434383202099737353 ) ) ;
#81706=CARTESIAN_POINT ( 'NONE',  ( -0.3458507752293906723, -0.3458507752293910609, -1.080708661417322691 ) ) ;
#81709=CARTESIAN_POINT ( 'NONE',  ( -0.1974969037888704149, -0.3420746716998661063, -0.9297900262467193588 ) ) ;
#81721=CARTESIAN_POINT ( 'NONE',  ( 0.3460692066303959202, -0.1998031496062991630, -1.756561679790026309 ) ) ;
#81723=CARTESIAN_POINT ( 'NONE',  ( 0.3917322834645669549, 0.1049643490035304660, -1.376640419947506189 ) ) ;
#81736=CARTESIAN_POINT ( 'NONE',  ( 0.3917322834645670104, 2.398668435337828261E-17, -1.147637795275590733 ) ) ;
#81752=CARTESIAN_POINT ( 'NONE',  ( -0.1998031496062994683, 0.3460692066303958092, -1.115485564304461885 ) ) ;
#81754=CARTESIAN_POINT ( 'NONE',  ( -9.594673741351313045E-17, 0.3917322834645670104, -2.039370078740157410 ) ) ;
#81758=CARTESIAN_POINT ( 'NONE',  ( -0.1265901696524986964, -0.4724409448818899238, -0.2296587926509186250 ) ) ;
#81759=CARTESIAN_POINT ( 'NONE',  ( 0.3949938075777411073, -0.1058382717557499464, -2.946194225721785909 ) ) ;
#81762=CARTESIAN_POINT ( 'NONE',  ( 0.3392501089628018884, -0.1958661417322834220, -1.356955380577427928 ) ) ;
#81764=CARTESIAN_POINT ( 'NONE',  ( 0.1265901696524989462, 0.4724409448818897572, -2.670603674540682260 ) ) ;
#81765=CARTESIAN_POINT ( 'NONE',  ( 0.1265901696524989184, 0.4724409448818898127, -0.8576115485564304031 ) ) ;
#81770=CARTESIAN_POINT ( 'NONE',  ( -0.1958661417322834497, -0.3392501089628018884, -0.7755712353992633146 ) ) ;
#81778=CARTESIAN_POINT ( 'NONE',  ( -0.3917322834645670104, -0.1049643490035307020, -2.247394643865828545 ) ) ;
#81784=CARTESIAN_POINT ( 'NONE',  ( -0.3917322834645670104, -7.196005306013484475E-17, -1.541338582677165503 ) ) ;
#81794=CARTESIAN_POINT ( 'NONE',  ( 0.1958661417322834775, 0.3392501089628018884, -2.656167979002624691 ) ) ;
#81801=CARTESIAN_POINT ( 'NONE',  ( -0.3917322834645670104, -7.196005306013484475E-17, -0.5964566929133858775 ) ) ;
#81802=CARTESIAN_POINT ( 'NONE',  ( 0.4091458600556404646, -0.2362204724409448231, 0.1332020997375328031 ) ) ;
#81803=CARTESIAN_POINT ( 'NONE',  ( -0.2925321140481930149, -0.2925321140481933480, -2.340551181102362488 ) ) ;
#81813=CARTESIAN_POINT ( 'NONE',  ( -0.3460692066303957537, -0.1998031496062994405, -0.2867454068241469534 ) ) ;
#81816=CARTESIAN_POINT ( 'NONE',  ( -0.1049643490035307020, 0.3917322834645669549, -0.1561679790026246351 ) ) ;
#81823=CARTESIAN_POINT ( 'NONE',  ( 0.1958661417322834497, 0.3392501089628018329, -1.799193282643357428 ) ) ;
#81832=CARTESIAN_POINT ( 'NONE',  ( 0.2867679344610366554, 0.2867679344610366554, -0.7644550113198971264 ) ) ;
#81836=CARTESIAN_POINT ( 'NONE',  ( -0.2362204724409451284, 0.4091458600556402425, -1.979658792650918597 ) ) ;
#81856=CARTESIAN_POINT ( 'NONE',  ( -0.2925321140481932369, 0.2925321140481931259, -2.458661417322834719 ) ) ;
#81861=CARTESIAN_POINT ( 'NONE',  ( -0.3996062992125987146, 0.1070741851644051862, -2.395013123359580387 ) ) ;
#81862=CARTESIAN_POINT ( 'NONE',  ( -9.674558042662121740E-17, 0.3949938075777409963, -1.574803149606299302 ) ) ;
#81863=CARTESIAN_POINT ( 'NONE',  ( -0.3460692066303960868, 0.1998031496062990242, -2.703412073490813583 ) ) ;
#81865=CARTESIAN_POINT ( 'NONE',  ( 0.3392501089628018329, 0.1958661417322835607, -0.5958005249343831800 ) ) ;
#81869=CARTESIAN_POINT ( 'NONE',  ( -0.1974969037888706924, 0.3420746716998658843, -2.452099737532808632 ) ) ;
#81873=CARTESIAN_POINT ( 'NONE',  ( 5.785732909357575061E-17, -0.4724409448818898682, -2.283464566929133799 ) ) ;
#81874=CARTESIAN_POINT ( 'NONE',  ( -0.3996062992125986035, -7.340648628747425578E-17, -2.086614173228346303 ) ) ;
#81881=CARTESIAN_POINT ( 'NONE',  ( -0.3392501089628017219, -0.1958661417322836718, 0.1778215223097112108 ) ) ;
#81888=CARTESIAN_POINT ( 'NONE',  ( 0.2867679344610365999, 0.2867679344610365999, -0.3799212598425197318 ) ) ;
#81889=CARTESIAN_POINT ( 'NONE',  ( -0.3392501089628017219, -0.1958661417322836718, -1.619422572178477848 ) ) ;
#81890=CARTESIAN_POINT ( 'NONE',  ( -0.3392501089628017219, -0.1958661417322836718, -2.091863517060367439 ) ) ;
#81893=CARTESIAN_POINT ( 'NONE',  ( 4.837279021331060870E-17, -0.3949938075777409963, -2.755905511811023167 ) ) ;
#81897=CARTESIAN_POINT ( 'NONE',  ( 0.2925321140481932369, -0.2925321140481932369, -1.358267716535433101 ) ) ;
#81900=CARTESIAN_POINT ( 'NONE',  ( 0.4724409448818898682, 2.892866454678787531E-17, -0.1948818897637795422 ) ) ;
#81902=CARTESIAN_POINT ( 'NONE',  ( 0.3917322834645669549, 0.1049643490035304660, -0.3667979002624672802 ) ) ;
#81907=CARTESIAN_POINT ( 'NONE',  ( 0.2867679344610365999, 0.2867679344610365999, -0.1299212598425196485 ) ) ;
#81912=CARTESIAN_POINT ( 'NONE',  ( 0.4091458600556404646, -0.2362204724409448231, -1.837270341207349000 ) ) ;
#81915=CARTESIAN_POINT ( 'NONE',  ( 0.4724409448818897017, 0.1265901696524990294, -0.9120734908136483021 ) ) ;
#81923=CARTESIAN_POINT ( 'NONE',  ( -0.2867679344610366554, 0.2867679344610365444, -0.5721591619084497315 ) ) ;
#81925=CARTESIAN_POINT ( 'NONE',  ( -0.1049643490035307020, 0.3917322834645669549, -1.036089238845144367 ) ) ;
#81930=CARTESIAN_POINT ( 'NONE',  ( -0.1049643490035307020, 0.3917322834645669549, -2.360892388451444113 ) ) ;
#81933=CARTESIAN_POINT ( 'NONE',  ( -0.4091458600556405756, 0.2362204724409446288, -0.7329396325459317518 ) ) ;
#81943=CARTESIAN_POINT ( 'NONE',  ( 4.893765752498283308E-17, -0.3996062992125985480, -2.045275590551181022 ) ) ;
#81951=CARTESIAN_POINT ( 'NONE',  ( 0.3460692066303959202, -0.1998031496062991630, -0.8116797900262466836 ) ) ;
#81952=CARTESIAN_POINT ( 'NONE',  ( -0.2925321140481930704, -0.2925321140481933480, -0.5314960629921260393 ) ) ;
#81953=CARTESIAN_POINT ( 'NONE',  ( -0.2891555358219911054, 0.2891555358219909388, -0.1771653543307087630 ) ) ;
#81959=CARTESIAN_POINT ( 'NONE',  ( -0.3420746716998662729, 0.1974969037888702206, -1.205380577427821454 ) ) ;
#81964=CARTESIAN_POINT ( 'NONE',  ( 0.4091458600556404646, -0.2362204724409448231, -1.049868766404199460 ) ) ;
#81965=CARTESIAN_POINT ( 'NONE',  ( 0.1998031496062992740, 0.3460692066303959757, -2.191601049868766360 ) ) ;
#81968=CARTESIAN_POINT ( 'NONE',  ( 0.3917322834645670659, -0.1049643490035303273, -0.7382082921597920011 ) ) ;
#81981=CARTESIAN_POINT ( 'NONE',  ( -0.1049643490035302024, -0.3917322834645671215, -0.8517060367454066805 ) ) ;
#81984=CARTESIAN_POINT ( 'NONE',  ( -0.2891555358219908833, -0.2891555358219912164, -1.318897637795275912 ) ) ;
#81996=CARTESIAN_POINT ( 'NONE',  ( 0.1049643490035304938, -0.3917322834645669549, 0.1450131233595799429 ) ) ;
#82002=CARTESIAN_POINT ( 'NONE',  ( -0.2925321140481932924, 0.2925321140481931814, -1.909448818897637512 ) ) ;
#82005=CARTESIAN_POINT ( 'NONE',  ( 0.1998031496062994128, -0.3460692066303957537, -1.428477690288713964 ) ) ;
#82009=CARTESIAN_POINT ( 'NONE',  ( -0.3458507752293909498, 0.3458507752293907833, -0.4921259842519684624 ) ) ;
#82012=CARTESIAN_POINT ( 'NONE',  ( -0.2867679344610365999, 0.2867679344610364889, -0.01181102362204719709 ) ) ;
#82018=CARTESIAN_POINT ( 'NONE',  ( 0.4724409448818897572, -0.1265901696524988906, -2.550524934383202158 ) ) ;
#82021=CARTESIAN_POINT ( 'NONE',  ( -0.1058382717557497660, -0.3949938075777411073, -2.353674540682414218 ) ) ;
#82032=CARTESIAN_POINT ( 'NONE',  ( 0.1265901696524989184, 0.4724409448818898127, -1.015091863517060267 ) ) ;
#82044=CARTESIAN_POINT ( 'NONE',  ( 0.1070741851644054776, -0.3996062992125984925, -0.7919947506561679784 ) ) ;
#82045=CARTESIAN_POINT ( 'NONE',  ( 0.3392501089628018884, -0.1958661417322834220, -2.394356955380577467 ) ) ;
#82054=CARTESIAN_POINT ( 'NONE',  ( 0.2362204724409449064, 0.4091458600556404646, -2.191601049868766360 ) ) ;
#82059=EDGE_CURVE ( 'NONE', #5054, #6583, #70722, .T. ) ;
#82061=CARTESIAN_POINT ( 'NONE',  ( -0.1958661417322834220, -0.3392501089628018884, -1.410104986876640654 ) ) ;
#82062=CARTESIAN_POINT ( 'NONE',  ( 0.2065800153021795649, 0.3330030935778863221, -1.220472440944882164 ) ) ;
#82066=CARTESIAN_POINT ( 'NONE',  ( -0.3996062992125986035, 0.1070741851644051584, -2.314304461942256808 ) ) ;
#82068=CARTESIAN_POINT ( 'NONE',  ( -0.3460692066303960868, 0.1998031496062990242, -0.8136482939632546652 ) ) ;
#82071=CARTESIAN_POINT ( 'NONE',  ( 0.3917322834645670104, 2.398668435337828261E-17, -2.472440944881889813 ) ) ;
#82083=CARTESIAN_POINT ( 'NONE',  ( -0.1958661417322834220, -0.3392501089628018884, -2.669947506561679784 ) ) ;
#82086=CARTESIAN_POINT ( 'NONE',  ( 0.1058382717557499880, 0.3949938075777411073, -0.1509186351706037210 ) ) ;
#82093=CARTESIAN_POINT ( 'NONE',  ( 0.2867679344610366554, 0.2867679344610366554, -1.551856586123046888 ) ) ;
#82095=CARTESIAN_POINT ( 'NONE',  ( 0.3392501089628018329, 0.1958661417322835607, -2.578083989501311901 ) ) ;
#82101=CARTESIAN_POINT ( 'NONE',  ( -0.3996062992125986035, -0.1070741851644056997, -0.9908136482939633449 ) ) ;
#82103=CARTESIAN_POINT ( 'NONE',  ( -0.3460692066303960313, 0.1998031496062989965, -0.2604986876640419946 ) ) ;
#82105=CARTESIAN_POINT ( 'NONE',  ( 0.2925321140481932369, -0.2925321140481932369, -2.303149606299212060 ) ) ;
#82106=CARTESIAN_POINT ( 'NONE',  ( 0.2867679344610365999, 0.2867679344610365999, -1.482283464566929387 ) ) ;
#82110=CARTESIAN_POINT ( 'NONE',  ( -0.4091458600556405756, 0.2362204724409446288, -1.047900262467191590 ) ) ;
#82113=CARTESIAN_POINT ( 'NONE',  ( 0.2891555358219910499, -0.2891555358219909944, -0.9625984251968502381 ) ) ;
#82125=CARTESIAN_POINT ( 'NONE',  ( 0.3996062992125985480, 2.446882876249141654E-17, -1.769685039370078927 ) ) ;
#82141=CARTESIAN_POINT ( 'NONE',  ( -9.594673741351313045E-17, 0.3917322834645670104, -1.029527559055118280 ) ) ;
#82157=CARTESIAN_POINT ( 'NONE',  ( -0.4724409448818898682, -8.678599364036362592E-17, -0.5118110236220472231 ) ) ;
#82161=CARTESIAN_POINT ( 'NONE',  ( 0.000000000000000000, 0.000000000000000000, -1.220472440944881942 ) ) ;
#82164=CARTESIAN_POINT ( 'NONE',  ( -0.1265901696524993347, 0.4724409448818895907, -0.4790026246719158998 ) ) ;
#82165=CARTESIAN_POINT ( 'NONE',  ( -0.1070741851644056997, 0.3996062992125986035, 0.1509186351706036100 ) ) ;
#82168=CARTESIAN_POINT ( 'NONE',  ( 0.3917322834645670104, 2.398668435337828261E-17, -1.527559055118110409 ) ) ;
#82170=CARTESIAN_POINT ( 'NONE',  ( 5.785732909357575061E-17, -0.4724409448818898682, -2.283464566929133799 ) ) ;
#82177=CARTESIAN_POINT ( 'NONE',  ( 0.3392501089628018329, -0.1958661417322834497, -0.6574609991787909724 ) ) ;
#82184=CARTESIAN_POINT ( 'NONE',  ( 0.3917322834645670659, 2.398668435337828261E-17, -2.004612491634857552 ) ) ;
#82191=CARTESIAN_POINT ( 'NONE',  ( 0.3392501089628018884, -0.1958661417322834220, -1.291994750656167978 ) ) ;
#82200=CARTESIAN_POINT ( 'NONE',  ( -0.3917322834645671215, 0.1049643490035301469, -2.702099737532808632 ) ) ;
#82207=CARTESIAN_POINT ( 'NONE',  ( 0.2867679344610365999, 0.2867679344610365999, -1.324803149606299302 ) ) ;
#82208=CARTESIAN_POINT ( 'NONE',  ( 0.3458507752293908943, 0.3458507752293908943, 0.1003937007874015769 ) ) ;
#82210=CARTESIAN_POINT ( 'NONE',  ( 0.2925321140481932369, 0.2925321140481932369, -2.734251968503936148 ) ) ;
#82220=CARTESIAN_POINT ( 'NONE',  ( 0.3460692066303958092, 0.1998031496062993018, -0.5229658792650918597 ) ) ;
#82222=CARTESIAN_POINT ( 'NONE',  ( -0.1958661417322836718, 0.3392501089628017219, -0.3202099737532808077 ) ) ;
#82238=CARTESIAN_POINT ( 'NONE',  ( -9.594673741351313045E-17, 0.3917322834645670659, -0.9416203656506056952 ) ) ;
#82242=CARTESIAN_POINT ( 'NONE',  ( 0.1265901696524990294, -0.4724409448818896462, -2.051837270341206665 ) ) ;
#82262=CARTESIAN_POINT ( 'NONE',  ( -9.787531504996566615E-17, 0.3996062992125985480, -2.596456692913385655 ) ) ;
#82267=CARTESIAN_POINT ( 'NONE',  ( -0.3460692066303960868, 0.1998031496062990242, -2.230971128608923770 ) ) ;
#82268=CARTESIAN_POINT ( 'NONE',  ( 0.3949938075777411073, -0.1058382717557499464, -1.686351706036745668 ) ) ;
#82269=CARTESIAN_POINT ( 'NONE',  ( -0.2925321140481932924, 0.2925321140481931814, -2.854330708661417138 ) ) ;
#82270=CARTESIAN_POINT ( 'NONE',  ( 0.4724409448818897017, 0.1265901696524990294, -2.486876640419947382 ) ) ;
#82271=CARTESIAN_POINT ( 'NONE',  ( 0.1958661417322836440, -0.3392501089628017219, -0.3989501312335957950 ) ) ;
#82275=CARTESIAN_POINT ( 'NONE',  ( -0.1974969037888706924, 0.3420746716998658843, -2.609580052493438718 ) ) ;
#82279=CARTESIAN_POINT ( 'NONE',  ( -0.1265901696524986964, -0.4724409448818899238, -2.749343832020996636 ) ) ;
#82280=CARTESIAN_POINT ( 'NONE',  ( 0.3996062992125986590, -0.1070741851644053111, -2.316272965879265122 ) ) ;
#82281=DIRECTION ( 'NONE',  ( 0.000000000000000000, 0.000000000000000000, 1.000000000000000000 ) ) ;
#82286=CARTESIAN_POINT ( 'NONE',  ( -0.3392501089628017219, -0.1958661417322836718, -0.2946194225721785465 ) ) ;
#82293=CARTESIAN_POINT ( 'NONE',  ( -0.2867679344610365999, 0.2867679344610364889, -0.4192913385826772532 ) ) ;
#82294=CARTESIAN_POINT ( 'NONE',  ( -0.1958661417322836718, 0.3392501089628017219, -1.580052493438320216 ) ) ;
#82295=CARTESIAN_POINT ( 'NONE',  ( 0.1958661417322836440, -0.3392501089628017219, -2.603674540682414218 ) ) ;
#82298=CARTESIAN_POINT ( 'NONE',  ( -0.1974969037888706647, 0.3420746716998658843, -2.690288713910760965 ) ) ;
#82302=CARTESIAN_POINT ( 'NONE',  ( -0.3996062992125987146, 0.1070741851644051862, -1.292650918635170454 ) ) ;
#82307=CARTESIAN_POINT ( 'NONE',  ( -0.3917322834645671215, 0.1049643490035301469, -0.2749343832020998413 ) ) ;
#82316=CARTESIAN_POINT ( 'NONE',  ( -0.1265901696524993347, 0.4724409448818895907, -2.053805774278214979 ) ) ;
#82324=CARTESIAN_POINT ( 'NONE',  ( 0.4091458600556404646, -0.2362204724409448231, -2.701443569553806157 ) ) ;
#82327=CARTESIAN_POINT ( 'NONE',  ( -0.3917322834645669549, -7.196005306013483243E-17, -0.5918442012785283257 ) ) ;
#82330=CARTESIAN_POINT ( 'NONE',  ( 0.1958661417322834775, 0.3392501089628018884, -0.8589238845144357981 ) ) ;
#82335=CARTESIAN_POINT ( 'NONE',  ( 0.1049643490035304938, -0.3917322834645669549, -2.754593175853017328 ) ) ;
#82338=CARTESIAN_POINT ( 'NONE',  ( -0.2362204724409447953, -0.4091458600556404646, -0.9297900262467192478 ) ) ;
#82345=CARTESIAN_POINT ( 'NONE',  ( 0.000000000000000000, 0.000000000000000000, -1.220472440944881942 ) ) ;
#82350=CARTESIAN_POINT ( 'NONE',  ( 0.3460692066303959202, -0.1998031496062991630, -2.071522309711285814 ) ) ;
#82351=( BOUNDED_SURFACE ( )  B_SPLINE_SURFACE ( 1, 2, ( 
 ( #32759, #6667, #58426, #32339, #58001, #365, #26021, #19714, #7517, #2031, #58854, #20972, #71487, #14674, #40331, #46631, #28112, #59676, #54182, #39493, #65180, #22213, #72327, #33185, #27697, #14259, #66846, #52520, #53361, #8759, #53766, #79071, #78650, #21387, #34434, #47456, #78228, #8348, #34850, #71908, #66010, #47042, #34014, #52937, #72735, #20561, #33598, #79477, #21793, #39917, #1211, #79895, #26861, #9179, #46213, #65606, #7937, #59263, #60513, #2454, #15081, #73150, #41157, #1620, #40739, #27276, #66423, #60100, #15499, #13834, #2861, #28524, #30590, #17566, #28934, #4922, #73984, #68081, #80312, #55834, #36904, #68489, #73574, #36488, #43199, #55011, #81542, #4091, #48700, #55422, #16330, #15920, #67256, #61754, #35258, #80720, #47870, #74398, #16742, #23034, #4504, #36083, #56256, #41567, #9589, #81952, #42382, #60922, #29760, #41974, #68894, #54603, #81129, #10828, #30171, #23446, #10425, #49110, #62164, #23861, #22627, #74816, #11245, #48288, #17161, #42794, #49528, #29352, #75221, #67667, #62580, #3273, #10004, #35669, #61333, #3687, #19191, #19609, #64233, #57484, #6149, #13312, #12894, #70123, #77279, #51576, #32239, #24678, #6568, #83177, #63810, #31823, #82360, #57897, #45271, #25497, #62994, #58320, #264, #38136, #31404, #69722, #51163, #12066, #25917, #12474, #37724, #50346, #70967, #43612, #38965, #64648, #6985, #30991, #76859, #44840, #76044, #32654, #24265, #70538, #5333, #49938, #75636, #38553, #57069, #63398, #17974, #5733, #69313, #11663, #82763, #18388, #37322, #56659, #44029, #25085, #50758, #76458, #18785, #44429, #8662, #52415, #71383, #66748, #52000, #79377, #33080, #77705, #20458, #20035, #47359, #14982, #20874, #59998, #53670, #45686, #72227, #13732, #14577, #78124, #34334, #9083, #7410, #7834, #34754, #21696, #65071, #41059, #26760, #46527, #58747, #2354, #73048, #21288, #26339, #72634, #15397, #33501, #28010, #40229, #1521, #8248, #46110, #39386, #1109, #65911, #71803, #59163, #683, #27175, #52838, #78549, #40641, #33913, #14156, #39812, #65502, #59577, #1934, #27597, #53256, #78968, #46942, #66323, #74300, #81037, #42703, #48605, #67570, #10329, #23349, #36396, #41474, #80627, #23765, #60823, #9902, #35991, #35573, #41876, #61661, #9488, #62071, #73476, #22531, #68400, #80215, #67159, #55328, #55740, #17066, #4002, #42286, #49436, #49020, #22938, #30077, #4409, #10739, #3174, #81448, #29667, #61236, #3591, #75130, #28424, #74717, #48193, #47775, #73889, #17475, #16646, #29256, #15826, #43106, #35162, #16229, #28838, #67984, #54501, #22115, #54920, #68802, #11148, #60414, #2765, #54084, #79799, #36806, #30495, #82671, #24173, #31726, #17881, #18695, #5235, #51478, #83081, #12797, #51066, #44337, #57798, #11564, #11973, #25818, #43516, #43934, #44745, #19096, #63714, #24987, #30899, #62482, #19512, #38039, #25403, #69215, #37223, #70440, #50662, #76766, #6054, #62900, #56566, #82267, #38453, #76362, #70028, #24585, #64139, #18289, #5642, #37628, #57390, #69628, #6472, #75541, #50252, #12381, #75949, #32142, #165, #63304, #31309, #77181, #45166, #56973, #70872, #4817, #81861, #56158, #49842, #1833, #33404, #77607, #8149, #8562, #27493, #59893, #2245, #53570, #26664, #21188, #20354, #66224, #72118, #46427, #78862, #19940, #584, #46842, #39283, #65816, #40130, #71701, #52319, #52737, #27911, #72536, #47256, #58218, #32555, #1421, #78025, #33814, #21594, #71283, #58643, #32976, #14477, #14884, #59479, #78447, #20773, #13631, #53150, #40544, #34231, #51900, #13221, #79279, #27077, #46005, #1011, #38869, #14055, #64548, #6885, #39710, #64970, #26239, #45590, #7306, #65401, #7738, #59066, #35056, #55222, #80929, #41372, #60314, #55632, #40958, #68300, #22012, #66640, #9386, #8977, #36291, #3900, #9797, #48914, #42598, #34650, #61133 ),
 ( #73788, #10636, #2663, #16542, #60722, #28322, #3072, #22836, #35469, #48088, #53983, #74615, #47672, #28738, #15716, #54820, #67053, #79695, #73367, #61965, #29560, #35887, #16124, #54399, #4304, #72945, #80111, #3485, #22429, #67882, #41770, #80524, #67463, #29967, #61557, #16959, #23244, #48495, #81341, #29151, #74196, #23656, #42187, #10220, #15297, #31618, #76256, #11872, #43409, #75028, #32038, #50553, #37935, #56049, #49737, #57280, #37524, #12278, #18591, #81758, #75437, #11456, #63612, #5539, #63198, #17776, #25296, #30796, #18185, #50146, #12692, #5949, #69522, #50962, #18992, #43003, #31204, #68697, #56871, #69108, #82977, #57697, #24068, #56462, #59, #44640, #30383, #6366, #37114, #82565, #62798, #76659, #38351, #69923, #17373, #70337, #64026, #82164, #49326, #24884, #75843, #44234, #5132, #11038, #36696, #62371, #4709, #24480, #43818, #52219, #77922, #909, #66859, #13951, #9601, #77076, #19410, #60934, #58542, #45061, #39609, #51796, #22225, #6779, #65298, #47469, #9190, #7636, #32874, #58968, #73161, #2873, #32451, #45902, #73587, #26134, #26565, #1325, #20253, #7203, #26974, #58113, #28536, #38766, #71182, #34862, #45485, #479, #21805, #47881, #60524, #52639, #33307, #15931, #15510, #71599, #79909, #54193, #41578, #77501, #67268, #79490, #41169, #35269, #19836, #25713, #51373, #70764, #64443, #13114, #13524, #39180, #64864, #48713, #42806, #74411, #36916, #74828, #16755, #29364, #62592, #22639, #49950, #43624, #81964, #10016, #42394, #68906, #11258, #55024, #73996, #69326, #54614, #24279, #35681, #80324, #23046, #48299, #68093, #36500, #36095, #4106, #75648, #16343, #30183, #10438, #41986, #61766, #62176, #49122, #29772, #67680, #4935, #61347, #55433, #80732, #68500, #81142, #3700, #23457, #17988, #17577, #49539, #17172, #10840, #56268, #3284, #4514, #55845, #81554, #23872, #75234, #43210, #30602, #11676, #37333, #28949, #77291, #70551, #695, #37737, #38150, #52012, #44042, #70135, #70979, #45284, #6580, #25511, #57081, #5345, #45699, #64245, #51590, #69735, #63411, #13324, #51176, #25931, #32251, #12079, #5746, #25098, #19622, #19204, #76872, #31417, #38977, #44442, #31836, #63822, #57912, #12486, #276, #18400, #82776, #44853, #50770, #12906, #38565, #6161, #57497, #64660, #26351, #76471, #18798, #6999, #24691, #83188, #32666, #58333, #77717, #20047, #71395, #13744, #63006, #31004, #56672, #82372, #50359, #76056, #46538, #9094, #14994, #72644, #21707, #20470, #26772, #73061, #65513, #8673, #66335, #14587, #78561, #78978, #28437, #15411, #73488, #1121, #58759, #27607, #52850, #34344, #47786, #14168, #1532, #59174, #7422, #2777, #53680, #59588, #41071, #34767, #33092, #53268, #52427, #21299, #7845, #47371, #22128, #46123, #72238, #39401, #60426, #71818, #79811, #33512, #1945, #39825, #66760, #54096, #60009, #65084, #28021, #78137, #40240, #27186, #46952, #65923, #40651, #20887, #8260, #33925, #2365, #79388, #48618, #15838, #42299, #67996, #74312, #55752, #4014, #81873, #67172, #9501, #49854, #16659, #35174, #29678, #41889, #11161, #80227, #55341, #36407, #81460, #81049, #22951, #49032, #62082, #75142, #22543, #36003, #62495, #16242, #10342, #74728, #61673, #80639, #17077, #48206, #17487, #28851, #61249, #23777, #35586, #73901, #10750, #36820, #49448, #42714, #23361, #4830, #4422, #68410, #68815, #43118, #30508, #67582, #56170, #30089, #24185, #41486, #9914, #60835, #3187, #54513, #3603, #29268, #54932, #6066, #82682, #37639, #31737, #63316, #25830, #63726, #5654, #18301, #51489, #11576, #38882, #32569, #70883, #82279, #31320, #57810, #177, #43945, #62914, #58231, #43530, #13232, #24597, #69229, #12393, #56578, #70452, #64561, #64150, #6898, #598, #26254, #56985, #77192, #24999, #45177, #51078, #25414, #19524, #50265, #5247, #75554, #69640, #44756, #19108 ) ),
 .UNSPECIFIED., .F., .F., .F. ) 
 B_SPLINE_SURFACE_WITH_KNOTS ( ( 2, 2 ),
 ( 3, 2, 2, 2, 2, 2, 2, 2, 2, 2, 2, 2, 2, 2, 2, 2, 2, 2, 2, 2, 2, 2, 2, 2, 2, 2, 2, 2, 2, 2, 2, 2, 2, 2, 2, 2, 2, 2, 2, 2, 2, 2, 2, 2, 2, 2, 2, 2, 2, 2, 2, 2, 2, 2, 2, 2, 2, 2, 2, 2, 2, 2, 2, 2, 2, 2, 2, 2, 2, 2, 2, 2, 2, 2, 2, 2, 2, 2, 2, 2, 2, 2, 2, 2, 2, 2, 2, 2, 2, 2, 2, 2, 2, 2, 2, 2, 2, 2, 2, 2, 2, 2, 2, 2, 2, 2, 2, 2, 2, 2, 2, 2, 2, 2, 2, 2, 2, 2, 2, 2, 2, 2, 2, 2, 2, 2, 2, 2, 2, 2, 2, 2, 2, 2, 2, 2, 2, 2, 2, 2, 2, 2, 2, 2, 2, 2, 2, 2, 2, 2, 2, 2, 2, 2, 2, 2, 2, 2, 2, 2, 2, 2, 2, 2, 2, 2, 2, 2, 2, 2, 2, 2, 2, 2, 2, 2, 2, 2, 2, 2, 2, 2, 2, 2, 2, 2, 2, 2, 2, 2, 2, 2, 2, 2, 2, 2, 2, 2, 2, 2, 2, 2, 2, 2, 2, 2, 2, 2, 2, 2, 2, 2, 2, 2, 2, 2, 2, 2, 2, 2, 2, 2, 2, 2, 2, 2, 2, 2, 2, 2, 2, 2, 2, 2, 2, 2, 2, 3 ),
 ( 0.000000000000000000, 1.000000000000000000 ),
 ( 0.000000000000000000, 0.004166666666666666609, 0.008333333333333333218, 0.01250000000000000069, 0.01666666666666666644, 0.02083333333333333218, 0.02500000000000000139, 0.02916666666666666713, 0.03333333333333333287, 0.03749999999999999861, 0.04166666666666666435, 0.04583333333333333010, 0.05000000000000000278, 0.05416666666666666852, 0.05833333333333333426, 0.06250000000000000000, 0.06666666666666666574, 0.07083333333333333148, 0.07499999999999999722, 0.07916666666666666297, 0.08333333333333332871, 0.08749999999999999445, 0.09166666666666666019, 0.09583333333333333981, 0.1000000000000000056, 0.1041666666666666713, 0.1083333333333333370, 0.1125000000000000028, 0.1166666666666666685, 0.1208333333333333343, 0.1250000000000000000, 0.1291666666666666796, 0.1333333333333333315, 0.1375000000000000111, 0.1416666666666666630, 0.1458333333333333426, 0.1499999999999999944, 0.1541666666666666741, 0.1583333333333333259, 0.1625000000000000056, 0.1666666666666666574, 0.1708333333333333370, 0.1749999999999999889, 0.1791666666666666685, 0.1833333333333333204, 0.1875000000000000000, 0.1916666666666666796, 0.1958333333333333315, 0.2000000000000000111, 0.2041666666666666630, 0.2083333333333333426, 0.2124999999999999944, 0.2166666666666666741, 0.2208333333333333259, 0.2250000000000000056, 0.2291666666666666574, 0.2333333333333333370, 0.2374999999999999889, 0.2416666666666666685, 0.2458333333333333204, 0.2500000000000000000, 0.2541666666666666519, 0.2583333333333333592, 0.2625000000000000111, 0.2666666666666666630, 0.2708333333333333148, 0.2750000000000000222, 0.2791666666666666741, 0.2833333333333333259, 0.2874999999999999778, 0.2916666666666666852, 0.2958333333333333370, 0.2999999999999999889, 0.3041666666666666408, 0.3083333333333333481, 0.3125000000000000000, 0.3166666666666666519, 0.3208333333333333592, 0.3250000000000000111, 0.3291666666666666630, 0.3333333333333333148, 0.3375000000000000222, 0.3416666666666666741, 0.3458333333333333259, 0.3499999999999999778, 0.3541666666666666852, 0.3583333333333333370, 0.3624999999999999889, 0.3666666666666666408, 0.3708333333333333481, 0.3750000000000000000, 0.3791666666666666519, 0.3833333333333333592, 0.3875000000000000111, 0.3916666666666666630, 0.3958333333333333148, 0.4000000000000000222, 0.4041666666666666741, 0.4083333333333333259, 0.4124999999999999778, 0.4166666666666666852, 0.4208333333333333370, 0.4249999999999999889, 0.4291666666666666408, 0.4333333333333333481, 0.4375000000000000000, 0.4416666666666666519, 0.4458333333333333592, 0.4500000000000000111, 0.4541666666666666630, 0.4583333333333333148, 0.4625000000000000222, 0.4666666666666666741, 0.4708333333333333259, 0.4749999999999999778, 0.4791666666666666852, 0.4833333333333333370, 0.4874999999999999889, 0.4916666666666666408, 0.4958333333333333481, 0.5000000000000000000, 0.5041666666666666519, 0.5083333333333333037, 0.5124999999999999556, 0.5166666666666667185, 0.5208333333333333703, 0.5250000000000000222, 0.5291666666666666741, 0.5333333333333333259, 0.5374999999999999778, 0.5416666666666666297, 0.5458333333333332815, 0.5500000000000000444, 0.5541666666666666963, 0.5583333333333333481, 0.5625000000000000000, 0.5666666666666666519, 0.5708333333333333037, 0.5749999999999999556, 0.5791666666666667185, 0.5833333333333333703, 0.5875000000000000222, 0.5916666666666666741, 0.5958333333333333259, 0.5999999999999999778, 0.6041666666666666297, 0.6083333333333332815, 0.6125000000000000444, 0.6166666666666666963, 0.6208333333333333481, 0.6250000000000000000, 0.6291666666666666519, 0.6333333333333333037, 0.6374999999999999556, 0.6416666666666667185, 0.6458333333333333703, 0.6500000000000000222, 0.6541666666666666741, 0.6583333333333333259, 0.6624999999999999778, 0.6666666666666666297, 0.6708333333333332815, 0.6750000000000000444, 0.6791666666666666963, 0.6833333333333333481, 0.6875000000000000000, 0.6916666666666666519, 0.6958333333333333037, 0.6999999999999999556, 0.7041666666666667185, 0.7083333333333333703, 0.7125000000000000222, 0.7166666666666666741, 0.7208333333333333259, 0.7249999999999999778, 0.7291666666666666297, 0.7333333333333332815, 0.7375000000000000444, 0.7416666666666666963, 0.7458333333333333481, 0.7500000000000000000, 0.7541666666666666519, 0.7583333333333333037, 0.7624999999999999556, 0.7666666666666667185, 0.7708333333333333703, 0.7750000000000000222, 0.7791666666666666741, 0.7833333333333333259, 0.7874999999999999778, 0.7916666666666666297, 0.7958333333333332815, 0.8000000000000000444, 0.8041666666666666963, 0.8083333333333333481, 0.8125000000000000000, 0.8166666666666666519, 0.8208333333333333037, 0.8249999999999999556, 0.8291666666666667185, 0.8333333333333333703, 0.8375000000000000222, 0.8416666666666666741, 0.8458333333333333259, 0.8499999999999999778, 0.8541666666666666297, 0.8583333333333332815, 0.8625000000000000444, 0.8666666666666666963, 0.8708333333333333481, 0.8750000000000000000, 0.8791666666666666519, 0.8833333333333333037, 0.8874999999999999556, 0.8916666666666667185, 0.8958333333333333703, 0.9000000000000000222, 0.9041666666666666741, 0.9083333333333333259, 0.9124999999999999778, 0.9166666666666666297, 0.9208333333333332815, 0.9250000000000000444, 0.9291666666666666963, 0.9333333333333333481, 0.9375000000000000000, 0.9416666666666666519, 0.9458333333333333037, 0.9499999999999999556, 0.9541666666666667185, 0.9583333333333333703, 0.9625000000000000222, 0.9666666666666666741, 0.9708333333333333259, 0.9749999999999999778, 0.9791666666666666297, 0.9833333333333332815, 0.9875000000000000444 ),
 .UNSPECIFIED. ) 
 GEOMETRIC_REPRESENTATION_ITEM ( )  RATIONAL_B_SPLINE_SURFACE ( (
 ( 1.000000000000000000, 0.9659258262890683122, 1.000000000000000000, 0.9659258262890683122, 1.000000000000000000, 0.9659258262890683122, 1.000000000000000000, 0.9659258262890683122, 1.000000000000000000, 0.9659258262890683122, 1.000000000000000000, 0.9659258262890683122, 1.000000000000000000, 0.9659258262890683122, 1.000000000000000000, 0.9659258262890683122, 1.000000000000000000, 0.9659258262890683122, 1.000000000000000000, 0.9659258262890683122, 1.000000000000000000, 0.9659258262890683122, 1.000000000000000000, 0.9659258262890683122, 1.000000000000000000, 0.9659258262890683122, 1.000000000000000000, 0.9659258262890683122, 1.000000000000000000, 0.9659258262890683122, 1.000000000000000000, 0.9659258262890683122, 1.000000000000000000, 0.9659258262890683122, 1.000000000000000000, 0.9659258262890683122, 1.000000000000000000, 0.9659258262890683122, 1.000000000000000000, 0.9659258262890683122, 1.000000000000000000, 0.9659258262890683122, 1.000000000000000000, 0.9659258262890683122, 1.000000000000000000, 0.9659258262890683122, 1.000000000000000000, 0.9659258262890683122, 1.000000000000000000, 0.9659258262890683122, 1.000000000000000000, 0.9659258262890683122, 1.000000000000000000, 0.9659258262890683122, 1.000000000000000000, 0.9659258262890683122, 1.000000000000000000, 0.9659258262890683122, 1.000000000000000000, 0.9659258262890683122, 1.000000000000000000, 0.9659258262890683122, 1.000000000000000000, 0.9659258262890683122, 1.000000000000000000, 0.9659258262890683122, 1.000000000000000000, 0.9659258262890683122, 1.000000000000000000, 0.9659258262890683122, 1.000000000000000000, 0.9659258262890683122, 1.000000000000000000, 0.9659258262890683122, 1.000000000000000000, 0.9659258262890683122, 1.000000000000000000, 0.9659258262890683122, 1.000000000000000000, 0.9659258262890683122, 1.000000000000000000, 0.9659258262890683122, 1.000000000000000000, 0.9659258262890683122, 1.000000000000000000, 0.9659258262890683122, 1.000000000000000000, 0.9659258262890683122, 1.000000000000000000, 0.9659258262890683122, 1.000000000000000000, 0.9659258262890683122, 1.000000000000000000, 0.9659258262890683122, 1.000000000000000000, 0.9659258262890683122, 1.000000000000000000, 0.9659258262890683122, 1.000000000000000000, 0.9659258262890683122, 1.000000000000000000, 0.9659258262890683122, 1.000000000000000000, 0.9659258262890683122, 1.000000000000000000, 0.9659258262890683122, 1.000000000000000000, 0.9659258262890683122, 1.000000000000000000, 0.9659258262890683122, 1.000000000000000000, 0.9659258262890683122, 1.000000000000000000, 0.9659258262890683122, 1.000000000000000000, 0.9659258262890683122, 1.000000000000000000, 0.9659258262890683122, 1.000000000000000000, 0.9659258262890683122, 1.000000000000000000, 0.9659258262890683122, 1.000000000000000000, 0.9659258262890683122, 1.000000000000000000, 0.9659258262890683122, 1.000000000000000000, 0.9659258262890683122, 1.000000000000000000, 0.9659258262890683122, 1.000000000000000000, 0.9659258262890683122, 1.000000000000000000, 0.9659258262890683122, 1.000000000000000000, 0.9659258262890683122, 1.000000000000000000, 0.9659258262890683122, 1.000000000000000000, 0.9659258262890683122, 1.000000000000000000, 0.9659258262890683122, 1.000000000000000000, 0.9659258262890683122, 1.000000000000000000, 0.9659258262890683122, 1.000000000000000000, 0.9659258262890683122, 1.000000000000000000, 0.9659258262890683122, 1.000000000000000000, 0.9659258262890683122, 1.000000000000000000, 0.9659258262890683122, 1.000000000000000000, 0.9659258262890683122, 1.000000000000000000, 0.9659258262890683122, 1.000000000000000000, 0.9659258262890683122, 1.000000000000000000, 0.9659258262890683122, 1.000000000000000000, 0.9659258262890683122, 1.000000000000000000, 0.9659258262890683122, 1.000000000000000000, 0.9659258262890683122, 1.000000000000000000, 0.9659258262890683122, 1.000000000000000000, 0.9659258262890683122, 1.000000000000000000, 0.9659258262890683122, 1.000000000000000000, 0.9659258262890683122, 1.000000000000000000, 0.9659258262890683122, 1.000000000000000000, 0.9659258262890683122, 1.000000000000000000, 0.9659258262890683122, 1.000000000000000000, 0.9659258262890683122, 1.000000000000000000, 0.9659258262890683122, 1.000000000000000000, 0.9659258262890683122, 1.000000000000000000, 0.9659258262890683122, 1.000000000000000000, 0.9659258262890683122, 1.000000000000000000, 0.9659258262890683122, 1.000000000000000000, 0.9659258262890683122, 1.000000000000000000, 0.9659258262890683122, 1.000000000000000000, 0.9659258262890683122, 1.000000000000000000, 0.9659258262890683122, 1.000000000000000000, 0.9659258262890683122, 1.000000000000000000, 0.9659258262890683122, 1.000000000000000000, 0.9659258262890683122, 1.000000000000000000, 0.9659258262890683122, 1.000000000000000000, 0.9659258262890683122, 1.000000000000000000, 0.9659258262890683122, 1.000000000000000000, 0.9659258262890683122, 1.000000000000000000, 0.9659258262890683122, 1.000000000000000000, 0.9659258262890683122, 1.000000000000000000, 0.9659258262890683122, 1.000000000000000000, 0.9659258262890683122, 1.000000000000000000, 0.9659258262890683122, 1.000000000000000000, 0.9659258262890683122, 1.000000000000000000, 0.9659258262890683122, 1.000000000000000000, 0.9659258262890683122, 1.000000000000000000, 0.9659258262890683122, 1.000000000000000000, 0.9659258262890683122, 1.000000000000000000, 0.9659258262890683122, 1.000000000000000000, 0.9659258262890683122, 1.000000000000000000, 0.9659258262890683122, 1.000000000000000000, 0.9659258262890683122, 1.000000000000000000, 0.9659258262890683122, 1.000000000000000000, 0.9659258262890683122, 1.000000000000000000, 0.9659258262890683122, 1.000000000000000000, 0.9659258262890683122, 1.000000000000000000, 0.9659258262890683122, 1.000000000000000000, 0.9659258262890683122, 1.000000000000000000, 0.9659258262890683122, 1.000000000000000000, 0.9659258262890683122, 1.000000000000000000, 0.9659258262890683122, 1.000000000000000000, 0.9659258262890683122, 1.000000000000000000, 0.9659258262890683122, 1.000000000000000000, 0.9659258262890683122, 1.000000000000000000, 0.9659258262890683122, 1.000000000000000000, 0.9659258262890683122, 1.000000000000000000, 0.9659258262890683122, 1.000000000000000000, 0.9659258262890683122, 1.000000000000000000, 0.9659258262890683122, 1.000000000000000000, 0.9659258262890683122, 1.000000000000000000, 0.9659258262890683122, 1.000000000000000000, 0.9659258262890683122, 1.000000000000000000, 0.9659258262890683122, 1.000000000000000000, 0.9659258262890683122, 1.000000000000000000, 0.9659258262890683122, 1.000000000000000000, 0.9659258262890683122, 1.000000000000000000, 0.9659258262890683122, 1.000000000000000000, 0.9659258262890683122, 1.000000000000000000, 0.9659258262890683122, 1.000000000000000000, 0.9659258262890683122, 1.000000000000000000, 0.9659258262890683122, 1.000000000000000000, 0.9659258262890683122, 1.000000000000000000, 0.9659258262890683122, 1.000000000000000000, 0.9659258262890683122, 1.000000000000000000, 0.9659258262890683122, 1.000000000000000000, 0.9659258262890683122, 1.000000000000000000, 0.9659258262890683122, 1.000000000000000000, 0.9659258262890683122, 1.000000000000000000, 0.9659258262890683122, 1.000000000000000000, 0.9659258262890683122, 1.000000000000000000, 0.9659258262890683122, 1.000000000000000000, 0.9659258262890683122, 1.000000000000000000, 0.9659258262890683122, 1.000000000000000000, 0.9659258262890683122, 1.000000000000000000, 0.9659258262890683122, 1.000000000000000000, 0.9659258262890683122, 1.000000000000000000, 0.9659258262890683122, 1.000000000000000000, 0.9659258262890683122, 1.000000000000000000, 0.9659258262890683122, 1.000000000000000000, 0.9659258262890683122, 1.000000000000000000, 0.9659258262890683122, 1.000000000000000000, 0.9659258262890683122, 1.000000000000000000, 0.9659258262890683122, 1.000000000000000000, 0.9659258262890683122, 1.000000000000000000, 0.9659258262890683122, 1.000000000000000000, 0.9659258262890683122, 1.000000000000000000, 0.9659258262890683122, 1.000000000000000000, 0.9659258262890683122, 1.000000000000000000, 0.9659258262890683122, 1.000000000000000000, 0.9659258262890683122, 1.000000000000000000, 0.9659258262890683122, 1.000000000000000000, 0.9659258262890683122, 1.000000000000000000, 0.9659258262890683122, 1.000000000000000000, 0.9659258262890683122, 1.000000000000000000, 0.9659258262890683122, 1.000000000000000000, 0.9659258262890683122, 1.000000000000000000, 0.9659258262890683122, 1.000000000000000000, 0.9659258262890683122, 1.000000000000000000, 0.9659258262890683122, 1.000000000000000000, 0.9659258262890683122, 1.000000000000000000, 0.9659258262890683122, 1.000000000000000000, 0.9659258262890683122, 1.000000000000000000, 0.9659258262890683122, 1.000000000000000000, 0.9659258262890683122, 1.000000000000000000, 0.9659258262890683122, 1.000000000000000000, 0.9659258262890683122, 1.000000000000000000, 0.9659258262890683122, 1.000000000000000000, 0.9659258262890683122, 1.000000000000000000, 0.9659258262890683122, 1.000000000000000000, 0.9659258262890683122, 1.000000000000000000, 0.9659258262890683122, 1.000000000000000000, 0.9659258262890683122, 1.000000000000000000, 0.9659258262890683122, 1.000000000000000000, 0.9659258262890683122, 1.000000000000000000, 0.9659258262890683122, 1.000000000000000000, 0.9659258262890683122, 1.000000000000000000, 0.9659258262890683122, 1.000000000000000000, 0.9659258262890683122, 1.000000000000000000, 0.9659258262890683122, 1.000000000000000000, 0.9659258262890683122, 1.000000000000000000, 0.9659258262890683122, 1.000000000000000000, 0.9659258262890683122, 1.000000000000000000, 0.9659258262890683122, 1.000000000000000000, 0.9659258262890683122, 1.000000000000000000, 0.9659258262890683122, 1.000000000000000000, 0.9659258262890683122, 1.000000000000000000, 0.9659258262890683122, 1.000000000000000000, 0.9659258262890683122, 1.000000000000000000, 0.9659258262890683122, 1.000000000000000000, 0.9659258262890683122, 1.000000000000000000, 0.9659258262890683122, 1.000000000000000000, 0.9659258262890683122, 1.000000000000000000, 0.9659258262890683122, 1.000000000000000000, 0.9659258262890683122, 1.000000000000000000, 0.9659258262890683122, 1.000000000000000000, 0.9659258262890683122, 1.000000000000000000, 0.9659258262890683122, 1.000000000000000000, 0.9659258262890683122, 1.000000000000000000, 0.9659258262890683122, 1.000000000000000000, 0.9659258262890683122, 1.000000000000000000, 0.9659258262890683122, 1.000000000000000000, 0.9659258262890683122, 1.000000000000000000, 0.9659258262890683122, 1.000000000000000000, 0.9659258262890683122, 1.000000000000000000, 0.9659258262890683122, 1.000000000000000000, 0.9659258262890683122, 1.000000000000000000, 0.9659258262890683122, 1.000000000000000000),
 ( 1.000000000000000000, 0.9659258262890683122, 1.000000000000000000, 0.9659258262890683122, 1.000000000000000000, 0.9659258262890683122, 1.000000000000000000, 0.9659258262890683122, 1.000000000000000000, 0.9659258262890683122, 1.000000000000000000, 0.9659258262890683122, 1.000000000000000000, 0.9659258262890683122, 1.000000000000000000, 0.9659258262890683122, 1.000000000000000000, 0.9659258262890683122, 1.000000000000000000, 0.9659258262890683122, 1.000000000000000000, 0.9659258262890683122, 1.000000000000000000, 0.9659258262890683122, 1.000000000000000000, 0.9659258262890683122, 1.000000000000000000, 0.9659258262890683122, 1.000000000000000000, 0.9659258262890683122, 1.000000000000000000, 0.9659258262890683122, 1.000000000000000000, 0.9659258262890683122, 1.000000000000000000, 0.9659258262890683122, 1.000000000000000000, 0.9659258262890683122, 1.000000000000000000, 0.9659258262890683122, 1.000000000000000000, 0.9659258262890683122, 1.000000000000000000, 0.9659258262890683122, 1.000000000000000000, 0.9659258262890683122, 1.000000000000000000, 0.9659258262890683122, 1.000000000000000000, 0.9659258262890683122, 1.000000000000000000, 0.9659258262890683122, 1.000000000000000000, 0.9659258262890683122, 1.000000000000000000, 0.9659258262890683122, 1.000000000000000000, 0.9659258262890683122, 1.000000000000000000, 0.9659258262890683122, 1.000000000000000000, 0.9659258262890683122, 1.000000000000000000, 0.9659258262890683122, 1.000000000000000000, 0.9659258262890683122, 1.000000000000000000, 0.9659258262890683122, 1.000000000000000000, 0.9659258262890683122, 1.000000000000000000, 0.9659258262890683122, 1.000000000000000000, 0.9659258262890683122, 1.000000000000000000, 0.9659258262890683122, 1.000000000000000000, 0.9659258262890683122, 1.000000000000000000, 0.9659258262890683122, 1.000000000000000000, 0.9659258262890683122, 1.000000000000000000, 0.9659258262890683122, 1.000000000000000000, 0.9659258262890683122, 1.000000000000000000, 0.9659258262890683122, 1.000000000000000000, 0.9659258262890683122, 1.000000000000000000, 0.9659258262890683122, 1.000000000000000000, 0.9659258262890683122, 1.000000000000000000, 0.9659258262890683122, 1.000000000000000000, 0.9659258262890683122, 1.000000000000000000, 0.9659258262890683122, 1.000000000000000000, 0.9659258262890683122, 1.000000000000000000, 0.9659258262890683122, 1.000000000000000000, 0.9659258262890683122, 1.000000000000000000, 0.9659258262890683122, 1.000000000000000000, 0.9659258262890683122, 1.000000000000000000, 0.9659258262890683122, 1.000000000000000000, 0.9659258262890683122, 1.000000000000000000, 0.9659258262890683122, 1.000000000000000000, 0.9659258262890683122, 1.000000000000000000, 0.9659258262890683122, 1.000000000000000000, 0.9659258262890683122, 1.000000000000000000, 0.9659258262890683122, 1.000000000000000000, 0.9659258262890683122, 1.000000000000000000, 0.9659258262890683122, 1.000000000000000000, 0.9659258262890683122, 1.000000000000000000, 0.9659258262890683122, 1.000000000000000000, 0.9659258262890683122, 1.000000000000000000, 0.9659258262890683122, 1.000000000000000000, 0.9659258262890683122, 1.000000000000000000, 0.9659258262890683122, 1.000000000000000000, 0.9659258262890683122, 1.000000000000000000, 0.9659258262890683122, 1.000000000000000000, 0.9659258262890683122, 1.000000000000000000, 0.9659258262890683122, 1.000000000000000000, 0.9659258262890683122, 1.000000000000000000, 0.9659258262890683122, 1.000000000000000000, 0.9659258262890683122, 1.000000000000000000, 0.9659258262890683122, 1.000000000000000000, 0.9659258262890683122, 1.000000000000000000, 0.9659258262890683122, 1.000000000000000000, 0.9659258262890683122, 1.000000000000000000, 0.9659258262890683122, 1.000000000000000000, 0.9659258262890683122, 1.000000000000000000, 0.9659258262890683122, 1.000000000000000000, 0.9659258262890683122, 1.000000000000000000, 0.9659258262890683122, 1.000000000000000000, 0.9659258262890683122, 1.000000000000000000, 0.9659258262890683122, 1.000000000000000000, 0.9659258262890683122, 1.000000000000000000, 0.9659258262890683122, 1.000000000000000000, 0.9659258262890683122, 1.000000000000000000, 0.9659258262890683122, 1.000000000000000000, 0.9659258262890683122, 1.000000000000000000, 0.9659258262890683122, 1.000000000000000000, 0.9659258262890683122, 1.000000000000000000, 0.9659258262890683122, 1.000000000000000000, 0.9659258262890683122, 1.000000000000000000, 0.9659258262890683122, 1.000000000000000000, 0.9659258262890683122, 1.000000000000000000, 0.9659258262890683122, 1.000000000000000000, 0.9659258262890683122, 1.000000000000000000, 0.9659258262890683122, 1.000000000000000000, 0.9659258262890683122, 1.000000000000000000, 0.9659258262890683122, 1.000000000000000000, 0.9659258262890683122, 1.000000000000000000, 0.9659258262890683122, 1.000000000000000000, 0.9659258262890683122, 1.000000000000000000, 0.9659258262890683122, 1.000000000000000000, 0.9659258262890683122, 1.000000000000000000, 0.9659258262890683122, 1.000000000000000000, 0.9659258262890683122, 1.000000000000000000, 0.9659258262890683122, 1.000000000000000000, 0.9659258262890683122, 1.000000000000000000, 0.9659258262890683122, 1.000000000000000000, 0.9659258262890683122, 1.000000000000000000, 0.9659258262890683122, 1.000000000000000000, 0.9659258262890683122, 1.000000000000000000, 0.9659258262890683122, 1.000000000000000000, 0.9659258262890683122, 1.000000000000000000, 0.9659258262890683122, 1.000000000000000000, 0.9659258262890683122, 1.000000000000000000, 0.9659258262890683122, 1.000000000000000000, 0.9659258262890683122, 1.000000000000000000, 0.9659258262890683122, 1.000000000000000000, 0.9659258262890683122, 1.000000000000000000, 0.9659258262890683122, 1.000000000000000000, 0.9659258262890683122, 1.000000000000000000, 0.9659258262890683122, 1.000000000000000000, 0.9659258262890683122, 1.000000000000000000, 0.9659258262890683122, 1.000000000000000000, 0.9659258262890683122, 1.000000000000000000, 0.9659258262890683122, 1.000000000000000000, 0.9659258262890683122, 1.000000000000000000, 0.9659258262890683122, 1.000000000000000000, 0.9659258262890683122, 1.000000000000000000, 0.9659258262890683122, 1.000000000000000000, 0.9659258262890683122, 1.000000000000000000, 0.9659258262890683122, 1.000000000000000000, 0.9659258262890683122, 1.000000000000000000, 0.9659258262890683122, 1.000000000000000000, 0.9659258262890683122, 1.000000000000000000, 0.9659258262890683122, 1.000000000000000000, 0.9659258262890683122, 1.000000000000000000, 0.9659258262890683122, 1.000000000000000000, 0.9659258262890683122, 1.000000000000000000, 0.9659258262890683122, 1.000000000000000000, 0.9659258262890683122, 1.000000000000000000, 0.9659258262890683122, 1.000000000000000000, 0.9659258262890683122, 1.000000000000000000, 0.9659258262890683122, 1.000000000000000000, 0.9659258262890683122, 1.000000000000000000, 0.9659258262890683122, 1.000000000000000000, 0.9659258262890683122, 1.000000000000000000, 0.9659258262890683122, 1.000000000000000000, 0.9659258262890683122, 1.000000000000000000, 0.9659258262890683122, 1.000000000000000000, 0.9659258262890683122, 1.000000000000000000, 0.9659258262890683122, 1.000000000000000000, 0.9659258262890683122, 1.000000000000000000, 0.9659258262890683122, 1.000000000000000000, 0.9659258262890683122, 1.000000000000000000, 0.9659258262890683122, 1.000000000000000000, 0.9659258262890683122, 1.000000000000000000, 0.9659258262890683122, 1.000000000000000000, 0.9659258262890683122, 1.000000000000000000, 0.9659258262890683122, 1.000000000000000000, 0.9659258262890683122, 1.000000000000000000, 0.9659258262890683122, 1.000000000000000000, 0.9659258262890683122, 1.000000000000000000, 0.9659258262890683122, 1.000000000000000000, 0.9659258262890683122, 1.000000000000000000, 0.9659258262890683122, 1.000000000000000000, 0.9659258262890683122, 1.000000000000000000, 0.9659258262890683122, 1.000000000000000000, 0.9659258262890683122, 1.000000000000000000, 0.9659258262890683122, 1.000000000000000000, 0.9659258262890683122, 1.000000000000000000, 0.9659258262890683122, 1.000000000000000000, 0.9659258262890683122, 1.000000000000000000, 0.9659258262890683122, 1.000000000000000000, 0.9659258262890683122, 1.000000000000000000, 0.9659258262890683122, 1.000000000000000000, 0.9659258262890683122, 1.000000000000000000, 0.9659258262890683122, 1.000000000000000000, 0.9659258262890683122, 1.000000000000000000, 0.9659258262890683122, 1.000000000000000000, 0.9659258262890683122, 1.000000000000000000, 0.9659258262890683122, 1.000000000000000000, 0.9659258262890683122, 1.000000000000000000, 0.9659258262890683122, 1.000000000000000000, 0.9659258262890683122, 1.000000000000000000, 0.9659258262890683122, 1.000000000000000000, 0.9659258262890683122, 1.000000000000000000, 0.9659258262890683122, 1.000000000000000000, 0.9659258262890683122, 1.000000000000000000, 0.9659258262890683122, 1.000000000000000000, 0.9659258262890683122, 1.000000000000000000, 0.9659258262890683122, 1.000000000000000000, 0.9659258262890683122, 1.000000000000000000, 0.9659258262890683122, 1.000000000000000000, 0.9659258262890683122, 1.000000000000000000, 0.9659258262890683122, 1.000000000000000000, 0.9659258262890683122, 1.000000000000000000, 0.9659258262890683122, 1.000000000000000000, 0.9659258262890683122, 1.000000000000000000, 0.9659258262890683122, 1.000000000000000000, 0.9659258262890683122, 1.000000000000000000, 0.9659258262890683122, 1.000000000000000000, 0.9659258262890683122, 1.000000000000000000, 0.9659258262890683122, 1.000000000000000000, 0.9659258262890683122, 1.000000000000000000, 0.9659258262890683122, 1.000000000000000000, 0.9659258262890683122, 1.000000000000000000, 0.9659258262890683122, 1.000000000000000000, 0.9659258262890683122, 1.000000000000000000, 0.9659258262890683122, 1.000000000000000000, 0.9659258262890683122, 1.000000000000000000, 0.9659258262890683122, 1.000000000000000000, 0.9659258262890683122, 1.000000000000000000, 0.9659258262890683122, 1.000000000000000000, 0.9659258262890683122, 1.000000000000000000, 0.9659258262890683122, 1.000000000000000000, 0.9659258262890683122, 1.000000000000000000, 0.9659258262890683122, 1.000000000000000000, 0.9659258262890683122, 1.000000000000000000, 0.9659258262890683122, 1.000000000000000000, 0.9659258262890683122, 1.000000000000000000, 0.9659258262890683122, 1.000000000000000000, 0.9659258262890683122, 1.000000000000000000, 0.9659258262890683122, 1.000000000000000000, 0.9659258262890683122, 1.000000000000000000, 0.9659258262890683122, 1.000000000000000000, 0.9659258262890683122, 1.000000000000000000, 0.9659258262890683122, 1.000000000000000000, 0.9659258262890683122, 1.000000000000000000, 0.9659258262890683122, 1.000000000000000000, 0.9659258262890683122, 1.000000000000000000) ) ) 
 REPRESENTATION_ITEM ( '' )  SURFACE ( )  );
#82359=CARTESIAN_POINT ( 'NONE',  ( 0.1998031496062992463, 0.3460692066303959202, -0.6935695538057742304 ) ) ;
#82360=CARTESIAN_POINT ( 'NONE',  ( -0.3460692066303958092, -0.1998031496062994683, -0.8398950131233595684 ) ) ;
#82361=CARTESIAN_POINT ( 'NONE',  ( 4.837279021331060870E-17, -0.3949938075777409963, -0.07874015748031501505 ) ) ;
#82367=CARTESIAN_POINT ( 'NONE',  ( 0.3420746716998660508, -0.1974969037888704149, -1.284120734908136718 ) ) ;
#82372=CARTESIAN_POINT ( 'NONE',  ( -0.2362204724409447953, -0.4091458600556404646, -1.797900262467191590 ) ) ;
#82387=CARTESIAN_POINT ( 'NONE',  ( 0.3392501089628018329, 0.1958661417322835607, -1.383202099737532942 ) ) ;
#82390=CARTESIAN_POINT ( 'NONE',  ( -0.3949938075777411628, 0.1058382717557497937, -1.450131233595800762 ) ) ;
#82391=ORIENTED_EDGE ( 'NONE', *, *, #55872, .T. ) ;
#82395=CARTESIAN_POINT ( 'NONE',  ( 0.2925321140481932369, 0.2925321140481932369, -0.1377952755905512139 ) ) ;
#82402=CARTESIAN_POINT ( 'NONE',  ( -9.594673741351313045E-17, 0.3917322834645670104, 0.2303149606299211838 ) ) ;
#82408=CARTESIAN_POINT ( 'NONE',  ( 0.1070741851644054915, -0.3996062992125986035, -2.132545931758530244 ) ) ;
#82411=CARTESIAN_POINT ( 'NONE',  ( -0.2925321140481932369, 0.2925321140481931259, -1.671259842519685179 ) ) ;
#82415=CARTESIAN_POINT ( 'NONE',  ( -0.4724409448818898682, -8.678599364036362592E-17, -0.9842519685039369248 ) ) ;
#82417=CARTESIAN_POINT ( 'NONE',  ( 0.3917322834645669549, 0.1049643490035304660, 0.04068241469816277767 ) ) ;
#82423=CARTESIAN_POINT ( 'NONE',  ( -0.1070741851644051862, -0.3996062992125986590, 0.1660104986876640154 ) ) ;
#82425=CARTESIAN_POINT ( 'NONE',  ( 0.3949938075777408852, 0.1058382717557500435, -2.406167979002624691 ) ) ;
#82439=AXIS2_PLACEMENT_3D ( 'NONE', #71168, #5934, #82963 ) ;
#82448=CARTESIAN_POINT ( 'NONE',  ( 0.2925321140481932369, -0.2925321140481931814, -0.6476377952755905110 ) ) ;
#82450=CARTESIAN_POINT ( 'NONE',  ( 0.2867679344610365999, -0.2867679344610365444, -2.072834645669291209 ) ) ;
#82465=CARTESIAN_POINT ( 'NONE',  ( 0.3917322834645669549, 0.1049643490035304660, -2.099081364829396446 ) ) ;
#82467=EDGE_CURVE ( 'NONE', #24385, #53683, #64824, .T. ) ;
#82470=CARTESIAN_POINT ( 'NONE',  ( -0.4724409448818898682, 5.785732909357575061E-17, -2.755905511811024056 ) ) ;
#82473=CARTESIAN_POINT ( 'NONE',  ( -0.1070741851644056997, 0.3996062992125986035, -1.108923884514435798 ) ) ;
#82475=CARTESIAN_POINT ( 'NONE',  ( 0.3917322834645670104, -0.1049643490035303411, -2.780839895013122565 ) ) ;
#82483=DIRECTION ( 'NONE',  ( 1.000000000000000000, 0.000000000000000000, 0.000000000000000000 ) ) ;
#82488=CARTESIAN_POINT ( 'NONE',  ( -0.3917322834645669549, -0.1049643490035306603, 0.1194225721784776956 ) ) ;
#82491=CARTESIAN_POINT ( 'NONE',  ( -0.3949938075777411628, 0.1058382717557497937, -0.1902887139107612702 ) ) ;
#82492=ORIENTED_EDGE ( 'NONE', *, *, #75384, .T. ) ;
#82494=CYLINDRICAL_SURFACE ( 'NONE', #46193, 0.4724409448818898682 ) ;
#82498=CARTESIAN_POINT ( 'NONE',  ( -0.1049643490035307158, 0.3917322834645670104, -1.735583620243781322 ) ) ;
#82500=CARTESIAN_POINT ( 'NONE',  ( 0.1958661417322836440, -0.3392501089628017219, -2.538713910761154491 ) ) ;
#82505=CARTESIAN_POINT ( 'NONE',  ( 0.2925321140481932369, 0.2925321140481932369, -0.9251968503937008093 ) ) ;
#82507=CARTESIAN_POINT ( 'NONE',  ( 0.1070741851644053388, 0.3996062992125986035, -0.3851706036745406458 ) ) ;
#82509=CARTESIAN_POINT ( 'NONE',  ( 0.3460692066303959202, 0.1998031496062993295, -2.335958005249343827 ) ) ;
#82510=CARTESIAN_POINT ( 'NONE',  ( 0.1958661417322836440, -0.3392501089628017219, -1.751312335958005395 ) ) ;
#82514=CARTESIAN_POINT ( 'NONE',  ( -0.4724409448818898682, -8.678599364036362592E-17, -1.218503937007874072 ) ) ;
#82517=CARTESIAN_POINT ( 'NONE',  ( -0.1974969037888706924, 0.3420746716998658843, -1.034776902887139194 ) ) ;
#82528=CARTESIAN_POINT ( 'NONE',  ( 0.1070741851644053388, 0.3996062992125986035, -1.802493438320210029 ) ) ;
#82543=CARTESIAN_POINT ( 'NONE',  ( -0.1049643490035302024, -0.3917322834645671215, -1.101706036745407014 ) ) ;
#82552=CARTESIAN_POINT ( 'NONE',  ( -0.2362204724409447953, -0.4091458600556404646, -2.585301837270341352 ) ) ;
#82562=CARTESIAN_POINT ( 'NONE',  ( -0.1958661417322834220, -0.3392501089628018884, -1.947506561679789971 ) ) ;
#82565=CARTESIAN_POINT ( 'NONE',  ( 0.4724409448818897572, -0.1265901696524988906, -0.4265091863517060933 ) ) ;
#82566=CARTESIAN_POINT ( 'NONE',  ( -0.1998031496062994683, 0.3460692066303958092, 0.1443569553805774119 ) ) ;
#82569=CARTESIAN_POINT ( 'NONE',  ( -0.3917322834645669549, -0.1049643490035306603, -1.455380577427821676 ) ) ;
#82578=CARTESIAN_POINT ( 'NONE',  ( 0.1049643490035304522, -0.3917322834645668994, -0.7952562747693419087 ) ) ;
#82585=CARTESIAN_POINT ( 'NONE',  ( 0.1958661417322836718, -0.3392501089628017219, -1.978365772474752537 ) ) ;
#82587=ORIENTED_EDGE ( 'NONE', *, *, #65801, .F. ) ;
#82593=CARTESIAN_POINT ( 'NONE',  ( -0.2867679344610364334, -0.2867679344610367109, -1.561023622047243986 ) ) ;
#82604=CARTESIAN_POINT ( 'NONE',  ( -9.594673741351313045E-17, 0.3917322834645670104, -2.826771653543306506 ) ) ;
#82611=CARTESIAN_POINT ( 'NONE',  ( 0.3917322834645670104, -0.1049643490035303411, -1.141076115485564202 ) ) ;
#82612=CARTESIAN_POINT ( 'NONE',  ( -0.4724409448818898682, -8.678599364036362592E-17, 0.04133858267716534335 ) ) ;
#82614=CARTESIAN_POINT ( 'NONE',  ( 0.1998031496062992463, 0.3460692066303959202, -2.740813648293963567 ) ) ;
#82625=CARTESIAN_POINT ( 'NONE',  ( 0.3996062992125985480, 2.446882876249141654E-17, -0.5098425196850393526 ) ) ;
#82627=CARTESIAN_POINT ( 'NONE',  ( 0.3392501089628018884, -0.1958661417322834220, -0.4120734908136482466 ) ) ;
#82642=CARTESIAN_POINT ( 'NONE',  ( 0.1958661417322836718, -0.3392501089628017219, -1.033483882710973134 ) ) ;
#82646=CARTESIAN_POINT ( 'NONE',  ( 0.4091458600556404646, -0.2362204724409448231, -2.543963254593176071 ) ) ;
#82665=CARTESIAN_POINT ( 'NONE',  ( -0.3460692066303958092, -0.1998031496062994683, -0.5249343832020997302 ) ) ;
#82666=CARTESIAN_POINT ( 'NONE',  ( -0.3996062992125984925, -0.1070741851644056858, -2.799868766404198794 ) ) ;
#82671=CARTESIAN_POINT ( 'NONE',  ( 0.3996062992125986035, 2.446882876249141962E-17, -2.007874015748031482 ) ) ;
#82672=CARTESIAN_POINT ( 'NONE',  ( 0.3949938075777409963, 2.418639510665530435E-17, -1.377952755905511584 ) ) ;
#82675=CARTESIAN_POINT ( 'NONE',  ( 4.797336870675656522E-17, -0.3917322834645670104, -0.5433070866141732624 ) ) ;
#82678=CARTESIAN_POINT ( 'NONE',  ( 0.2891555358219910499, 0.2891555358219910499, -2.734251968503936592 ) ) ;
#82682=CARTESIAN_POINT ( 'NONE',  ( 0.2362204724409449064, 0.4091458600556404646, -2.664041994750656173 ) ) ;
#82683=CARTESIAN_POINT ( 'NONE',  ( -9.787531504996567848E-17, 0.3996062992125986035, -2.047244094488188892 ) ) ;
#82690=CARTESIAN_POINT ( 'NONE',  ( -0.3917322834645669549, -0.1049643490035306603, -0.2880577427821523484 ) ) ;
#82697=CARTESIAN_POINT ( 'NONE',  ( -0.3917322834645670104, -7.196005306013484475E-17, -0.5964566929133858775 ) ) ;
#82698=CARTESIAN_POINT ( 'NONE',  ( -0.1049643490035307020, 0.3917322834645669549, -1.416010498687664043 ) ) ;
#82699=CARTESIAN_POINT ( 'NONE',  ( -0.3917322834645669549, -0.1049643490035306603, -2.715223097112861250 ) ) ;
#82700=VERTEX_POINT ( 'NONE', #31783 ) ;
#82701=CARTESIAN_POINT ( 'NONE',  ( 0.3996062992125986590, -0.1070741851644053111, 0.04593175853018371252 ) ) ;
#82705=CARTESIAN_POINT ( 'NONE',  ( -0.1070741851644056997, 0.3996062992125986035, -1.581364829396325389 ) ) ;
#82707=CARTESIAN_POINT ( 'NONE',  ( -0.2362204724409451284, 0.4091458600556402425, -2.452099737532808188 ) ) ;
#82710=CARTESIAN_POINT ( 'NONE',  ( -0.3392501089628017219, -0.1958661417322836718, -0.2946194225721785465 ) ) ;
#82719=CARTESIAN_POINT ( 'NONE',  ( 5.785732909357575061E-17, -0.4724409448818898682, -1.968503937007873850 ) ) ;
#82726=CARTESIAN_POINT ( 'NONE',  ( -0.2362204724409447953, -0.4091458600556404646, -2.270341207349081181 ) ) ;
#82730=CARTESIAN_POINT ( 'NONE',  ( -0.3917322834645669549, -7.196005306013483243E-17, -0.4343638863178984622 ) ) ;
#82732=CARTESIAN_POINT ( 'NONE',  ( 0.2867679344610366554, 0.2867679344610366554, -0.6948818897637795144 ) ) ;
#82737=CARTESIAN_POINT ( 'NONE',  ( -0.3917322834645671215, 0.1049643490035301469, -2.702099737532808632 ) ) ;
#82740=CARTESIAN_POINT ( 'NONE',  ( -0.3458507752293906723, -0.3458507752293910609, -1.395669291338582196 ) ) ;
#82751=CARTESIAN_POINT ( 'NONE',  ( 0.3996062992125986035, -0.1070741851644052972, -2.235564304461942431 ) ) ;
#82755=CARTESIAN_POINT ( 'NONE',  ( 0.3996062992125986035, -0.1070741851644052972, -1.290682414698162805 ) ) ;
#82762=CARTESIAN_POINT ( 'NONE',  ( -0.3996062992125984925, -0.1070741851644056719, -0.7526246719160104570 ) ) ;
#82763=CARTESIAN_POINT ( 'NONE',  ( 0.1998031496062992740, 0.3460692066303959757, -1.089238845144356871 ) ) ;
#82764=CARTESIAN_POINT ( 'NONE',  ( 0.3949938075777409408, 0.1058382717557500574, -0.4396325459317587114 ) ) ;
#82769=CARTESIAN_POINT ( 'NONE',  ( -0.4091458600556402980, -0.2362204724409451284, -2.333989501312335957 ) ) ;
#82770=CARTESIAN_POINT ( 'NONE',  ( 0.3949938075777409408, -0.1058382717557499186, -1.290682414698162583 ) ) ;
#82776=CARTESIAN_POINT ( 'NONE',  ( -0.1265901696524986964, -0.4724409448818899238, -1.646981627296587591 ) ) ;
#82777=CARTESIAN_POINT ( 'NONE',  ( 0.3996062992125986035, 2.446882876249141962E-17, -2.637795275590551380 ) ) ;
#82790=CARTESIAN_POINT ( 'NONE',  ( -0.3917322834645670104, -7.196005306013484475E-17, -1.448818897637795367 ) ) ;
#82793=CARTESIAN_POINT ( 'NONE',  ( 0.3949938075777411073, -0.1058382717557499464, -1.528871391076115804 ) ) ;
#82794=EDGE_LOOP ( 'NONE', ( #32591, #55452, #55771, #77525, #23795, #55125, #45738 ) ) ;
#82798=CARTESIAN_POINT ( 'NONE',  ( -0.3996062992125986035, -7.340648628747425578E-17, -0.1968503937007874127 ) ) ;
#82805=CARTESIAN_POINT ( 'NONE',  ( 0.2867679344610365999, 0.2867679344610365999, -0.06496062992125994917 ) ) ;
#82813=CARTESIAN_POINT ( 'NONE',  ( -0.1070741851644056997, 0.3996062992125984925, -1.500656167979002031 ) ) ;
#82818=CARTESIAN_POINT ( 'NONE',  ( 0.4091458600556404646, -0.2362204724409448231, -1.049868766404199460 ) ) ;
#82820=CARTESIAN_POINT ( 'NONE',  ( 0.1049643490035303689, 0.3917322834645670104, 0.01443569553805778768 ) ) ;
#82823=CARTESIAN_POINT ( 'NONE',  ( -0.2867679344610366554, 0.2867679344610365444, -2.151574803149606030 ) ) ;
#82829=CARTESIAN_POINT ( 'NONE',  ( -0.2362204724409447953, -0.4091458600556404646, -2.662073490813648746 ) ) ;
#82832=CARTESIAN_POINT ( 'NONE',  ( -0.3949938075777409963, -7.255918531996591613E-17, -2.163385826771653697 ) ) ;
#82856=CARTESIAN_POINT ( 'NONE',  ( -0.3460692066303960313, 0.1998031496062989965, -0.5754593175853018883 ) ) ;
#82857=CARTESIAN_POINT ( 'NONE',  ( -0.1958661417322836718, 0.3392501089628017219, -2.145013123359580387 ) ) ;
#82866=CARTESIAN_POINT ( 'NONE',  ( 0.1265901696524990572, -0.4724409448818897017, -0.7152230971128609172 ) ) ;
#82867=CARTESIAN_POINT ( 'NONE',  ( -0.1958661417322833942, -0.3392501089628018884, -2.267079683235907694 ) ) ;
#82872=CARTESIAN_POINT ( 'NONE',  ( 0.2867679344610365999, -0.2867679344610365444, -2.072834645669291209 ) ) ;
#82873=CARTESIAN_POINT ( 'NONE',  ( 0.1882840440723353992, 0.3436793299028297333, -1.220472440944881942 ) ) ;
#82878=AXIS2_PLACEMENT_3D ( 'NONE', #19476, #43888, #50616 ) ;
#82883=CARTESIAN_POINT ( 'NONE',  ( -0.2925321140481932924, 0.2925321140481931814, -1.122047244094488194 ) ) ;
#82885=CARTESIAN_POINT ( 'NONE',  ( -0.1049643490035302024, -0.3917322834645671215, -2.898950131233595684 ) ) ;
#82897=CARTESIAN_POINT ( 'NONE',  ( -9.594673741351313045E-17, 0.3917322834645670104, -0.1496062992125983815 ) ) ;
#82900=CARTESIAN_POINT ( 'NONE',  ( -0.1058382717557497937, -0.3949938075777411628, -0.07217847769028878924 ) ) ;
#82907=CARTESIAN_POINT ( 'NONE',  ( 0.1049643490035303967, 0.3917322834645670659, -1.879940575624358789 ) ) ;
#82909=CARTESIAN_POINT ( 'NONE',  ( 0.3917322834645669549, 0.1049643490035304660, -2.729002624671915900 ) ) ;
#82914=CARTESIAN_POINT ( 'NONE',  ( -9.787531504996567848E-17, 0.3996062992125986035, -0.7874015748031496509 ) ) ;
#82916=CARTESIAN_POINT ( 'NONE',  ( 0.1070741851644054776, -0.3996062992125984925, -0.4770341207349080848 ) ) ;
#82917=CARTESIAN_POINT ( 'NONE',  ( 0.3996062992125985480, 2.446882876249141654E-17, -0.1948818897637795700 ) ) ;
#82919=CARTESIAN_POINT ( 'NONE',  ( 0.1998031496062992740, 0.3460692066303959757, -2.664041994750656173 ) ) ;
#82920=CARTESIAN_POINT ( 'NONE',  ( -9.594673741351313045E-17, 0.3917322834645670104, -1.816929133858267820 ) ) ;
#82925=CARTESIAN_POINT ( 'NONE',  ( 0.3458507752293908943, 0.3458507752293908943, -1.316929133858267598 ) ) ;
#82928=CARTESIAN_POINT ( 'NONE',  ( 0.1974969037888704704, 0.3420746716998660508, -1.008530183727033958 ) ) ;
#82938=CARTESIAN_POINT ( 'NONE',  ( 0.3996062992125985480, 2.446882876249141654E-17, -2.242125984251968518 ) ) ;
#82955=CARTESIAN_POINT ( 'NONE',  ( 0.3917322834645669549, 0.1049643490035304660, -0.9967191601049870675 ) ) ;
#82958=CARTESIAN_POINT ( 'NONE',  ( 0.000000000000000000, 0.000000000000000000, -1.929133858267716661 ) ) ;
#82963=DIRECTION ( 'NONE',  ( 1.000000000000000000, 0.000000000000000000, 0.000000000000000000 ) ) ;
#82974=CARTESIAN_POINT ( 'NONE',  ( -0.2867679344610366554, 0.2867679344610365444, -2.059055118110236116 ) ) ;
#82977=CARTESIAN_POINT ( 'NONE',  ( -0.4091458600556402980, -0.2362204724409451284, -0.3674540682414698112 ) ) ;
#82978=CARTESIAN_POINT ( 'NONE',  ( -0.2891555358219908833, -0.2891555358219912164, -2.578740157480315265 ) ) ;
#82981=CARTESIAN_POINT ( 'NONE',  ( -0.2867679344610364334, -0.2867679344610367109, -1.311023622047244430 ) ) ;
#82983=CARTESIAN_POINT ( 'NONE',  ( -0.01150853369506071172, 0.3951562584566651326, -2.755905511811586273 ) ) ;
#82986=CARTESIAN_POINT ( 'NONE',  ( -1.157146581871515012E-16, 0.4724409448818898682, 0.000000000000000000 ) ) ;
#82990=CARTESIAN_POINT ( 'NONE',  ( 0.1958661417322834497, 0.3392501089628018329, -0.6968310779189482718 ) ) ;
#82997=CARTESIAN_POINT ( 'NONE',  ( -0.1049643490035307158, 0.3917322834645670104, -2.050544250165041493 ) ) ;
#83004=CARTESIAN_POINT ( 'NONE',  ( 0.1049643490035303689, 0.3917322834645670104, -1.337926509186352142 ) ) ;
#83009=CARTESIAN_POINT ( 'NONE',  ( -0.009627693921946872679, 0.3964540044758437243, 2.415985422253605141E-12 ) ) ;
#83013=CARTESIAN_POINT ( 'NONE',  ( -0.1958661417322834220, -0.3392501089628018884, -2.892388451443569153 ) ) ;
#83019=DIRECTION ( 'NONE',  ( 0.000000000000000000, -0.000000000000000000, 1.000000000000000000 ) ) ;
#83020=CARTESIAN_POINT ( 'NONE',  ( -0.3917322834645669549, -0.1049643490035306603, -1.232939632545931863 ) ) ;
#83021=CARTESIAN_POINT ( 'NONE',  ( 0.4091458600556403535, 0.2362204724409449896, -0.2080052493438320216 ) ) ;
#83024=CARTESIAN_POINT ( 'NONE',  ( -0.2925321140481930149, -0.2925321140481933480, -2.655511811023622215 ) ) ;
#83029=CARTESIAN_POINT ( 'NONE',  ( 0.3949938075777408852, 0.1058382717557500435, 0.1135170603674540979 ) ) ;
#83035=CARTESIAN_POINT ( 'NONE',  ( 0.3460692066303958092, 0.1998031496062993018, -0.3654855643044619407 ) ) ;
#83037=CARTESIAN_POINT ( 'NONE',  ( 0.3392501089628018884, -0.1958661417322834220, -0.09711286089238840846 ) ) ;
#83051=CARTESIAN_POINT ( 'NONE',  ( -0.1958661417322836995, 0.3392501089628017219, -0.7972634102700281167 ) ) ;
#83056=CARTESIAN_POINT ( 'NONE',  ( -0.1265901696524986964, -0.4724409448818899238, -2.353674540682414218 ) ) ;
#83075=CARTESIAN_POINT ( 'NONE',  ( -0.1998031496062994683, 0.3460692066303958092, -0.4855643044619422644 ) ) ;
#83076=CARTESIAN_POINT ( 'NONE',  ( 0.3460692066303959202, -0.1998031496062991630, -2.543963254593176071 ) ) ;
#83081=CARTESIAN_POINT ( 'NONE',  ( -0.1070741851644056997, 0.3996062992125986035, -2.053805774278214979 ) ) ;
#83082=CARTESIAN_POINT ( 'NONE',  ( 0.3949938075777409408, 0.1058382717557500574, -1.384514435695538337 ) ) ;
#83083=CARTESIAN_POINT ( 'NONE',  ( -0.3996062992125987146, 0.1070741851644051862, -2.867454068241469756 ) ) ;
#83085=CARTESIAN_POINT ( 'NONE',  ( -0.1958661417322834220, -0.3392501089628018884, -0.8451443569553805935 ) ) ;
#83088=CARTESIAN_POINT ( 'NONE',  ( -0.2891555358219911054, 0.2891555358219909388, -2.773622047244094446 ) ) ;
#83093=CARTESIAN_POINT ( 'NONE',  ( 0.2362204724409449064, 0.4091458600556404646, -0.06364829396325459576 ) ) ;
#83094=CARTESIAN_POINT ( 'NONE',  ( 4.893765752498283924E-17, -0.3996062992125986035, -1.968503937007873850 ) ) ;
#83102=CARTESIAN_POINT ( 'NONE',  ( 0.3917322834645670104, 2.398668435337828261E-17, -0.04527559055118119541 ) ) ;
#83110=CARTESIAN_POINT ( 'NONE',  ( -0.3917322834645671215, 0.1049643490035301469, -0.4324146981627298159 ) ) ;
#83111=CARTESIAN_POINT ( 'NONE',  ( 4.797336870675656522E-17, -0.3917322834645670104, -1.330708661417322691 ) ) ;
#83112=CARTESIAN_POINT ( 'NONE',  ( -0.1049643490035307020, 0.3917322834645669549, -2.675853018372703396 ) ) ;
#83115=CARTESIAN_POINT ( 'NONE',  ( -0.1998031496062991907, -0.3460692066303959757, 0.09186351706036742504 ) ) ;
#83116=EDGE_LOOP ( 'NONE', ( #39182, #57118, #28128, #49230 ) ) ;
#83119=CARTESIAN_POINT ( 'NONE',  ( 0.3996062992125986035, 2.446882876249141962E-17, -1.377952755905511806 ) ) ;
#83123=CARTESIAN_POINT ( 'NONE',  ( 0.1958661417322834775, 0.3392501089628018884, -0.7014435695538058235 ) ) ;
#83132=CARTESIAN_POINT ( 'NONE',  ( -0.4724409448818899238, 0.1265901696524986686, -2.080052493438320216 ) ) ;
#83142=CARTESIAN_POINT ( 'NONE',  ( 4.797336870675655290E-17, -0.3917322834645669549, -0.9461749099399457963 ) ) ;
#83143=B_SPLINE_CURVE_WITH_KNOTS ( 'NONE', 3,
 ( #68026, #60039, #60454, #55370, #41918, #10370, #36028, #67612, #48647, #9943, #35615, #61278, #2395, #61702, #41102, #3631, #79417, #29299 ),
 .UNSPECIFIED., .F., .F.,
 ( 4, 2, 2, 2, 2, 2, 2, 2, 4 ),
 ( 0.000000000000000000, 2.503579457949756240E-05, 5.007158915899512480E-05, 0.0001001431783179882574, 0.0002002863566359730724, 0.0004005727132719426212, 0.0008011454265438807971, 0.001602290853087756173, 0.003204581706175506708 ),
 .UNSPECIFIED. ) ;
#83145=CARTESIAN_POINT ( 'NONE',  ( -0.1049643490035307020, 0.3917322834645669549, -0.8786089238845143923 ) ) ;
#83150=CARTESIAN_POINT ( 'NONE',  ( -0.1049643490035307020, 0.3917322834645669549, -2.675853018372703396 ) ) ;
#83153=CARTESIAN_POINT ( 'NONE',  ( 0.1265901696524990294, -0.4724409448818896462, -1.106955380577427706 ) ) ;
#83161=DIRECTION ( 'NONE',  ( 0.000000000000000000, 0.000000000000000000, 1.000000000000000000 ) ) ;
#83166=CARTESIAN_POINT ( 'NONE',  ( 0.2925321140481932369, 0.2925321140481932369, -2.261811023622047223 ) ) ;
#83170=CARTESIAN_POINT ( 'NONE',  ( -0.3460692066303960313, 0.1998031496062989965, -1.520341207349081403 ) ) ;
#83176=CARTESIAN_POINT ( 'NONE',  ( 0.2925321140481931814, 0.2925321140481931814, -0.6870078740157479213 ) ) ;
#83177=CARTESIAN_POINT ( 'NONE',  ( -0.3996062992125987146, 0.1070741851644051862, -0.8202099737532806412 ) ) ;
#83178=CARTESIAN_POINT ( 'NONE',  ( -0.3949938075777409408, -0.1058382717557502933, -0.04593175853018378885 ) ) ;
#83183=CARTESIAN_POINT ( 'NONE',  ( 4.837279021331061486E-17, -0.3949938075777409963, -1.415354330708661346 ) ) ;
#83188=CARTESIAN_POINT ( 'NONE',  ( -1.157146581871515012E-16, 0.4724409448818898682, -1.732283464566929165 ) ) ;
#83197=CARTESIAN_POINT ( 'NONE',  ( 0.1049643490035303689, 0.3917322834645668994, -1.963235277394014267 ) ) ;
#83204=CARTESIAN_POINT ( 'NONE',  ( -0.1958661417322836718, 0.3392501089628017219, -1.580052493438320216 ) ) ;
#83207=CARTESIAN_POINT ( 'NONE',  ( 0.3949938075777409408, 0.1058382717557500574, -1.699475065616798064 ) ) ;
#83212=CARTESIAN_POINT ( 'NONE',  ( 0.3460692066303959757, -0.1998031496062991907, -0.1049868766404199599 ) ) ;
#83220=CARTESIAN_POINT ( 'NONE',  ( 4.797336870675656522E-17, -0.3917322834645670104, -0.4783464566929135353 ) ) ;
#83227=CARTESIAN_POINT ( 'NONE',  ( -0.3996062992125984925, -0.1070741851644056858, -1.854986876640420057 ) ) ;
#83232=CARTESIAN_POINT ( 'NONE',  ( -0.1265901696524986964, -0.4724409448818899238, -0.8595800524934383846 ) ) ;
#83234=CARTESIAN_POINT ( 'NONE',  ( -9.594673741351313045E-17, 0.3917322834645670104, 0.007874015748031542791 ) ) ;
#83239=CARTESIAN_POINT ( 'NONE',  ( 5.785732909357575061E-17, -0.4724409448818898682, -2.832677165354331006 ) ) ;
#83243=CARTESIAN_POINT ( 'NONE',  ( 0.3420746716998660508, 0.1974969037888705814, -2.412729658792650778 ) ) ;
#83250=CARTESIAN_POINT ( 'NONE',  ( 0.1958661417322836440, -0.3392501089628017219, -1.343832020997375531 ) ) ;
#83253=CARTESIAN_POINT ( 'NONE',  ( -1.157146581871515012E-16, 0.4724409448818898682, 0.08070866141732283006 ) ) ;
#83266=CARTESIAN_POINT ( 'NONE',  ( 0.3996062992125984925, 0.1070741851644054637, -1.303805774278215202 ) ) ;
#83267=CARTESIAN_POINT ( 'NONE',  ( -0.3917322834645671215, 0.1049643490035301469, -2.164698162729658648 ) ) ;
#83278=CARTESIAN_POINT ( 'NONE',  ( 0.3392501089628018884, -0.1958661417322833942, -1.991489132054804934 ) ) ;
#83284=CARTESIAN_POINT ( 'NONE',  ( 0.3917322834645669549, 0.1049643490035304660, -1.784120734908136274 ) ) ;
#83285=CARTESIAN_POINT ( 'NONE',  ( -0.2316922116739030535, 0.3165741174739047370, -1.220472440944881498 ) ) ;
#83289=CARTESIAN_POINT ( 'NONE',  ( -0.2925321140481930149, -0.2925321140481933480, -2.655511811023621771 ) ) ;
#83291=CARTESIAN_POINT ( 'NONE',  ( 0.1998031496062992740, 0.3460692066303959757, -1.246719160104986734 ) ) ;
#83292=VERTEX_POINT ( 'NONE', #40691 ) ;
#83293=CARTESIAN_POINT ( 'NONE',  ( -0.3392501089628017219, -0.1958661417322836718, -2.879265091863516979 ) ) ;
#83308=CARTESIAN_POINT ( 'NONE',  ( -0.1958661417322836718, 0.3392501089628017219, -0.1627296587926508609 ) ) ;
#83309=CARTESIAN_POINT ( 'NONE',  ( 0.1998031496062992740, 0.3460692066303959757, -2.506561679790026087 ) ) ;
ENDSEC;
END-ISO-10303-21;
